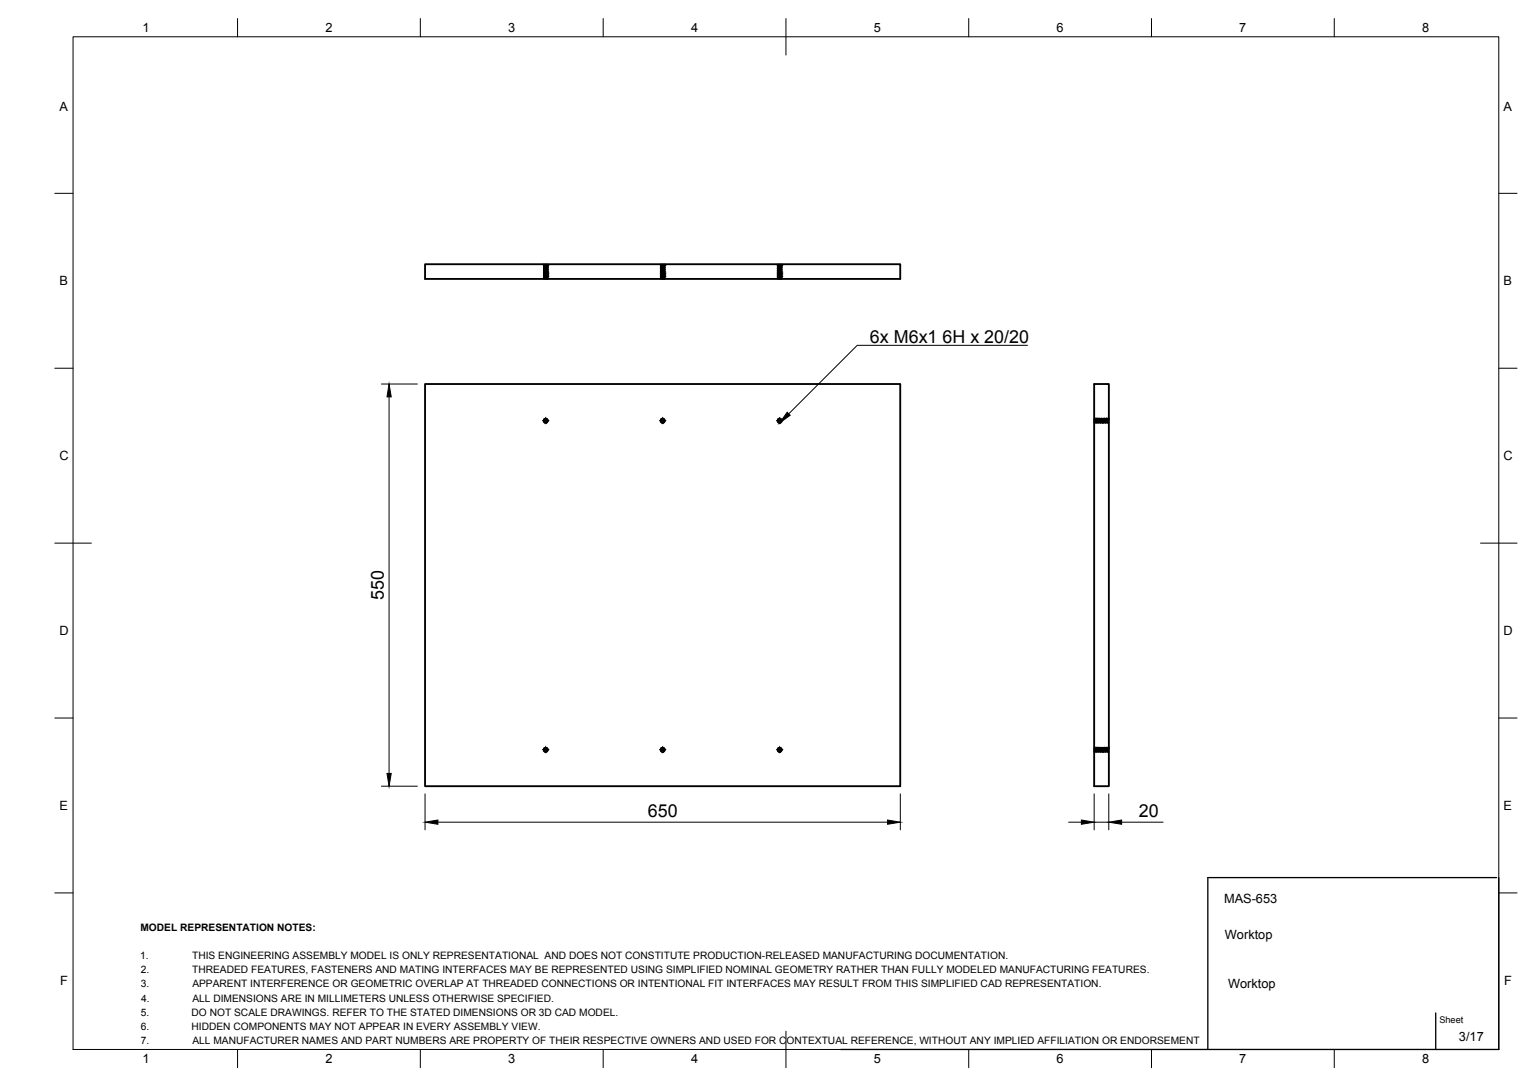
ISO-10303-21;
HEADER;
/* Generated by software containing ST-Developer
 * from STEP Tools, Inc. (www.steptools.com) 
 */

FILE_DESCRIPTION(
/* description */ ('Independent compact industrial fixture table, bolted aluminum worktop
 on connected adjustable support base. Whole-mm nominal dimensions. No
 load rating assigned.'),
/* implementation_level */ '2;1');

FILE_NAME(
/* name */ 'Worktop.step',
/* time_stamp */ '2026-11-07T17:47:58-08:00',
/* author */ (''),
/* organization */ (''),
/* preprocessor_version */ 'ST-DEVELOPER v20.2',
/* originating_system */ 'Autodesk Translation Framework v15.17.0.0',
/* authorisation */ '');

FILE_SCHEMA (('AUTOMOTIVE_DESIGN { 1 0 10303 214 3 1 1 }'));
ENDSEC;

DATA;
#10=MECHANICAL_DESIGN_GEOMETRIC_PRESENTATION_REPRESENTATION('',(#2265),#97475);
#362=B_SPLINE_SURFACE_WITH_KNOTS('',3,3,((#81643,#81644,#81645,#81646,#81647,
#81648,#81649,#81650,#81651,#81652,#81653,#81654,#81655,#81656,#81657,#81658,
#81659,#81660,#81661,#81662,#81663,#81664,#81665,#81666,#81667,#81668,#81669,
#81670,#81671,#81672,#81673,#81674,#81675,#81676,#81677,#81678,#81679,#81680,
#81681,#81682,#81683,#81684,#81685,#81686,#81687,#81688,#81689,#81690,#81691,
#81692,#81693,#81694,#81695,#81696,#81697,#81698,#81699,#81700,#81701,#81702,
#81703,#81704,#81705,#81706,#81707,#81708,#81709,#81710,#81711,#81712,#81713,
#81714,#81715,#81716,#81717,#81718,#81719,#81720,#81721,#81722,#81723,#81724,
#81725,#81726,#81727,#81728,#81729,#81730,#81731,#81732,#81733,#81734,#81735,
#81736,#81737,#81738,#81739,#81740,#81741,#81742,#81743,#81744,#81745,#81746,
#81747,#81748,#81749,#81750,#81751,#81752,#81753,#81754,#81755,#81756,#81757,
#81758,#81759,#81760,#81761,#81762,#81763,#81764,#81765,#81766,#81767,#81768,
#81769,#81770,#81771,#81772,#81773),(#81774,#81775,#81776,#81777,#81778,
#81779,#81780,#81781,#81782,#81783,#81784,#81785,#81786,#81787,#81788,#81789,
#81790,#81791,#81792,#81793,#81794,#81795,#81796,#81797,#81798,#81799,#81800,
#81801,#81802,#81803,#81804,#81805,#81806,#81807,#81808,#81809,#81810,#81811,
#81812,#81813,#81814,#81815,#81816,#81817,#81818,#81819,#81820,#81821,#81822,
#81823,#81824,#81825,#81826,#81827,#81828,#81829,#81830,#81831,#81832,#81833,
#81834,#81835,#81836,#81837,#81838,#81839,#81840,#81841,#81842,#81843,#81844,
#81845,#81846,#81847,#81848,#81849,#81850,#81851,#81852,#81853,#81854,#81855,
#81856,#81857,#81858,#81859,#81860,#81861,#81862,#81863,#81864,#81865,#81866,
#81867,#81868,#81869,#81870,#81871,#81872,#81873,#81874,#81875,#81876,#81877,
#81878,#81879,#81880,#81881,#81882,#81883,#81884,#81885,#81886,#81887,#81888,
#81889,#81890,#81891,#81892,#81893,#81894,#81895,#81896,#81897,#81898,#81899,
#81900,#81901,#81902,#81903,#81904),(#81905,#81906,#81907,#81908,#81909,
#81910,#81911,#81912,#81913,#81914,#81915,#81916,#81917,#81918,#81919,#81920,
#81921,#81922,#81923,#81924,#81925,#81926,#81927,#81928,#81929,#81930,#81931,
#81932,#81933,#81934,#81935,#81936,#81937,#81938,#81939,#81940,#81941,#81942,
#81943,#81944,#81945,#81946,#81947,#81948,#81949,#81950,#81951,#81952,#81953,
#81954,#81955,#81956,#81957,#81958,#81959,#81960,#81961,#81962,#81963,#81964,
#81965,#81966,#81967,#81968,#81969,#81970,#81971,#81972,#81973,#81974,#81975,
#81976,#81977,#81978,#81979,#81980,#81981,#81982,#81983,#81984,#81985,#81986,
#81987,#81988,#81989,#81990,#81991,#81992,#81993,#81994,#81995,#81996,#81997,
#81998,#81999,#82000,#82001,#82002,#82003,#82004,#82005,#82006,#82007,#82008,
#82009,#82010,#82011,#82012,#82013,#82014,#82015,#82016,#82017,#82018,#82019,
#82020,#82021,#82022,#82023,#82024,#82025,#82026,#82027,#82028,#82029,#82030,
#82031,#82032,#82033,#82034,#82035),(#82036,#82037,#82038,#82039,#82040,
#82041,#82042,#82043,#82044,#82045,#82046,#82047,#82048,#82049,#82050,#82051,
#82052,#82053,#82054,#82055,#82056,#82057,#82058,#82059,#82060,#82061,#82062,
#82063,#82064,#82065,#82066,#82067,#82068,#82069,#82070,#82071,#82072,#82073,
#82074,#82075,#82076,#82077,#82078,#82079,#82080,#82081,#82082,#82083,#82084,
#82085,#82086,#82087,#82088,#82089,#82090,#82091,#82092,#82093,#82094,#82095,
#82096,#82097,#82098,#82099,#82100,#82101,#82102,#82103,#82104,#82105,#82106,
#82107,#82108,#82109,#82110,#82111,#82112,#82113,#82114,#82115,#82116,#82117,
#82118,#82119,#82120,#82121,#82122,#82123,#82124,#82125,#82126,#82127,#82128,
#82129,#82130,#82131,#82132,#82133,#82134,#82135,#82136,#82137,#82138,#82139,
#82140,#82141,#82142,#82143,#82144,#82145,#82146,#82147,#82148,#82149,#82150,
#82151,#82152,#82153,#82154,#82155,#82156,#82157,#82158,#82159,#82160,#82161,
#82162,#82163,#82164,#82165,#82166)),.UNSPECIFIED.,.F.,.F.,.F.,(4,4),(4,
1,1,1,1,1,1,1,1,1,1,1,1,1,1,1,1,1,1,1,1,1,1,1,1,1,1,1,1,1,1,1,1,1,1,1,1,
1,1,1,1,1,1,1,1,1,1,1,1,1,1,1,1,1,1,1,1,1,1,1,1,1,1,1,1,1,1,1,1,1,1,1,1,
1,1,1,1,1,1,1,1,1,1,1,1,1,1,1,1,1,1,1,1,1,1,1,1,1,1,1,1,1,1,1,1,1,1,1,1,
1,1,1,1,1,1,1,1,1,1,1,1,1,1,1,1,1,1,1,4),(0.,0.0642013499338863),(11.8589888623077,
12.8564939485313,13.8539990347549,14.8515041209785,15.8490092072021,16.8465142934257,
17.8440193796493,18.8415244658729,19.8390295520965,20.8365346383201,21.8340397245437,
22.8315448107673,23.8290498969909,24.8265549832145,25.8240600694381,26.8215651556617,
27.8190702418853,28.8165753281089,29.8140804143324,30.811585500556,31.8090905867796,
32.8065956730032,33.8041007592268,34.8016058454504,35.799110931674,36.7966160178976,
37.7941211041212,38.7916261903448,39.7891312765684,40.786636362792,41.7841414490156,
42.7816465352392,43.7791516214628,44.7766567076864,45.77416179391,46.7716668801336,
47.7691719663572,48.7666770525807,49.7641821388043,50.7616872250279,51.7591923112515,
52.7566973974751,53.7542024836987,54.7517075699223,55.7492126561459,56.7467177423695,
57.7442228285931,58.7417279148167,59.7392330010403,60.7367380872639,61.7342431734875,
62.7317482597111,63.7292533459347,64.7267584321583,65.7242635183819,66.7217686046055,
67.7192736908291,68.7167787770527,69.7142838632763,70.7117889494998,71.7092940357234,
72.706799121947,73.7043042081706,74.7018092943942,75.6993143806178,76.6968194668414,
77.694324553065,78.6918296392886,79.6893347255122,80.6868398117358,81.6843448979594,
82.681849984183,83.6793550704066,84.6768601566302,85.6743652428538,86.6718703290774,
87.669375415301,88.6668805015246,89.6643855877482,90.6618906739717,91.6593957601953,
92.6569008464189,93.6544059326425,94.6519110188661,95.6494161050897,96.6469211913133,
97.6444262775369,98.6419313637605,99.6394364499841,100.636941536208,101.634446622431,
102.631951708655,103.629456794878,104.626961881102,105.624466967326,106.621972053549,
107.619477139773,108.616982225996,109.61448731222,110.611992398444,111.609497484667,
112.607002570891,113.604507657114,114.602012743338,115.599517829562,116.597022915785,
117.594528002009,118.592033088232,119.589538174456,120.58704326068,121.584548346903,
122.582053433127,123.57955851935,124.577063605574,125.574568691798,126.572073778021,
127.569578864245,128.567083950468,129.564589036692,130.562094122916,131.559599209139,
132.557104295363,133.554609381586,134.55211446781,135.549619554034,136.547124640257,
137.544629726481,138.542134812704,139.539639898928),.UNSPECIFIED.);
#363=B_SPLINE_SURFACE_WITH_KNOTS('',3,3,((#82380,#82381,#82382,#82383,#82384,
#82385,#82386,#82387,#82388,#82389,#82390,#82391,#82392,#82393,#82394,#82395,
#82396,#82397,#82398,#82399,#82400,#82401,#82402,#82403,#82404,#82405,#82406,
#82407,#82408,#82409,#82410,#82411,#82412,#82413,#82414,#82415,#82416,#82417,
#82418,#82419,#82420,#82421,#82422,#82423,#82424,#82425,#82426,#82427,#82428,
#82429,#82430,#82431,#82432,#82433,#82434,#82435,#82436,#82437,#82438,#82439,
#82440,#82441,#82442,#82443,#82444,#82445,#82446,#82447,#82448,#82449,#82450,
#82451,#82452,#82453,#82454,#82455,#82456,#82457,#82458,#82459,#82460,#82461,
#82462,#82463,#82464,#82465,#82466,#82467,#82468,#82469,#82470,#82471,#82472,
#82473,#82474,#82475,#82476,#82477,#82478,#82479,#82480,#82481,#82482,#82483,
#82484,#82485,#82486,#82487,#82488,#82489,#82490,#82491,#82492,#82493,#82494,
#82495,#82496,#82497,#82498,#82499,#82500,#82501,#82502,#82503,#82504,#82505,
#82506,#82507,#82508,#82509,#82510),(#82511,#82512,#82513,#82514,#82515,
#82516,#82517,#82518,#82519,#82520,#82521,#82522,#82523,#82524,#82525,#82526,
#82527,#82528,#82529,#82530,#82531,#82532,#82533,#82534,#82535,#82536,#82537,
#82538,#82539,#82540,#82541,#82542,#82543,#82544,#82545,#82546,#82547,#82548,
#82549,#82550,#82551,#82552,#82553,#82554,#82555,#82556,#82557,#82558,#82559,
#82560,#82561,#82562,#82563,#82564,#82565,#82566,#82567,#82568,#82569,#82570,
#82571,#82572,#82573,#82574,#82575,#82576,#82577,#82578,#82579,#82580,#82581,
#82582,#82583,#82584,#82585,#82586,#82587,#82588,#82589,#82590,#82591,#82592,
#82593,#82594,#82595,#82596,#82597,#82598,#82599,#82600,#82601,#82602,#82603,
#82604,#82605,#82606,#82607,#82608,#82609,#82610,#82611,#82612,#82613,#82614,
#82615,#82616,#82617,#82618,#82619,#82620,#82621,#82622,#82623,#82624,#82625,
#82626,#82627,#82628,#82629,#82630,#82631,#82632,#82633,#82634,#82635,#82636,
#82637,#82638,#82639,#82640,#82641),(#82642,#82643,#82644,#82645,#82646,
#82647,#82648,#82649,#82650,#82651,#82652,#82653,#82654,#82655,#82656,#82657,
#82658,#82659,#82660,#82661,#82662,#82663,#82664,#82665,#82666,#82667,#82668,
#82669,#82670,#82671,#82672,#82673,#82674,#82675,#82676,#82677,#82678,#82679,
#82680,#82681,#82682,#82683,#82684,#82685,#82686,#82687,#82688,#82689,#82690,
#82691,#82692,#82693,#82694,#82695,#82696,#82697,#82698,#82699,#82700,#82701,
#82702,#82703,#82704,#82705,#82706,#82707,#82708,#82709,#82710,#82711,#82712,
#82713,#82714,#82715,#82716,#82717,#82718,#82719,#82720,#82721,#82722,#82723,
#82724,#82725,#82726,#82727,#82728,#82729,#82730,#82731,#82732,#82733,#82734,
#82735,#82736,#82737,#82738,#82739,#82740,#82741,#82742,#82743,#82744,#82745,
#82746,#82747,#82748,#82749,#82750,#82751,#82752,#82753,#82754,#82755,#82756,
#82757,#82758,#82759,#82760,#82761,#82762,#82763,#82764,#82765,#82766,#82767,
#82768,#82769,#82770,#82771,#82772),(#82773,#82774,#82775,#82776,#82777,
#82778,#82779,#82780,#82781,#82782,#82783,#82784,#82785,#82786,#82787,#82788,
#82789,#82790,#82791,#82792,#82793,#82794,#82795,#82796,#82797,#82798,#82799,
#82800,#82801,#82802,#82803,#82804,#82805,#82806,#82807,#82808,#82809,#82810,
#82811,#82812,#82813,#82814,#82815,#82816,#82817,#82818,#82819,#82820,#82821,
#82822,#82823,#82824,#82825,#82826,#82827,#82828,#82829,#82830,#82831,#82832,
#82833,#82834,#82835,#82836,#82837,#82838,#82839,#82840,#82841,#82842,#82843,
#82844,#82845,#82846,#82847,#82848,#82849,#82850,#82851,#82852,#82853,#82854,
#82855,#82856,#82857,#82858,#82859,#82860,#82861,#82862,#82863,#82864,#82865,
#82866,#82867,#82868,#82869,#82870,#82871,#82872,#82873,#82874,#82875,#82876,
#82877,#82878,#82879,#82880,#82881,#82882,#82883,#82884,#82885,#82886,#82887,
#82888,#82889,#82890,#82891,#82892,#82893,#82894,#82895,#82896,#82897,#82898,
#82899,#82900,#82901,#82902,#82903)),.UNSPECIFIED.,.F.,.F.,.F.,(4,4),(4,
1,1,1,1,1,1,1,1,1,1,1,1,1,1,1,1,1,1,1,1,1,1,1,1,1,1,1,1,1,1,1,1,1,1,1,1,
1,1,1,1,1,1,1,1,1,1,1,1,1,1,1,1,1,1,1,1,1,1,1,1,1,1,1,1,1,1,1,1,1,1,1,1,
1,1,1,1,1,1,1,1,1,1,1,1,1,1,1,1,1,1,1,1,1,1,1,1,1,1,1,1,1,1,1,1,1,1,1,1,
1,1,1,1,1,1,1,1,1,1,1,1,1,1,1,1,1,1,1,4),(0.,0.0642013499338863),(14.3984001269718,
15.3959052131954,16.393410299419,17.3909153856426,18.3884204718662,19.3859255580897,
20.3834306443133,21.3809357305369,22.3784408167605,23.3759459029841,24.3734509892077,
25.3709560754313,26.3684611616549,27.3659662478785,28.3634713341021,29.3609764203257,
30.3584815065493,31.3559865927729,32.3534916789965,33.3509967652201,34.3485018514437,
35.3460069376673,36.3435120238909,37.3410171101145,38.3385221963381,39.3360272825616,
40.3335323687852,41.3310374550088,42.3285425412324,43.326047627456,44.3235527136796,
45.3210577999032,46.3185628861268,47.3160679723504,48.313573058574,49.3110781447976,
50.3085832310212,51.3060883172448,52.3035934034684,53.301098489692,54.2986035759156,
55.2961086621392,56.2936137483628,57.2911188345864,58.28862392081,59.2861290070336,
60.2836340932571,61.2811391794807,62.2786442657043,63.2761493519279,64.2736544381515,
65.2711595243751,66.2686646105987,67.2661696968223,68.2636747830459,69.2611798692695,
70.2586849554931,71.2561900417167,72.2536951279403,73.2512002141639,74.2487053003875,
75.2462103866111,76.2437154728347,77.2412205590583,78.2387256452818,79.2362307315055,
80.233735817729,81.2312409039526,82.2287459901762,83.2262510763998,84.2237561626234,
85.221261248847,86.2187663350706,87.2162714212942,88.2137765075178,89.2112815937414,
90.208786679965,91.2062917661886,92.2037968524122,93.2013019386358,94.1988070248594,
95.196312111083,96.1938171973066,97.1913222835302,98.1888273697538,99.1863324559774,
100.183837542201,101.181342628425,102.178847714648,103.176352800872,104.173857887095,
105.171362973319,106.168868059543,107.166373145766,108.16387823199,109.161383318213,
110.158888404437,111.15639349066,112.153898576884,113.151403663108,114.148908749331,
115.146413835555,116.143918921778,117.141424008002,118.138929094226,119.136434180449,
120.133939266673,121.131444352896,122.12894943912,123.126454525344,124.123959611567,
125.121464697791,126.118969784014,127.116474870238,128.113979956462,129.111485042685,
130.108990128909,131.106495215132,132.104000301356,133.10150538758,134.099010473803,
135.096515560027,136.09402064625,137.091525732474,138.089030818698,139.086535904921,
140.084040991145,141.081546077368,142.079051163592),.UNSPECIFIED.);
#364=B_SPLINE_SURFACE_WITH_KNOTS('',3,3,((#84085,#84086,#84087,#84088,#84089,
#84090,#84091,#84092,#84093,#84094,#84095,#84096,#84097,#84098,#84099,#84100,
#84101,#84102,#84103,#84104,#84105,#84106,#84107,#84108,#84109,#84110,#84111,
#84112,#84113,#84114,#84115,#84116,#84117,#84118,#84119,#84120,#84121,#84122,
#84123,#84124,#84125,#84126,#84127,#84128,#84129,#84130,#84131,#84132,#84133,
#84134,#84135,#84136,#84137,#84138,#84139,#84140,#84141,#84142,#84143,#84144,
#84145,#84146,#84147,#84148,#84149,#84150,#84151,#84152,#84153,#84154,#84155,
#84156,#84157,#84158,#84159,#84160,#84161,#84162,#84163,#84164,#84165,#84166,
#84167,#84168,#84169,#84170,#84171,#84172,#84173,#84174,#84175,#84176,#84177,
#84178,#84179,#84180,#84181,#84182,#84183,#84184,#84185,#84186,#84187,#84188,
#84189,#84190,#84191,#84192,#84193,#84194,#84195,#84196,#84197,#84198,#84199,
#84200,#84201,#84202,#84203,#84204,#84205,#84206,#84207,#84208,#84209,#84210,
#84211,#84212,#84213,#84214,#84215),(#84216,#84217,#84218,#84219,#84220,
#84221,#84222,#84223,#84224,#84225,#84226,#84227,#84228,#84229,#84230,#84231,
#84232,#84233,#84234,#84235,#84236,#84237,#84238,#84239,#84240,#84241,#84242,
#84243,#84244,#84245,#84246,#84247,#84248,#84249,#84250,#84251,#84252,#84253,
#84254,#84255,#84256,#84257,#84258,#84259,#84260,#84261,#84262,#84263,#84264,
#84265,#84266,#84267,#84268,#84269,#84270,#84271,#84272,#84273,#84274,#84275,
#84276,#84277,#84278,#84279,#84280,#84281,#84282,#84283,#84284,#84285,#84286,
#84287,#84288,#84289,#84290,#84291,#84292,#84293,#84294,#84295,#84296,#84297,
#84298,#84299,#84300,#84301,#84302,#84303,#84304,#84305,#84306,#84307,#84308,
#84309,#84310,#84311,#84312,#84313,#84314,#84315,#84316,#84317,#84318,#84319,
#84320,#84321,#84322,#84323,#84324,#84325,#84326,#84327,#84328,#84329,#84330,
#84331,#84332,#84333,#84334,#84335,#84336,#84337,#84338,#84339,#84340,#84341,
#84342,#84343,#84344,#84345,#84346),(#84347,#84348,#84349,#84350,#84351,
#84352,#84353,#84354,#84355,#84356,#84357,#84358,#84359,#84360,#84361,#84362,
#84363,#84364,#84365,#84366,#84367,#84368,#84369,#84370,#84371,#84372,#84373,
#84374,#84375,#84376,#84377,#84378,#84379,#84380,#84381,#84382,#84383,#84384,
#84385,#84386,#84387,#84388,#84389,#84390,#84391,#84392,#84393,#84394,#84395,
#84396,#84397,#84398,#84399,#84400,#84401,#84402,#84403,#84404,#84405,#84406,
#84407,#84408,#84409,#84410,#84411,#84412,#84413,#84414,#84415,#84416,#84417,
#84418,#84419,#84420,#84421,#84422,#84423,#84424,#84425,#84426,#84427,#84428,
#84429,#84430,#84431,#84432,#84433,#84434,#84435,#84436,#84437,#84438,#84439,
#84440,#84441,#84442,#84443,#84444,#84445,#84446,#84447,#84448,#84449,#84450,
#84451,#84452,#84453,#84454,#84455,#84456,#84457,#84458,#84459,#84460,#84461,
#84462,#84463,#84464,#84465,#84466,#84467,#84468,#84469,#84470,#84471,#84472,
#84473,#84474,#84475,#84476,#84477),(#84478,#84479,#84480,#84481,#84482,
#84483,#84484,#84485,#84486,#84487,#84488,#84489,#84490,#84491,#84492,#84493,
#84494,#84495,#84496,#84497,#84498,#84499,#84500,#84501,#84502,#84503,#84504,
#84505,#84506,#84507,#84508,#84509,#84510,#84511,#84512,#84513,#84514,#84515,
#84516,#84517,#84518,#84519,#84520,#84521,#84522,#84523,#84524,#84525,#84526,
#84527,#84528,#84529,#84530,#84531,#84532,#84533,#84534,#84535,#84536,#84537,
#84538,#84539,#84540,#84541,#84542,#84543,#84544,#84545,#84546,#84547,#84548,
#84549,#84550,#84551,#84552,#84553,#84554,#84555,#84556,#84557,#84558,#84559,
#84560,#84561,#84562,#84563,#84564,#84565,#84566,#84567,#84568,#84569,#84570,
#84571,#84572,#84573,#84574,#84575,#84576,#84577,#84578,#84579,#84580,#84581,
#84582,#84583,#84584,#84585,#84586,#84587,#84588,#84589,#84590,#84591,#84592,
#84593,#84594,#84595,#84596,#84597,#84598,#84599,#84600,#84601,#84602,#84603,
#84604,#84605,#84606,#84607,#84608)),.UNSPECIFIED.,.F.,.F.,.F.,(4,4),(4,
1,1,1,1,1,1,1,1,1,1,1,1,1,1,1,1,1,1,1,1,1,1,1,1,1,1,1,1,1,1,1,1,1,1,1,1,
1,1,1,1,1,1,1,1,1,1,1,1,1,1,1,1,1,1,1,1,1,1,1,1,1,1,1,1,1,1,1,1,1,1,1,1,
1,1,1,1,1,1,1,1,1,1,1,1,1,1,1,1,1,1,1,1,1,1,1,1,1,1,1,1,1,1,1,1,1,1,1,1,
1,1,1,1,1,1,1,1,1,1,1,1,1,1,1,1,1,1,1,4),(0.,0.0642013499338864),(11.8589888623077,
12.8564939485313,13.8539990347549,14.8515041209785,15.8490092072021,16.8465142934257,
17.8440193796493,18.8415244658729,19.8390295520965,20.8365346383201,21.8340397245437,
22.8315448107673,23.8290498969909,24.8265549832144,25.824060069438,26.8215651556616,
27.8190702418852,28.8165753281088,29.8140804143324,30.811585500556,31.8090905867796,
32.8065956730032,33.8041007592268,34.8016058454504,35.799110931674,36.7966160178976,
37.7941211041212,38.7916261903448,39.7891312765684,40.786636362792,41.7841414490156,
42.7816465352392,43.7791516214628,44.7766567076863,45.7741617939099,46.7716668801335,
47.7691719663571,48.7666770525807,49.7641821388043,50.7616872250279,51.7591923112515,
52.7566973974751,53.7542024836987,54.7517075699223,55.7492126561459,56.7467177423695,
57.7442228285931,58.7417279148167,59.7392330010403,60.7367380872639,61.7342431734875,
62.7317482597111,63.7292533459347,64.7267584321582,65.7242635183818,66.7217686046054,
67.719273690829,68.7167787770526,69.7142838632762,70.7117889494998,71.7092940357234,
72.706799121947,73.7043042081706,74.7018092943942,75.6993143806178,76.6968194668414,
77.694324553065,78.6918296392886,79.6893347255122,80.6868398117358,81.6843448979594,
82.681849984183,83.6793550704066,84.6768601566301,85.6743652428537,86.6718703290773,
87.6693754153009,88.6668805015245,89.6643855877481,90.6618906739717,91.6593957601953,
92.6569008464189,93.6544059326425,94.6519110188661,95.6494161050897,96.6469211913133,
97.6444262775369,98.6419313637605,99.6394364499841,100.636941536208,101.634446622431,
102.631951708655,103.629456794878,104.626961881102,105.624466967326,106.621972053549,
107.619477139773,108.616982225996,109.61448731222,110.611992398444,111.609497484667,
112.607002570891,113.604507657114,114.602012743338,115.599517829562,116.597022915785,
117.594528002009,118.592033088232,119.589538174456,120.58704326068,121.584548346903,
122.582053433127,123.57955851935,124.577063605574,125.574568691798,126.572073778021,
127.569578864245,128.567083950468,129.564589036692,130.562094122916,131.559599209139,
132.557104295363,133.554609381586,134.55211446781,135.549619554033,136.547124640257,
137.544629726481,138.542134812704,139.539639898928),.UNSPECIFIED.);
#365=B_SPLINE_SURFACE_WITH_KNOTS('',3,3,((#84728,#84729,#84730,#84731,#84732,
#84733,#84734,#84735,#84736,#84737,#84738,#84739,#84740,#84741,#84742,#84743,
#84744,#84745,#84746,#84747,#84748,#84749,#84750,#84751,#84752,#84753,#84754,
#84755,#84756,#84757,#84758,#84759,#84760,#84761,#84762,#84763,#84764,#84765,
#84766,#84767,#84768,#84769,#84770,#84771,#84772,#84773,#84774,#84775,#84776,
#84777,#84778,#84779,#84780,#84781,#84782,#84783,#84784,#84785,#84786,#84787,
#84788,#84789,#84790,#84791,#84792,#84793,#84794,#84795,#84796,#84797,#84798,
#84799,#84800,#84801,#84802,#84803,#84804,#84805,#84806,#84807,#84808,#84809,
#84810,#84811,#84812,#84813,#84814,#84815,#84816,#84817,#84818,#84819,#84820,
#84821,#84822,#84823,#84824,#84825,#84826,#84827,#84828,#84829,#84830,#84831,
#84832,#84833,#84834,#84835,#84836,#84837,#84838,#84839,#84840,#84841,#84842,
#84843,#84844,#84845,#84846,#84847,#84848,#84849,#84850,#84851,#84852,#84853,
#84854,#84855,#84856,#84857,#84858),(#84859,#84860,#84861,#84862,#84863,
#84864,#84865,#84866,#84867,#84868,#84869,#84870,#84871,#84872,#84873,#84874,
#84875,#84876,#84877,#84878,#84879,#84880,#84881,#84882,#84883,#84884,#84885,
#84886,#84887,#84888,#84889,#84890,#84891,#84892,#84893,#84894,#84895,#84896,
#84897,#84898,#84899,#84900,#84901,#84902,#84903,#84904,#84905,#84906,#84907,
#84908,#84909,#84910,#84911,#84912,#84913,#84914,#84915,#84916,#84917,#84918,
#84919,#84920,#84921,#84922,#84923,#84924,#84925,#84926,#84927,#84928,#84929,
#84930,#84931,#84932,#84933,#84934,#84935,#84936,#84937,#84938,#84939,#84940,
#84941,#84942,#84943,#84944,#84945,#84946,#84947,#84948,#84949,#84950,#84951,
#84952,#84953,#84954,#84955,#84956,#84957,#84958,#84959,#84960,#84961,#84962,
#84963,#84964,#84965,#84966,#84967,#84968,#84969,#84970,#84971,#84972,#84973,
#84974,#84975,#84976,#84977,#84978,#84979,#84980,#84981,#84982,#84983,#84984,
#84985,#84986,#84987,#84988,#84989),(#84990,#84991,#84992,#84993,#84994,
#84995,#84996,#84997,#84998,#84999,#85000,#85001,#85002,#85003,#85004,#85005,
#85006,#85007,#85008,#85009,#85010,#85011,#85012,#85013,#85014,#85015,#85016,
#85017,#85018,#85019,#85020,#85021,#85022,#85023,#85024,#85025,#85026,#85027,
#85028,#85029,#85030,#85031,#85032,#85033,#85034,#85035,#85036,#85037,#85038,
#85039,#85040,#85041,#85042,#85043,#85044,#85045,#85046,#85047,#85048,#85049,
#85050,#85051,#85052,#85053,#85054,#85055,#85056,#85057,#85058,#85059,#85060,
#85061,#85062,#85063,#85064,#85065,#85066,#85067,#85068,#85069,#85070,#85071,
#85072,#85073,#85074,#85075,#85076,#85077,#85078,#85079,#85080,#85081,#85082,
#85083,#85084,#85085,#85086,#85087,#85088,#85089,#85090,#85091,#85092,#85093,
#85094,#85095,#85096,#85097,#85098,#85099,#85100,#85101,#85102,#85103,#85104,
#85105,#85106,#85107,#85108,#85109,#85110,#85111,#85112,#85113,#85114,#85115,
#85116,#85117,#85118,#85119,#85120),(#85121,#85122,#85123,#85124,#85125,
#85126,#85127,#85128,#85129,#85130,#85131,#85132,#85133,#85134,#85135,#85136,
#85137,#85138,#85139,#85140,#85141,#85142,#85143,#85144,#85145,#85146,#85147,
#85148,#85149,#85150,#85151,#85152,#85153,#85154,#85155,#85156,#85157,#85158,
#85159,#85160,#85161,#85162,#85163,#85164,#85165,#85166,#85167,#85168,#85169,
#85170,#85171,#85172,#85173,#85174,#85175,#85176,#85177,#85178,#85179,#85180,
#85181,#85182,#85183,#85184,#85185,#85186,#85187,#85188,#85189,#85190,#85191,
#85192,#85193,#85194,#85195,#85196,#85197,#85198,#85199,#85200,#85201,#85202,
#85203,#85204,#85205,#85206,#85207,#85208,#85209,#85210,#85211,#85212,#85213,
#85214,#85215,#85216,#85217,#85218,#85219,#85220,#85221,#85222,#85223,#85224,
#85225,#85226,#85227,#85228,#85229,#85230,#85231,#85232,#85233,#85234,#85235,
#85236,#85237,#85238,#85239,#85240,#85241,#85242,#85243,#85244,#85245,#85246,
#85247,#85248,#85249,#85250,#85251)),.UNSPECIFIED.,.F.,.F.,.F.,(4,4),(4,
1,1,1,1,1,1,1,1,1,1,1,1,1,1,1,1,1,1,1,1,1,1,1,1,1,1,1,1,1,1,1,1,1,1,1,1,
1,1,1,1,1,1,1,1,1,1,1,1,1,1,1,1,1,1,1,1,1,1,1,1,1,1,1,1,1,1,1,1,1,1,1,1,
1,1,1,1,1,1,1,1,1,1,1,1,1,1,1,1,1,1,1,1,1,1,1,1,1,1,1,1,1,1,1,1,1,1,1,1,
1,1,1,1,1,1,1,1,1,1,1,1,1,1,1,1,1,1,1,4),(0.,0.0642013499338864),(14.3984001269717,
15.3959052131953,16.3934102994189,17.3909153856425,18.3884204718661,19.3859255580897,
20.3834306443133,21.3809357305369,22.3784408167605,23.3759459029841,24.3734509892077,
25.3709560754313,26.3684611616549,27.3659662478785,28.3634713341021,29.3609764203257,
30.3584815065493,31.3559865927729,32.3534916789965,33.3509967652201,34.3485018514437,
35.3460069376672,36.3435120238908,37.3410171101144,38.338522196338,39.3360272825616,
40.3335323687852,41.3310374550088,42.3285425412324,43.326047627456,44.3235527136796,
45.3210577999032,46.3185628861268,47.3160679723504,48.313573058574,49.3110781447976,
50.3085832310212,51.3060883172448,52.3035934034684,53.301098489692,54.2986035759156,
55.2961086621392,56.2936137483628,57.2911188345863,58.2886239208099,59.2861290070335,
60.2836340932571,61.2811391794807,62.2786442657043,63.2761493519279,64.2736544381515,
65.2711595243751,66.2686646105987,67.2661696968223,68.2636747830459,69.2611798692695,
70.2586849554931,71.2561900417167,72.2536951279403,73.2512002141639,74.2487053003875,
75.2462103866111,76.2437154728347,77.2412205590582,78.2387256452818,79.2362307315054,
80.233735817729,81.2312409039526,82.2287459901762,83.2262510763998,84.2237561626234,
85.221261248847,86.2187663350706,87.2162714212942,88.2137765075178,89.2112815937414,
90.208786679965,91.2062917661886,92.2037968524122,93.2013019386358,94.1988070248594,
95.196312111083,96.1938171973066,97.1913222835302,98.1888273697538,99.1863324559773,
100.183837542201,101.181342628425,102.178847714648,103.176352800872,104.173857887095,
105.171362973319,106.168868059543,107.166373145766,108.16387823199,109.161383318213,
110.158888404437,111.15639349066,112.153898576884,113.151403663108,114.148908749331,
115.146413835555,116.143918921778,117.141424008002,118.138929094226,119.136434180449,
120.133939266673,121.131444352896,122.12894943912,123.126454525344,124.123959611567,
125.121464697791,126.118969784014,127.116474870238,128.113979956462,129.111485042685,
130.108990128909,131.106495215132,132.104000301356,133.10150538758,134.099010473803,
135.096515560027,136.09402064625,137.091525732474,138.089030818698,139.086535904921,
140.084040991145,141.081546077368,142.079051163592),.UNSPECIFIED.);
#366=B_SPLINE_SURFACE_WITH_KNOTS('',3,3,((#85390,#85391,#85392,#85393,#85394,
#85395,#85396,#85397,#85398,#85399,#85400,#85401,#85402,#85403,#85404,#85405,
#85406,#85407,#85408,#85409,#85410,#85411,#85412,#85413,#85414,#85415,#85416,
#85417,#85418,#85419,#85420,#85421,#85422,#85423,#85424,#85425,#85426,#85427,
#85428,#85429,#85430,#85431,#85432,#85433,#85434,#85435,#85436,#85437,#85438,
#85439,#85440,#85441,#85442,#85443,#85444,#85445,#85446,#85447,#85448,#85449,
#85450,#85451,#85452,#85453,#85454,#85455,#85456,#85457,#85458,#85459,#85460,
#85461,#85462,#85463,#85464,#85465,#85466,#85467,#85468,#85469,#85470,#85471,
#85472,#85473,#85474,#85475,#85476,#85477,#85478,#85479,#85480,#85481,#85482,
#85483,#85484,#85485,#85486,#85487,#85488,#85489,#85490,#85491,#85492,#85493,
#85494,#85495,#85496,#85497,#85498,#85499,#85500,#85501,#85502,#85503,#85504,
#85505,#85506,#85507,#85508,#85509,#85510,#85511,#85512,#85513,#85514,#85515,
#85516,#85517,#85518,#85519,#85520),(#85521,#85522,#85523,#85524,#85525,
#85526,#85527,#85528,#85529,#85530,#85531,#85532,#85533,#85534,#85535,#85536,
#85537,#85538,#85539,#85540,#85541,#85542,#85543,#85544,#85545,#85546,#85547,
#85548,#85549,#85550,#85551,#85552,#85553,#85554,#85555,#85556,#85557,#85558,
#85559,#85560,#85561,#85562,#85563,#85564,#85565,#85566,#85567,#85568,#85569,
#85570,#85571,#85572,#85573,#85574,#85575,#85576,#85577,#85578,#85579,#85580,
#85581,#85582,#85583,#85584,#85585,#85586,#85587,#85588,#85589,#85590,#85591,
#85592,#85593,#85594,#85595,#85596,#85597,#85598,#85599,#85600,#85601,#85602,
#85603,#85604,#85605,#85606,#85607,#85608,#85609,#85610,#85611,#85612,#85613,
#85614,#85615,#85616,#85617,#85618,#85619,#85620,#85621,#85622,#85623,#85624,
#85625,#85626,#85627,#85628,#85629,#85630,#85631,#85632,#85633,#85634,#85635,
#85636,#85637,#85638,#85639,#85640,#85641,#85642,#85643,#85644,#85645,#85646,
#85647,#85648,#85649,#85650,#85651),(#85652,#85653,#85654,#85655,#85656,
#85657,#85658,#85659,#85660,#85661,#85662,#85663,#85664,#85665,#85666,#85667,
#85668,#85669,#85670,#85671,#85672,#85673,#85674,#85675,#85676,#85677,#85678,
#85679,#85680,#85681,#85682,#85683,#85684,#85685,#85686,#85687,#85688,#85689,
#85690,#85691,#85692,#85693,#85694,#85695,#85696,#85697,#85698,#85699,#85700,
#85701,#85702,#85703,#85704,#85705,#85706,#85707,#85708,#85709,#85710,#85711,
#85712,#85713,#85714,#85715,#85716,#85717,#85718,#85719,#85720,#85721,#85722,
#85723,#85724,#85725,#85726,#85727,#85728,#85729,#85730,#85731,#85732,#85733,
#85734,#85735,#85736,#85737,#85738,#85739,#85740,#85741,#85742,#85743,#85744,
#85745,#85746,#85747,#85748,#85749,#85750,#85751,#85752,#85753,#85754,#85755,
#85756,#85757,#85758,#85759,#85760,#85761,#85762,#85763,#85764,#85765,#85766,
#85767,#85768,#85769,#85770,#85771,#85772,#85773,#85774,#85775,#85776,#85777,
#85778,#85779,#85780,#85781,#85782),(#85783,#85784,#85785,#85786,#85787,
#85788,#85789,#85790,#85791,#85792,#85793,#85794,#85795,#85796,#85797,#85798,
#85799,#85800,#85801,#85802,#85803,#85804,#85805,#85806,#85807,#85808,#85809,
#85810,#85811,#85812,#85813,#85814,#85815,#85816,#85817,#85818,#85819,#85820,
#85821,#85822,#85823,#85824,#85825,#85826,#85827,#85828,#85829,#85830,#85831,
#85832,#85833,#85834,#85835,#85836,#85837,#85838,#85839,#85840,#85841,#85842,
#85843,#85844,#85845,#85846,#85847,#85848,#85849,#85850,#85851,#85852,#85853,
#85854,#85855,#85856,#85857,#85858,#85859,#85860,#85861,#85862,#85863,#85864,
#85865,#85866,#85867,#85868,#85869,#85870,#85871,#85872,#85873,#85874,#85875,
#85876,#85877,#85878,#85879,#85880,#85881,#85882,#85883,#85884,#85885,#85886,
#85887,#85888,#85889,#85890,#85891,#85892,#85893,#85894,#85895,#85896,#85897,
#85898,#85899,#85900,#85901,#85902,#85903,#85904,#85905,#85906,#85907,#85908,
#85909,#85910,#85911,#85912,#85913)),.UNSPECIFIED.,.F.,.F.,.F.,(4,4),(4,
1,1,1,1,1,1,1,1,1,1,1,1,1,1,1,1,1,1,1,1,1,1,1,1,1,1,1,1,1,1,1,1,1,1,1,1,
1,1,1,1,1,1,1,1,1,1,1,1,1,1,1,1,1,1,1,1,1,1,1,1,1,1,1,1,1,1,1,1,1,1,1,1,
1,1,1,1,1,1,1,1,1,1,1,1,1,1,1,1,1,1,1,1,1,1,1,1,1,1,1,1,1,1,1,1,1,1,1,1,
1,1,1,1,1,1,1,1,1,1,1,1,1,1,1,1,1,1,1,4),(0.,0.0642013499338879),(11.8589888623077,
12.8564939485313,13.8539990347549,14.8515041209785,15.8490092072021,16.8465142934257,
17.8440193796493,18.8415244658729,19.8390295520965,20.8365346383201,21.8340397245437,
22.8315448107673,23.8290498969909,24.8265549832145,25.8240600694381,26.8215651556617,
27.8190702418853,28.8165753281089,29.8140804143324,30.811585500556,31.8090905867796,
32.8065956730032,33.8041007592268,34.8016058454504,35.799110931674,36.7966160178976,
37.7941211041212,38.7916261903448,39.7891312765684,40.786636362792,41.7841414490156,
42.7816465352392,43.7791516214628,44.7766567076864,45.77416179391,46.7716668801336,
47.7691719663572,48.7666770525808,49.7641821388044,50.7616872250279,51.7591923112515,
52.7566973974751,53.7542024836987,54.7517075699223,55.7492126561459,56.7467177423695,
57.7442228285931,58.7417279148167,59.7392330010403,60.7367380872639,61.7342431734875,
62.7317482597111,63.7292533459347,64.7267584321583,65.7242635183819,66.7217686046055,
67.7192736908291,68.7167787770527,69.7142838632763,70.7117889494998,71.7092940357234,
72.706799121947,73.7043042081706,74.7018092943942,75.6993143806178,76.6968194668414,
77.694324553065,78.6918296392886,79.6893347255122,80.6868398117358,81.6843448979594,
82.681849984183,83.6793550704066,84.6768601566302,85.6743652428538,86.6718703290774,
87.669375415301,88.6668805015246,89.6643855877482,90.6618906739718,91.6593957601954,
92.6569008464189,93.6544059326425,94.6519110188661,95.6494161050897,96.6469211913133,
97.6444262775369,98.6419313637605,99.6394364499841,100.636941536208,101.634446622431,
102.631951708655,103.629456794878,104.626961881102,105.624466967326,106.621972053549,
107.619477139773,108.616982225996,109.61448731222,110.611992398444,111.609497484667,
112.607002570891,113.604507657114,114.602012743338,115.599517829562,116.597022915785,
117.594528002009,118.592033088232,119.589538174456,120.58704326068,121.584548346903,
122.582053433127,123.57955851935,124.577063605574,125.574568691798,126.572073778021,
127.569578864245,128.567083950468,129.564589036692,130.562094122916,131.559599209139,
132.557104295363,133.554609381586,134.55211446781,135.549619554034,136.547124640257,
137.544629726481,138.542134812704,139.539639898928),.UNSPECIFIED.);
#367=B_SPLINE_SURFACE_WITH_KNOTS('',3,3,((#86033,#86034,#86035,#86036,#86037,
#86038,#86039,#86040,#86041,#86042,#86043,#86044,#86045,#86046,#86047,#86048,
#86049,#86050,#86051,#86052,#86053,#86054,#86055,#86056,#86057,#86058,#86059,
#86060,#86061,#86062,#86063,#86064,#86065,#86066,#86067,#86068,#86069,#86070,
#86071,#86072,#86073,#86074,#86075,#86076,#86077,#86078,#86079,#86080,#86081,
#86082,#86083,#86084,#86085,#86086,#86087,#86088,#86089,#86090,#86091,#86092,
#86093,#86094,#86095,#86096,#86097,#86098,#86099,#86100,#86101,#86102,#86103,
#86104,#86105,#86106,#86107,#86108,#86109,#86110,#86111,#86112,#86113,#86114,
#86115,#86116,#86117,#86118,#86119,#86120,#86121,#86122,#86123,#86124,#86125,
#86126,#86127,#86128,#86129,#86130,#86131,#86132,#86133,#86134,#86135,#86136,
#86137,#86138,#86139,#86140,#86141,#86142,#86143,#86144,#86145,#86146,#86147,
#86148,#86149,#86150,#86151,#86152,#86153,#86154,#86155,#86156,#86157,#86158,
#86159,#86160,#86161,#86162,#86163),(#86164,#86165,#86166,#86167,#86168,
#86169,#86170,#86171,#86172,#86173,#86174,#86175,#86176,#86177,#86178,#86179,
#86180,#86181,#86182,#86183,#86184,#86185,#86186,#86187,#86188,#86189,#86190,
#86191,#86192,#86193,#86194,#86195,#86196,#86197,#86198,#86199,#86200,#86201,
#86202,#86203,#86204,#86205,#86206,#86207,#86208,#86209,#86210,#86211,#86212,
#86213,#86214,#86215,#86216,#86217,#86218,#86219,#86220,#86221,#86222,#86223,
#86224,#86225,#86226,#86227,#86228,#86229,#86230,#86231,#86232,#86233,#86234,
#86235,#86236,#86237,#86238,#86239,#86240,#86241,#86242,#86243,#86244,#86245,
#86246,#86247,#86248,#86249,#86250,#86251,#86252,#86253,#86254,#86255,#86256,
#86257,#86258,#86259,#86260,#86261,#86262,#86263,#86264,#86265,#86266,#86267,
#86268,#86269,#86270,#86271,#86272,#86273,#86274,#86275,#86276,#86277,#86278,
#86279,#86280,#86281,#86282,#86283,#86284,#86285,#86286,#86287,#86288,#86289,
#86290,#86291,#86292,#86293,#86294),(#86295,#86296,#86297,#86298,#86299,
#86300,#86301,#86302,#86303,#86304,#86305,#86306,#86307,#86308,#86309,#86310,
#86311,#86312,#86313,#86314,#86315,#86316,#86317,#86318,#86319,#86320,#86321,
#86322,#86323,#86324,#86325,#86326,#86327,#86328,#86329,#86330,#86331,#86332,
#86333,#86334,#86335,#86336,#86337,#86338,#86339,#86340,#86341,#86342,#86343,
#86344,#86345,#86346,#86347,#86348,#86349,#86350,#86351,#86352,#86353,#86354,
#86355,#86356,#86357,#86358,#86359,#86360,#86361,#86362,#86363,#86364,#86365,
#86366,#86367,#86368,#86369,#86370,#86371,#86372,#86373,#86374,#86375,#86376,
#86377,#86378,#86379,#86380,#86381,#86382,#86383,#86384,#86385,#86386,#86387,
#86388,#86389,#86390,#86391,#86392,#86393,#86394,#86395,#86396,#86397,#86398,
#86399,#86400,#86401,#86402,#86403,#86404,#86405,#86406,#86407,#86408,#86409,
#86410,#86411,#86412,#86413,#86414,#86415,#86416,#86417,#86418,#86419,#86420,
#86421,#86422,#86423,#86424,#86425),(#86426,#86427,#86428,#86429,#86430,
#86431,#86432,#86433,#86434,#86435,#86436,#86437,#86438,#86439,#86440,#86441,
#86442,#86443,#86444,#86445,#86446,#86447,#86448,#86449,#86450,#86451,#86452,
#86453,#86454,#86455,#86456,#86457,#86458,#86459,#86460,#86461,#86462,#86463,
#86464,#86465,#86466,#86467,#86468,#86469,#86470,#86471,#86472,#86473,#86474,
#86475,#86476,#86477,#86478,#86479,#86480,#86481,#86482,#86483,#86484,#86485,
#86486,#86487,#86488,#86489,#86490,#86491,#86492,#86493,#86494,#86495,#86496,
#86497,#86498,#86499,#86500,#86501,#86502,#86503,#86504,#86505,#86506,#86507,
#86508,#86509,#86510,#86511,#86512,#86513,#86514,#86515,#86516,#86517,#86518,
#86519,#86520,#86521,#86522,#86523,#86524,#86525,#86526,#86527,#86528,#86529,
#86530,#86531,#86532,#86533,#86534,#86535,#86536,#86537,#86538,#86539,#86540,
#86541,#86542,#86543,#86544,#86545,#86546,#86547,#86548,#86549,#86550,#86551,
#86552,#86553,#86554,#86555,#86556)),.UNSPECIFIED.,.F.,.F.,.F.,(4,4),(4,
1,1,1,1,1,1,1,1,1,1,1,1,1,1,1,1,1,1,1,1,1,1,1,1,1,1,1,1,1,1,1,1,1,1,1,1,
1,1,1,1,1,1,1,1,1,1,1,1,1,1,1,1,1,1,1,1,1,1,1,1,1,1,1,1,1,1,1,1,1,1,1,1,
1,1,1,1,1,1,1,1,1,1,1,1,1,1,1,1,1,1,1,1,1,1,1,1,1,1,1,1,1,1,1,1,1,1,1,1,
1,1,1,1,1,1,1,1,1,1,1,1,1,1,1,1,1,1,1,4),(0.,0.0642013499338879),(14.3984001269718,
15.3959052131954,16.393410299419,17.3909153856426,18.3884204718662,19.3859255580897,
20.3834306443133,21.3809357305369,22.3784408167605,23.3759459029841,24.3734509892077,
25.3709560754313,26.3684611616549,27.3659662478785,28.3634713341021,29.3609764203257,
30.3584815065493,31.3559865927729,32.3534916789965,33.3509967652201,34.3485018514437,
35.3460069376673,36.3435120238909,37.3410171101145,38.3385221963381,39.3360272825617,
40.3335323687852,41.3310374550088,42.3285425412324,43.326047627456,44.3235527136796,
45.3210577999032,46.3185628861268,47.3160679723504,48.313573058574,49.3110781447976,
50.3085832310212,51.3060883172448,52.3035934034684,53.301098489692,54.2986035759156,
55.2961086621392,56.2936137483628,57.2911188345864,58.28862392081,59.2861290070336,
60.2836340932571,61.2811391794807,62.2786442657043,63.2761493519279,64.2736544381515,
65.2711595243751,66.2686646105987,67.2661696968223,68.2636747830459,69.2611798692695,
70.2586849554931,71.2561900417167,72.2536951279403,73.2512002141639,74.2487053003875,
75.2462103866111,76.2437154728347,77.2412205590583,78.2387256452819,79.2362307315055,
80.2337358177291,81.2312409039526,82.2287459901762,83.2262510763998,84.2237561626234,
85.221261248847,86.2187663350706,87.2162714212942,88.2137765075178,89.2112815937414,
90.208786679965,91.2062917661886,92.2037968524122,93.2013019386358,94.1988070248594,
95.196312111083,96.1938171973066,97.1913222835302,98.1888273697538,99.1863324559774,
100.183837542201,101.181342628425,102.178847714648,103.176352800872,104.173857887095,
105.171362973319,106.168868059543,107.166373145766,108.16387823199,109.161383318213,
110.158888404437,111.15639349066,112.153898576884,113.151403663108,114.148908749331,
115.146413835555,116.143918921778,117.141424008002,118.138929094226,119.136434180449,
120.133939266673,121.131444352896,122.12894943912,123.126454525344,124.123959611567,
125.121464697791,126.118969784014,127.116474870238,128.113979956462,129.111485042685,
130.108990128909,131.106495215132,132.104000301356,133.10150538758,134.099010473803,
135.096515560027,136.09402064625,137.091525732474,138.089030818698,139.086535904921,
140.084040991145,141.081546077368,142.079051163592),.UNSPECIFIED.);
#368=B_SPLINE_SURFACE_WITH_KNOTS('',3,3,((#86695,#86696,#86697,#86698,#86699,
#86700,#86701,#86702,#86703,#86704,#86705,#86706,#86707,#86708,#86709,#86710,
#86711,#86712,#86713,#86714,#86715,#86716,#86717,#86718,#86719,#86720,#86721,
#86722,#86723,#86724,#86725,#86726,#86727,#86728,#86729,#86730,#86731,#86732,
#86733,#86734,#86735,#86736,#86737,#86738,#86739,#86740,#86741,#86742,#86743,
#86744,#86745,#86746,#86747,#86748,#86749,#86750,#86751,#86752,#86753,#86754,
#86755,#86756,#86757,#86758,#86759,#86760,#86761,#86762,#86763,#86764,#86765,
#86766,#86767,#86768,#86769,#86770,#86771,#86772,#86773,#86774,#86775,#86776,
#86777,#86778,#86779,#86780,#86781,#86782,#86783,#86784,#86785,#86786,#86787,
#86788,#86789,#86790,#86791,#86792,#86793,#86794,#86795,#86796,#86797,#86798,
#86799,#86800,#86801,#86802,#86803,#86804,#86805,#86806,#86807,#86808,#86809,
#86810,#86811,#86812,#86813,#86814,#86815,#86816,#86817,#86818,#86819,#86820,
#86821,#86822,#86823,#86824,#86825),(#86826,#86827,#86828,#86829,#86830,
#86831,#86832,#86833,#86834,#86835,#86836,#86837,#86838,#86839,#86840,#86841,
#86842,#86843,#86844,#86845,#86846,#86847,#86848,#86849,#86850,#86851,#86852,
#86853,#86854,#86855,#86856,#86857,#86858,#86859,#86860,#86861,#86862,#86863,
#86864,#86865,#86866,#86867,#86868,#86869,#86870,#86871,#86872,#86873,#86874,
#86875,#86876,#86877,#86878,#86879,#86880,#86881,#86882,#86883,#86884,#86885,
#86886,#86887,#86888,#86889,#86890,#86891,#86892,#86893,#86894,#86895,#86896,
#86897,#86898,#86899,#86900,#86901,#86902,#86903,#86904,#86905,#86906,#86907,
#86908,#86909,#86910,#86911,#86912,#86913,#86914,#86915,#86916,#86917,#86918,
#86919,#86920,#86921,#86922,#86923,#86924,#86925,#86926,#86927,#86928,#86929,
#86930,#86931,#86932,#86933,#86934,#86935,#86936,#86937,#86938,#86939,#86940,
#86941,#86942,#86943,#86944,#86945,#86946,#86947,#86948,#86949,#86950,#86951,
#86952,#86953,#86954,#86955,#86956),(#86957,#86958,#86959,#86960,#86961,
#86962,#86963,#86964,#86965,#86966,#86967,#86968,#86969,#86970,#86971,#86972,
#86973,#86974,#86975,#86976,#86977,#86978,#86979,#86980,#86981,#86982,#86983,
#86984,#86985,#86986,#86987,#86988,#86989,#86990,#86991,#86992,#86993,#86994,
#86995,#86996,#86997,#86998,#86999,#87000,#87001,#87002,#87003,#87004,#87005,
#87006,#87007,#87008,#87009,#87010,#87011,#87012,#87013,#87014,#87015,#87016,
#87017,#87018,#87019,#87020,#87021,#87022,#87023,#87024,#87025,#87026,#87027,
#87028,#87029,#87030,#87031,#87032,#87033,#87034,#87035,#87036,#87037,#87038,
#87039,#87040,#87041,#87042,#87043,#87044,#87045,#87046,#87047,#87048,#87049,
#87050,#87051,#87052,#87053,#87054,#87055,#87056,#87057,#87058,#87059,#87060,
#87061,#87062,#87063,#87064,#87065,#87066,#87067,#87068,#87069,#87070,#87071,
#87072,#87073,#87074,#87075,#87076,#87077,#87078,#87079,#87080,#87081,#87082,
#87083,#87084,#87085,#87086,#87087),(#87088,#87089,#87090,#87091,#87092,
#87093,#87094,#87095,#87096,#87097,#87098,#87099,#87100,#87101,#87102,#87103,
#87104,#87105,#87106,#87107,#87108,#87109,#87110,#87111,#87112,#87113,#87114,
#87115,#87116,#87117,#87118,#87119,#87120,#87121,#87122,#87123,#87124,#87125,
#87126,#87127,#87128,#87129,#87130,#87131,#87132,#87133,#87134,#87135,#87136,
#87137,#87138,#87139,#87140,#87141,#87142,#87143,#87144,#87145,#87146,#87147,
#87148,#87149,#87150,#87151,#87152,#87153,#87154,#87155,#87156,#87157,#87158,
#87159,#87160,#87161,#87162,#87163,#87164,#87165,#87166,#87167,#87168,#87169,
#87170,#87171,#87172,#87173,#87174,#87175,#87176,#87177,#87178,#87179,#87180,
#87181,#87182,#87183,#87184,#87185,#87186,#87187,#87188,#87189,#87190,#87191,
#87192,#87193,#87194,#87195,#87196,#87197,#87198,#87199,#87200,#87201,#87202,
#87203,#87204,#87205,#87206,#87207,#87208,#87209,#87210,#87211,#87212,#87213,
#87214,#87215,#87216,#87217,#87218)),.UNSPECIFIED.,.F.,.F.,.F.,(4,4),(4,
1,1,1,1,1,1,1,1,1,1,1,1,1,1,1,1,1,1,1,1,1,1,1,1,1,1,1,1,1,1,1,1,1,1,1,1,
1,1,1,1,1,1,1,1,1,1,1,1,1,1,1,1,1,1,1,1,1,1,1,1,1,1,1,1,1,1,1,1,1,1,1,1,
1,1,1,1,1,1,1,1,1,1,1,1,1,1,1,1,1,1,1,1,1,1,1,1,1,1,1,1,1,1,1,1,1,1,1,1,
1,1,1,1,1,1,1,1,1,1,1,1,1,1,1,1,1,1,1,4),(0.,0.0642013499338879),(11.8589888623077,
12.8564939485313,13.8539990347549,14.8515041209785,15.8490092072021,16.8465142934257,
17.8440193796493,18.8415244658729,19.8390295520965,20.8365346383201,21.8340397245437,
22.8315448107673,23.8290498969909,24.8265549832145,25.8240600694381,26.8215651556617,
27.8190702418853,28.8165753281089,29.8140804143324,30.811585500556,31.8090905867796,
32.8065956730032,33.8041007592268,34.8016058454504,35.799110931674,36.7966160178976,
37.7941211041212,38.7916261903448,39.7891312765684,40.786636362792,41.7841414490156,
42.7816465352392,43.7791516214628,44.7766567076864,45.77416179391,46.7716668801336,
47.7691719663572,48.7666770525807,49.7641821388043,50.7616872250279,51.7591923112515,
52.7566973974751,53.7542024836987,54.7517075699223,55.7492126561459,56.7467177423695,
57.7442228285931,58.7417279148167,59.7392330010403,60.7367380872639,61.7342431734875,
62.7317482597111,63.7292533459347,64.7267584321583,65.7242635183819,66.7217686046055,
67.7192736908291,68.7167787770527,69.7142838632763,70.7117889494998,71.7092940357234,
72.706799121947,73.7043042081706,74.7018092943942,75.6993143806178,76.6968194668414,
77.694324553065,78.6918296392886,79.6893347255122,80.6868398117358,81.6843448979594,
82.681849984183,83.6793550704066,84.6768601566302,85.6743652428538,86.6718703290774,
87.669375415301,88.6668805015246,89.6643855877482,90.6618906739717,91.6593957601953,
92.6569008464189,93.6544059326425,94.6519110188661,95.6494161050897,96.6469211913133,
97.6444262775369,98.6419313637605,99.6394364499841,100.636941536208,101.634446622431,
102.631951708655,103.629456794878,104.626961881102,105.624466967326,106.621972053549,
107.619477139773,108.616982225996,109.61448731222,110.611992398444,111.609497484667,
112.607002570891,113.604507657114,114.602012743338,115.599517829562,116.597022915785,
117.594528002009,118.592033088232,119.589538174456,120.58704326068,121.584548346903,
122.582053433127,123.57955851935,124.577063605574,125.574568691798,126.572073778021,
127.569578864245,128.567083950468,129.564589036692,130.562094122916,131.559599209139,
132.557104295363,133.554609381586,134.55211446781,135.549619554034,136.547124640257,
137.544629726481,138.542134812704,139.539639898928),.UNSPECIFIED.);
#369=B_SPLINE_SURFACE_WITH_KNOTS('',3,3,((#87338,#87339,#87340,#87341,#87342,
#87343,#87344,#87345,#87346,#87347,#87348,#87349,#87350,#87351,#87352,#87353,
#87354,#87355,#87356,#87357,#87358,#87359,#87360,#87361,#87362,#87363,#87364,
#87365,#87366,#87367,#87368,#87369,#87370,#87371,#87372,#87373,#87374,#87375,
#87376,#87377,#87378,#87379,#87380,#87381,#87382,#87383,#87384,#87385,#87386,
#87387,#87388,#87389,#87390,#87391,#87392,#87393,#87394,#87395,#87396,#87397,
#87398,#87399,#87400,#87401,#87402,#87403,#87404,#87405,#87406,#87407,#87408,
#87409,#87410,#87411,#87412,#87413,#87414,#87415,#87416,#87417,#87418,#87419,
#87420,#87421,#87422,#87423,#87424,#87425,#87426,#87427,#87428,#87429,#87430,
#87431,#87432,#87433,#87434,#87435,#87436,#87437,#87438,#87439,#87440,#87441,
#87442,#87443,#87444,#87445,#87446,#87447,#87448,#87449,#87450,#87451,#87452,
#87453,#87454,#87455,#87456,#87457,#87458,#87459,#87460,#87461,#87462,#87463,
#87464,#87465,#87466,#87467,#87468),(#87469,#87470,#87471,#87472,#87473,
#87474,#87475,#87476,#87477,#87478,#87479,#87480,#87481,#87482,#87483,#87484,
#87485,#87486,#87487,#87488,#87489,#87490,#87491,#87492,#87493,#87494,#87495,
#87496,#87497,#87498,#87499,#87500,#87501,#87502,#87503,#87504,#87505,#87506,
#87507,#87508,#87509,#87510,#87511,#87512,#87513,#87514,#87515,#87516,#87517,
#87518,#87519,#87520,#87521,#87522,#87523,#87524,#87525,#87526,#87527,#87528,
#87529,#87530,#87531,#87532,#87533,#87534,#87535,#87536,#87537,#87538,#87539,
#87540,#87541,#87542,#87543,#87544,#87545,#87546,#87547,#87548,#87549,#87550,
#87551,#87552,#87553,#87554,#87555,#87556,#87557,#87558,#87559,#87560,#87561,
#87562,#87563,#87564,#87565,#87566,#87567,#87568,#87569,#87570,#87571,#87572,
#87573,#87574,#87575,#87576,#87577,#87578,#87579,#87580,#87581,#87582,#87583,
#87584,#87585,#87586,#87587,#87588,#87589,#87590,#87591,#87592,#87593,#87594,
#87595,#87596,#87597,#87598,#87599),(#87600,#87601,#87602,#87603,#87604,
#87605,#87606,#87607,#87608,#87609,#87610,#87611,#87612,#87613,#87614,#87615,
#87616,#87617,#87618,#87619,#87620,#87621,#87622,#87623,#87624,#87625,#87626,
#87627,#87628,#87629,#87630,#87631,#87632,#87633,#87634,#87635,#87636,#87637,
#87638,#87639,#87640,#87641,#87642,#87643,#87644,#87645,#87646,#87647,#87648,
#87649,#87650,#87651,#87652,#87653,#87654,#87655,#87656,#87657,#87658,#87659,
#87660,#87661,#87662,#87663,#87664,#87665,#87666,#87667,#87668,#87669,#87670,
#87671,#87672,#87673,#87674,#87675,#87676,#87677,#87678,#87679,#87680,#87681,
#87682,#87683,#87684,#87685,#87686,#87687,#87688,#87689,#87690,#87691,#87692,
#87693,#87694,#87695,#87696,#87697,#87698,#87699,#87700,#87701,#87702,#87703,
#87704,#87705,#87706,#87707,#87708,#87709,#87710,#87711,#87712,#87713,#87714,
#87715,#87716,#87717,#87718,#87719,#87720,#87721,#87722,#87723,#87724,#87725,
#87726,#87727,#87728,#87729,#87730),(#87731,#87732,#87733,#87734,#87735,
#87736,#87737,#87738,#87739,#87740,#87741,#87742,#87743,#87744,#87745,#87746,
#87747,#87748,#87749,#87750,#87751,#87752,#87753,#87754,#87755,#87756,#87757,
#87758,#87759,#87760,#87761,#87762,#87763,#87764,#87765,#87766,#87767,#87768,
#87769,#87770,#87771,#87772,#87773,#87774,#87775,#87776,#87777,#87778,#87779,
#87780,#87781,#87782,#87783,#87784,#87785,#87786,#87787,#87788,#87789,#87790,
#87791,#87792,#87793,#87794,#87795,#87796,#87797,#87798,#87799,#87800,#87801,
#87802,#87803,#87804,#87805,#87806,#87807,#87808,#87809,#87810,#87811,#87812,
#87813,#87814,#87815,#87816,#87817,#87818,#87819,#87820,#87821,#87822,#87823,
#87824,#87825,#87826,#87827,#87828,#87829,#87830,#87831,#87832,#87833,#87834,
#87835,#87836,#87837,#87838,#87839,#87840,#87841,#87842,#87843,#87844,#87845,
#87846,#87847,#87848,#87849,#87850,#87851,#87852,#87853,#87854,#87855,#87856,
#87857,#87858,#87859,#87860,#87861)),.UNSPECIFIED.,.F.,.F.,.F.,(4,4),(4,
1,1,1,1,1,1,1,1,1,1,1,1,1,1,1,1,1,1,1,1,1,1,1,1,1,1,1,1,1,1,1,1,1,1,1,1,
1,1,1,1,1,1,1,1,1,1,1,1,1,1,1,1,1,1,1,1,1,1,1,1,1,1,1,1,1,1,1,1,1,1,1,1,
1,1,1,1,1,1,1,1,1,1,1,1,1,1,1,1,1,1,1,1,1,1,1,1,1,1,1,1,1,1,1,1,1,1,1,1,
1,1,1,1,1,1,1,1,1,1,1,1,1,1,1,1,1,1,1,4),(0.,0.0642013499338879),(14.3984001269718,
15.3959052131954,16.393410299419,17.3909153856426,18.3884204718662,19.3859255580897,
20.3834306443133,21.3809357305369,22.3784408167605,23.3759459029841,24.3734509892077,
25.3709560754313,26.3684611616549,27.3659662478785,28.3634713341021,29.3609764203257,
30.3584815065493,31.3559865927729,32.3534916789965,33.3509967652201,34.3485018514437,
35.3460069376673,36.3435120238909,37.3410171101145,38.3385221963381,39.3360272825616,
40.3335323687852,41.3310374550088,42.3285425412324,43.326047627456,44.3235527136796,
45.3210577999032,46.3185628861268,47.3160679723504,48.313573058574,49.3110781447976,
50.3085832310212,51.3060883172448,52.3035934034684,53.301098489692,54.2986035759156,
55.2961086621392,56.2936137483628,57.2911188345864,58.28862392081,59.2861290070336,
60.2836340932571,61.2811391794807,62.2786442657043,63.2761493519279,64.2736544381515,
65.2711595243751,66.2686646105987,67.2661696968223,68.2636747830459,69.2611798692695,
70.2586849554931,71.2561900417167,72.2536951279403,73.2512002141639,74.2487053003875,
75.2462103866111,76.2437154728347,77.2412205590583,78.2387256452818,79.2362307315055,
80.233735817729,81.2312409039526,82.2287459901762,83.2262510763998,84.2237561626234,
85.221261248847,86.2187663350706,87.2162714212942,88.2137765075178,89.2112815937414,
90.208786679965,91.2062917661886,92.2037968524122,93.2013019386358,94.1988070248594,
95.196312111083,96.1938171973066,97.1913222835302,98.1888273697538,99.1863324559774,
100.183837542201,101.181342628425,102.178847714648,103.176352800872,104.173857887095,
105.171362973319,106.168868059543,107.166373145766,108.16387823199,109.161383318213,
110.158888404437,111.15639349066,112.153898576884,113.151403663108,114.148908749331,
115.146413835555,116.143918921778,117.141424008002,118.138929094226,119.136434180449,
120.133939266673,121.131444352896,122.12894943912,123.126454525344,124.123959611567,
125.121464697791,126.118969784014,127.116474870238,128.113979956462,129.111485042685,
130.108990128909,131.106495215132,132.104000301356,133.10150538758,134.099010473803,
135.096515560027,136.09402064625,137.091525732474,138.089030818698,139.086535904921,
140.084040991145,141.081546077368,142.079051163592),.UNSPECIFIED.);
#370=B_SPLINE_SURFACE_WITH_KNOTS('',3,3,((#88000,#88001,#88002,#88003,#88004,
#88005,#88006,#88007,#88008,#88009,#88010,#88011,#88012,#88013,#88014,#88015,
#88016,#88017,#88018,#88019,#88020,#88021,#88022,#88023,#88024,#88025,#88026,
#88027,#88028,#88029,#88030,#88031,#88032,#88033,#88034,#88035,#88036,#88037,
#88038,#88039,#88040,#88041,#88042,#88043,#88044,#88045,#88046,#88047,#88048,
#88049,#88050,#88051,#88052,#88053,#88054,#88055,#88056,#88057,#88058,#88059,
#88060,#88061,#88062,#88063,#88064,#88065,#88066,#88067,#88068,#88069,#88070,
#88071,#88072,#88073,#88074,#88075,#88076,#88077,#88078,#88079,#88080,#88081,
#88082,#88083,#88084,#88085,#88086,#88087,#88088,#88089,#88090,#88091,#88092,
#88093,#88094,#88095,#88096,#88097,#88098,#88099,#88100,#88101,#88102,#88103,
#88104,#88105,#88106,#88107,#88108,#88109,#88110,#88111,#88112,#88113,#88114,
#88115,#88116,#88117,#88118,#88119,#88120,#88121,#88122,#88123,#88124,#88125,
#88126,#88127,#88128,#88129,#88130),(#88131,#88132,#88133,#88134,#88135,
#88136,#88137,#88138,#88139,#88140,#88141,#88142,#88143,#88144,#88145,#88146,
#88147,#88148,#88149,#88150,#88151,#88152,#88153,#88154,#88155,#88156,#88157,
#88158,#88159,#88160,#88161,#88162,#88163,#88164,#88165,#88166,#88167,#88168,
#88169,#88170,#88171,#88172,#88173,#88174,#88175,#88176,#88177,#88178,#88179,
#88180,#88181,#88182,#88183,#88184,#88185,#88186,#88187,#88188,#88189,#88190,
#88191,#88192,#88193,#88194,#88195,#88196,#88197,#88198,#88199,#88200,#88201,
#88202,#88203,#88204,#88205,#88206,#88207,#88208,#88209,#88210,#88211,#88212,
#88213,#88214,#88215,#88216,#88217,#88218,#88219,#88220,#88221,#88222,#88223,
#88224,#88225,#88226,#88227,#88228,#88229,#88230,#88231,#88232,#88233,#88234,
#88235,#88236,#88237,#88238,#88239,#88240,#88241,#88242,#88243,#88244,#88245,
#88246,#88247,#88248,#88249,#88250,#88251,#88252,#88253,#88254,#88255,#88256,
#88257,#88258,#88259,#88260,#88261),(#88262,#88263,#88264,#88265,#88266,
#88267,#88268,#88269,#88270,#88271,#88272,#88273,#88274,#88275,#88276,#88277,
#88278,#88279,#88280,#88281,#88282,#88283,#88284,#88285,#88286,#88287,#88288,
#88289,#88290,#88291,#88292,#88293,#88294,#88295,#88296,#88297,#88298,#88299,
#88300,#88301,#88302,#88303,#88304,#88305,#88306,#88307,#88308,#88309,#88310,
#88311,#88312,#88313,#88314,#88315,#88316,#88317,#88318,#88319,#88320,#88321,
#88322,#88323,#88324,#88325,#88326,#88327,#88328,#88329,#88330,#88331,#88332,
#88333,#88334,#88335,#88336,#88337,#88338,#88339,#88340,#88341,#88342,#88343,
#88344,#88345,#88346,#88347,#88348,#88349,#88350,#88351,#88352,#88353,#88354,
#88355,#88356,#88357,#88358,#88359,#88360,#88361,#88362,#88363,#88364,#88365,
#88366,#88367,#88368,#88369,#88370,#88371,#88372,#88373,#88374,#88375,#88376,
#88377,#88378,#88379,#88380,#88381,#88382,#88383,#88384,#88385,#88386,#88387,
#88388,#88389,#88390,#88391,#88392),(#88393,#88394,#88395,#88396,#88397,
#88398,#88399,#88400,#88401,#88402,#88403,#88404,#88405,#88406,#88407,#88408,
#88409,#88410,#88411,#88412,#88413,#88414,#88415,#88416,#88417,#88418,#88419,
#88420,#88421,#88422,#88423,#88424,#88425,#88426,#88427,#88428,#88429,#88430,
#88431,#88432,#88433,#88434,#88435,#88436,#88437,#88438,#88439,#88440,#88441,
#88442,#88443,#88444,#88445,#88446,#88447,#88448,#88449,#88450,#88451,#88452,
#88453,#88454,#88455,#88456,#88457,#88458,#88459,#88460,#88461,#88462,#88463,
#88464,#88465,#88466,#88467,#88468,#88469,#88470,#88471,#88472,#88473,#88474,
#88475,#88476,#88477,#88478,#88479,#88480,#88481,#88482,#88483,#88484,#88485,
#88486,#88487,#88488,#88489,#88490,#88491,#88492,#88493,#88494,#88495,#88496,
#88497,#88498,#88499,#88500,#88501,#88502,#88503,#88504,#88505,#88506,#88507,
#88508,#88509,#88510,#88511,#88512,#88513,#88514,#88515,#88516,#88517,#88518,
#88519,#88520,#88521,#88522,#88523)),.UNSPECIFIED.,.F.,.F.,.F.,(4,4),(4,
1,1,1,1,1,1,1,1,1,1,1,1,1,1,1,1,1,1,1,1,1,1,1,1,1,1,1,1,1,1,1,1,1,1,1,1,
1,1,1,1,1,1,1,1,1,1,1,1,1,1,1,1,1,1,1,1,1,1,1,1,1,1,1,1,1,1,1,1,1,1,1,1,
1,1,1,1,1,1,1,1,1,1,1,1,1,1,1,1,1,1,1,1,1,1,1,1,1,1,1,1,1,1,1,1,1,1,1,1,
1,1,1,1,1,1,1,1,1,1,1,1,1,1,1,1,1,1,1,4),(0.,0.0642013499338864),(11.8589888623077,
12.8564939485313,13.8539990347549,14.8515041209785,15.8490092072021,16.8465142934256,
17.8440193796492,18.8415244658728,19.8390295520964,20.83653463832,21.8340397245436,
22.8315448107672,23.8290498969908,24.8265549832144,25.824060069438,26.8215651556616,
27.8190702418852,28.8165753281088,29.8140804143324,30.811585500556,31.8090905867796,
32.8065956730032,33.8041007592268,34.8016058454504,35.799110931674,36.7966160178976,
37.7941211041212,38.7916261903448,39.7891312765683,40.7866363627919,41.7841414490155,
42.7816465352391,43.7791516214627,44.7766567076863,45.7741617939099,46.7716668801335,
47.7691719663571,48.7666770525807,49.7641821388043,50.7616872250279,51.7591923112515,
52.7566973974751,53.7542024836987,54.7517075699223,55.7492126561459,56.7467177423695,
57.7442228285931,58.7417279148167,59.7392330010403,60.7367380872638,61.7342431734874,
62.731748259711,63.7292533459346,64.7267584321582,65.7242635183818,66.7217686046054,
67.719273690829,68.7167787770526,69.7142838632762,70.7117889494998,71.7092940357234,
72.706799121947,73.7043042081706,74.7018092943942,75.6993143806178,76.6968194668414,
77.694324553065,78.6918296392886,79.6893347255122,80.6868398117358,81.6843448979593,
82.6818499841829,83.6793550704065,84.6768601566301,85.6743652428537,86.6718703290773,
87.6693754153009,88.6668805015245,89.6643855877481,90.6618906739717,91.6593957601953,
92.6569008464189,93.6544059326425,94.6519110188661,95.6494161050897,96.6469211913133,
97.6444262775369,98.6419313637605,99.6394364499841,100.636941536208,101.634446622431,
102.631951708655,103.629456794878,104.626961881102,105.624466967326,106.621972053549,
107.619477139773,108.616982225996,109.61448731222,110.611992398444,111.609497484667,
112.607002570891,113.604507657114,114.602012743338,115.599517829562,116.597022915785,
117.594528002009,118.592033088232,119.589538174456,120.58704326068,121.584548346903,
122.582053433127,123.57955851935,124.577063605574,125.574568691798,126.572073778021,
127.569578864245,128.567083950468,129.564589036692,130.562094122916,131.559599209139,
132.557104295363,133.554609381586,134.55211446781,135.549619554034,136.547124640257,
137.544629726481,138.542134812704,139.539639898928),.UNSPECIFIED.);
#371=B_SPLINE_SURFACE_WITH_KNOTS('',3,3,((#88643,#88644,#88645,#88646,#88647,
#88648,#88649,#88650,#88651,#88652,#88653,#88654,#88655,#88656,#88657,#88658,
#88659,#88660,#88661,#88662,#88663,#88664,#88665,#88666,#88667,#88668,#88669,
#88670,#88671,#88672,#88673,#88674,#88675,#88676,#88677,#88678,#88679,#88680,
#88681,#88682,#88683,#88684,#88685,#88686,#88687,#88688,#88689,#88690,#88691,
#88692,#88693,#88694,#88695,#88696,#88697,#88698,#88699,#88700,#88701,#88702,
#88703,#88704,#88705,#88706,#88707,#88708,#88709,#88710,#88711,#88712,#88713,
#88714,#88715,#88716,#88717,#88718,#88719,#88720,#88721,#88722,#88723,#88724,
#88725,#88726,#88727,#88728,#88729,#88730,#88731,#88732,#88733,#88734,#88735,
#88736,#88737,#88738,#88739,#88740,#88741,#88742,#88743,#88744,#88745,#88746,
#88747,#88748,#88749,#88750,#88751,#88752,#88753,#88754,#88755,#88756,#88757,
#88758,#88759,#88760,#88761,#88762,#88763,#88764,#88765,#88766,#88767,#88768,
#88769,#88770,#88771,#88772,#88773),(#88774,#88775,#88776,#88777,#88778,
#88779,#88780,#88781,#88782,#88783,#88784,#88785,#88786,#88787,#88788,#88789,
#88790,#88791,#88792,#88793,#88794,#88795,#88796,#88797,#88798,#88799,#88800,
#88801,#88802,#88803,#88804,#88805,#88806,#88807,#88808,#88809,#88810,#88811,
#88812,#88813,#88814,#88815,#88816,#88817,#88818,#88819,#88820,#88821,#88822,
#88823,#88824,#88825,#88826,#88827,#88828,#88829,#88830,#88831,#88832,#88833,
#88834,#88835,#88836,#88837,#88838,#88839,#88840,#88841,#88842,#88843,#88844,
#88845,#88846,#88847,#88848,#88849,#88850,#88851,#88852,#88853,#88854,#88855,
#88856,#88857,#88858,#88859,#88860,#88861,#88862,#88863,#88864,#88865,#88866,
#88867,#88868,#88869,#88870,#88871,#88872,#88873,#88874,#88875,#88876,#88877,
#88878,#88879,#88880,#88881,#88882,#88883,#88884,#88885,#88886,#88887,#88888,
#88889,#88890,#88891,#88892,#88893,#88894,#88895,#88896,#88897,#88898,#88899,
#88900,#88901,#88902,#88903,#88904),(#88905,#88906,#88907,#88908,#88909,
#88910,#88911,#88912,#88913,#88914,#88915,#88916,#88917,#88918,#88919,#88920,
#88921,#88922,#88923,#88924,#88925,#88926,#88927,#88928,#88929,#88930,#88931,
#88932,#88933,#88934,#88935,#88936,#88937,#88938,#88939,#88940,#88941,#88942,
#88943,#88944,#88945,#88946,#88947,#88948,#88949,#88950,#88951,#88952,#88953,
#88954,#88955,#88956,#88957,#88958,#88959,#88960,#88961,#88962,#88963,#88964,
#88965,#88966,#88967,#88968,#88969,#88970,#88971,#88972,#88973,#88974,#88975,
#88976,#88977,#88978,#88979,#88980,#88981,#88982,#88983,#88984,#88985,#88986,
#88987,#88988,#88989,#88990,#88991,#88992,#88993,#88994,#88995,#88996,#88997,
#88998,#88999,#89000,#89001,#89002,#89003,#89004,#89005,#89006,#89007,#89008,
#89009,#89010,#89011,#89012,#89013,#89014,#89015,#89016,#89017,#89018,#89019,
#89020,#89021,#89022,#89023,#89024,#89025,#89026,#89027,#89028,#89029,#89030,
#89031,#89032,#89033,#89034,#89035),(#89036,#89037,#89038,#89039,#89040,
#89041,#89042,#89043,#89044,#89045,#89046,#89047,#89048,#89049,#89050,#89051,
#89052,#89053,#89054,#89055,#89056,#89057,#89058,#89059,#89060,#89061,#89062,
#89063,#89064,#89065,#89066,#89067,#89068,#89069,#89070,#89071,#89072,#89073,
#89074,#89075,#89076,#89077,#89078,#89079,#89080,#89081,#89082,#89083,#89084,
#89085,#89086,#89087,#89088,#89089,#89090,#89091,#89092,#89093,#89094,#89095,
#89096,#89097,#89098,#89099,#89100,#89101,#89102,#89103,#89104,#89105,#89106,
#89107,#89108,#89109,#89110,#89111,#89112,#89113,#89114,#89115,#89116,#89117,
#89118,#89119,#89120,#89121,#89122,#89123,#89124,#89125,#89126,#89127,#89128,
#89129,#89130,#89131,#89132,#89133,#89134,#89135,#89136,#89137,#89138,#89139,
#89140,#89141,#89142,#89143,#89144,#89145,#89146,#89147,#89148,#89149,#89150,
#89151,#89152,#89153,#89154,#89155,#89156,#89157,#89158,#89159,#89160,#89161,
#89162,#89163,#89164,#89165,#89166)),.UNSPECIFIED.,.F.,.F.,.F.,(4,4),(4,
1,1,1,1,1,1,1,1,1,1,1,1,1,1,1,1,1,1,1,1,1,1,1,1,1,1,1,1,1,1,1,1,1,1,1,1,
1,1,1,1,1,1,1,1,1,1,1,1,1,1,1,1,1,1,1,1,1,1,1,1,1,1,1,1,1,1,1,1,1,1,1,1,
1,1,1,1,1,1,1,1,1,1,1,1,1,1,1,1,1,1,1,1,1,1,1,1,1,1,1,1,1,1,1,1,1,1,1,1,
1,1,1,1,1,1,1,1,1,1,1,1,1,1,1,1,1,1,1,4),(0.,0.0642013499338864),(14.3984001269717,
15.3959052131953,16.3934102994189,17.3909153856425,18.3884204718661,19.3859255580897,
20.3834306443133,21.3809357305369,22.3784408167605,23.3759459029841,24.3734509892077,
25.3709560754313,26.3684611616549,27.3659662478785,28.363471334102,29.3609764203256,
30.3584815065492,31.3559865927728,32.3534916789964,33.35099676522,34.3485018514436,
35.3460069376672,36.3435120238908,37.3410171101144,38.338522196338,39.3360272825616,
40.3335323687852,41.3310374550088,42.3285425412324,43.326047627456,44.3235527136796,
45.3210577999032,46.3185628861268,47.3160679723504,48.3135730585739,49.3110781447975,
50.3085832310211,51.3060883172447,52.3035934034683,53.3010984896919,54.2986035759155,
55.2961086621391,56.2936137483627,57.2911188345863,58.2886239208099,59.2861290070335,
60.2836340932571,61.2811391794807,62.2786442657043,63.2761493519279,64.2736544381515,
65.2711595243751,66.2686646105986,67.2661696968223,68.2636747830458,69.2611798692694,
70.258684955493,71.2561900417166,72.2536951279402,73.2512002141638,74.2487053003874,
75.246210386611,76.2437154728346,77.2412205590582,78.2387256452818,79.2362307315054,
80.233735817729,81.2312409039526,82.2287459901762,83.2262510763998,84.2237561626234,
85.221261248847,86.2187663350706,87.2162714212942,88.2137765075177,89.2112815937413,
90.2087866799649,91.2062917661885,92.2037968524121,93.2013019386357,94.1988070248593,
95.1963121110829,96.1938171973065,97.1913222835301,98.1888273697537,99.1863324559773,
100.183837542201,101.181342628424,102.178847714648,103.176352800872,104.173857887095,
105.171362973319,106.168868059542,107.166373145766,108.16387823199,109.161383318213,
110.158888404437,111.15639349066,112.153898576884,113.151403663108,114.148908749331,
115.146413835555,116.143918921778,117.141424008002,118.138929094226,119.136434180449,
120.133939266673,121.131444352896,122.12894943912,123.126454525344,124.123959611567,
125.121464697791,126.118969784014,127.116474870238,128.113979956462,129.111485042685,
130.108990128909,131.106495215132,132.104000301356,133.10150538758,134.099010473803,
135.096515560027,136.09402064625,137.091525732474,138.089030818697,139.086535904921,
140.084040991145,141.081546077368,142.079051163592),.UNSPECIFIED.);
#372=B_SPLINE_SURFACE_WITH_KNOTS('',3,3,((#89305,#89306,#89307,#89308,#89309,
#89310,#89311,#89312,#89313,#89314,#89315,#89316,#89317,#89318,#89319,#89320,
#89321,#89322,#89323,#89324,#89325,#89326,#89327,#89328,#89329,#89330,#89331,
#89332,#89333,#89334,#89335,#89336,#89337,#89338,#89339,#89340,#89341,#89342,
#89343,#89344,#89345,#89346,#89347,#89348,#89349,#89350,#89351,#89352,#89353,
#89354,#89355,#89356,#89357,#89358,#89359,#89360,#89361,#89362,#89363,#89364,
#89365,#89366,#89367,#89368,#89369,#89370,#89371,#89372,#89373,#89374,#89375,
#89376,#89377,#89378,#89379,#89380,#89381,#89382,#89383,#89384,#89385,#89386,
#89387,#89388,#89389,#89390,#89391,#89392,#89393,#89394,#89395,#89396,#89397,
#89398,#89399,#89400,#89401,#89402,#89403,#89404,#89405,#89406,#89407,#89408,
#89409,#89410,#89411,#89412,#89413,#89414,#89415,#89416,#89417,#89418,#89419,
#89420,#89421,#89422,#89423,#89424,#89425,#89426,#89427,#89428,#89429,#89430,
#89431,#89432,#89433,#89434,#89435),(#89436,#89437,#89438,#89439,#89440,
#89441,#89442,#89443,#89444,#89445,#89446,#89447,#89448,#89449,#89450,#89451,
#89452,#89453,#89454,#89455,#89456,#89457,#89458,#89459,#89460,#89461,#89462,
#89463,#89464,#89465,#89466,#89467,#89468,#89469,#89470,#89471,#89472,#89473,
#89474,#89475,#89476,#89477,#89478,#89479,#89480,#89481,#89482,#89483,#89484,
#89485,#89486,#89487,#89488,#89489,#89490,#89491,#89492,#89493,#89494,#89495,
#89496,#89497,#89498,#89499,#89500,#89501,#89502,#89503,#89504,#89505,#89506,
#89507,#89508,#89509,#89510,#89511,#89512,#89513,#89514,#89515,#89516,#89517,
#89518,#89519,#89520,#89521,#89522,#89523,#89524,#89525,#89526,#89527,#89528,
#89529,#89530,#89531,#89532,#89533,#89534,#89535,#89536,#89537,#89538,#89539,
#89540,#89541,#89542,#89543,#89544,#89545,#89546,#89547,#89548,#89549,#89550,
#89551,#89552,#89553,#89554,#89555,#89556,#89557,#89558,#89559,#89560,#89561,
#89562,#89563,#89564,#89565,#89566),(#89567,#89568,#89569,#89570,#89571,
#89572,#89573,#89574,#89575,#89576,#89577,#89578,#89579,#89580,#89581,#89582,
#89583,#89584,#89585,#89586,#89587,#89588,#89589,#89590,#89591,#89592,#89593,
#89594,#89595,#89596,#89597,#89598,#89599,#89600,#89601,#89602,#89603,#89604,
#89605,#89606,#89607,#89608,#89609,#89610,#89611,#89612,#89613,#89614,#89615,
#89616,#89617,#89618,#89619,#89620,#89621,#89622,#89623,#89624,#89625,#89626,
#89627,#89628,#89629,#89630,#89631,#89632,#89633,#89634,#89635,#89636,#89637,
#89638,#89639,#89640,#89641,#89642,#89643,#89644,#89645,#89646,#89647,#89648,
#89649,#89650,#89651,#89652,#89653,#89654,#89655,#89656,#89657,#89658,#89659,
#89660,#89661,#89662,#89663,#89664,#89665,#89666,#89667,#89668,#89669,#89670,
#89671,#89672,#89673,#89674,#89675,#89676,#89677,#89678,#89679,#89680,#89681,
#89682,#89683,#89684,#89685,#89686,#89687,#89688,#89689,#89690,#89691,#89692,
#89693,#89694,#89695,#89696,#89697),(#89698,#89699,#89700,#89701,#89702,
#89703,#89704,#89705,#89706,#89707,#89708,#89709,#89710,#89711,#89712,#89713,
#89714,#89715,#89716,#89717,#89718,#89719,#89720,#89721,#89722,#89723,#89724,
#89725,#89726,#89727,#89728,#89729,#89730,#89731,#89732,#89733,#89734,#89735,
#89736,#89737,#89738,#89739,#89740,#89741,#89742,#89743,#89744,#89745,#89746,
#89747,#89748,#89749,#89750,#89751,#89752,#89753,#89754,#89755,#89756,#89757,
#89758,#89759,#89760,#89761,#89762,#89763,#89764,#89765,#89766,#89767,#89768,
#89769,#89770,#89771,#89772,#89773,#89774,#89775,#89776,#89777,#89778,#89779,
#89780,#89781,#89782,#89783,#89784,#89785,#89786,#89787,#89788,#89789,#89790,
#89791,#89792,#89793,#89794,#89795,#89796,#89797,#89798,#89799,#89800,#89801,
#89802,#89803,#89804,#89805,#89806,#89807,#89808,#89809,#89810,#89811,#89812,
#89813,#89814,#89815,#89816,#89817,#89818,#89819,#89820,#89821,#89822,#89823,
#89824,#89825,#89826,#89827,#89828)),.UNSPECIFIED.,.F.,.F.,.F.,(4,4),(4,
1,1,1,1,1,1,1,1,1,1,1,1,1,1,1,1,1,1,1,1,1,1,1,1,1,1,1,1,1,1,1,1,1,1,1,1,
1,1,1,1,1,1,1,1,1,1,1,1,1,1,1,1,1,1,1,1,1,1,1,1,1,1,1,1,1,1,1,1,1,1,1,1,
1,1,1,1,1,1,1,1,1,1,1,1,1,1,1,1,1,1,1,1,1,1,1,1,1,1,1,1,1,1,1,1,1,1,1,1,
1,1,1,1,1,1,1,1,1,1,1,1,1,1,1,1,1,1,1,4),(0.,0.0642013499338863),(11.8589888623077,
12.8564939485313,13.8539990347549,14.8515041209785,15.8490092072021,16.8465142934257,
17.8440193796493,18.8415244658729,19.8390295520965,20.8365346383201,21.8340397245437,
22.8315448107673,23.8290498969909,24.8265549832145,25.8240600694381,26.8215651556617,
27.8190702418853,28.8165753281089,29.8140804143324,30.811585500556,31.8090905867796,
32.8065956730032,33.8041007592268,34.8016058454504,35.799110931674,36.7966160178976,
37.7941211041212,38.7916261903448,39.7891312765684,40.786636362792,41.7841414490156,
42.7816465352392,43.7791516214628,44.7766567076864,45.77416179391,46.7716668801336,
47.7691719663572,48.7666770525807,49.7641821388043,50.7616872250279,51.7591923112515,
52.7566973974751,53.7542024836987,54.7517075699223,55.7492126561459,56.7467177423695,
57.7442228285931,58.7417279148167,59.7392330010403,60.7367380872639,61.7342431734875,
62.7317482597111,63.7292533459347,64.7267584321583,65.7242635183819,66.7217686046055,
67.7192736908291,68.7167787770527,69.7142838632763,70.7117889494998,71.7092940357234,
72.706799121947,73.7043042081706,74.7018092943942,75.6993143806178,76.6968194668414,
77.694324553065,78.6918296392886,79.6893347255122,80.6868398117358,81.6843448979594,
82.681849984183,83.6793550704066,84.6768601566302,85.6743652428538,86.6718703290774,
87.669375415301,88.6668805015246,89.6643855877482,90.6618906739717,91.6593957601953,
92.6569008464189,93.6544059326425,94.6519110188661,95.6494161050897,96.6469211913133,
97.6444262775369,98.6419313637605,99.6394364499841,100.636941536208,101.634446622431,
102.631951708655,103.629456794878,104.626961881102,105.624466967326,106.621972053549,
107.619477139773,108.616982225996,109.61448731222,110.611992398444,111.609497484667,
112.607002570891,113.604507657114,114.602012743338,115.599517829562,116.597022915785,
117.594528002009,118.592033088232,119.589538174456,120.58704326068,121.584548346903,
122.582053433127,123.57955851935,124.577063605574,125.574568691798,126.572073778021,
127.569578864245,128.567083950468,129.564589036692,130.562094122916,131.559599209139,
132.557104295363,133.554609381586,134.55211446781,135.549619554034,136.547124640257,
137.544629726481,138.542134812704,139.539639898928),.UNSPECIFIED.);
#373=B_SPLINE_SURFACE_WITH_KNOTS('',3,3,((#89948,#89949,#89950,#89951,#89952,
#89953,#89954,#89955,#89956,#89957,#89958,#89959,#89960,#89961,#89962,#89963,
#89964,#89965,#89966,#89967,#89968,#89969,#89970,#89971,#89972,#89973,#89974,
#89975,#89976,#89977,#89978,#89979,#89980,#89981,#89982,#89983,#89984,#89985,
#89986,#89987,#89988,#89989,#89990,#89991,#89992,#89993,#89994,#89995,#89996,
#89997,#89998,#89999,#90000,#90001,#90002,#90003,#90004,#90005,#90006,#90007,
#90008,#90009,#90010,#90011,#90012,#90013,#90014,#90015,#90016,#90017,#90018,
#90019,#90020,#90021,#90022,#90023,#90024,#90025,#90026,#90027,#90028,#90029,
#90030,#90031,#90032,#90033,#90034,#90035,#90036,#90037,#90038,#90039,#90040,
#90041,#90042,#90043,#90044,#90045,#90046,#90047,#90048,#90049,#90050,#90051,
#90052,#90053,#90054,#90055,#90056,#90057,#90058,#90059,#90060,#90061,#90062,
#90063,#90064,#90065,#90066,#90067,#90068,#90069,#90070,#90071,#90072,#90073,
#90074,#90075,#90076,#90077,#90078),(#90079,#90080,#90081,#90082,#90083,
#90084,#90085,#90086,#90087,#90088,#90089,#90090,#90091,#90092,#90093,#90094,
#90095,#90096,#90097,#90098,#90099,#90100,#90101,#90102,#90103,#90104,#90105,
#90106,#90107,#90108,#90109,#90110,#90111,#90112,#90113,#90114,#90115,#90116,
#90117,#90118,#90119,#90120,#90121,#90122,#90123,#90124,#90125,#90126,#90127,
#90128,#90129,#90130,#90131,#90132,#90133,#90134,#90135,#90136,#90137,#90138,
#90139,#90140,#90141,#90142,#90143,#90144,#90145,#90146,#90147,#90148,#90149,
#90150,#90151,#90152,#90153,#90154,#90155,#90156,#90157,#90158,#90159,#90160,
#90161,#90162,#90163,#90164,#90165,#90166,#90167,#90168,#90169,#90170,#90171,
#90172,#90173,#90174,#90175,#90176,#90177,#90178,#90179,#90180,#90181,#90182,
#90183,#90184,#90185,#90186,#90187,#90188,#90189,#90190,#90191,#90192,#90193,
#90194,#90195,#90196,#90197,#90198,#90199,#90200,#90201,#90202,#90203,#90204,
#90205,#90206,#90207,#90208,#90209),(#90210,#90211,#90212,#90213,#90214,
#90215,#90216,#90217,#90218,#90219,#90220,#90221,#90222,#90223,#90224,#90225,
#90226,#90227,#90228,#90229,#90230,#90231,#90232,#90233,#90234,#90235,#90236,
#90237,#90238,#90239,#90240,#90241,#90242,#90243,#90244,#90245,#90246,#90247,
#90248,#90249,#90250,#90251,#90252,#90253,#90254,#90255,#90256,#90257,#90258,
#90259,#90260,#90261,#90262,#90263,#90264,#90265,#90266,#90267,#90268,#90269,
#90270,#90271,#90272,#90273,#90274,#90275,#90276,#90277,#90278,#90279,#90280,
#90281,#90282,#90283,#90284,#90285,#90286,#90287,#90288,#90289,#90290,#90291,
#90292,#90293,#90294,#90295,#90296,#90297,#90298,#90299,#90300,#90301,#90302,
#90303,#90304,#90305,#90306,#90307,#90308,#90309,#90310,#90311,#90312,#90313,
#90314,#90315,#90316,#90317,#90318,#90319,#90320,#90321,#90322,#90323,#90324,
#90325,#90326,#90327,#90328,#90329,#90330,#90331,#90332,#90333,#90334,#90335,
#90336,#90337,#90338,#90339,#90340),(#90341,#90342,#90343,#90344,#90345,
#90346,#90347,#90348,#90349,#90350,#90351,#90352,#90353,#90354,#90355,#90356,
#90357,#90358,#90359,#90360,#90361,#90362,#90363,#90364,#90365,#90366,#90367,
#90368,#90369,#90370,#90371,#90372,#90373,#90374,#90375,#90376,#90377,#90378,
#90379,#90380,#90381,#90382,#90383,#90384,#90385,#90386,#90387,#90388,#90389,
#90390,#90391,#90392,#90393,#90394,#90395,#90396,#90397,#90398,#90399,#90400,
#90401,#90402,#90403,#90404,#90405,#90406,#90407,#90408,#90409,#90410,#90411,
#90412,#90413,#90414,#90415,#90416,#90417,#90418,#90419,#90420,#90421,#90422,
#90423,#90424,#90425,#90426,#90427,#90428,#90429,#90430,#90431,#90432,#90433,
#90434,#90435,#90436,#90437,#90438,#90439,#90440,#90441,#90442,#90443,#90444,
#90445,#90446,#90447,#90448,#90449,#90450,#90451,#90452,#90453,#90454,#90455,
#90456,#90457,#90458,#90459,#90460,#90461,#90462,#90463,#90464,#90465,#90466,
#90467,#90468,#90469,#90470,#90471)),.UNSPECIFIED.,.F.,.F.,.F.,(4,4),(4,
1,1,1,1,1,1,1,1,1,1,1,1,1,1,1,1,1,1,1,1,1,1,1,1,1,1,1,1,1,1,1,1,1,1,1,1,
1,1,1,1,1,1,1,1,1,1,1,1,1,1,1,1,1,1,1,1,1,1,1,1,1,1,1,1,1,1,1,1,1,1,1,1,
1,1,1,1,1,1,1,1,1,1,1,1,1,1,1,1,1,1,1,1,1,1,1,1,1,1,1,1,1,1,1,1,1,1,1,1,
1,1,1,1,1,1,1,1,1,1,1,1,1,1,1,1,1,1,1,4),(0.,0.0642013499338863),(14.3984001269718,
15.3959052131954,16.393410299419,17.3909153856426,18.3884204718662,19.3859255580897,
20.3834306443133,21.3809357305369,22.3784408167605,23.3759459029841,24.3734509892077,
25.3709560754313,26.3684611616549,27.3659662478785,28.3634713341021,29.3609764203257,
30.3584815065493,31.3559865927729,32.3534916789965,33.3509967652201,34.3485018514437,
35.3460069376673,36.3435120238909,37.3410171101145,38.3385221963381,39.3360272825617,
40.3335323687852,41.3310374550088,42.3285425412324,43.326047627456,44.3235527136796,
45.3210577999032,46.3185628861268,47.3160679723504,48.313573058574,49.3110781447976,
50.3085832310212,51.3060883172448,52.3035934034684,53.301098489692,54.2986035759156,
55.2961086621392,56.2936137483628,57.2911188345864,58.28862392081,59.2861290070336,
60.2836340932571,61.2811391794807,62.2786442657043,63.2761493519279,64.2736544381515,
65.2711595243751,66.2686646105987,67.2661696968223,68.2636747830459,69.2611798692695,
70.2586849554931,71.2561900417167,72.2536951279403,73.2512002141639,74.2487053003875,
75.2462103866111,76.2437154728347,77.2412205590583,78.2387256452819,79.2362307315055,
80.2337358177291,81.2312409039527,82.2287459901763,83.2262510763998,84.2237561626234,
85.221261248847,86.2187663350706,87.2162714212942,88.2137765075178,89.2112815937414,
90.208786679965,91.2062917661886,92.2037968524122,93.2013019386358,94.1988070248594,
95.196312111083,96.1938171973066,97.1913222835302,98.1888273697538,99.1863324559774,
100.183837542201,101.181342628425,102.178847714648,103.176352800872,104.173857887095,
105.171362973319,106.168868059543,107.166373145766,108.16387823199,109.161383318213,
110.158888404437,111.156393490661,112.153898576884,113.151403663108,114.148908749331,
115.146413835555,116.143918921778,117.141424008002,118.138929094226,119.136434180449,
120.133939266673,121.131444352896,122.12894943912,123.126454525344,124.123959611567,
125.121464697791,126.118969784014,127.116474870238,128.113979956462,129.111485042685,
130.108990128909,131.106495215132,132.104000301356,133.10150538758,134.099010473803,
135.096515560027,136.09402064625,137.091525732474,138.089030818698,139.086535904921,
140.084040991145,141.081546077368,142.079051163592),.UNSPECIFIED.);
#1479=B_SPLINE_CURVE_WITH_KNOTS('',3,(#72986,#72987,#72988,#72989),
 .UNSPECIFIED.,.F.,.F.,(4,4),(126.973269284569,127.68065103662),
 .UNSPECIFIED.);
#1480=B_SPLINE_CURVE_WITH_KNOTS('',3,(#72992,#72993,#72994,#72995,#72996,
#72997,#72998,#72999,#73000,#73001),.UNSPECIFIED.,.F.,.F.,(4,3,3,4),(-125.663706143592,
-124.688135777949,-123.690630691726,-123.229495242053),.UNSPECIFIED.);
#1481=B_SPLINE_CURVE_WITH_KNOTS('',3,(#73006,#73007,#73008,#73009,#73010,
#73011,#73012,#73013,#73014,#73015,#73016,#73017,#73018,#73019,#73020,#73021,
#73022,#73023,#73024,#73025,#73026,#73027,#73028,#73029,#73030),
 .UNSPECIFIED.,.F.,.F.,(4,3,3,3,3,3,3,3,4),(120.690083977389,120.698115433055,
121.695620519279,122.693125605502,123.690630691726,124.688135777949,125.685640864173,
126.683145950397,126.973269284569),.UNSPECIFIED.);
#1482=B_SPLINE_CURVE_WITH_KNOTS('',3,(#73031,#73032,#73033,#73034,#73035,
#73036,#73037,#73038,#73039,#73040,#73041,#73042,#73043,#73044,#73045,#73046,
#73047,#73048,#73049,#73050,#73051,#73052),.UNSPECIFIED.,.F.,.F.,(4,3,3,
3,3,3,3,4),(-123.229495242053,-122.693125605502,-121.695620519279,-120.698115433055,
-119.700610346831,-118.703105260608,-117.705600174384,-116.946309934874),
 .UNSPECIFIED.);
#1483=B_SPLINE_CURVE_WITH_KNOTS('',3,(#73057,#73058,#73059,#73060,#73061,
#73062,#73063,#73064,#73065,#73066,#73067,#73068,#73069,#73070,#73071,#73072,
#73073,#73074,#73075,#73076,#73077,#73078),.UNSPECIFIED.,.F.,.F.,(4,3,3,
3,3,3,3,4),(114.40689867021,114.713084915713,115.710590001937,116.708095088161,
117.705600174384,118.703105260608,119.700610346831,120.690083977389),
 .UNSPECIFIED.);
#1484=B_SPLINE_CURVE_WITH_KNOTS('',3,(#73079,#73080,#73081,#73082,#73083,
#73084,#73085,#73086,#73087,#73088,#73089,#73090,#73091,#73092,#73093,#73094,
#73095,#73096,#73097,#73098,#73099,#73100,#73101,#73102,#73103),
 .UNSPECIFIED.,.F.,.F.,(4,3,3,3,3,3,3,3,4),(-116.946309934874,-116.708095088161,
-115.710590001937,-114.713084915713,-113.71557982949,-112.718074743266,
-111.720569657043,-110.723064570819,-110.663124627694),.UNSPECIFIED.);
#1485=B_SPLINE_CURVE_WITH_KNOTS('',3,(#73108,#73109,#73110,#73111,#73112,
#73113,#73114,#73115,#73116,#73117,#73118,#73119,#73120,#73121,#73122,#73123,
#73124,#73125,#73126,#73127,#73128,#73129),.UNSPECIFIED.,.F.,.F.,(4,3,3,
3,3,3,3,4),(108.12371336303,108.728054398372,109.725559484595,110.723064570819,
111.720569657043,112.718074743266,113.71557982949,114.40689867021),
 .UNSPECIFIED.);
#1486=B_SPLINE_CURVE_WITH_KNOTS('',3,(#73130,#73131,#73132,#73133,#73134,
#73135,#73136,#73137,#73138,#73139,#73140,#73141,#73142,#73143,#73144,#73145,
#73146,#73147,#73148,#73149,#73150,#73151),.UNSPECIFIED.,.F.,.F.,(4,3,3,
3,3,3,3,4),(-110.663124627694,-109.725559484595,-108.728054398372,-107.730549312148,
-106.733044225925,-105.735539139701,-104.738034053478,-104.379939320515),
 .UNSPECIFIED.);
#1487=B_SPLINE_CURVE_WITH_KNOTS('',3,(#73156,#73157,#73158,#73159,#73160,
#73161,#73162,#73163,#73164,#73165,#73166,#73167,#73168,#73169,#73170,#73171,
#73172,#73173,#73174,#73175,#73176,#73177),.UNSPECIFIED.,.F.,.F.,(4,3,3,
3,3,3,3,4),(101.840528055851,102.74302388103,103.740528967254,104.738034053477,
105.735539139701,106.733044225925,107.730549312148,108.12371336303),
 .UNSPECIFIED.);
#1488=B_SPLINE_CURVE_WITH_KNOTS('',3,(#73178,#73179,#73180,#73181,#73182,
#73183,#73184,#73185,#73186,#73187,#73188,#73189,#73190,#73191,#73192,#73193,
#73194,#73195,#73196,#73197,#73198,#73199),.UNSPECIFIED.,.F.,.F.,(4,3,3,
3,3,3,3,4),(-104.379939320515,-103.740528967254,-102.74302388103,-101.745518794807,
-100.748013708583,-99.7505086223595,-98.7530035361359,-98.0967540133351),
 .UNSPECIFIED.);
#1489=B_SPLINE_CURVE_WITH_KNOTS('',3,(#73204,#73205,#73206,#73207,#73208,
#73209,#73210,#73211,#73212,#73213,#73214,#73215,#73216,#73217,#73218,#73219,
#73220,#73221,#73222,#73223,#73224,#73225,#73226,#73227,#73228),
 .UNSPECIFIED.,.F.,.F.,(4,3,3,3,3,3,3,3,4),(95.5573427486709,95.7604882774651,
96.7579933636887,97.7554984499123,98.7530035361359,99.7505086223595,100.748013708583,
101.745518794807,101.840528055851),.UNSPECIFIED.);
#1490=B_SPLINE_CURVE_WITH_KNOTS('',3,(#73229,#73230,#73231,#73232,#73233,
#73234,#73235,#73236,#73237,#73238,#73239,#73240,#73241,#73242,#73243,#73244,
#73245,#73246,#73247,#73248,#73249,#73250),.UNSPECIFIED.,.F.,.F.,(4,3,3,
3,3,3,3,4),(-98.0967540133351,-97.7554984499123,-96.7579933636887,-95.7604882774651,
-94.7629831912415,-93.7654781050179,-92.7679730187944,-91.8135687061555),
 .UNSPECIFIED.);
#1491=B_SPLINE_CURVE_WITH_KNOTS('',3,(#73255,#73256,#73257,#73258,#73259,
#73260,#73261,#73262,#73263,#73264,#73265,#73266,#73267,#73268,#73269,#73270,
#73271,#73272,#73273,#73274,#73275,#73276),.UNSPECIFIED.,.F.,.F.,(4,3,3,
3,3,3,3,4),(89.2741574414913,89.7754577601236,90.7729628463471,91.7704679325708,
92.7679730187943,93.7654781050179,94.7629831912415,95.5573427486709),
 .UNSPECIFIED.);
#1492=B_SPLINE_CURVE_WITH_KNOTS('',3,(#73277,#73278,#73279,#73280,#73281,
#73282,#73283,#73284,#73285,#73286,#73287,#73288,#73289,#73290,#73291,#73292,
#73293,#73294,#73295,#73296,#73297,#73298,#73299,#73300,#73301),
 .UNSPECIFIED.,.F.,.F.,(4,3,3,3,3,3,3,3,4),(-91.8135687061555,-91.7704679325708,
-90.7729628463472,-89.7754577601236,-88.7779526739,-87.7804475876764,-86.7829425014528,
-85.7854374152292,-85.5303833989759),.UNSPECIFIED.);
#1493=B_SPLINE_CURVE_WITH_KNOTS('',3,(#73306,#73307,#73308,#73309,#73310,
#73311,#73312,#73313,#73314,#73315,#73316,#73317,#73318,#73319,#73320,#73321,
#73322,#73323,#73324,#73325,#73326,#73327),.UNSPECIFIED.,.F.,.F.,(4,3,3,
3,3,3,3,4),(82.9909721343117,83.790427242782,84.7879323290056,85.7854374152292,
86.7829425014528,87.7804475876764,88.7779526739,89.2741574414913),
 .UNSPECIFIED.);
#1494=B_SPLINE_CURVE_WITH_KNOTS('',3,(#73328,#73329,#73330,#73331,#73332,
#73333,#73334,#73335,#73336,#73337,#73338,#73339,#73340,#73341,#73342,#73343,
#73344,#73345,#73346,#73347,#73348,#73349),.UNSPECIFIED.,.F.,.F.,(4,3,3,
3,3,3,3,4),(-85.5303833989759,-84.7879323290056,-83.790427242782,-82.7929221565584,
-81.7954170703348,-80.7979119841112,-79.8004068978876,-79.2471980917963),
 .UNSPECIFIED.);
#1495=B_SPLINE_CURVE_WITH_KNOTS('',3,(#73354,#73355,#73356,#73357,#73358,
#73359,#73360,#73361,#73362,#73363,#73364,#73365,#73366,#73367,#73368,#73369,
#73370,#73371,#73372,#73373,#73374,#73375,#73376,#73377,#73378),
 .UNSPECIFIED.,.F.,.F.,(4,3,3,3,3,3,3,3,4),(76.7077868271321,76.8078916392168,
77.8053967254404,78.802901811664,79.8004068978876,80.7979119841112,81.7954170703348,
82.7929221565584,82.9909721343117),.UNSPECIFIED.);
#1496=B_SPLINE_CURVE_WITH_KNOTS('',3,(#73379,#73380,#73381,#73382,#73383,
#73384,#73385,#73386,#73387,#73388,#73389,#73390,#73391,#73392,#73393,#73394,
#73395,#73396,#73397,#73398,#73399,#73400),.UNSPECIFIED.,.F.,.F.,(4,3,3,
3,3,3,3,4),(-79.2471980917963,-78.802901811664,-77.8053967254404,-76.8078916392168,
-75.8103865529932,-74.8128814667696,-73.815376380546,-72.9640127846167),
 .UNSPECIFIED.);
#1497=B_SPLINE_CURVE_WITH_KNOTS('',3,(#73405,#73406,#73407,#73408,#73409,
#73410,#73411,#73412,#73413,#73414,#73415,#73416,#73417,#73418,#73419,#73420,
#73421,#73422,#73423,#73424,#73425,#73426),.UNSPECIFIED.,.F.,.F.,(4,3,3,
3,3,3,3,4),(70.4246015199526,70.8228611218752,71.8203662080989,72.8178712943224,
73.815376380546,74.8128814667696,75.8103865529932,76.7077868271321),
 .UNSPECIFIED.);
#1498=B_SPLINE_CURVE_WITH_KNOTS('',3,(#73427,#73428,#73429,#73430,#73431,
#73432,#73433,#73434,#73435,#73436,#73437,#73438,#73439,#73440,#73441,#73442,
#73443,#73444,#73445,#73446,#73447,#73448,#73449,#73450,#73451),
 .UNSPECIFIED.,.F.,.F.,(4,3,3,3,3,3,3,3,4),(-72.9640127846167,-72.8178712943224,
-71.8203662080988,-70.8228611218752,-69.8253560356517,-68.8278509494281,
-67.8303458632045,-66.8328407769809,-66.6808274774371),.UNSPECIFIED.);
#1499=B_SPLINE_CURVE_WITH_KNOTS('',3,(#73456,#73457,#73458,#73459,#73460,
#73461,#73462,#73463,#73464,#73465,#73466,#73467,#73468,#73469,#73470,#73471,
#73472,#73473,#73474,#73475,#73476,#73477),.UNSPECIFIED.,.F.,.F.,(4,3,3,
3,3,3,3,4),(64.141416212773,64.8378306045337,65.8353356907573,66.8328407769809,
67.8303458632045,68.8278509494281,69.8253560356517,70.4246015199526),
 .UNSPECIFIED.);
#1500=B_SPLINE_CURVE_WITH_KNOTS('',3,(#73478,#73479,#73480,#73481,#73482,
#73483,#73484,#73485,#73486,#73487,#73488,#73489,#73490,#73491,#73492,#73493,
#73494,#73495,#73496,#73497,#73498,#73499),.UNSPECIFIED.,.F.,.F.,(4,3,3,
3,3,3,3,4),(-66.6808274774371,-65.8353356907573,-64.8378306045337,-63.8403255183101,
-62.8428204320865,-61.8453153458629,-60.8478102596393,-60.3976421702575),
 .UNSPECIFIED.);
#1501=B_SPLINE_CURVE_WITH_KNOTS('',3,(#73504,#73505,#73506,#73507,#73508,
#73509,#73510,#73511,#73512,#73513,#73514,#73515,#73516,#73517,#73518,#73519,
#73520,#73521,#73522,#73523,#73524,#73525),.UNSPECIFIED.,.F.,.F.,(4,3,3,
3,3,3,3,4),(57.8582309055934,58.8528000871921,59.8503051734157,60.8478102596393,
61.8453153458629,62.8428204320865,63.8403255183101,64.141416212773),
 .UNSPECIFIED.);
#1502=B_SPLINE_CURVE_WITH_KNOTS('',3,(#73526,#73527,#73528,#73529,#73530,
#73531,#73532,#73533,#73534,#73535,#73536,#73537,#73538,#73539,#73540,#73541,
#73542,#73543,#73544,#73545,#73546,#73547),.UNSPECIFIED.,.F.,.F.,(4,3,3,
3,3,3,3,4),(-60.3976421702575,-59.8503051734157,-58.8528000871921,-57.8552950009685,
-56.8577899147449,-55.8602848285214,-54.8627797422977,-54.1144568630779),
 .UNSPECIFIED.);
#1503=B_SPLINE_CURVE_WITH_KNOTS('',3,(#73552,#73553,#73554,#73555,#73556,
#73557,#73558,#73559,#73560,#73561,#73562,#73563,#73564,#73565,#73566,#73567,
#73568,#73569,#73570,#73571,#73572,#73573,#73574,#73575,#73576),
 .UNSPECIFIED.,.F.,.F.,(4,3,3,3,3,3,3,3,4),(51.5750455984138,51.8702644836269,
52.8677695698506,53.8652746560741,54.8627797422977,55.8602848285213,56.8577899147449,
57.8552950009686,57.8582309055934),.UNSPECIFIED.);
#1504=B_SPLINE_CURVE_WITH_KNOTS('',3,(#73577,#73578,#73579,#73580,#73581,
#73582,#73583,#73584,#73585,#73586,#73587,#73588,#73589,#73590,#73591,#73592,
#73593,#73594,#73595,#73596,#73597,#73598,#73599,#73600,#73601),
 .UNSPECIFIED.,.F.,.F.,(4,3,3,3,3,3,3,3,4),(-54.1144568630779,-53.8652746560741,
-52.8677695698505,-51.870264483627,-50.8727593974034,-49.8752543111798,
-48.8777492249562,-47.8802441387326,-47.8312715558983),.UNSPECIFIED.);
#1505=B_SPLINE_CURVE_WITH_KNOTS('',3,(#73606,#73607,#73608,#73609,#73610,
#73611,#73612,#73613,#73614,#73615,#73616,#73617,#73618,#73619,#73620,#73621,
#73622,#73623,#73624,#73625,#73626,#73627),.UNSPECIFIED.,.F.,.F.,(4,3,3,
3,3,3,3,4),(45.2918602912342,45.8852339662854,46.882739052509,47.8802441387326,
48.8777492249562,49.8752543111798,50.8727593974034,51.5750455984138),
 .UNSPECIFIED.);
#1506=B_SPLINE_CURVE_WITH_KNOTS('',3,(#73628,#73629,#73630,#73631,#73632,
#73633,#73634,#73635,#73636,#73637,#73638,#73639,#73640,#73641,#73642,#73643,
#73644,#73645,#73646,#73647,#73648,#73649),.UNSPECIFIED.,.F.,.F.,(4,3,3,
3,3,3,3,4),(-47.8312715558983,-46.882739052509,-45.8852339662854,-44.8877288800618,
-43.8902237938382,-42.8927187076146,-41.895213621391,-41.5480862487187),
 .UNSPECIFIED.);
#1507=B_SPLINE_CURVE_WITH_KNOTS('',3,(#73654,#73655,#73656,#73657,#73658,
#73659,#73660,#73661,#73662,#73663,#73664,#73665,#73666,#73667,#73668,#73669,
#73670,#73671,#73672,#73673,#73674,#73675),.UNSPECIFIED.,.F.,.F.,(4,3,3,
3,3,3,3,4),(39.0086749840546,39.9002034489438,40.8977085351674,41.895213621391,
42.8927187076146,43.8902237938382,44.8877288800618,45.2918602912342),
 .UNSPECIFIED.);
#1508=B_SPLINE_CURVE_WITH_KNOTS('',3,(#73676,#73677,#73678,#73679,#73680,
#73681,#73682,#73683,#73684,#73685,#73686,#73687,#73688,#73689,#73690,#73691,
#73692,#73693,#73694,#73695,#73696,#73697),.UNSPECIFIED.,.F.,.F.,(4,3,3,
3,3,3,3,4),(-41.5480862487187,-40.8977085351674,-39.9002034489438,-38.9026983627202,
-37.9051932764966,-36.907688190273,-35.9101831040494,-35.2649009415391),
 .UNSPECIFIED.);
#1509=B_SPLINE_CURVE_WITH_KNOTS('',3,(#73702,#73703,#73704,#73705,#73706,
#73707,#73708,#73709,#73710,#73711,#73712,#73713,#73714,#73715,#73716,#73717,
#73718,#73719,#73720,#73721,#73722,#73723,#73724,#73725,#73726),
 .UNSPECIFIED.,.F.,.F.,(4,3,3,3,3,3,3,3,4),(32.725489676875,32.9176678453786,
33.9151729316022,34.9126780178258,35.9101831040494,36.907688190273,37.9051932764966,
38.9026983627202,39.0086749840546),.UNSPECIFIED.);
#1510=B_SPLINE_CURVE_WITH_KNOTS('',3,(#73727,#73728,#73729,#73730,#73731,
#73732,#73733,#73734,#73735,#73736,#73737,#73738,#73739,#73740,#73741,#73742,
#73743,#73744,#73745,#73746,#73747,#73748),.UNSPECIFIED.,.F.,.F.,(4,3,3,
3,3,3,3,4),(-35.2649009415391,-34.9126780178258,-33.9151729316022,-32.9176678453786,
-31.920162759155,-30.9226576729315,-29.9251525867079,-28.9817156343596),
 .UNSPECIFIED.);
#1511=B_SPLINE_CURVE_WITH_KNOTS('',3,(#73753,#73754,#73755,#73756,#73757,
#73758,#73759,#73760,#73761,#73762,#73763,#73764,#73765,#73766,#73767,#73768,
#73769,#73770,#73771,#73772,#73773,#73774),.UNSPECIFIED.,.F.,.F.,(4,3,3,
3,3,3,3,4),(26.4423043696954,26.9326373280371,27.9301424142607,28.9276475004843,
29.9251525867079,30.9226576729315,31.920162759155,32.725489676875),
 .UNSPECIFIED.);
#1512=B_SPLINE_CURVE_WITH_KNOTS('',3,(#73775,#73776,#73777,#73778,#73779,
#73780,#73781,#73782,#73783,#73784,#73785,#73786,#73787,#73788,#73789,#73790,
#73791,#73792,#73793,#73794,#73795,#73796,#73797,#73798,#73799),
 .UNSPECIFIED.,.F.,.F.,(4,3,3,3,3,3,3,3,4),(-28.9817156343596,-28.9276475004843,
-27.9301424142607,-26.9326373280371,-25.9351322418135,-24.9376271555899,
-23.9401220693663,-22.9426169831427,-22.69853032718),.UNSPECIFIED.);
#1513=B_SPLINE_CURVE_WITH_KNOTS('',3,(#73804,#73805,#73806,#73807,#73808,
#73809,#73810,#73811,#73812,#73813,#73814,#73815,#73816,#73817,#73818,#73819,
#73820,#73821,#73822,#73823,#73824,#73825),.UNSPECIFIED.,.F.,.F.,(4,3,3,
3,3,3,3,4),(20.1591190625158,20.9476068106955,21.9451118969191,22.9426169831427,
23.9401220693663,24.9376271555899,25.9351322418135,26.4423043696954),
 .UNSPECIFIED.);
#1514=B_SPLINE_CURVE_WITH_KNOTS('',3,(#73826,#73827,#73828,#73829,#73830,
#73831,#73832,#73833,#73834,#73835,#73836,#73837,#73838,#73839,#73840,#73841,
#73842,#73843,#73844,#73845,#73846,#73847),.UNSPECIFIED.,.F.,.F.,(4,3,3,
3,3,3,3,4),(-22.69853032718,-21.9451118969191,-20.9476068106955,-19.9501017244719,
-18.9525966382483,-17.9550915520247,-16.9575864658011,-16.4153450200004),
 .UNSPECIFIED.);
#1515=B_SPLINE_CURVE_WITH_KNOTS('',3,(#73852,#73853,#73854,#73855,#73856,
#73857,#73858,#73859,#73860,#73861,#73862,#73863,#73864,#73865,#73866,#73867,
#73868,#73869,#73870,#73871,#73872,#73873,#73874,#73875,#73876),
 .UNSPECIFIED.,.F.,.F.,(4,3,3,3,3,3,3,3,4),(13.8759337553362,13.9650712071303,
14.9625762933539,15.9600813795775,16.9575864658011,17.9550915520247,18.9525966382483,
19.9501017244719,20.1591190625158),.UNSPECIFIED.);
#1516=B_SPLINE_CURVE_WITH_KNOTS('',3,(#73877,#73878,#73879,#73880,#73881,
#73882,#73883,#73884,#73885,#73886,#73887,#73888,#73889,#73890,#73891,#73892,
#73893,#73894,#73895,#73896,#73897,#73898),.UNSPECIFIED.,.F.,.F.,(4,3,3,
3,3,3,3,4),(-16.4153450200004,-15.9600813795775,-14.9625762933539,-13.9650712071303,
-12.9675661209067,-11.9700610346831,-10.9725559484595,-10.1321597128208),
 .UNSPECIFIED.);
#1517=B_SPLINE_CURVE_WITH_KNOTS('',3,(#73904,#73905,#73906,#73907,#73908,
#73909,#73910,#73911,#73912,#73913,#73914,#73915,#73916),.UNSPECIFIED.,
 .F.,.F.,(4,3,3,3,4),(-3.8489744056412,-2.99251525867078,-1.99501017244719,
-0.997505086223591,0.),.UNSPECIFIED.);
#1518=B_SPLINE_CURVE_WITH_KNOTS('',3,(#73919,#73920,#73921,#73922,#73923,
#73924,#73925,#73926,#73927,#73928,#73929,#73930,#73931,#73932,#73933,#73934,
#73935,#73936,#73937),.UNSPECIFIED.,.F.,.F.,(4,3,3,3,3,3,4),(2.01694489302841,
2.99251525867078,3.99002034489438,4.98752543111797,5.98503051734157,6.98253560356516,
7.59274844815666),.UNSPECIFIED.);
#1519=B_SPLINE_CURVE_WITH_KNOTS('',3,(#73943,#73944,#73945,#73946),
 .UNSPECIFIED.,.F.,.F.,(4,4),(126.973269284569,127.68065103662),
 .UNSPECIFIED.);
#1520=B_SPLINE_CURVE_WITH_KNOTS('',3,(#73949,#73950,#73951,#73952,#73953,
#73954,#73955,#73956,#73957,#73958),.UNSPECIFIED.,.F.,.F.,(4,3,3,4),(-125.663706143592,
-124.688135777949,-123.690630691726,-123.229495242053),.UNSPECIFIED.);
#1521=B_SPLINE_CURVE_WITH_KNOTS('',3,(#73963,#73964,#73965,#73966,#73967,
#73968,#73969,#73970,#73971,#73972,#73973,#73974,#73975,#73976,#73977,#73978,
#73979,#73980,#73981,#73982,#73983,#73984,#73985,#73986,#73987),
 .UNSPECIFIED.,.F.,.F.,(4,3,3,3,3,3,3,3,4),(120.690083977389,120.698115433055,
121.695620519279,122.693125605502,123.690630691726,124.688135777949,125.685640864173,
126.683145950397,126.973269284569),.UNSPECIFIED.);
#1522=B_SPLINE_CURVE_WITH_KNOTS('',3,(#73988,#73989,#73990,#73991,#73992,
#73993,#73994,#73995,#73996,#73997,#73998,#73999,#74000,#74001,#74002,#74003,
#74004,#74005,#74006,#74007,#74008,#74009),.UNSPECIFIED.,.F.,.F.,(4,3,3,
3,3,3,3,4),(-123.229495242053,-122.693125605502,-121.695620519279,-120.698115433055,
-119.700610346831,-118.703105260608,-117.705600174384,-116.946309934874),
 .UNSPECIFIED.);
#1523=B_SPLINE_CURVE_WITH_KNOTS('',3,(#74014,#74015,#74016,#74017,#74018,
#74019,#74020,#74021,#74022,#74023,#74024,#74025,#74026,#74027,#74028,#74029,
#74030,#74031,#74032,#74033,#74034,#74035),.UNSPECIFIED.,.F.,.F.,(4,3,3,
3,3,3,3,4),(114.40689867021,114.713084915713,115.710590001937,116.708095088161,
117.705600174384,118.703105260608,119.700610346831,120.690083977389),
 .UNSPECIFIED.);
#1524=B_SPLINE_CURVE_WITH_KNOTS('',3,(#74036,#74037,#74038,#74039,#74040,
#74041,#74042,#74043,#74044,#74045,#74046,#74047,#74048,#74049,#74050,#74051,
#74052,#74053,#74054,#74055,#74056,#74057,#74058,#74059,#74060),
 .UNSPECIFIED.,.F.,.F.,(4,3,3,3,3,3,3,3,4),(-116.946309934874,-116.708095088161,
-115.710590001937,-114.713084915713,-113.71557982949,-112.718074743266,
-111.720569657043,-110.723064570819,-110.663124627694),.UNSPECIFIED.);
#1525=B_SPLINE_CURVE_WITH_KNOTS('',3,(#74065,#74066,#74067,#74068,#74069,
#74070,#74071,#74072,#74073,#74074,#74075,#74076,#74077,#74078,#74079,#74080,
#74081,#74082,#74083,#74084,#74085,#74086),.UNSPECIFIED.,.F.,.F.,(4,3,3,
3,3,3,3,4),(108.12371336303,108.728054398372,109.725559484595,110.723064570819,
111.720569657043,112.718074743266,113.71557982949,114.40689867021),
 .UNSPECIFIED.);
#1526=B_SPLINE_CURVE_WITH_KNOTS('',3,(#74087,#74088,#74089,#74090,#74091,
#74092,#74093,#74094,#74095,#74096,#74097,#74098,#74099,#74100,#74101,#74102,
#74103,#74104,#74105,#74106,#74107,#74108),.UNSPECIFIED.,.F.,.F.,(4,3,3,
3,3,3,3,4),(-110.663124627694,-109.725559484595,-108.728054398372,-107.730549312148,
-106.733044225925,-105.735539139701,-104.738034053477,-104.379939320515),
 .UNSPECIFIED.);
#1527=B_SPLINE_CURVE_WITH_KNOTS('',3,(#74113,#74114,#74115,#74116,#74117,
#74118,#74119,#74120,#74121,#74122,#74123,#74124,#74125,#74126,#74127,#74128,
#74129,#74130,#74131,#74132,#74133,#74134),.UNSPECIFIED.,.F.,.F.,(4,3,3,
3,3,3,3,4),(101.84052805585,102.74302388103,103.740528967254,104.738034053477,
105.735539139701,106.733044225925,107.730549312148,108.12371336303),
 .UNSPECIFIED.);
#1528=B_SPLINE_CURVE_WITH_KNOTS('',3,(#74135,#74136,#74137,#74138,#74139,
#74140,#74141,#74142,#74143,#74144,#74145,#74146,#74147,#74148,#74149,#74150,
#74151,#74152,#74153,#74154,#74155,#74156),.UNSPECIFIED.,.F.,.F.,(4,3,3,
3,3,3,3,4),(-104.379939320515,-103.740528967254,-102.74302388103,-101.745518794807,
-100.748013708583,-99.7505086223595,-98.7530035361359,-98.096754013335),
 .UNSPECIFIED.);
#1529=B_SPLINE_CURVE_WITH_KNOTS('',3,(#74161,#74162,#74163,#74164,#74165,
#74166,#74167,#74168,#74169,#74170,#74171,#74172,#74173,#74174,#74175,#74176,
#74177,#74178,#74179,#74180,#74181,#74182,#74183,#74184,#74185),
 .UNSPECIFIED.,.F.,.F.,(4,3,3,3,3,3,3,3,4),(95.5573427486709,95.7604882774651,
96.7579933636887,97.7554984499123,98.7530035361359,99.7505086223595,100.748013708583,
101.745518794807,101.84052805585),.UNSPECIFIED.);
#1530=B_SPLINE_CURVE_WITH_KNOTS('',3,(#74186,#74187,#74188,#74189,#74190,
#74191,#74192,#74193,#74194,#74195,#74196,#74197,#74198,#74199,#74200,#74201,
#74202,#74203,#74204,#74205,#74206,#74207),.UNSPECIFIED.,.F.,.F.,(4,3,3,
3,3,3,3,4),(-98.096754013335,-97.7554984499123,-96.7579933636887,-95.7604882774651,
-94.7629831912415,-93.7654781050179,-92.7679730187943,-91.8135687061554),
 .UNSPECIFIED.);
#1531=B_SPLINE_CURVE_WITH_KNOTS('',3,(#74212,#74213,#74214,#74215,#74216,
#74217,#74218,#74219,#74220,#74221,#74222,#74223,#74224,#74225,#74226,#74227,
#74228,#74229,#74230,#74231,#74232,#74233),.UNSPECIFIED.,.F.,.F.,(4,3,3,
3,3,3,3,4),(89.2741574414913,89.7754577601235,90.7729628463471,91.7704679325707,
92.7679730187943,93.7654781050179,94.7629831912415,95.5573427486709),
 .UNSPECIFIED.);
#1532=B_SPLINE_CURVE_WITH_KNOTS('',3,(#74234,#74235,#74236,#74237,#74238,
#74239,#74240,#74241,#74242,#74243,#74244,#74245,#74246,#74247,#74248,#74249,
#74250,#74251,#74252,#74253,#74254,#74255,#74256,#74257,#74258),
 .UNSPECIFIED.,.F.,.F.,(4,3,3,3,3,3,3,3,4),(-91.8135687061554,-91.7704679325708,
-90.7729628463471,-89.7754577601236,-88.7779526739,-87.7804475876764,-86.7829425014528,
-85.7854374152292,-85.5303833989758),.UNSPECIFIED.);
#1533=B_SPLINE_CURVE_WITH_KNOTS('',3,(#74263,#74264,#74265,#74266,#74267,
#74268,#74269,#74270,#74271,#74272,#74273,#74274,#74275,#74276,#74277,#74278,
#74279,#74280,#74281,#74282,#74283,#74284),.UNSPECIFIED.,.F.,.F.,(4,3,3,
3,3,3,3,4),(82.9909721343117,83.790427242782,84.7879323290056,85.7854374152292,
86.7829425014528,87.7804475876763,88.7779526739,89.2741574414913),
 .UNSPECIFIED.);
#1534=B_SPLINE_CURVE_WITH_KNOTS('',3,(#74285,#74286,#74287,#74288,#74289,
#74290,#74291,#74292,#74293,#74294,#74295,#74296,#74297,#74298,#74299,#74300,
#74301,#74302,#74303,#74304,#74305,#74306),.UNSPECIFIED.,.F.,.F.,(4,3,3,
3,3,3,3,4),(-85.5303833989758,-84.7879323290056,-83.790427242782,-82.7929221565584,
-81.7954170703348,-80.7979119841112,-79.8004068978876,-79.2471980917962),
 .UNSPECIFIED.);
#1535=B_SPLINE_CURVE_WITH_KNOTS('',3,(#74311,#74312,#74313,#74314,#74315,
#74316,#74317,#74318,#74319,#74320,#74321,#74322,#74323,#74324,#74325,#74326,
#74327,#74328,#74329,#74330,#74331,#74332,#74333,#74334,#74335),
 .UNSPECIFIED.,.F.,.F.,(4,3,3,3,3,3,3,3,4),(76.7077868271321,76.8078916392168,
77.8053967254404,78.802901811664,79.8004068978876,80.7979119841112,81.7954170703348,
82.7929221565584,82.9909721343117),.UNSPECIFIED.);
#1536=B_SPLINE_CURVE_WITH_KNOTS('',3,(#74336,#74337,#74338,#74339,#74340,
#74341,#74342,#74343,#74344,#74345,#74346,#74347,#74348,#74349,#74350,#74351,
#74352,#74353,#74354,#74355,#74356,#74357),.UNSPECIFIED.,.F.,.F.,(4,3,3,
3,3,3,3,4),(-79.2471980917962,-78.802901811664,-77.8053967254404,-76.8078916392168,
-75.8103865529932,-74.8128814667696,-73.815376380546,-72.9640127846167),
 .UNSPECIFIED.);
#1537=B_SPLINE_CURVE_WITH_KNOTS('',3,(#74362,#74363,#74364,#74365,#74366,
#74367,#74368,#74369,#74370,#74371,#74372,#74373,#74374,#74375,#74376,#74377,
#74378,#74379,#74380,#74381,#74382,#74383),.UNSPECIFIED.,.F.,.F.,(4,3,3,
3,3,3,3,4),(70.4246015199525,70.8228611218752,71.8203662080988,72.8178712943224,
73.815376380546,74.8128814667696,75.8103865529932,76.7077868271321),
 .UNSPECIFIED.);
#1538=B_SPLINE_CURVE_WITH_KNOTS('',3,(#74384,#74385,#74386,#74387,#74388,
#74389,#74390,#74391,#74392,#74393,#74394,#74395,#74396,#74397,#74398,#74399,
#74400,#74401,#74402,#74403,#74404,#74405,#74406,#74407,#74408),
 .UNSPECIFIED.,.F.,.F.,(4,3,3,3,3,3,3,3,4),(-72.9640127846167,-72.8178712943224,
-71.8203662080988,-70.8228611218752,-69.8253560356517,-68.827850949428,
-67.8303458632045,-66.8328407769809,-66.680827477437),.UNSPECIFIED.);
#1539=B_SPLINE_CURVE_WITH_KNOTS('',3,(#74413,#74414,#74415,#74416,#74417,
#74418,#74419,#74420,#74421,#74422,#74423,#74424,#74425,#74426,#74427,#74428,
#74429,#74430,#74431,#74432,#74433,#74434),.UNSPECIFIED.,.F.,.F.,(4,3,3,
3,3,3,3,4),(64.1414162127729,64.8378306045337,65.8353356907573,66.8328407769808,
67.8303458632045,68.827850949428,69.8253560356517,70.4246015199525),
 .UNSPECIFIED.);
#1540=B_SPLINE_CURVE_WITH_KNOTS('',3,(#74435,#74436,#74437,#74438,#74439,
#74440,#74441,#74442,#74443,#74444,#74445,#74446,#74447,#74448,#74449,#74450,
#74451,#74452,#74453,#74454,#74455,#74456),.UNSPECIFIED.,.F.,.F.,(4,3,3,
3,3,3,3,4),(-66.680827477437,-65.8353356907573,-64.8378306045337,-63.8403255183101,
-62.8428204320865,-61.8453153458629,-60.8478102596393,-60.3976421702575),
 .UNSPECIFIED.);
#1541=B_SPLINE_CURVE_WITH_KNOTS('',3,(#74461,#74462,#74463,#74464,#74465,
#74466,#74467,#74468,#74469,#74470,#74471,#74472,#74473,#74474,#74475,#74476,
#74477,#74478,#74479,#74480,#74481,#74482),.UNSPECIFIED.,.F.,.F.,(4,3,3,
3,3,3,3,4),(57.8582309055933,58.8528000871921,59.8503051734157,60.8478102596393,
61.8453153458629,62.8428204320865,63.8403255183101,64.1414162127729),
 .UNSPECIFIED.);
#1542=B_SPLINE_CURVE_WITH_KNOTS('',3,(#74483,#74484,#74485,#74486,#74487,
#74488,#74489,#74490,#74491,#74492,#74493,#74494,#74495,#74496,#74497,#74498,
#74499,#74500,#74501,#74502,#74503,#74504),.UNSPECIFIED.,.F.,.F.,(4,3,3,
3,3,3,3,4),(-60.3976421702575,-59.8503051734157,-58.8528000871921,-57.8552950009685,
-56.8577899147449,-55.8602848285213,-54.8627797422977,-54.1144568630779),
 .UNSPECIFIED.);
#1543=B_SPLINE_CURVE_WITH_KNOTS('',3,(#74509,#74510,#74511,#74512,#74513,
#74514,#74515,#74516,#74517,#74518,#74519,#74520,#74521,#74522,#74523,#74524,
#74525,#74526,#74527,#74528,#74529,#74530,#74531,#74532,#74533),
 .UNSPECIFIED.,.F.,.F.,(4,3,3,3,3,3,3,3,4),(51.5750455984137,51.8702644836269,
52.8677695698505,53.8652746560741,54.8627797422977,55.8602848285213,56.8577899147449,
57.8552950009685,57.8582309055933),.UNSPECIFIED.);
#1544=B_SPLINE_CURVE_WITH_KNOTS('',3,(#74534,#74535,#74536,#74537,#74538,
#74539,#74540,#74541,#74542,#74543,#74544,#74545,#74546,#74547,#74548,#74549,
#74550,#74551,#74552,#74553,#74554,#74555,#74556,#74557,#74558),
 .UNSPECIFIED.,.F.,.F.,(4,3,3,3,3,3,3,3,4),(-54.1144568630779,-53.8652746560741,
-52.8677695698505,-51.8702644836269,-50.8727593974033,-49.8752543111797,
-48.8777492249561,-47.8802441387326,-47.8312715558983),.UNSPECIFIED.);
#1545=B_SPLINE_CURVE_WITH_KNOTS('',3,(#74563,#74564,#74565,#74566,#74567,
#74568,#74569,#74570,#74571,#74572,#74573,#74574,#74575,#74576,#74577,#74578,
#74579,#74580,#74581,#74582,#74583,#74584),.UNSPECIFIED.,.F.,.F.,(4,3,3,
3,3,3,3,4),(45.2918602912341,45.8852339662854,46.882739052509,47.8802441387326,
48.8777492249562,49.8752543111798,50.8727593974033,51.5750455984137),
 .UNSPECIFIED.);
#1546=B_SPLINE_CURVE_WITH_KNOTS('',3,(#74585,#74586,#74587,#74588,#74589,
#74590,#74591,#74592,#74593,#74594,#74595,#74596,#74597,#74598,#74599,#74600,
#74601,#74602,#74603,#74604,#74605,#74606),.UNSPECIFIED.,.F.,.F.,(4,3,3,
3,3,3,3,4),(-47.8312715558983,-46.882739052509,-45.8852339662854,-44.8877288800618,
-43.8902237938382,-42.8927187076146,-41.895213621391,-41.5480862487187),
 .UNSPECIFIED.);
#1547=B_SPLINE_CURVE_WITH_KNOTS('',3,(#74611,#74612,#74613,#74614,#74615,
#74616,#74617,#74618,#74619,#74620,#74621,#74622,#74623,#74624,#74625,#74626,
#74627,#74628,#74629,#74630,#74631,#74632),.UNSPECIFIED.,.F.,.F.,(4,3,3,
3,3,3,3,4),(39.0086749840545,39.9002034489438,40.8977085351674,41.895213621391,
42.8927187076146,43.8902237938382,44.8877288800618,45.2918602912341),
 .UNSPECIFIED.);
#1548=B_SPLINE_CURVE_WITH_KNOTS('',3,(#74633,#74634,#74635,#74636,#74637,
#74638,#74639,#74640,#74641,#74642,#74643,#74644,#74645,#74646,#74647,#74648,
#74649,#74650,#74651,#74652,#74653,#74654),.UNSPECIFIED.,.F.,.F.,(4,3,3,
3,3,3,3,4),(-41.5480862487187,-40.8977085351674,-39.9002034489438,-38.9026983627202,
-37.9051932764966,-36.907688190273,-35.9101831040494,-35.2649009415391),
 .UNSPECIFIED.);
#1549=B_SPLINE_CURVE_WITH_KNOTS('',3,(#74659,#74660,#74661,#74662,#74663,
#74664,#74665,#74666,#74667,#74668,#74669,#74670,#74671,#74672,#74673,#74674,
#74675,#74676,#74677,#74678,#74679,#74680,#74681,#74682,#74683),
 .UNSPECIFIED.,.F.,.F.,(4,3,3,3,3,3,3,3,4),(32.725489676875,32.9176678453786,
33.9151729316022,34.9126780178258,35.9101831040494,36.907688190273,37.9051932764966,
38.9026983627202,39.0086749840545),.UNSPECIFIED.);
#1550=B_SPLINE_CURVE_WITH_KNOTS('',3,(#74684,#74685,#74686,#74687,#74688,
#74689,#74690,#74691,#74692,#74693,#74694,#74695,#74696,#74697,#74698,#74699,
#74700,#74701,#74702,#74703,#74704,#74705),.UNSPECIFIED.,.F.,.F.,(4,3,3,
3,3,3,3,4),(-35.2649009415391,-34.9126780178258,-33.9151729316022,-32.9176678453786,
-31.920162759155,-30.9226576729314,-29.9251525867078,-28.9817156343595),
 .UNSPECIFIED.);
#1551=B_SPLINE_CURVE_WITH_KNOTS('',3,(#74710,#74711,#74712,#74713,#74714,
#74715,#74716,#74717,#74718,#74719,#74720,#74721,#74722,#74723,#74724,#74725,
#74726,#74727,#74728,#74729,#74730,#74731),.UNSPECIFIED.,.F.,.F.,(4,3,3,
3,3,3,3,4),(26.4423043696954,26.9326373280371,27.9301424142607,28.9276475004843,
29.9251525867078,30.9226576729314,31.920162759155,32.725489676875),
 .UNSPECIFIED.);
#1552=B_SPLINE_CURVE_WITH_KNOTS('',3,(#74732,#74733,#74734,#74735,#74736,
#74737,#74738,#74739,#74740,#74741,#74742,#74743,#74744,#74745,#74746,#74747,
#74748,#74749,#74750,#74751,#74752,#74753,#74754,#74755,#74756),
 .UNSPECIFIED.,.F.,.F.,(4,3,3,3,3,3,3,3,4),(-28.9817156343595,-28.9276475004842,
-27.9301424142607,-26.9326373280371,-25.9351322418135,-24.9376271555899,
-23.9401220693663,-22.9426169831427,-22.6985303271799),.UNSPECIFIED.);
#1553=B_SPLINE_CURVE_WITH_KNOTS('',3,(#74761,#74762,#74763,#74764,#74765,
#74766,#74767,#74768,#74769,#74770,#74771,#74772,#74773,#74774,#74775,#74776,
#74777,#74778,#74779,#74780,#74781,#74782),.UNSPECIFIED.,.F.,.F.,(4,3,3,
3,3,3,3,4),(20.1591190625158,20.9476068106955,21.9451118969191,22.9426169831427,
23.9401220693663,24.9376271555899,25.9351322418135,26.4423043696954),
 .UNSPECIFIED.);
#1554=B_SPLINE_CURVE_WITH_KNOTS('',3,(#74783,#74784,#74785,#74786,#74787,
#74788,#74789,#74790,#74791,#74792,#74793,#74794,#74795,#74796,#74797,#74798,
#74799,#74800,#74801,#74802,#74803,#74804),.UNSPECIFIED.,.F.,.F.,(4,3,3,
3,3,3,3,4),(-22.6985303271799,-21.9451118969191,-20.9476068106955,-19.9501017244719,
-18.9525966382483,-17.9550915520247,-16.9575864658011,-16.4153450200003),
 .UNSPECIFIED.);
#1555=B_SPLINE_CURVE_WITH_KNOTS('',3,(#74809,#74810,#74811,#74812,#74813,
#74814,#74815,#74816,#74817,#74818,#74819,#74820,#74821,#74822,#74823,#74824,
#74825,#74826,#74827,#74828,#74829,#74830,#74831,#74832,#74833),
 .UNSPECIFIED.,.F.,.F.,(4,3,3,3,3,3,3,3,4),(13.8759337553362,13.9650712071303,
14.9625762933539,15.9600813795775,16.9575864658011,17.9550915520247,18.9525966382483,
19.9501017244719,20.1591190625158),.UNSPECIFIED.);
#1556=B_SPLINE_CURVE_WITH_KNOTS('',3,(#74834,#74835,#74836,#74837,#74838,
#74839,#74840,#74841,#74842,#74843,#74844,#74845,#74846,#74847,#74848,#74849,
#74850,#74851,#74852,#74853,#74854,#74855),.UNSPECIFIED.,.F.,.F.,(4,3,3,
3,3,3,3,4),(-16.4153450200003,-15.9600813795775,-14.9625762933539,-13.9650712071303,
-12.9675661209067,-11.9700610346831,-10.9725559484595,-10.1321597128207),
 .UNSPECIFIED.);
#1557=B_SPLINE_CURVE_WITH_KNOTS('',3,(#74861,#74862,#74863,#74864,#74865,
#74866,#74867,#74868,#74869,#74870,#74871,#74872,#74873),.UNSPECIFIED.,
 .F.,.F.,(4,3,3,3,4),(-3.84897440564117,-2.99251525867078,-1.99501017244719,
-0.997505086223592,0.),.UNSPECIFIED.);
#1558=B_SPLINE_CURVE_WITH_KNOTS('',3,(#74876,#74877,#74878,#74879,#74880,
#74881,#74882,#74883,#74884,#74885,#74886,#74887,#74888,#74889,#74890,#74891,
#74892,#74893,#74894),.UNSPECIFIED.,.F.,.F.,(4,3,3,3,3,3,4),(2.01694489302822,
2.99251525867079,3.99002034489439,4.98752543111798,5.98503051734158,6.98253560356517,
7.59274844815661),.UNSPECIFIED.);
#1559=B_SPLINE_CURVE_WITH_KNOTS('',3,(#74900,#74901,#74902,#74903),
 .UNSPECIFIED.,.F.,.F.,(4,4),(126.973269284569,127.68065103662),
 .UNSPECIFIED.);
#1560=B_SPLINE_CURVE_WITH_KNOTS('',3,(#74906,#74907,#74908,#74909,#74910,
#74911,#74912,#74913,#74914,#74915),.UNSPECIFIED.,.F.,.F.,(4,3,3,4),(-125.663706143592,
-124.688135777949,-123.690630691726,-123.229495242053),.UNSPECIFIED.);
#1561=B_SPLINE_CURVE_WITH_KNOTS('',3,(#74920,#74921,#74922,#74923,#74924,
#74925,#74926,#74927,#74928,#74929,#74930,#74931,#74932,#74933,#74934,#74935,
#74936,#74937,#74938,#74939,#74940,#74941,#74942,#74943,#74944),
 .UNSPECIFIED.,.F.,.F.,(4,3,3,3,3,3,3,3,4),(120.690083977389,120.698115433055,
121.695620519279,122.693125605502,123.690630691726,124.688135777949,125.685640864173,
126.683145950397,126.973269284569),.UNSPECIFIED.);
#1562=B_SPLINE_CURVE_WITH_KNOTS('',3,(#74945,#74946,#74947,#74948,#74949,
#74950,#74951,#74952,#74953,#74954,#74955,#74956,#74957,#74958,#74959,#74960,
#74961,#74962,#74963,#74964,#74965,#74966),.UNSPECIFIED.,.F.,.F.,(4,3,3,
3,3,3,3,4),(-123.229495242053,-122.693125605502,-121.695620519279,-120.698115433055,
-119.700610346831,-118.703105260608,-117.705600174384,-116.946309934874),
 .UNSPECIFIED.);
#1563=B_SPLINE_CURVE_WITH_KNOTS('',3,(#74971,#74972,#74973,#74974,#74975,
#74976,#74977,#74978,#74979,#74980,#74981,#74982,#74983,#74984,#74985,#74986,
#74987,#74988,#74989,#74990,#74991,#74992),.UNSPECIFIED.,.F.,.F.,(4,3,3,
3,3,3,3,4),(114.40689867021,114.713084915713,115.710590001937,116.708095088161,
117.705600174384,118.703105260608,119.700610346831,120.690083977389),
 .UNSPECIFIED.);
#1564=B_SPLINE_CURVE_WITH_KNOTS('',3,(#74993,#74994,#74995,#74996,#74997,
#74998,#74999,#75000,#75001,#75002,#75003,#75004,#75005,#75006,#75007,#75008,
#75009,#75010,#75011,#75012,#75013,#75014,#75015,#75016,#75017),
 .UNSPECIFIED.,.F.,.F.,(4,3,3,3,3,3,3,3,4),(-116.946309934874,-116.708095088161,
-115.710590001937,-114.713084915713,-113.71557982949,-112.718074743266,
-111.720569657043,-110.723064570819,-110.663124627694),.UNSPECIFIED.);
#1565=B_SPLINE_CURVE_WITH_KNOTS('',3,(#75022,#75023,#75024,#75025,#75026,
#75027,#75028,#75029,#75030,#75031,#75032,#75033,#75034,#75035,#75036,#75037,
#75038,#75039,#75040,#75041,#75042,#75043),.UNSPECIFIED.,.F.,.F.,(4,3,3,
3,3,3,3,4),(108.12371336303,108.728054398372,109.725559484595,110.723064570819,
111.720569657043,112.718074743266,113.71557982949,114.40689867021),
 .UNSPECIFIED.);
#1566=B_SPLINE_CURVE_WITH_KNOTS('',3,(#75044,#75045,#75046,#75047,#75048,
#75049,#75050,#75051,#75052,#75053,#75054,#75055,#75056,#75057,#75058,#75059,
#75060,#75061,#75062,#75063,#75064,#75065),.UNSPECIFIED.,.F.,.F.,(4,3,3,
3,3,3,3,4),(-110.663124627694,-109.725559484595,-108.728054398372,-107.730549312148,
-106.733044225925,-105.735539139701,-104.738034053477,-104.379939320515),
 .UNSPECIFIED.);
#1567=B_SPLINE_CURVE_WITH_KNOTS('',3,(#75070,#75071,#75072,#75073,#75074,
#75075,#75076,#75077,#75078,#75079,#75080,#75081,#75082,#75083,#75084,#75085,
#75086,#75087,#75088,#75089,#75090,#75091),.UNSPECIFIED.,.F.,.F.,(4,3,3,
3,3,3,3,4),(101.84052805585,102.74302388103,103.740528967254,104.738034053477,
105.735539139701,106.733044225925,107.730549312148,108.12371336303),
 .UNSPECIFIED.);
#1568=B_SPLINE_CURVE_WITH_KNOTS('',3,(#75092,#75093,#75094,#75095,#75096,
#75097,#75098,#75099,#75100,#75101,#75102,#75103,#75104,#75105,#75106,#75107,
#75108,#75109,#75110,#75111,#75112,#75113),.UNSPECIFIED.,.F.,.F.,(4,3,3,
3,3,3,3,4),(-104.379939320515,-103.740528967254,-102.74302388103,-101.745518794807,
-100.748013708583,-99.7505086223595,-98.7530035361359,-98.096754013335),
 .UNSPECIFIED.);
#1569=B_SPLINE_CURVE_WITH_KNOTS('',3,(#75118,#75119,#75120,#75121,#75122,
#75123,#75124,#75125,#75126,#75127,#75128,#75129,#75130,#75131,#75132,#75133,
#75134,#75135,#75136,#75137,#75138,#75139,#75140,#75141,#75142),
 .UNSPECIFIED.,.F.,.F.,(4,3,3,3,3,3,3,3,4),(95.5573427486709,95.7604882774651,
96.7579933636887,97.7554984499123,98.7530035361359,99.7505086223595,100.748013708583,
101.745518794807,101.84052805585),.UNSPECIFIED.);
#1570=B_SPLINE_CURVE_WITH_KNOTS('',3,(#75143,#75144,#75145,#75146,#75147,
#75148,#75149,#75150,#75151,#75152,#75153,#75154,#75155,#75156,#75157,#75158,
#75159,#75160,#75161,#75162,#75163,#75164),.UNSPECIFIED.,.F.,.F.,(4,3,3,
3,3,3,3,4),(-98.096754013335,-97.7554984499123,-96.7579933636887,-95.7604882774651,
-94.7629831912415,-93.7654781050179,-92.7679730187943,-91.8135687061554),
 .UNSPECIFIED.);
#1571=B_SPLINE_CURVE_WITH_KNOTS('',3,(#75169,#75170,#75171,#75172,#75173,
#75174,#75175,#75176,#75177,#75178,#75179,#75180,#75181,#75182,#75183,#75184,
#75185,#75186,#75187,#75188,#75189,#75190),.UNSPECIFIED.,.F.,.F.,(4,3,3,
3,3,3,3,4),(89.2741574414913,89.7754577601236,90.7729628463471,91.7704679325707,
92.7679730187943,93.7654781050179,94.7629831912415,95.5573427486709),
 .UNSPECIFIED.);
#1572=B_SPLINE_CURVE_WITH_KNOTS('',3,(#75191,#75192,#75193,#75194,#75195,
#75196,#75197,#75198,#75199,#75200,#75201,#75202,#75203,#75204,#75205,#75206,
#75207,#75208,#75209,#75210,#75211,#75212,#75213,#75214,#75215),
 .UNSPECIFIED.,.F.,.F.,(4,3,3,3,3,3,3,3,4),(-91.8135687061554,-91.7704679325708,
-90.7729628463472,-89.7754577601236,-88.7779526739,-87.7804475876764,-86.7829425014528,
-85.7854374152292,-85.5303833989758),.UNSPECIFIED.);
#1573=B_SPLINE_CURVE_WITH_KNOTS('',3,(#75220,#75221,#75222,#75223,#75224,
#75225,#75226,#75227,#75228,#75229,#75230,#75231,#75232,#75233,#75234,#75235,
#75236,#75237,#75238,#75239,#75240,#75241),.UNSPECIFIED.,.F.,.F.,(4,3,3,
3,3,3,3,4),(82.9909721343117,83.790427242782,84.7879323290056,85.7854374152292,
86.7829425014528,87.7804475876764,88.7779526739,89.2741574414913),
 .UNSPECIFIED.);
#1574=B_SPLINE_CURVE_WITH_KNOTS('',3,(#75242,#75243,#75244,#75245,#75246,
#75247,#75248,#75249,#75250,#75251,#75252,#75253,#75254,#75255,#75256,#75257,
#75258,#75259,#75260,#75261,#75262,#75263),.UNSPECIFIED.,.F.,.F.,(4,3,3,
3,3,3,3,4),(-85.5303833989758,-84.7879323290056,-83.790427242782,-82.7929221565584,
-81.7954170703348,-80.7979119841112,-79.8004068978876,-79.2471980917962),
 .UNSPECIFIED.);
#1575=B_SPLINE_CURVE_WITH_KNOTS('',3,(#75268,#75269,#75270,#75271,#75272,
#75273,#75274,#75275,#75276,#75277,#75278,#75279,#75280,#75281,#75282,#75283,
#75284,#75285,#75286,#75287,#75288,#75289,#75290,#75291,#75292),
 .UNSPECIFIED.,.F.,.F.,(4,3,3,3,3,3,3,3,4),(76.7077868271321,76.8078916392168,
77.8053967254404,78.802901811664,79.8004068978876,80.7979119841112,81.7954170703348,
82.7929221565584,82.9909721343117),.UNSPECIFIED.);
#1576=B_SPLINE_CURVE_WITH_KNOTS('',3,(#75293,#75294,#75295,#75296,#75297,
#75298,#75299,#75300,#75301,#75302,#75303,#75304,#75305,#75306,#75307,#75308,
#75309,#75310,#75311,#75312,#75313,#75314),.UNSPECIFIED.,.F.,.F.,(4,3,3,
3,3,3,3,4),(-79.2471980917962,-78.802901811664,-77.8053967254404,-76.8078916392168,
-75.8103865529932,-74.8128814667696,-73.815376380546,-72.9640127846166),
 .UNSPECIFIED.);
#1577=B_SPLINE_CURVE_WITH_KNOTS('',3,(#75319,#75320,#75321,#75322,#75323,
#75324,#75325,#75326,#75327,#75328,#75329,#75330,#75331,#75332,#75333,#75334,
#75335,#75336,#75337,#75338,#75339,#75340),.UNSPECIFIED.,.F.,.F.,(4,3,3,
3,3,3,3,4),(70.4246015199525,70.8228611218752,71.8203662080988,72.8178712943224,
73.815376380546,74.8128814667696,75.8103865529932,76.7077868271321),
 .UNSPECIFIED.);
#1578=B_SPLINE_CURVE_WITH_KNOTS('',3,(#75341,#75342,#75343,#75344,#75345,
#75346,#75347,#75348,#75349,#75350,#75351,#75352,#75353,#75354,#75355,#75356,
#75357,#75358,#75359,#75360,#75361,#75362,#75363,#75364,#75365),
 .UNSPECIFIED.,.F.,.F.,(4,3,3,3,3,3,3,3,4),(-72.9640127846166,-72.8178712943224,
-71.8203662080988,-70.8228611218752,-69.8253560356517,-68.827850949428,
-67.8303458632045,-66.8328407769809,-66.680827477437),.UNSPECIFIED.);
#1579=B_SPLINE_CURVE_WITH_KNOTS('',3,(#75370,#75371,#75372,#75373,#75374,
#75375,#75376,#75377,#75378,#75379,#75380,#75381,#75382,#75383,#75384,#75385,
#75386,#75387,#75388,#75389,#75390,#75391),.UNSPECIFIED.,.F.,.F.,(4,3,3,
3,3,3,3,4),(64.1414162127729,64.8378306045337,65.8353356907573,66.8328407769809,
67.8303458632045,68.827850949428,69.8253560356517,70.4246015199525),
 .UNSPECIFIED.);
#1580=B_SPLINE_CURVE_WITH_KNOTS('',3,(#75392,#75393,#75394,#75395,#75396,
#75397,#75398,#75399,#75400,#75401,#75402,#75403,#75404,#75405,#75406,#75407,
#75408,#75409,#75410,#75411,#75412,#75413),.UNSPECIFIED.,.F.,.F.,(4,3,3,
3,3,3,3,4),(-66.680827477437,-65.8353356907573,-64.8378306045337,-63.8403255183101,
-62.8428204320865,-61.8453153458629,-60.8478102596393,-60.3976421702574),
 .UNSPECIFIED.);
#1581=B_SPLINE_CURVE_WITH_KNOTS('',3,(#75418,#75419,#75420,#75421,#75422,
#75423,#75424,#75425,#75426,#75427,#75428,#75429,#75430,#75431,#75432,#75433,
#75434,#75435,#75436,#75437,#75438,#75439),.UNSPECIFIED.,.F.,.F.,(4,3,3,
3,3,3,3,4),(57.8582309055933,58.8528000871921,59.8503051734157,60.8478102596393,
61.8453153458629,62.8428204320865,63.8403255183101,64.1414162127729),
 .UNSPECIFIED.);
#1582=B_SPLINE_CURVE_WITH_KNOTS('',3,(#75440,#75441,#75442,#75443,#75444,
#75445,#75446,#75447,#75448,#75449,#75450,#75451,#75452,#75453,#75454,#75455,
#75456,#75457,#75458,#75459,#75460,#75461),.UNSPECIFIED.,.F.,.F.,(4,3,3,
3,3,3,3,4),(-60.3976421702574,-59.8503051734157,-58.8528000871921,-57.8552950009685,
-56.8577899147449,-55.8602848285213,-54.8627797422977,-54.1144568630778),
 .UNSPECIFIED.);
#1583=B_SPLINE_CURVE_WITH_KNOTS('',3,(#75466,#75467,#75468,#75469,#75470,
#75471,#75472,#75473,#75474,#75475,#75476,#75477,#75478,#75479,#75480,#75481,
#75482,#75483,#75484,#75485,#75486,#75487,#75488,#75489,#75490),
 .UNSPECIFIED.,.F.,.F.,(4,3,3,3,3,3,3,3,4),(51.5750455984137,51.8702644836269,
52.8677695698506,53.8652746560741,54.8627797422977,55.8602848285213,56.8577899147449,
57.8552950009685,57.8582309055933),.UNSPECIFIED.);
#1584=B_SPLINE_CURVE_WITH_KNOTS('',3,(#75491,#75492,#75493,#75494,#75495,
#75496,#75497,#75498,#75499,#75500,#75501,#75502,#75503,#75504,#75505,#75506,
#75507,#75508,#75509,#75510,#75511,#75512,#75513,#75514,#75515),
 .UNSPECIFIED.,.F.,.F.,(4,3,3,3,3,3,3,3,4),(-54.1144568630778,-53.8652746560741,
-52.8677695698505,-51.8702644836269,-50.8727593974033,-49.8752543111797,
-48.8777492249561,-47.8802441387326,-47.8312715558983),.UNSPECIFIED.);
#1585=B_SPLINE_CURVE_WITH_KNOTS('',3,(#75520,#75521,#75522,#75523,#75524,
#75525,#75526,#75527,#75528,#75529,#75530,#75531,#75532,#75533,#75534,#75535,
#75536,#75537,#75538,#75539,#75540,#75541),.UNSPECIFIED.,.F.,.F.,(4,3,3,
3,3,3,3,4),(45.2918602912341,45.8852339662854,46.882739052509,47.8802441387326,
48.8777492249562,49.8752543111798,50.8727593974034,51.5750455984137),
 .UNSPECIFIED.);
#1586=B_SPLINE_CURVE_WITH_KNOTS('',3,(#75542,#75543,#75544,#75545,#75546,
#75547,#75548,#75549,#75550,#75551,#75552,#75553,#75554,#75555,#75556,#75557,
#75558,#75559,#75560,#75561,#75562,#75563),.UNSPECIFIED.,.F.,.F.,(4,3,3,
3,3,3,3,4),(-47.8312715558983,-46.882739052509,-45.8852339662854,-44.8877288800618,
-43.8902237938382,-42.8927187076146,-41.895213621391,-41.5480862487187),
 .UNSPECIFIED.);
#1587=B_SPLINE_CURVE_WITH_KNOTS('',3,(#75568,#75569,#75570,#75571,#75572,
#75573,#75574,#75575,#75576,#75577,#75578,#75579,#75580,#75581,#75582,#75583,
#75584,#75585,#75586,#75587,#75588,#75589),.UNSPECIFIED.,.F.,.F.,(4,3,3,
3,3,3,3,4),(39.0086749840545,39.9002034489438,40.8977085351674,41.895213621391,
42.8927187076146,43.8902237938382,44.8877288800618,45.2918602912341),
 .UNSPECIFIED.);
#1588=B_SPLINE_CURVE_WITH_KNOTS('',3,(#75590,#75591,#75592,#75593,#75594,
#75595,#75596,#75597,#75598,#75599,#75600,#75601,#75602,#75603,#75604,#75605,
#75606,#75607,#75608,#75609,#75610,#75611),.UNSPECIFIED.,.F.,.F.,(4,3,3,
3,3,3,3,4),(-41.5480862487187,-40.8977085351674,-39.9002034489438,-38.9026983627202,
-37.9051932764966,-36.907688190273,-35.9101831040494,-35.2649009415391),
 .UNSPECIFIED.);
#1589=B_SPLINE_CURVE_WITH_KNOTS('',3,(#75616,#75617,#75618,#75619,#75620,
#75621,#75622,#75623,#75624,#75625,#75626,#75627,#75628,#75629,#75630,#75631,
#75632,#75633,#75634,#75635,#75636,#75637,#75638,#75639,#75640),
 .UNSPECIFIED.,.F.,.F.,(4,3,3,3,3,3,3,3,4),(32.7254896768749,32.9176678453786,
33.9151729316022,34.9126780178258,35.9101831040494,36.907688190273,37.9051932764966,
38.9026983627202,39.0086749840545),.UNSPECIFIED.);
#1590=B_SPLINE_CURVE_WITH_KNOTS('',3,(#75641,#75642,#75643,#75644,#75645,
#75646,#75647,#75648,#75649,#75650,#75651,#75652,#75653,#75654,#75655,#75656,
#75657,#75658,#75659,#75660,#75661,#75662),.UNSPECIFIED.,.F.,.F.,(4,3,3,
3,3,3,3,4),(-35.2649009415391,-34.9126780178258,-33.9151729316022,-32.9176678453786,
-31.920162759155,-30.9226576729314,-29.9251525867078,-28.9817156343595),
 .UNSPECIFIED.);
#1591=B_SPLINE_CURVE_WITH_KNOTS('',3,(#75667,#75668,#75669,#75670,#75671,
#75672,#75673,#75674,#75675,#75676,#75677,#75678,#75679,#75680,#75681,#75682,
#75683,#75684,#75685,#75686,#75687,#75688),.UNSPECIFIED.,.F.,.F.,(4,3,3,
3,3,3,3,4),(26.4423043696953,26.9326373280371,27.9301424142607,28.9276475004843,
29.9251525867078,30.9226576729314,31.920162759155,32.7254896768749),
 .UNSPECIFIED.);
#1592=B_SPLINE_CURVE_WITH_KNOTS('',3,(#75689,#75690,#75691,#75692,#75693,
#75694,#75695,#75696,#75697,#75698,#75699,#75700,#75701,#75702,#75703,#75704,
#75705,#75706,#75707,#75708,#75709,#75710,#75711,#75712,#75713),
 .UNSPECIFIED.,.F.,.F.,(4,3,3,3,3,3,3,3,4),(-28.9817156343595,-28.9276475004843,
-27.9301424142607,-26.9326373280371,-25.9351322418135,-24.9376271555899,
-23.9401220693663,-22.9426169831427,-22.6985303271799),.UNSPECIFIED.);
#1593=B_SPLINE_CURVE_WITH_KNOTS('',3,(#75718,#75719,#75720,#75721,#75722,
#75723,#75724,#75725,#75726,#75727,#75728,#75729,#75730,#75731,#75732,#75733,
#75734,#75735,#75736,#75737,#75738,#75739),.UNSPECIFIED.,.F.,.F.,(4,3,3,
3,3,3,3,4),(20.1591190625158,20.9476068106955,21.9451118969191,22.9426169831427,
23.9401220693663,24.9376271555899,25.9351322418135,26.4423043696953),
 .UNSPECIFIED.);
#1594=B_SPLINE_CURVE_WITH_KNOTS('',3,(#75740,#75741,#75742,#75743,#75744,
#75745,#75746,#75747,#75748,#75749,#75750,#75751,#75752,#75753,#75754,#75755,
#75756,#75757,#75758,#75759,#75760,#75761),.UNSPECIFIED.,.F.,.F.,(4,3,3,
3,3,3,3,4),(-22.6985303271799,-21.9451118969191,-20.9476068106955,-19.9501017244719,
-18.9525966382483,-17.9550915520247,-16.9575864658011,-16.4153450200003),
 .UNSPECIFIED.);
#1595=B_SPLINE_CURVE_WITH_KNOTS('',3,(#75766,#75767,#75768,#75769,#75770,
#75771,#75772,#75773,#75774,#75775,#75776,#75777,#75778,#75779,#75780,#75781,
#75782,#75783,#75784,#75785,#75786,#75787,#75788,#75789,#75790),
 .UNSPECIFIED.,.F.,.F.,(4,3,3,3,3,3,3,3,4),(13.8759337553362,13.9650712071303,
14.9625762933539,15.9600813795775,16.9575864658011,17.9550915520247,18.9525966382483,
19.9501017244719,20.1591190625158),.UNSPECIFIED.);
#1596=B_SPLINE_CURVE_WITH_KNOTS('',3,(#75791,#75792,#75793,#75794,#75795,
#75796,#75797,#75798,#75799,#75800,#75801,#75802,#75803,#75804,#75805,#75806,
#75807,#75808,#75809,#75810,#75811,#75812),.UNSPECIFIED.,.F.,.F.,(4,3,3,
3,3,3,3,4),(-16.4153450200003,-15.9600813795775,-14.9625762933539,-13.9650712071303,
-12.9675661209067,-11.9700610346831,-10.9725559484596,-10.1321597128207),
 .UNSPECIFIED.);
#1597=B_SPLINE_CURVE_WITH_KNOTS('',3,(#75818,#75819,#75820,#75821,#75822,
#75823,#75824,#75825,#75826,#75827,#75828,#75829,#75830),.UNSPECIFIED.,
 .F.,.F.,(4,3,3,3,4),(-3.84897440564113,-2.99251525867078,-1.99501017244719,
-0.997505086223595,0.),.UNSPECIFIED.);
#1598=B_SPLINE_CURVE_WITH_KNOTS('',3,(#75833,#75834,#75835,#75836,#75837,
#75838,#75839,#75840,#75841,#75842,#75843,#75844,#75845,#75846,#75847,#75848,
#75849,#75850,#75851),.UNSPECIFIED.,.F.,.F.,(4,3,3,3,3,3,4),(2.01694489302847,
2.99251525867078,3.99002034489437,4.98752543111797,5.98503051734157,6.98253560356516,
7.59274844815659),.UNSPECIFIED.);
#1599=B_SPLINE_CURVE_WITH_KNOTS('',3,(#75857,#75858,#75859,#75860),
 .UNSPECIFIED.,.F.,.F.,(4,4),(126.973269284569,127.68065103662),
 .UNSPECIFIED.);
#1600=B_SPLINE_CURVE_WITH_KNOTS('',3,(#75863,#75864,#75865,#75866,#75867,
#75868,#75869,#75870,#75871,#75872),.UNSPECIFIED.,.F.,.F.,(4,3,3,4),(-125.663706143592,
-124.688135777949,-123.690630691726,-123.229495242053),.UNSPECIFIED.);
#1601=B_SPLINE_CURVE_WITH_KNOTS('',3,(#75877,#75878,#75879,#75880,#75881,
#75882,#75883,#75884,#75885,#75886,#75887,#75888,#75889,#75890,#75891,#75892,
#75893,#75894,#75895,#75896,#75897,#75898,#75899,#75900,#75901),
 .UNSPECIFIED.,.F.,.F.,(4,3,3,3,3,3,3,3,4),(120.690083977389,120.698115433055,
121.695620519279,122.693125605502,123.690630691726,124.688135777949,125.685640864173,
126.683145950397,126.973269284569),.UNSPECIFIED.);
#1602=B_SPLINE_CURVE_WITH_KNOTS('',3,(#75902,#75903,#75904,#75905,#75906,
#75907,#75908,#75909,#75910,#75911,#75912,#75913,#75914,#75915,#75916,#75917,
#75918,#75919,#75920,#75921,#75922,#75923),.UNSPECIFIED.,.F.,.F.,(4,3,3,
3,3,3,3,4),(-123.229495242053,-122.693125605502,-121.695620519279,-120.698115433055,
-119.700610346831,-118.703105260608,-117.705600174384,-116.946309934874),
 .UNSPECIFIED.);
#1603=B_SPLINE_CURVE_WITH_KNOTS('',3,(#75928,#75929,#75930,#75931,#75932,
#75933,#75934,#75935,#75936,#75937,#75938,#75939,#75940,#75941,#75942,#75943,
#75944,#75945,#75946,#75947,#75948,#75949),.UNSPECIFIED.,.F.,.F.,(4,3,3,
3,3,3,3,4),(114.40689867021,114.713084915713,115.710590001937,116.708095088161,
117.705600174384,118.703105260608,119.700610346831,120.690083977389),
 .UNSPECIFIED.);
#1604=B_SPLINE_CURVE_WITH_KNOTS('',3,(#75950,#75951,#75952,#75953,#75954,
#75955,#75956,#75957,#75958,#75959,#75960,#75961,#75962,#75963,#75964,#75965,
#75966,#75967,#75968,#75969,#75970,#75971,#75972,#75973,#75974),
 .UNSPECIFIED.,.F.,.F.,(4,3,3,3,3,3,3,3,4),(-116.946309934874,-116.708095088161,
-115.710590001937,-114.713084915713,-113.71557982949,-112.718074743266,
-111.720569657043,-110.723064570819,-110.663124627694),.UNSPECIFIED.);
#1605=B_SPLINE_CURVE_WITH_KNOTS('',3,(#75979,#75980,#75981,#75982,#75983,
#75984,#75985,#75986,#75987,#75988,#75989,#75990,#75991,#75992,#75993,#75994,
#75995,#75996,#75997,#75998,#75999,#76000),.UNSPECIFIED.,.F.,.F.,(4,3,3,
3,3,3,3,4),(108.12371336303,108.728054398372,109.725559484595,110.723064570819,
111.720569657043,112.718074743266,113.71557982949,114.40689867021),
 .UNSPECIFIED.);
#1606=B_SPLINE_CURVE_WITH_KNOTS('',3,(#76001,#76002,#76003,#76004,#76005,
#76006,#76007,#76008,#76009,#76010,#76011,#76012,#76013,#76014,#76015,#76016,
#76017,#76018,#76019,#76020,#76021,#76022),.UNSPECIFIED.,.F.,.F.,(4,3,3,
3,3,3,3,4),(-110.663124627694,-109.725559484596,-108.728054398372,-107.730549312148,
-106.733044225925,-105.735539139701,-104.738034053478,-104.379939320515),
 .UNSPECIFIED.);
#1607=B_SPLINE_CURVE_WITH_KNOTS('',3,(#76027,#76028,#76029,#76030,#76031,
#76032,#76033,#76034,#76035,#76036,#76037,#76038,#76039,#76040,#76041,#76042,
#76043,#76044,#76045,#76046,#76047,#76048),.UNSPECIFIED.,.F.,.F.,(4,3,3,
3,3,3,3,4),(101.84052805585,102.74302388103,103.740528967254,104.738034053478,
105.735539139701,106.733044225925,107.730549312148,108.12371336303),
 .UNSPECIFIED.);
#1608=B_SPLINE_CURVE_WITH_KNOTS('',3,(#76049,#76050,#76051,#76052,#76053,
#76054,#76055,#76056,#76057,#76058,#76059,#76060,#76061,#76062,#76063,#76064,
#76065,#76066,#76067,#76068,#76069,#76070),.UNSPECIFIED.,.F.,.F.,(4,3,3,
3,3,3,3,4),(-104.379939320515,-103.740528967254,-102.74302388103,-101.745518794807,
-100.748013708583,-99.7505086223595,-98.7530035361359,-98.096754013335),
 .UNSPECIFIED.);
#1609=B_SPLINE_CURVE_WITH_KNOTS('',3,(#76075,#76076,#76077,#76078,#76079,
#76080,#76081,#76082,#76083,#76084,#76085,#76086,#76087,#76088,#76089,#76090,
#76091,#76092,#76093,#76094,#76095,#76096,#76097,#76098,#76099),
 .UNSPECIFIED.,.F.,.F.,(4,3,3,3,3,3,3,3,4),(95.5573427486709,95.7604882774652,
96.7579933636887,97.7554984499123,98.7530035361359,99.7505086223595,100.748013708583,
101.745518794807,101.84052805585),.UNSPECIFIED.);
#1610=B_SPLINE_CURVE_WITH_KNOTS('',3,(#76100,#76101,#76102,#76103,#76104,
#76105,#76106,#76107,#76108,#76109,#76110,#76111,#76112,#76113,#76114,#76115,
#76116,#76117,#76118,#76119,#76120,#76121),.UNSPECIFIED.,.F.,.F.,(4,3,3,
3,3,3,3,4),(-98.096754013335,-97.7554984499123,-96.7579933636887,-95.7604882774651,
-94.7629831912416,-93.7654781050179,-92.7679730187944,-91.8135687061554),
 .UNSPECIFIED.);
#1611=B_SPLINE_CURVE_WITH_KNOTS('',3,(#76126,#76127,#76128,#76129,#76130,
#76131,#76132,#76133,#76134,#76135,#76136,#76137,#76138,#76139,#76140,#76141,
#76142,#76143,#76144,#76145,#76146,#76147),.UNSPECIFIED.,.F.,.F.,(4,3,3,
3,3,3,3,4),(89.2741574414913,89.7754577601236,90.7729628463472,91.7704679325708,
92.7679730187944,93.765478105018,94.7629831912415,95.5573427486709),
 .UNSPECIFIED.);
#1612=B_SPLINE_CURVE_WITH_KNOTS('',3,(#76148,#76149,#76150,#76151,#76152,
#76153,#76154,#76155,#76156,#76157,#76158,#76159,#76160,#76161,#76162,#76163,
#76164,#76165,#76166,#76167,#76168,#76169,#76170,#76171,#76172),
 .UNSPECIFIED.,.F.,.F.,(4,3,3,3,3,3,3,3,4),(-91.8135687061554,-91.7704679325708,
-90.7729628463472,-89.7754577601236,-88.7779526739,-87.7804475876764,-86.7829425014528,
-85.7854374152292,-85.5303833989758),.UNSPECIFIED.);
#1613=B_SPLINE_CURVE_WITH_KNOTS('',3,(#76177,#76178,#76179,#76180,#76181,
#76182,#76183,#76184,#76185,#76186,#76187,#76188,#76189,#76190,#76191,#76192,
#76193,#76194,#76195,#76196,#76197,#76198),.UNSPECIFIED.,.F.,.F.,(4,3,3,
3,3,3,3,4),(82.9909721343117,83.790427242782,84.7879323290056,85.7854374152292,
86.7829425014528,87.7804475876764,88.7779526739,89.2741574414913),
 .UNSPECIFIED.);
#1614=B_SPLINE_CURVE_WITH_KNOTS('',3,(#76199,#76200,#76201,#76202,#76203,
#76204,#76205,#76206,#76207,#76208,#76209,#76210,#76211,#76212,#76213,#76214,
#76215,#76216,#76217,#76218,#76219,#76220),.UNSPECIFIED.,.F.,.F.,(4,3,3,
3,3,3,3,4),(-85.5303833989758,-84.7879323290056,-83.790427242782,-82.7929221565584,
-81.7954170703348,-80.7979119841112,-79.8004068978876,-79.2471980917962),
 .UNSPECIFIED.);
#1615=B_SPLINE_CURVE_WITH_KNOTS('',3,(#76225,#76226,#76227,#76228,#76229,
#76230,#76231,#76232,#76233,#76234,#76235,#76236,#76237,#76238,#76239,#76240,
#76241,#76242,#76243,#76244,#76245,#76246,#76247,#76248,#76249),
 .UNSPECIFIED.,.F.,.F.,(4,3,3,3,3,3,3,3,4),(76.7077868271321,76.8078916392168,
77.8053967254404,78.802901811664,79.8004068978876,80.7979119841112,81.7954170703348,
82.7929221565584,82.9909721343117),.UNSPECIFIED.);
#1616=B_SPLINE_CURVE_WITH_KNOTS('',3,(#76250,#76251,#76252,#76253,#76254,
#76255,#76256,#76257,#76258,#76259,#76260,#76261,#76262,#76263,#76264,#76265,
#76266,#76267,#76268,#76269,#76270,#76271),.UNSPECIFIED.,.F.,.F.,(4,3,3,
3,3,3,3,4),(-79.2471980917962,-78.802901811664,-77.8053967254404,-76.8078916392168,
-75.8103865529932,-74.8128814667696,-73.815376380546,-72.9640127846166),
 .UNSPECIFIED.);
#1617=B_SPLINE_CURVE_WITH_KNOTS('',3,(#76276,#76277,#76278,#76279,#76280,
#76281,#76282,#76283,#76284,#76285,#76286,#76287,#76288,#76289,#76290,#76291,
#76292,#76293,#76294,#76295,#76296,#76297),.UNSPECIFIED.,.F.,.F.,(4,3,3,
3,3,3,3,4),(70.4246015199525,70.8228611218753,71.8203662080989,72.8178712943224,
73.815376380546,74.8128814667696,75.8103865529932,76.7077868271321),
 .UNSPECIFIED.);
#1618=B_SPLINE_CURVE_WITH_KNOTS('',3,(#76298,#76299,#76300,#76301,#76302,
#76303,#76304,#76305,#76306,#76307,#76308,#76309,#76310,#76311,#76312,#76313,
#76314,#76315,#76316,#76317,#76318,#76319,#76320,#76321,#76322),
 .UNSPECIFIED.,.F.,.F.,(4,3,3,3,3,3,3,3,4),(-72.9640127846166,-72.8178712943224,
-71.8203662080988,-70.8228611218752,-69.8253560356517,-68.8278509494281,
-67.8303458632045,-66.8328407769809,-66.680827477437),.UNSPECIFIED.);
#1619=B_SPLINE_CURVE_WITH_KNOTS('',3,(#76327,#76328,#76329,#76330,#76331,
#76332,#76333,#76334,#76335,#76336,#76337,#76338,#76339,#76340,#76341,#76342,
#76343,#76344,#76345,#76346,#76347,#76348),.UNSPECIFIED.,.F.,.F.,(4,3,3,
3,3,3,3,4),(64.1414162127729,64.8378306045337,65.8353356907573,66.8328407769809,
67.8303458632045,68.8278509494281,69.8253560356517,70.4246015199525),
 .UNSPECIFIED.);
#1620=B_SPLINE_CURVE_WITH_KNOTS('',3,(#76349,#76350,#76351,#76352,#76353,
#76354,#76355,#76356,#76357,#76358,#76359,#76360,#76361,#76362,#76363,#76364,
#76365,#76366,#76367,#76368,#76369,#76370),.UNSPECIFIED.,.F.,.F.,(4,3,3,
3,3,3,3,4),(-66.680827477437,-65.8353356907573,-64.8378306045337,-63.8403255183101,
-62.8428204320865,-61.8453153458629,-60.8478102596393,-60.3976421702575),
 .UNSPECIFIED.);
#1621=B_SPLINE_CURVE_WITH_KNOTS('',3,(#76375,#76376,#76377,#76378,#76379,
#76380,#76381,#76382,#76383,#76384,#76385,#76386,#76387,#76388,#76389,#76390,
#76391,#76392,#76393,#76394,#76395,#76396),.UNSPECIFIED.,.F.,.F.,(4,3,3,
3,3,3,3,4),(57.8582309055933,58.8528000871921,59.8503051734157,60.8478102596393,
61.8453153458629,62.8428204320865,63.8403255183101,64.1414162127729),
 .UNSPECIFIED.);
#1622=B_SPLINE_CURVE_WITH_KNOTS('',3,(#76397,#76398,#76399,#76400,#76401,
#76402,#76403,#76404,#76405,#76406,#76407,#76408,#76409,#76410,#76411,#76412,
#76413,#76414,#76415,#76416,#76417,#76418),.UNSPECIFIED.,.F.,.F.,(4,3,3,
3,3,3,3,4),(-60.3976421702575,-59.8503051734157,-58.8528000871921,-57.8552950009685,
-56.8577899147449,-55.8602848285213,-54.8627797422977,-54.1144568630778),
 .UNSPECIFIED.);
#1623=B_SPLINE_CURVE_WITH_KNOTS('',3,(#76423,#76424,#76425,#76426,#76427,
#76428,#76429,#76430,#76431,#76432,#76433,#76434,#76435,#76436,#76437,#76438,
#76439,#76440,#76441,#76442,#76443,#76444,#76445,#76446,#76447),
 .UNSPECIFIED.,.F.,.F.,(4,3,3,3,3,3,3,3,4),(51.5750455984137,51.870264483627,
52.8677695698506,53.8652746560741,54.8627797422977,55.8602848285213,56.8577899147449,
57.8552950009685,57.8582309055933),.UNSPECIFIED.);
#1624=B_SPLINE_CURVE_WITH_KNOTS('',3,(#76448,#76449,#76450,#76451,#76452,
#76453,#76454,#76455,#76456,#76457,#76458,#76459,#76460,#76461,#76462,#76463,
#76464,#76465,#76466,#76467,#76468,#76469,#76470,#76471,#76472),
 .UNSPECIFIED.,.F.,.F.,(4,3,3,3,3,3,3,3,4),(-54.1144568630778,-53.8652746560741,
-52.8677695698505,-51.870264483627,-50.8727593974034,-49.8752543111798,
-48.8777492249562,-47.8802441387326,-47.8312715558983),.UNSPECIFIED.);
#1625=B_SPLINE_CURVE_WITH_KNOTS('',3,(#76477,#76478,#76479,#76480,#76481,
#76482,#76483,#76484,#76485,#76486,#76487,#76488,#76489,#76490,#76491,#76492,
#76493,#76494,#76495,#76496,#76497,#76498),.UNSPECIFIED.,.F.,.F.,(4,3,3,
3,3,3,3,4),(45.2918602912341,45.8852339662854,46.882739052509,47.8802441387326,
48.8777492249562,49.8752543111798,50.8727593974034,51.5750455984137),
 .UNSPECIFIED.);
#1626=B_SPLINE_CURVE_WITH_KNOTS('',3,(#76499,#76500,#76501,#76502,#76503,
#76504,#76505,#76506,#76507,#76508,#76509,#76510,#76511,#76512,#76513,#76514,
#76515,#76516,#76517,#76518,#76519,#76520),.UNSPECIFIED.,.F.,.F.,(4,3,3,
3,3,3,3,4),(-47.8312715558983,-46.882739052509,-45.8852339662854,-44.8877288800618,
-43.8902237938382,-42.8927187076146,-41.895213621391,-41.5480862487187),
 .UNSPECIFIED.);
#1627=B_SPLINE_CURVE_WITH_KNOTS('',3,(#76525,#76526,#76527,#76528,#76529,
#76530,#76531,#76532,#76533,#76534,#76535,#76536,#76537,#76538,#76539,#76540,
#76541,#76542,#76543,#76544,#76545,#76546),.UNSPECIFIED.,.F.,.F.,(4,3,3,
3,3,3,3,4),(39.0086749840545,39.9002034489438,40.8977085351674,41.895213621391,
42.8927187076146,43.8902237938382,44.8877288800618,45.2918602912341),
 .UNSPECIFIED.);
#1628=B_SPLINE_CURVE_WITH_KNOTS('',3,(#76547,#76548,#76549,#76550,#76551,
#76552,#76553,#76554,#76555,#76556,#76557,#76558,#76559,#76560,#76561,#76562,
#76563,#76564,#76565,#76566,#76567,#76568),.UNSPECIFIED.,.F.,.F.,(4,3,3,
3,3,3,3,4),(-41.5480862487187,-40.8977085351674,-39.9002034489438,-38.9026983627202,
-37.9051932764966,-36.907688190273,-35.9101831040494,-35.2649009415391),
 .UNSPECIFIED.);
#1629=B_SPLINE_CURVE_WITH_KNOTS('',3,(#76573,#76574,#76575,#76576,#76577,
#76578,#76579,#76580,#76581,#76582,#76583,#76584,#76585,#76586,#76587,#76588,
#76589,#76590,#76591,#76592,#76593,#76594,#76595,#76596,#76597),
 .UNSPECIFIED.,.F.,.F.,(4,3,3,3,3,3,3,3,4),(32.725489676875,32.9176678453786,
33.9151729316022,34.9126780178258,35.9101831040494,36.907688190273,37.9051932764966,
38.9026983627202,39.0086749840545),.UNSPECIFIED.);
#1630=B_SPLINE_CURVE_WITH_KNOTS('',3,(#76598,#76599,#76600,#76601,#76602,
#76603,#76604,#76605,#76606,#76607,#76608,#76609,#76610,#76611,#76612,#76613,
#76614,#76615,#76616,#76617,#76618,#76619),.UNSPECIFIED.,.F.,.F.,(4,3,3,
3,3,3,3,4),(-35.2649009415391,-34.9126780178258,-33.9151729316022,-32.9176678453786,
-31.920162759155,-30.9226576729315,-29.9251525867079,-28.9817156343595),
 .UNSPECIFIED.);
#1631=B_SPLINE_CURVE_WITH_KNOTS('',3,(#76624,#76625,#76626,#76627,#76628,
#76629,#76630,#76631,#76632,#76633,#76634,#76635,#76636,#76637,#76638,#76639,
#76640,#76641,#76642,#76643,#76644,#76645),.UNSPECIFIED.,.F.,.F.,(4,3,3,
3,3,3,3,4),(26.4423043696954,26.9326373280371,27.9301424142607,28.9276475004843,
29.9251525867079,30.9226576729315,31.920162759155,32.725489676875),
 .UNSPECIFIED.);
#1632=B_SPLINE_CURVE_WITH_KNOTS('',3,(#76646,#76647,#76648,#76649,#76650,
#76651,#76652,#76653,#76654,#76655,#76656,#76657,#76658,#76659,#76660,#76661,
#76662,#76663,#76664,#76665,#76666,#76667,#76668,#76669,#76670),
 .UNSPECIFIED.,.F.,.F.,(4,3,3,3,3,3,3,3,4),(-28.9817156343595,-28.9276475004843,
-27.9301424142607,-26.9326373280371,-25.9351322418135,-24.9376271555899,
-23.9401220693663,-22.9426169831427,-22.6985303271799),.UNSPECIFIED.);
#1633=B_SPLINE_CURVE_WITH_KNOTS('',3,(#76675,#76676,#76677,#76678,#76679,
#76680,#76681,#76682,#76683,#76684,#76685,#76686,#76687,#76688,#76689,#76690,
#76691,#76692,#76693,#76694,#76695,#76696),.UNSPECIFIED.,.F.,.F.,(4,3,3,
3,3,3,3,4),(20.1591190625158,20.9476068106955,21.9451118969191,22.9426169831427,
23.9401220693663,24.9376271555899,25.9351322418135,26.4423043696954),
 .UNSPECIFIED.);
#1634=B_SPLINE_CURVE_WITH_KNOTS('',3,(#76697,#76698,#76699,#76700,#76701,
#76702,#76703,#76704,#76705,#76706,#76707,#76708,#76709,#76710,#76711,#76712,
#76713,#76714,#76715,#76716,#76717,#76718),.UNSPECIFIED.,.F.,.F.,(4,3,3,
3,3,3,3,4),(-22.6985303271799,-21.9451118969191,-20.9476068106955,-19.9501017244719,
-18.9525966382483,-17.9550915520247,-16.9575864658011,-16.4153450200003),
 .UNSPECIFIED.);
#1635=B_SPLINE_CURVE_WITH_KNOTS('',3,(#76723,#76724,#76725,#76726,#76727,
#76728,#76729,#76730,#76731,#76732,#76733,#76734,#76735,#76736,#76737,#76738,
#76739,#76740,#76741,#76742,#76743,#76744,#76745,#76746,#76747),
 .UNSPECIFIED.,.F.,.F.,(4,3,3,3,3,3,3,3,4),(13.8759337553362,13.9650712071303,
14.9625762933539,15.9600813795775,16.9575864658011,17.9550915520247,18.9525966382483,
19.9501017244719,20.1591190625158),.UNSPECIFIED.);
#1636=B_SPLINE_CURVE_WITH_KNOTS('',3,(#76748,#76749,#76750,#76751,#76752,
#76753,#76754,#76755,#76756,#76757,#76758,#76759,#76760,#76761,#76762,#76763,
#76764,#76765,#76766,#76767,#76768,#76769),.UNSPECIFIED.,.F.,.F.,(4,3,3,
3,3,3,3,4),(-16.4153450200003,-15.9600813795775,-14.9625762933539,-13.9650712071303,
-12.9675661209067,-11.9700610346831,-10.9725559484596,-10.1321597128207),
 .UNSPECIFIED.);
#1637=B_SPLINE_CURVE_WITH_KNOTS('',3,(#76775,#76776,#76777,#76778,#76779,
#76780,#76781,#76782,#76783,#76784,#76785,#76786,#76787),.UNSPECIFIED.,
 .F.,.F.,(4,3,3,3,4),(-3.84897440564114,-2.99251525867078,-1.99501017244719,
-0.997505086223593,0.),.UNSPECIFIED.);
#1638=B_SPLINE_CURVE_WITH_KNOTS('',3,(#76790,#76791,#76792,#76793,#76794,
#76795,#76796,#76797,#76798,#76799,#76800,#76801,#76802,#76803,#76804,#76805,
#76806,#76807,#76808),.UNSPECIFIED.,.F.,.F.,(4,3,3,3,3,3,4),(2.01694489302824,
2.99251525867079,3.99002034489439,4.98752543111799,5.98503051734158,6.98253560356518,
7.5927484481566),.UNSPECIFIED.);
#1639=B_SPLINE_CURVE_WITH_KNOTS('',3,(#76814,#76815,#76816,#76817),
 .UNSPECIFIED.,.F.,.F.,(4,4),(126.973269284569,127.68065103662),
 .UNSPECIFIED.);
#1640=B_SPLINE_CURVE_WITH_KNOTS('',3,(#76820,#76821,#76822,#76823,#76824,
#76825,#76826,#76827,#76828,#76829),.UNSPECIFIED.,.F.,.F.,(4,3,3,4),(-125.663706143592,
-124.688135777949,-123.690630691726,-123.229495242053),.UNSPECIFIED.);
#1641=B_SPLINE_CURVE_WITH_KNOTS('',3,(#76834,#76835,#76836,#76837,#76838,
#76839,#76840,#76841,#76842,#76843,#76844,#76845,#76846,#76847,#76848,#76849,
#76850,#76851,#76852,#76853,#76854,#76855,#76856,#76857,#76858),
 .UNSPECIFIED.,.F.,.F.,(4,3,3,3,3,3,3,3,4),(120.690083977389,120.698115433055,
121.695620519279,122.693125605502,123.690630691726,124.688135777949,125.685640864173,
126.683145950397,126.973269284569),.UNSPECIFIED.);
#1642=B_SPLINE_CURVE_WITH_KNOTS('',3,(#76859,#76860,#76861,#76862,#76863,
#76864,#76865,#76866,#76867,#76868,#76869,#76870,#76871,#76872,#76873,#76874,
#76875,#76876,#76877,#76878,#76879,#76880),.UNSPECIFIED.,.F.,.F.,(4,3,3,
3,3,3,3,4),(-123.229495242053,-122.693125605502,-121.695620519279,-120.698115433055,
-119.700610346831,-118.703105260608,-117.705600174384,-116.946309934874),
 .UNSPECIFIED.);
#1643=B_SPLINE_CURVE_WITH_KNOTS('',3,(#76885,#76886,#76887,#76888,#76889,
#76890,#76891,#76892,#76893,#76894,#76895,#76896,#76897,#76898,#76899,#76900,
#76901,#76902,#76903,#76904,#76905,#76906),.UNSPECIFIED.,.F.,.F.,(4,3,3,
3,3,3,3,4),(114.40689867021,114.713084915713,115.710590001937,116.708095088161,
117.705600174384,118.703105260608,119.700610346831,120.690083977389),
 .UNSPECIFIED.);
#1644=B_SPLINE_CURVE_WITH_KNOTS('',3,(#76907,#76908,#76909,#76910,#76911,
#76912,#76913,#76914,#76915,#76916,#76917,#76918,#76919,#76920,#76921,#76922,
#76923,#76924,#76925,#76926,#76927,#76928,#76929,#76930,#76931),
 .UNSPECIFIED.,.F.,.F.,(4,3,3,3,3,3,3,3,4),(-116.946309934874,-116.708095088161,
-115.710590001937,-114.713084915713,-113.71557982949,-112.718074743266,
-111.720569657043,-110.723064570819,-110.663124627694),.UNSPECIFIED.);
#1645=B_SPLINE_CURVE_WITH_KNOTS('',3,(#76936,#76937,#76938,#76939,#76940,
#76941,#76942,#76943,#76944,#76945,#76946,#76947,#76948,#76949,#76950,#76951,
#76952,#76953,#76954,#76955,#76956,#76957),.UNSPECIFIED.,.F.,.F.,(4,3,3,
3,3,3,3,4),(108.12371336303,108.728054398372,109.725559484595,110.723064570819,
111.720569657043,112.718074743266,113.71557982949,114.40689867021),
 .UNSPECIFIED.);
#1646=B_SPLINE_CURVE_WITH_KNOTS('',3,(#76958,#76959,#76960,#76961,#76962,
#76963,#76964,#76965,#76966,#76967,#76968,#76969,#76970,#76971,#76972,#76973,
#76974,#76975,#76976,#76977,#76978,#76979),.UNSPECIFIED.,.F.,.F.,(4,3,3,
3,3,3,3,4),(-110.663124627694,-109.725559484595,-108.728054398372,-107.730549312148,
-106.733044225925,-105.735539139701,-104.738034053477,-104.379939320515),
 .UNSPECIFIED.);
#1647=B_SPLINE_CURVE_WITH_KNOTS('',3,(#76984,#76985,#76986,#76987,#76988,
#76989,#76990,#76991,#76992,#76993,#76994,#76995,#76996,#76997,#76998,#76999,
#77000,#77001,#77002,#77003,#77004,#77005),.UNSPECIFIED.,.F.,.F.,(4,3,3,
3,3,3,3,4),(101.84052805585,102.74302388103,103.740528967254,104.738034053478,
105.735539139701,106.733044225925,107.730549312148,108.12371336303),
 .UNSPECIFIED.);
#1648=B_SPLINE_CURVE_WITH_KNOTS('',3,(#77006,#77007,#77008,#77009,#77010,
#77011,#77012,#77013,#77014,#77015,#77016,#77017,#77018,#77019,#77020,#77021,
#77022,#77023,#77024,#77025,#77026,#77027),.UNSPECIFIED.,.F.,.F.,(4,3,3,
3,3,3,3,4),(-104.379939320515,-103.740528967254,-102.74302388103,-101.745518794807,
-100.748013708583,-99.7505086223595,-98.7530035361359,-98.096754013335),
 .UNSPECIFIED.);
#1649=B_SPLINE_CURVE_WITH_KNOTS('',3,(#77032,#77033,#77034,#77035,#77036,
#77037,#77038,#77039,#77040,#77041,#77042,#77043,#77044,#77045,#77046,#77047,
#77048,#77049,#77050,#77051,#77052,#77053,#77054,#77055,#77056),
 .UNSPECIFIED.,.F.,.F.,(4,3,3,3,3,3,3,3,4),(95.5573427486709,95.7604882774652,
96.7579933636888,97.7554984499123,98.7530035361359,99.7505086223595,100.748013708583,
101.745518794807,101.84052805585),.UNSPECIFIED.);
#1650=B_SPLINE_CURVE_WITH_KNOTS('',3,(#77057,#77058,#77059,#77060,#77061,
#77062,#77063,#77064,#77065,#77066,#77067,#77068,#77069,#77070,#77071,#77072,
#77073,#77074,#77075,#77076,#77077,#77078),.UNSPECIFIED.,.F.,.F.,(4,3,3,
3,3,3,3,4),(-98.096754013335,-97.7554984499123,-96.7579933636887,-95.7604882774651,
-94.7629831912415,-93.7654781050179,-92.7679730187943,-91.8135687061554),
 .UNSPECIFIED.);
#1651=B_SPLINE_CURVE_WITH_KNOTS('',3,(#77083,#77084,#77085,#77086,#77087,
#77088,#77089,#77090,#77091,#77092,#77093,#77094,#77095,#77096,#77097,#77098,
#77099,#77100,#77101,#77102,#77103,#77104),.UNSPECIFIED.,.F.,.F.,(4,3,3,
3,3,3,3,4),(89.2741574414913,89.7754577601236,90.7729628463472,91.7704679325708,
92.7679730187944,93.765478105018,94.7629831912416,95.5573427486709),
 .UNSPECIFIED.);
#1652=B_SPLINE_CURVE_WITH_KNOTS('',3,(#77105,#77106,#77107,#77108,#77109,
#77110,#77111,#77112,#77113,#77114,#77115,#77116,#77117,#77118,#77119,#77120,
#77121,#77122,#77123,#77124,#77125,#77126,#77127,#77128,#77129),
 .UNSPECIFIED.,.F.,.F.,(4,3,3,3,3,3,3,3,4),(-91.8135687061554,-91.7704679325707,
-90.7729628463472,-89.7754577601236,-88.7779526739,-87.7804475876764,-86.7829425014528,
-85.7854374152292,-85.5303833989758),.UNSPECIFIED.);
#1653=B_SPLINE_CURVE_WITH_KNOTS('',3,(#77134,#77135,#77136,#77137,#77138,
#77139,#77140,#77141,#77142,#77143,#77144,#77145,#77146,#77147,#77148,#77149,
#77150,#77151,#77152,#77153,#77154,#77155),.UNSPECIFIED.,.F.,.F.,(4,3,3,
3,3,3,3,4),(82.9909721343117,83.790427242782,84.7879323290056,85.7854374152292,
86.7829425014528,87.7804475876764,88.7779526739,89.2741574414913),
 .UNSPECIFIED.);
#1654=B_SPLINE_CURVE_WITH_KNOTS('',3,(#77156,#77157,#77158,#77159,#77160,
#77161,#77162,#77163,#77164,#77165,#77166,#77167,#77168,#77169,#77170,#77171,
#77172,#77173,#77174,#77175,#77176,#77177),.UNSPECIFIED.,.F.,.F.,(4,3,3,
3,3,3,3,4),(-85.5303833989758,-84.7879323290056,-83.790427242782,-82.7929221565584,
-81.7954170703348,-80.7979119841112,-79.8004068978876,-79.2471980917962),
 .UNSPECIFIED.);
#1655=B_SPLINE_CURVE_WITH_KNOTS('',3,(#77182,#77183,#77184,#77185,#77186,
#77187,#77188,#77189,#77190,#77191,#77192,#77193,#77194,#77195,#77196,#77197,
#77198,#77199,#77200,#77201,#77202,#77203,#77204,#77205,#77206),
 .UNSPECIFIED.,.F.,.F.,(4,3,3,3,3,3,3,3,4),(76.7077868271321,76.8078916392168,
77.8053967254404,78.802901811664,79.8004068978876,80.7979119841112,81.7954170703348,
82.7929221565584,82.9909721343117),.UNSPECIFIED.);
#1656=B_SPLINE_CURVE_WITH_KNOTS('',3,(#77207,#77208,#77209,#77210,#77211,
#77212,#77213,#77214,#77215,#77216,#77217,#77218,#77219,#77220,#77221,#77222,
#77223,#77224,#77225,#77226,#77227,#77228),.UNSPECIFIED.,.F.,.F.,(4,3,3,
3,3,3,3,4),(-79.2471980917962,-78.802901811664,-77.8053967254404,-76.8078916392168,
-75.8103865529932,-74.8128814667696,-73.815376380546,-72.9640127846166),
 .UNSPECIFIED.);
#1657=B_SPLINE_CURVE_WITH_KNOTS('',3,(#77233,#77234,#77235,#77236,#77237,
#77238,#77239,#77240,#77241,#77242,#77243,#77244,#77245,#77246,#77247,#77248,
#77249,#77250,#77251,#77252,#77253,#77254),.UNSPECIFIED.,.F.,.F.,(4,3,3,
3,3,3,3,4),(70.4246015199525,70.8228611218753,71.8203662080989,72.8178712943225,
73.8153763805461,74.8128814667697,75.8103865529933,76.7077868271321),
 .UNSPECIFIED.);
#1658=B_SPLINE_CURVE_WITH_KNOTS('',3,(#77255,#77256,#77257,#77258,#77259,
#77260,#77261,#77262,#77263,#77264,#77265,#77266,#77267,#77268,#77269,#77270,
#77271,#77272,#77273,#77274,#77275,#77276,#77277,#77278,#77279),
 .UNSPECIFIED.,.F.,.F.,(4,3,3,3,3,3,3,3,4),(-72.9640127846166,-72.8178712943224,
-71.8203662080988,-70.8228611218753,-69.8253560356517,-68.8278509494281,
-67.8303458632045,-66.8328407769809,-66.680827477437),.UNSPECIFIED.);
#1659=B_SPLINE_CURVE_WITH_KNOTS('',3,(#77284,#77285,#77286,#77287,#77288,
#77289,#77290,#77291,#77292,#77293,#77294,#77295,#77296,#77297,#77298,#77299,
#77300,#77301,#77302,#77303,#77304,#77305),.UNSPECIFIED.,.F.,.F.,(4,3,3,
3,3,3,3,4),(64.1414162127729,64.8378306045337,65.8353356907573,66.8328407769809,
67.8303458632045,68.8278509494281,69.8253560356517,70.4246015199525),
 .UNSPECIFIED.);
#1660=B_SPLINE_CURVE_WITH_KNOTS('',3,(#77306,#77307,#77308,#77309,#77310,
#77311,#77312,#77313,#77314,#77315,#77316,#77317,#77318,#77319,#77320,#77321,
#77322,#77323,#77324,#77325,#77326,#77327),.UNSPECIFIED.,.F.,.F.,(4,3,3,
3,3,3,3,4),(-66.680827477437,-65.8353356907573,-64.8378306045337,-63.8403255183101,
-62.8428204320865,-61.8453153458629,-60.8478102596393,-60.3976421702575),
 .UNSPECIFIED.);
#1661=B_SPLINE_CURVE_WITH_KNOTS('',3,(#77332,#77333,#77334,#77335,#77336,
#77337,#77338,#77339,#77340,#77341,#77342,#77343,#77344,#77345,#77346,#77347,
#77348,#77349,#77350,#77351,#77352,#77353),.UNSPECIFIED.,.F.,.F.,(4,3,3,
3,3,3,3,4),(57.8582309055933,58.8528000871921,59.8503051734157,60.8478102596393,
61.8453153458629,62.8428204320865,63.8403255183101,64.1414162127729),
 .UNSPECIFIED.);
#1662=B_SPLINE_CURVE_WITH_KNOTS('',3,(#77354,#77355,#77356,#77357,#77358,
#77359,#77360,#77361,#77362,#77363,#77364,#77365,#77366,#77367,#77368,#77369,
#77370,#77371,#77372,#77373,#77374,#77375),.UNSPECIFIED.,.F.,.F.,(4,3,3,
3,3,3,3,4),(-60.3976421702575,-59.8503051734157,-58.8528000871921,-57.8552950009685,
-56.8577899147449,-55.8602848285213,-54.8627797422977,-54.1144568630778),
 .UNSPECIFIED.);
#1663=B_SPLINE_CURVE_WITH_KNOTS('',3,(#77380,#77381,#77382,#77383,#77384,
#77385,#77386,#77387,#77388,#77389,#77390,#77391,#77392,#77393,#77394,#77395,
#77396,#77397,#77398,#77399,#77400,#77401,#77402,#77403,#77404),
 .UNSPECIFIED.,.F.,.F.,(4,3,3,3,3,3,3,3,4),(51.5750455984137,51.870264483627,
52.8677695698506,53.8652746560742,54.8627797422978,55.8602848285214,56.857789914745,
57.8552950009686,57.8582309055933),.UNSPECIFIED.);
#1664=B_SPLINE_CURVE_WITH_KNOTS('',3,(#77405,#77406,#77407,#77408,#77409,
#77410,#77411,#77412,#77413,#77414,#77415,#77416,#77417,#77418,#77419,#77420,
#77421,#77422,#77423,#77424,#77425,#77426,#77427,#77428,#77429),
 .UNSPECIFIED.,.F.,.F.,(4,3,3,3,3,3,3,3,4),(-54.1144568630778,-53.8652746560741,
-52.8677695698505,-51.8702644836269,-50.8727593974033,-49.8752543111798,
-48.8777492249562,-47.8802441387326,-47.8312715558983),.UNSPECIFIED.);
#1665=B_SPLINE_CURVE_WITH_KNOTS('',3,(#77434,#77435,#77436,#77437,#77438,
#77439,#77440,#77441,#77442,#77443,#77444,#77445,#77446,#77447,#77448,#77449,
#77450,#77451,#77452,#77453,#77454,#77455),.UNSPECIFIED.,.F.,.F.,(4,3,3,
3,3,3,3,4),(45.2918602912341,45.8852339662854,46.882739052509,47.8802441387326,
48.8777492249562,49.8752543111798,50.8727593974034,51.5750455984137),
 .UNSPECIFIED.);
#1666=B_SPLINE_CURVE_WITH_KNOTS('',3,(#77456,#77457,#77458,#77459,#77460,
#77461,#77462,#77463,#77464,#77465,#77466,#77467,#77468,#77469,#77470,#77471,
#77472,#77473,#77474,#77475,#77476,#77477),.UNSPECIFIED.,.F.,.F.,(4,3,3,
3,3,3,3,4),(-47.8312715558983,-46.882739052509,-45.8852339662854,-44.8877288800618,
-43.8902237938382,-42.8927187076146,-41.895213621391,-41.5480862487187),
 .UNSPECIFIED.);
#1667=B_SPLINE_CURVE_WITH_KNOTS('',3,(#77482,#77483,#77484,#77485,#77486,
#77487,#77488,#77489,#77490,#77491,#77492,#77493,#77494,#77495,#77496,#77497,
#77498,#77499,#77500,#77501,#77502,#77503),.UNSPECIFIED.,.F.,.F.,(4,3,3,
3,3,3,3,4),(39.0086749840545,39.9002034489438,40.8977085351674,41.895213621391,
42.8927187076146,43.8902237938382,44.8877288800618,45.2918602912341),
 .UNSPECIFIED.);
#1668=B_SPLINE_CURVE_WITH_KNOTS('',3,(#77504,#77505,#77506,#77507,#77508,
#77509,#77510,#77511,#77512,#77513,#77514,#77515,#77516,#77517,#77518,#77519,
#77520,#77521,#77522,#77523,#77524,#77525),.UNSPECIFIED.,.F.,.F.,(4,3,3,
3,3,3,3,4),(-41.5480862487187,-40.8977085351674,-39.9002034489438,-38.9026983627202,
-37.9051932764966,-36.907688190273,-35.9101831040494,-35.2649009415391),
 .UNSPECIFIED.);
#1669=B_SPLINE_CURVE_WITH_KNOTS('',3,(#77530,#77531,#77532,#77533,#77534,
#77535,#77536,#77537,#77538,#77539,#77540,#77541,#77542,#77543,#77544,#77545,
#77546,#77547,#77548,#77549,#77550,#77551,#77552,#77553,#77554),
 .UNSPECIFIED.,.F.,.F.,(4,3,3,3,3,3,3,3,4),(32.725489676875,32.9176678453786,
33.9151729316022,34.9126780178258,35.9101831040494,36.907688190273,37.9051932764966,
38.9026983627202,39.0086749840545),.UNSPECIFIED.);
#1670=B_SPLINE_CURVE_WITH_KNOTS('',3,(#77555,#77556,#77557,#77558,#77559,
#77560,#77561,#77562,#77563,#77564,#77565,#77566,#77567,#77568,#77569,#77570,
#77571,#77572,#77573,#77574,#77575,#77576),.UNSPECIFIED.,.F.,.F.,(4,3,3,
3,3,3,3,4),(-35.2649009415391,-34.9126780178258,-33.9151729316022,-32.9176678453786,
-31.920162759155,-30.9226576729314,-29.9251525867079,-28.9817156343595),
 .UNSPECIFIED.);
#1671=B_SPLINE_CURVE_WITH_KNOTS('',3,(#77581,#77582,#77583,#77584,#77585,
#77586,#77587,#77588,#77589,#77590,#77591,#77592,#77593,#77594,#77595,#77596,
#77597,#77598,#77599,#77600,#77601,#77602),.UNSPECIFIED.,.F.,.F.,(4,3,3,
3,3,3,3,4),(26.4423043696954,26.9326373280371,27.9301424142607,28.9276475004843,
29.9251525867079,30.9226576729315,31.920162759155,32.725489676875),
 .UNSPECIFIED.);
#1672=B_SPLINE_CURVE_WITH_KNOTS('',3,(#77603,#77604,#77605,#77606,#77607,
#77608,#77609,#77610,#77611,#77612,#77613,#77614,#77615,#77616,#77617,#77618,
#77619,#77620,#77621,#77622,#77623,#77624,#77625,#77626,#77627),
 .UNSPECIFIED.,.F.,.F.,(4,3,3,3,3,3,3,3,4),(-28.9817156343595,-28.9276475004843,
-27.9301424142607,-26.9326373280371,-25.9351322418135,-24.9376271555899,
-23.9401220693663,-22.9426169831427,-22.6985303271799),.UNSPECIFIED.);
#1673=B_SPLINE_CURVE_WITH_KNOTS('',3,(#77632,#77633,#77634,#77635,#77636,
#77637,#77638,#77639,#77640,#77641,#77642,#77643,#77644,#77645,#77646,#77647,
#77648,#77649,#77650,#77651,#77652,#77653),.UNSPECIFIED.,.F.,.F.,(4,3,3,
3,3,3,3,4),(20.1591190625158,20.9476068106955,21.9451118969191,22.9426169831427,
23.9401220693663,24.9376271555899,25.9351322418135,26.4423043696954),
 .UNSPECIFIED.);
#1674=B_SPLINE_CURVE_WITH_KNOTS('',3,(#77654,#77655,#77656,#77657,#77658,
#77659,#77660,#77661,#77662,#77663,#77664,#77665,#77666,#77667,#77668,#77669,
#77670,#77671,#77672,#77673,#77674,#77675),.UNSPECIFIED.,.F.,.F.,(4,3,3,
3,3,3,3,4),(-22.6985303271799,-21.9451118969191,-20.9476068106955,-19.9501017244719,
-18.9525966382483,-17.9550915520247,-16.9575864658011,-16.4153450200003),
 .UNSPECIFIED.);
#1675=B_SPLINE_CURVE_WITH_KNOTS('',3,(#77680,#77681,#77682,#77683,#77684,
#77685,#77686,#77687,#77688,#77689,#77690,#77691,#77692,#77693,#77694,#77695,
#77696,#77697,#77698,#77699,#77700,#77701,#77702,#77703,#77704),
 .UNSPECIFIED.,.F.,.F.,(4,3,3,3,3,3,3,3,4),(13.8759337553362,13.9650712071303,
14.9625762933539,15.9600813795775,16.9575864658011,17.9550915520247,18.9525966382483,
19.9501017244719,20.1591190625158),.UNSPECIFIED.);
#1676=B_SPLINE_CURVE_WITH_KNOTS('',3,(#77705,#77706,#77707,#77708,#77709,
#77710,#77711,#77712,#77713,#77714,#77715,#77716,#77717,#77718,#77719,#77720,
#77721,#77722,#77723,#77724,#77725,#77726),.UNSPECIFIED.,.F.,.F.,(4,3,3,
3,3,3,3,4),(-16.4153450200003,-15.9600813795775,-14.9625762933539,-13.9650712071303,
-12.9675661209067,-11.9700610346831,-10.9725559484595,-10.1321597128207),
 .UNSPECIFIED.);
#1677=B_SPLINE_CURVE_WITH_KNOTS('',3,(#77732,#77733,#77734,#77735,#77736,
#77737,#77738,#77739,#77740,#77741,#77742,#77743,#77744),.UNSPECIFIED.,
 .F.,.F.,(4,3,3,3,4),(-3.84897440564114,-2.99251525867079,-1.99501017244719,
-0.997505086223596,0.),.UNSPECIFIED.);
#1678=B_SPLINE_CURVE_WITH_KNOTS('',3,(#77747,#77748,#77749,#77750,#77751,
#77752,#77753,#77754,#77755,#77756,#77757,#77758,#77759,#77760,#77761,#77762,
#77763,#77764,#77765),.UNSPECIFIED.,.F.,.F.,(4,3,3,3,3,3,4),(2.01694489302841,
2.99251525867079,3.99002034489439,4.98752543111798,5.98503051734158,6.98253560356517,
7.5927484481566),.UNSPECIFIED.);
#1679=B_SPLINE_CURVE_WITH_KNOTS('',3,(#77771,#77772,#77773,#77774),
 .UNSPECIFIED.,.F.,.F.,(4,4),(126.973269284569,127.68065103662),
 .UNSPECIFIED.);
#1680=B_SPLINE_CURVE_WITH_KNOTS('',3,(#77777,#77778,#77779,#77780,#77781,
#77782,#77783,#77784,#77785,#77786),.UNSPECIFIED.,.F.,.F.,(4,3,3,4),(-125.663706143592,
-124.688135777949,-123.690630691726,-123.229495242053),.UNSPECIFIED.);
#1681=B_SPLINE_CURVE_WITH_KNOTS('',3,(#77791,#77792,#77793,#77794,#77795,
#77796,#77797,#77798,#77799,#77800,#77801,#77802,#77803,#77804,#77805,#77806,
#77807,#77808,#77809,#77810,#77811,#77812,#77813,#77814,#77815),
 .UNSPECIFIED.,.F.,.F.,(4,3,3,3,3,3,3,3,4),(120.690083977389,120.698115433055,
121.695620519279,122.693125605502,123.690630691726,124.688135777949,125.685640864173,
126.683145950397,126.973269284569),.UNSPECIFIED.);
#1682=B_SPLINE_CURVE_WITH_KNOTS('',3,(#77816,#77817,#77818,#77819,#77820,
#77821,#77822,#77823,#77824,#77825,#77826,#77827,#77828,#77829,#77830,#77831,
#77832,#77833,#77834,#77835,#77836,#77837),.UNSPECIFIED.,.F.,.F.,(4,3,3,
3,3,3,3,4),(-123.229495242053,-122.693125605502,-121.695620519279,-120.698115433055,
-119.700610346831,-118.703105260608,-117.705600174384,-116.946309934874),
 .UNSPECIFIED.);
#1683=B_SPLINE_CURVE_WITH_KNOTS('',3,(#77842,#77843,#77844,#77845,#77846,
#77847,#77848,#77849,#77850,#77851,#77852,#77853,#77854,#77855,#77856,#77857,
#77858,#77859,#77860,#77861,#77862,#77863),.UNSPECIFIED.,.F.,.F.,(4,3,3,
3,3,3,3,4),(114.40689867021,114.713084915713,115.710590001937,116.708095088161,
117.705600174384,118.703105260608,119.700610346831,120.690083977389),
 .UNSPECIFIED.);
#1684=B_SPLINE_CURVE_WITH_KNOTS('',3,(#77864,#77865,#77866,#77867,#77868,
#77869,#77870,#77871,#77872,#77873,#77874,#77875,#77876,#77877,#77878,#77879,
#77880,#77881,#77882,#77883,#77884,#77885,#77886,#77887,#77888),
 .UNSPECIFIED.,.F.,.F.,(4,3,3,3,3,3,3,3,4),(-116.946309934874,-116.708095088161,
-115.710590001937,-114.713084915713,-113.71557982949,-112.718074743266,
-111.720569657043,-110.723064570819,-110.663124627694),.UNSPECIFIED.);
#1685=B_SPLINE_CURVE_WITH_KNOTS('',3,(#77893,#77894,#77895,#77896,#77897,
#77898,#77899,#77900,#77901,#77902,#77903,#77904,#77905,#77906,#77907,#77908,
#77909,#77910,#77911,#77912,#77913,#77914),.UNSPECIFIED.,.F.,.F.,(4,3,3,
3,3,3,3,4),(108.12371336303,108.728054398372,109.725559484595,110.723064570819,
111.720569657043,112.718074743266,113.71557982949,114.40689867021),
 .UNSPECIFIED.);
#1686=B_SPLINE_CURVE_WITH_KNOTS('',3,(#77915,#77916,#77917,#77918,#77919,
#77920,#77921,#77922,#77923,#77924,#77925,#77926,#77927,#77928,#77929,#77930,
#77931,#77932,#77933,#77934,#77935,#77936),.UNSPECIFIED.,.F.,.F.,(4,3,3,
3,3,3,3,4),(-110.663124627694,-109.725559484595,-108.728054398372,-107.730549312148,
-106.733044225925,-105.735539139701,-104.738034053477,-104.379939320515),
 .UNSPECIFIED.);
#1687=B_SPLINE_CURVE_WITH_KNOTS('',3,(#77941,#77942,#77943,#77944,#77945,
#77946,#77947,#77948,#77949,#77950,#77951,#77952,#77953,#77954,#77955,#77956,
#77957,#77958,#77959,#77960,#77961,#77962),.UNSPECIFIED.,.F.,.F.,(4,3,3,
3,3,3,3,4),(101.84052805585,102.74302388103,103.740528967254,104.738034053478,
105.735539139701,106.733044225925,107.730549312148,108.12371336303),
 .UNSPECIFIED.);
#1688=B_SPLINE_CURVE_WITH_KNOTS('',3,(#77963,#77964,#77965,#77966,#77967,
#77968,#77969,#77970,#77971,#77972,#77973,#77974,#77975,#77976,#77977,#77978,
#77979,#77980,#77981,#77982,#77983,#77984),.UNSPECIFIED.,.F.,.F.,(4,3,3,
3,3,3,3,4),(-104.379939320515,-103.740528967254,-102.74302388103,-101.745518794807,
-100.748013708583,-99.7505086223595,-98.7530035361359,-98.096754013335),
 .UNSPECIFIED.);
#1689=B_SPLINE_CURVE_WITH_KNOTS('',3,(#77989,#77990,#77991,#77992,#77993,
#77994,#77995,#77996,#77997,#77998,#77999,#78000,#78001,#78002,#78003,#78004,
#78005,#78006,#78007,#78008,#78009,#78010,#78011,#78012,#78013),
 .UNSPECIFIED.,.F.,.F.,(4,3,3,3,3,3,3,3,4),(95.5573427486709,95.7604882774652,
96.7579933636888,97.7554984499123,98.7530035361359,99.7505086223595,100.748013708583,
101.745518794807,101.84052805585),.UNSPECIFIED.);
#1690=B_SPLINE_CURVE_WITH_KNOTS('',3,(#78014,#78015,#78016,#78017,#78018,
#78019,#78020,#78021,#78022,#78023,#78024,#78025,#78026,#78027,#78028,#78029,
#78030,#78031,#78032,#78033,#78034,#78035),.UNSPECIFIED.,.F.,.F.,(4,3,3,
3,3,3,3,4),(-98.096754013335,-97.7554984499123,-96.7579933636887,-95.7604882774651,
-94.7629831912415,-93.7654781050179,-92.7679730187943,-91.8135687061554),
 .UNSPECIFIED.);
#1691=B_SPLINE_CURVE_WITH_KNOTS('',3,(#78040,#78041,#78042,#78043,#78044,
#78045,#78046,#78047,#78048,#78049,#78050,#78051,#78052,#78053,#78054,#78055,
#78056,#78057,#78058,#78059,#78060,#78061),.UNSPECIFIED.,.F.,.F.,(4,3,3,
3,3,3,3,4),(89.2741574414913,89.7754577601236,90.7729628463472,91.7704679325708,
92.7679730187944,93.765478105018,94.7629831912416,95.5573427486709),
 .UNSPECIFIED.);
#1692=B_SPLINE_CURVE_WITH_KNOTS('',3,(#78062,#78063,#78064,#78065,#78066,
#78067,#78068,#78069,#78070,#78071,#78072,#78073,#78074,#78075,#78076,#78077,
#78078,#78079,#78080,#78081,#78082,#78083,#78084,#78085,#78086),
 .UNSPECIFIED.,.F.,.F.,(4,3,3,3,3,3,3,3,4),(-91.8135687061554,-91.7704679325708,
-90.7729628463472,-89.7754577601236,-88.7779526739,-87.7804475876764,-86.7829425014528,
-85.7854374152292,-85.5303833989758),.UNSPECIFIED.);
#1693=B_SPLINE_CURVE_WITH_KNOTS('',3,(#78091,#78092,#78093,#78094,#78095,
#78096,#78097,#78098,#78099,#78100,#78101,#78102,#78103,#78104,#78105,#78106,
#78107,#78108,#78109,#78110,#78111,#78112),.UNSPECIFIED.,.F.,.F.,(4,3,3,
3,3,3,3,4),(82.9909721343117,83.790427242782,84.7879323290056,85.7854374152292,
86.7829425014528,87.7804475876764,88.7779526739,89.2741574414913),
 .UNSPECIFIED.);
#1694=B_SPLINE_CURVE_WITH_KNOTS('',3,(#78113,#78114,#78115,#78116,#78117,
#78118,#78119,#78120,#78121,#78122,#78123,#78124,#78125,#78126,#78127,#78128,
#78129,#78130,#78131,#78132,#78133,#78134),.UNSPECIFIED.,.F.,.F.,(4,3,3,
3,3,3,3,4),(-85.5303833989758,-84.7879323290056,-83.790427242782,-82.7929221565584,
-81.7954170703348,-80.7979119841112,-79.8004068978876,-79.2471980917962),
 .UNSPECIFIED.);
#1695=B_SPLINE_CURVE_WITH_KNOTS('',3,(#78139,#78140,#78141,#78142,#78143,
#78144,#78145,#78146,#78147,#78148,#78149,#78150,#78151,#78152,#78153,#78154,
#78155,#78156,#78157,#78158,#78159,#78160,#78161,#78162,#78163),
 .UNSPECIFIED.,.F.,.F.,(4,3,3,3,3,3,3,3,4),(76.7077868271321,76.8078916392168,
77.8053967254404,78.802901811664,79.8004068978876,80.7979119841112,81.7954170703348,
82.7929221565584,82.9909721343117),.UNSPECIFIED.);
#1696=B_SPLINE_CURVE_WITH_KNOTS('',3,(#78164,#78165,#78166,#78167,#78168,
#78169,#78170,#78171,#78172,#78173,#78174,#78175,#78176,#78177,#78178,#78179,
#78180,#78181,#78182,#78183,#78184,#78185),.UNSPECIFIED.,.F.,.F.,(4,3,3,
3,3,3,3,4),(-79.2471980917962,-78.802901811664,-77.8053967254404,-76.8078916392168,
-75.8103865529932,-74.8128814667696,-73.815376380546,-72.9640127846166),
 .UNSPECIFIED.);
#1697=B_SPLINE_CURVE_WITH_KNOTS('',3,(#78190,#78191,#78192,#78193,#78194,
#78195,#78196,#78197,#78198,#78199,#78200,#78201,#78202,#78203,#78204,#78205,
#78206,#78207,#78208,#78209,#78210,#78211),.UNSPECIFIED.,.F.,.F.,(4,3,3,
3,3,3,3,4),(70.4246015199525,70.8228611218753,71.8203662080989,72.8178712943224,
73.8153763805461,74.8128814667696,75.8103865529933,76.7077868271321),
 .UNSPECIFIED.);
#1698=B_SPLINE_CURVE_WITH_KNOTS('',3,(#78212,#78213,#78214,#78215,#78216,
#78217,#78218,#78219,#78220,#78221,#78222,#78223,#78224,#78225,#78226,#78227,
#78228,#78229,#78230,#78231,#78232,#78233,#78234,#78235,#78236),
 .UNSPECIFIED.,.F.,.F.,(4,3,3,3,3,3,3,3,4),(-72.9640127846166,-72.8178712943224,
-71.8203662080988,-70.8228611218752,-69.8253560356517,-68.827850949428,
-67.8303458632045,-66.8328407769809,-66.680827477437),.UNSPECIFIED.);
#1699=B_SPLINE_CURVE_WITH_KNOTS('',3,(#78241,#78242,#78243,#78244,#78245,
#78246,#78247,#78248,#78249,#78250,#78251,#78252,#78253,#78254,#78255,#78256,
#78257,#78258,#78259,#78260,#78261,#78262),.UNSPECIFIED.,.F.,.F.,(4,3,3,
3,3,3,3,4),(64.1414162127729,64.8378306045337,65.8353356907573,66.8328407769809,
67.8303458632045,68.8278509494281,69.8253560356517,70.4246015199525),
 .UNSPECIFIED.);
#1700=B_SPLINE_CURVE_WITH_KNOTS('',3,(#78263,#78264,#78265,#78266,#78267,
#78268,#78269,#78270,#78271,#78272,#78273,#78274,#78275,#78276,#78277,#78278,
#78279,#78280,#78281,#78282,#78283,#78284),.UNSPECIFIED.,.F.,.F.,(4,3,3,
3,3,3,3,4),(-66.680827477437,-65.8353356907573,-64.8378306045337,-63.8403255183101,
-62.8428204320865,-61.8453153458629,-60.8478102596393,-60.3976421702574),
 .UNSPECIFIED.);
#1701=B_SPLINE_CURVE_WITH_KNOTS('',3,(#78289,#78290,#78291,#78292,#78293,
#78294,#78295,#78296,#78297,#78298,#78299,#78300,#78301,#78302,#78303,#78304,
#78305,#78306,#78307,#78308,#78309,#78310),.UNSPECIFIED.,.F.,.F.,(4,3,3,
3,3,3,3,4),(57.8582309055933,58.8528000871921,59.8503051734157,60.8478102596393,
61.8453153458629,62.8428204320865,63.8403255183101,64.1414162127729),
 .UNSPECIFIED.);
#1702=B_SPLINE_CURVE_WITH_KNOTS('',3,(#78311,#78312,#78313,#78314,#78315,
#78316,#78317,#78318,#78319,#78320,#78321,#78322,#78323,#78324,#78325,#78326,
#78327,#78328,#78329,#78330,#78331,#78332),.UNSPECIFIED.,.F.,.F.,(4,3,3,
3,3,3,3,4),(-60.3976421702574,-59.8503051734157,-58.8528000871921,-57.8552950009685,
-56.8577899147449,-55.8602848285213,-54.8627797422977,-54.1144568630778),
 .UNSPECIFIED.);
#1703=B_SPLINE_CURVE_WITH_KNOTS('',3,(#78337,#78338,#78339,#78340,#78341,
#78342,#78343,#78344,#78345,#78346,#78347,#78348,#78349,#78350,#78351,#78352,
#78353,#78354,#78355,#78356,#78357,#78358,#78359,#78360,#78361),
 .UNSPECIFIED.,.F.,.F.,(4,3,3,3,3,3,3,3,4),(51.5750455984137,51.870264483627,
52.8677695698506,53.8652746560742,54.8627797422977,55.8602848285214,56.8577899147449,
57.8552950009685,57.8582309055933),.UNSPECIFIED.);
#1704=B_SPLINE_CURVE_WITH_KNOTS('',3,(#78362,#78363,#78364,#78365,#78366,
#78367,#78368,#78369,#78370,#78371,#78372,#78373,#78374,#78375,#78376,#78377,
#78378,#78379,#78380,#78381,#78382,#78383,#78384,#78385,#78386),
 .UNSPECIFIED.,.F.,.F.,(4,3,3,3,3,3,3,3,4),(-54.1144568630778,-53.8652746560741,
-52.8677695698505,-51.8702644836269,-50.8727593974033,-49.8752543111797,
-48.8777492249561,-47.8802441387326,-47.8312715558983),.UNSPECIFIED.);
#1705=B_SPLINE_CURVE_WITH_KNOTS('',3,(#78391,#78392,#78393,#78394,#78395,
#78396,#78397,#78398,#78399,#78400,#78401,#78402,#78403,#78404,#78405,#78406,
#78407,#78408,#78409,#78410,#78411,#78412),.UNSPECIFIED.,.F.,.F.,(4,3,3,
3,3,3,3,4),(45.2918602912341,45.8852339662854,46.882739052509,47.8802441387326,
48.8777492249562,49.8752543111798,50.8727593974034,51.5750455984137),
 .UNSPECIFIED.);
#1706=B_SPLINE_CURVE_WITH_KNOTS('',3,(#78413,#78414,#78415,#78416,#78417,
#78418,#78419,#78420,#78421,#78422,#78423,#78424,#78425,#78426,#78427,#78428,
#78429,#78430,#78431,#78432,#78433,#78434),.UNSPECIFIED.,.F.,.F.,(4,3,3,
3,3,3,3,4),(-47.8312715558983,-46.882739052509,-45.8852339662854,-44.8877288800618,
-43.8902237938382,-42.8927187076146,-41.895213621391,-41.5480862487187),
 .UNSPECIFIED.);
#1707=B_SPLINE_CURVE_WITH_KNOTS('',3,(#78439,#78440,#78441,#78442,#78443,
#78444,#78445,#78446,#78447,#78448,#78449,#78450,#78451,#78452,#78453,#78454,
#78455,#78456,#78457,#78458,#78459,#78460),.UNSPECIFIED.,.F.,.F.,(4,3,3,
3,3,3,3,4),(39.0086749840545,39.9002034489438,40.8977085351674,41.895213621391,
42.8927187076146,43.8902237938382,44.8877288800618,45.2918602912341),
 .UNSPECIFIED.);
#1708=B_SPLINE_CURVE_WITH_KNOTS('',3,(#78461,#78462,#78463,#78464,#78465,
#78466,#78467,#78468,#78469,#78470,#78471,#78472,#78473,#78474,#78475,#78476,
#78477,#78478,#78479,#78480,#78481,#78482),.UNSPECIFIED.,.F.,.F.,(4,3,3,
3,3,3,3,4),(-41.5480862487187,-40.8977085351674,-39.9002034489438,-38.9026983627202,
-37.9051932764966,-36.907688190273,-35.9101831040494,-35.2649009415391),
 .UNSPECIFIED.);
#1709=B_SPLINE_CURVE_WITH_KNOTS('',3,(#78487,#78488,#78489,#78490,#78491,
#78492,#78493,#78494,#78495,#78496,#78497,#78498,#78499,#78500,#78501,#78502,
#78503,#78504,#78505,#78506,#78507,#78508,#78509,#78510,#78511),
 .UNSPECIFIED.,.F.,.F.,(4,3,3,3,3,3,3,3,4),(32.7254896768749,32.9176678453786,
33.9151729316022,34.9126780178258,35.9101831040494,36.907688190273,37.9051932764966,
38.9026983627202,39.0086749840545),.UNSPECIFIED.);
#1710=B_SPLINE_CURVE_WITH_KNOTS('',3,(#78512,#78513,#78514,#78515,#78516,
#78517,#78518,#78519,#78520,#78521,#78522,#78523,#78524,#78525,#78526,#78527,
#78528,#78529,#78530,#78531,#78532,#78533),.UNSPECIFIED.,.F.,.F.,(4,3,3,
3,3,3,3,4),(-35.2649009415391,-34.9126780178258,-33.9151729316022,-32.9176678453786,
-31.920162759155,-30.9226576729314,-29.9251525867078,-28.9817156343595),
 .UNSPECIFIED.);
#1711=B_SPLINE_CURVE_WITH_KNOTS('',3,(#78538,#78539,#78540,#78541,#78542,
#78543,#78544,#78545,#78546,#78547,#78548,#78549,#78550,#78551,#78552,#78553,
#78554,#78555,#78556,#78557,#78558,#78559),.UNSPECIFIED.,.F.,.F.,(4,3,3,
3,3,3,3,4),(26.4423043696953,26.9326373280371,27.9301424142607,28.9276475004843,
29.9251525867079,30.9226576729315,31.920162759155,32.7254896768749),
 .UNSPECIFIED.);
#1712=B_SPLINE_CURVE_WITH_KNOTS('',3,(#78560,#78561,#78562,#78563,#78564,
#78565,#78566,#78567,#78568,#78569,#78570,#78571,#78572,#78573,#78574,#78575,
#78576,#78577,#78578,#78579,#78580,#78581,#78582,#78583,#78584),
 .UNSPECIFIED.,.F.,.F.,(4,3,3,3,3,3,3,3,4),(-28.9817156343595,-28.9276475004843,
-27.9301424142607,-26.9326373280371,-25.9351322418135,-24.9376271555899,
-23.9401220693663,-22.9426169831427,-22.6985303271799),.UNSPECIFIED.);
#1713=B_SPLINE_CURVE_WITH_KNOTS('',3,(#78589,#78590,#78591,#78592,#78593,
#78594,#78595,#78596,#78597,#78598,#78599,#78600,#78601,#78602,#78603,#78604,
#78605,#78606,#78607,#78608,#78609,#78610),.UNSPECIFIED.,.F.,.F.,(4,3,3,
3,3,3,3,4),(20.1591190625158,20.9476068106955,21.9451118969191,22.9426169831427,
23.9401220693663,24.9376271555899,25.9351322418135,26.4423043696953),
 .UNSPECIFIED.);
#1714=B_SPLINE_CURVE_WITH_KNOTS('',3,(#78611,#78612,#78613,#78614,#78615,
#78616,#78617,#78618,#78619,#78620,#78621,#78622,#78623,#78624,#78625,#78626,
#78627,#78628,#78629,#78630,#78631,#78632),.UNSPECIFIED.,.F.,.F.,(4,3,3,
3,3,3,3,4),(-22.6985303271799,-21.9451118969191,-20.9476068106955,-19.9501017244719,
-18.9525966382483,-17.9550915520247,-16.9575864658011,-16.4153450200003),
 .UNSPECIFIED.);
#1715=B_SPLINE_CURVE_WITH_KNOTS('',3,(#78637,#78638,#78639,#78640,#78641,
#78642,#78643,#78644,#78645,#78646,#78647,#78648,#78649,#78650,#78651,#78652,
#78653,#78654,#78655,#78656,#78657,#78658,#78659,#78660,#78661),
 .UNSPECIFIED.,.F.,.F.,(4,3,3,3,3,3,3,3,4),(13.8759337553362,13.9650712071303,
14.9625762933539,15.9600813795775,16.9575864658011,17.9550915520247,18.9525966382483,
19.9501017244719,20.1591190625158),.UNSPECIFIED.);
#1716=B_SPLINE_CURVE_WITH_KNOTS('',3,(#78662,#78663,#78664,#78665,#78666,
#78667,#78668,#78669,#78670,#78671,#78672,#78673,#78674,#78675,#78676,#78677,
#78678,#78679,#78680,#78681,#78682,#78683),.UNSPECIFIED.,.F.,.F.,(4,3,3,
3,3,3,3,4),(-16.4153450200003,-15.9600813795775,-14.9625762933539,-13.9650712071303,
-12.9675661209067,-11.9700610346831,-10.9725559484596,-10.1321597128207),
 .UNSPECIFIED.);
#1717=B_SPLINE_CURVE_WITH_KNOTS('',3,(#78689,#78690,#78691,#78692,#78693,
#78694,#78695,#78696,#78697,#78698,#78699,#78700,#78701),.UNSPECIFIED.,
 .F.,.F.,(4,3,3,3,4),(-3.84897440564113,-2.99251525867078,-1.99501017244719,
-0.997505086223595,0.),.UNSPECIFIED.);
#1718=B_SPLINE_CURVE_WITH_KNOTS('',3,(#78704,#78705,#78706,#78707,#78708,
#78709,#78710,#78711,#78712,#78713,#78714,#78715,#78716,#78717,#78718,#78719,
#78720,#78721,#78722),.UNSPECIFIED.,.F.,.F.,(4,3,3,3,3,3,4),(2.01694489302833,
2.99251525867079,3.99002034489438,4.98752543111798,5.98503051734158,6.98253560356517,
7.59274844815659),.UNSPECIFIED.);
#1719=B_SPLINE_CURVE_WITH_KNOTS('',3,(#78728,#78729,#78730,#78731,#78732,
#78733,#78734,#78735),.UNSPECIFIED.,.F.,.F.,(4,1,1,1,1,4),(135.088484104361,
135.549619554034,136.547124640257,137.544629726481,138.542134812704,139.539639898928),
 .UNSPECIFIED.);
#1720=B_SPLINE_CURVE_WITH_KNOTS('',3,(#78738,#78739,#78740,#78741,#78742,
#78743,#78744,#78745,#78746),.UNSPECIFIED.,.F.,.F.,(4,1,1,1,1,1,4),(135.088484104361,
135.096515560027,136.09402064625,137.091525732474,138.089030818698,139.086535904921,
140.062106270563),.UNSPECIFIED.);
#1721=B_SPLINE_CURVE_WITH_KNOTS('',3,(#78751,#78752,#78753,#78754,#78755,
#78756,#78757,#78758,#78759,#78760),.UNSPECIFIED.,.F.,.F.,(4,1,1,1,1,1,
1,4),(128.805298797182,129.564589036692,130.562094122916,131.559599209139,
132.557104295363,133.554609381586,134.55211446781,135.088484104361),
 .UNSPECIFIED.);
#1722=B_SPLINE_CURVE_WITH_KNOTS('',3,(#78761,#78762,#78763,#78764,#78765,
#78766,#78767,#78768,#78769,#78770),.UNSPECIFIED.,.F.,.F.,(4,1,1,1,1,1,
1,4),(128.805298797182,129.111485042685,130.108990128909,131.106495215132,
132.104000301356,133.10150538758,134.099010473803,135.088484104361),
 .UNSPECIFIED.);
#1723=B_SPLINE_CURVE_WITH_KNOTS('',3,(#78775,#78776,#78777,#78778,#78779,
#78780,#78781,#78782,#78783,#78784,#78785),.UNSPECIFIED.,.F.,.F.,(4,1,1,
1,1,1,1,1,4),(122.522113490002,122.582053433127,123.57955851935,124.577063605574,
125.574568691798,126.572073778021,127.569578864245,128.567083950468,128.805298797182),
 .UNSPECIFIED.);
#1724=B_SPLINE_CURVE_WITH_KNOTS('',3,(#78786,#78787,#78788,#78789,#78790,
#78791,#78792,#78793,#78794,#78795),.UNSPECIFIED.,.F.,.F.,(4,1,1,1,1,1,
1,4),(122.522113490002,123.126454525344,124.123959611567,125.121464697791,
126.118969784014,127.116474870238,128.113979956462,128.805298797182),
 .UNSPECIFIED.);
#1725=B_SPLINE_CURVE_WITH_KNOTS('',3,(#78800,#78801,#78802,#78803,#78804,
#78805,#78806,#78807,#78808,#78809),.UNSPECIFIED.,.F.,.F.,(4,1,1,1,1,1,
1,4),(116.238928182822,116.597022915785,117.594528002009,118.592033088232,
119.589538174456,120.58704326068,121.584548346903,122.522113490002),
 .UNSPECIFIED.);
#1726=B_SPLINE_CURVE_WITH_KNOTS('',3,(#78810,#78811,#78812,#78813,#78814,
#78815,#78816,#78817,#78818,#78819),.UNSPECIFIED.,.F.,.F.,(4,1,1,1,1,1,
1,4),(116.238928182822,117.141424008002,118.138929094226,119.136434180449,
120.133939266673,121.131444352896,122.12894943912,122.522113490002),
 .UNSPECIFIED.);
#1727=B_SPLINE_CURVE_WITH_KNOTS('',3,(#78824,#78825,#78826,#78827,#78828,
#78829,#78830,#78831,#78832,#78833),.UNSPECIFIED.,.F.,.F.,(4,1,1,1,1,1,
1,4),(109.955742875643,110.611992398444,111.609497484667,112.607002570891,
113.604507657114,114.602012743338,115.599517829562,116.238928182822),
 .UNSPECIFIED.);
#1728=B_SPLINE_CURVE_WITH_KNOTS('',3,(#78834,#78835,#78836,#78837,#78838,
#78839,#78840,#78841,#78842,#78843,#78844),.UNSPECIFIED.,.F.,.F.,(4,1,1,
1,1,1,1,1,4),(109.955742875643,110.158888404437,111.156393490661,112.153898576884,
113.151403663108,114.148908749331,115.146413835555,116.143918921778,116.238928182822),
 .UNSPECIFIED.);
#1729=B_SPLINE_CURVE_WITH_KNOTS('',3,(#78849,#78850,#78851,#78852,#78853,
#78854,#78855,#78856,#78857,#78858),.UNSPECIFIED.,.F.,.F.,(4,1,1,1,1,1,
1,4),(103.672557568463,104.626961881102,105.624466967326,106.621972053549,
107.619477139773,108.616982225996,109.61448731222,109.955742875643),
 .UNSPECIFIED.);
#1730=B_SPLINE_CURVE_WITH_KNOTS('',3,(#78859,#78860,#78861,#78862,#78863,
#78864,#78865,#78866,#78867,#78868),.UNSPECIFIED.,.F.,.F.,(4,1,1,1,1,1,
1,4),(103.672557568463,104.173857887095,105.171362973319,106.168868059543,
107.166373145766,108.16387823199,109.161383318213,109.955742875643),
 .UNSPECIFIED.);
#1731=B_SPLINE_CURVE_WITH_KNOTS('',3,(#78873,#78874,#78875,#78876,#78877,
#78878,#78879,#78880,#78881,#78882,#78883),.UNSPECIFIED.,.F.,.F.,(4,1,1,
1,1,1,1,1,4),(97.3893722612835,97.6444262775369,98.6419313637605,99.6394364499841,
100.636941536208,101.634446622431,102.631951708655,103.629456794878,103.672557568463),
 .UNSPECIFIED.);
#1732=B_SPLINE_CURVE_WITH_KNOTS('',3,(#78884,#78885,#78886,#78887,#78888,
#78889,#78890,#78891,#78892,#78893),.UNSPECIFIED.,.F.,.F.,(4,1,1,1,1,1,
1,4),(97.3893722612836,98.1888273697538,99.1863324559774,100.183837542201,
101.181342628425,102.178847714648,103.176352800872,103.672557568463),
 .UNSPECIFIED.);
#1733=B_SPLINE_CURVE_WITH_KNOTS('',3,(#78898,#78899,#78900,#78901,#78902,
#78903,#78904,#78905,#78906,#78907),.UNSPECIFIED.,.F.,.F.,(4,1,1,1,1,1,
1,4),(91.106186954104,91.6593957601953,92.6569008464189,93.6544059326425,
94.6519110188661,95.6494161050897,96.6469211913133,97.3893722612835),
 .UNSPECIFIED.);
#1734=B_SPLINE_CURVE_WITH_KNOTS('',3,(#78908,#78909,#78910,#78911,#78912,
#78913,#78914,#78915,#78916,#78917,#78918),.UNSPECIFIED.,.F.,.F.,(4,1,1,
1,1,1,1,1,4),(91.106186954104,91.2062917661886,92.2037968524122,93.2013019386358,
94.1988070248594,95.196312111083,96.1938171973066,97.1913222835302,97.3893722612836),
 .UNSPECIFIED.);
#1735=B_SPLINE_CURVE_WITH_KNOTS('',3,(#78923,#78924,#78925,#78926,#78927,
#78928,#78929,#78930,#78931,#78932),.UNSPECIFIED.,.F.,.F.,(4,1,1,1,1,1,
1,4),(84.8230016469244,85.6743652428538,86.6718703290774,87.669375415301,
88.6668805015246,89.6643855877482,90.6618906739717,91.106186954104),
 .UNSPECIFIED.);
#1736=B_SPLINE_CURVE_WITH_KNOTS('',3,(#78933,#78934,#78935,#78936,#78937,
#78938,#78939,#78940,#78941,#78942),.UNSPECIFIED.,.F.,.F.,(4,1,1,1,1,1,
1,4),(84.8230016469244,85.221261248847,86.2187663350706,87.2162714212942,
88.2137765075178,89.2112815937414,90.208786679965,91.106186954104),
 .UNSPECIFIED.);
#1737=B_SPLINE_CURVE_WITH_KNOTS('',3,(#78947,#78948,#78949,#78950,#78951,
#78952,#78953,#78954,#78955,#78956,#78957),.UNSPECIFIED.,.F.,.F.,(4,1,1,
1,1,1,1,1,4),(78.5398163397448,78.6918296392886,79.6893347255122,80.6868398117358,
81.6843448979594,82.681849984183,83.6793550704066,84.6768601566302,84.8230016469244),
 .UNSPECIFIED.);
#1738=B_SPLINE_CURVE_WITH_KNOTS('',3,(#78958,#78959,#78960,#78961,#78962,
#78963,#78964,#78965,#78966,#78967),.UNSPECIFIED.,.F.,.F.,(4,1,1,1,1,1,
1,4),(78.5398163397448,79.2362307315055,80.2337358177291,81.2312409039527,
82.2287459901763,83.2262510763998,84.2237561626234,84.8230016469244),
 .UNSPECIFIED.);
#1739=B_SPLINE_CURVE_WITH_KNOTS('',3,(#78972,#78973,#78974,#78975,#78976,
#78977,#78978,#78979,#78980,#78981),.UNSPECIFIED.,.F.,.F.,(4,1,1,1,1,1,
1,4),(72.2566310325652,72.706799121947,73.7043042081706,74.7018092943942,
75.6993143806178,76.6968194668414,77.694324553065,78.5398163397448),
 .UNSPECIFIED.);
#1740=B_SPLINE_CURVE_WITH_KNOTS('',3,(#78982,#78983,#78984,#78985,#78986,
#78987,#78988,#78989,#78990,#78991),.UNSPECIFIED.,.F.,.F.,(4,1,1,1,1,1,
1,4),(72.2566310325652,73.2512002141639,74.2487053003875,75.2462103866111,
76.2437154728347,77.2412205590583,78.2387256452819,78.5398163397448),
 .UNSPECIFIED.);
#1741=B_SPLINE_CURVE_WITH_KNOTS('',3,(#78996,#78997,#78998,#78999,#79000,
#79001,#79002,#79003,#79004,#79005),.UNSPECIFIED.,.F.,.F.,(4,1,1,1,1,1,
1,4),(65.9734457253856,66.7217686046055,67.7192736908291,68.7167787770527,
69.7142838632763,70.7117889494998,71.7092940357234,72.2566310325652),
 .UNSPECIFIED.);
#1742=B_SPLINE_CURVE_WITH_KNOTS('',3,(#79006,#79007,#79008,#79009,#79010,
#79011,#79012,#79013,#79014,#79015,#79016),.UNSPECIFIED.,.F.,.F.,(4,1,1,
1,1,1,1,1,4),(65.9734457253856,66.2686646105987,67.2661696968223,68.2636747830459,
69.2611798692695,70.2586849554931,71.2561900417167,72.2536951279403,72.2566310325652),
 .UNSPECIFIED.);
#1743=B_SPLINE_CURVE_WITH_KNOTS('',3,(#79021,#79022,#79023,#79024,#79025,
#79026,#79027,#79028,#79029,#79030,#79031),.UNSPECIFIED.,.F.,.F.,(4,1,1,
1,1,1,1,1,4),(59.690260418206,59.7392330010403,60.7367380872639,61.7342431734875,
62.7317482597111,63.7292533459347,64.7267584321583,65.7242635183819,65.9734457253856),
 .UNSPECIFIED.);
#1744=B_SPLINE_CURVE_WITH_KNOTS('',3,(#79032,#79033,#79034,#79035,#79036,
#79037,#79038,#79039,#79040,#79041),.UNSPECIFIED.,.F.,.F.,(4,1,1,1,1,1,
1,4),(59.690260418206,60.2836340932571,61.2811391794807,62.2786442657043,
63.2761493519279,64.2736544381515,65.2711595243751,65.9734457253856),
 .UNSPECIFIED.);
#1745=B_SPLINE_CURVE_WITH_KNOTS('',3,(#79046,#79047,#79048,#79049,#79050,
#79051,#79052,#79053,#79054,#79055),.UNSPECIFIED.,.F.,.F.,(4,1,1,1,1,1,
1,4),(53.4070751110264,53.7542024836987,54.7517075699223,55.7492126561459,
56.7467177423695,57.7442228285931,58.7417279148167,59.690260418206),
 .UNSPECIFIED.);
#1746=B_SPLINE_CURVE_WITH_KNOTS('',3,(#79056,#79057,#79058,#79059,#79060,
#79061,#79062,#79063,#79064,#79065),.UNSPECIFIED.,.F.,.F.,(4,1,1,1,1,1,
1,4),(53.4070751110264,54.2986035759156,55.2961086621392,56.2936137483628,
57.2911188345864,58.28862392081,59.2861290070336,59.690260418206),
 .UNSPECIFIED.);
#1747=B_SPLINE_CURVE_WITH_KNOTS('',3,(#79070,#79071,#79072,#79073,#79074,
#79075,#79076,#79077,#79078,#79079),.UNSPECIFIED.,.F.,.F.,(4,1,1,1,1,1,
1,4),(47.1238898038468,47.7691719663572,48.7666770525807,49.7641821388043,
50.7616872250279,51.7591923112515,52.7566973974751,53.4070751110264),
 .UNSPECIFIED.);
#1748=B_SPLINE_CURVE_WITH_KNOTS('',3,(#79080,#79081,#79082,#79083,#79084,
#79085,#79086,#79087,#79088,#79089,#79090),.UNSPECIFIED.,.F.,.F.,(4,1,1,
1,1,1,1,1,4),(47.1238898038468,47.3160679723504,48.313573058574,49.3110781447976,
50.3085832310212,51.3060883172448,52.3035934034684,53.301098489692,53.4070751110264),
 .UNSPECIFIED.);
#1749=B_SPLINE_CURVE_WITH_KNOTS('',3,(#79095,#79096,#79097,#79098,#79099,
#79100,#79101,#79102,#79103,#79104),.UNSPECIFIED.,.F.,.F.,(4,1,1,1,1,1,
1,4),(40.8407044966672,41.7841414490156,42.7816465352392,43.7791516214628,
44.7766567076864,45.77416179391,46.7716668801336,47.1238898038468),
 .UNSPECIFIED.);
#1750=B_SPLINE_CURVE_WITH_KNOTS('',3,(#79105,#79106,#79107,#79108,#79109,
#79110,#79111,#79112,#79113,#79114),.UNSPECIFIED.,.F.,.F.,(4,1,1,1,1,1,
1,4),(40.8407044966673,41.3310374550088,42.3285425412324,43.326047627456,
44.3235527136796,45.3210577999032,46.3185628861268,47.1238898038468),
 .UNSPECIFIED.);
#1751=B_SPLINE_CURVE_WITH_KNOTS('',3,(#79119,#79120,#79121,#79122,#79123,
#79124,#79125,#79126,#79127,#79128,#79129),.UNSPECIFIED.,.F.,.F.,(4,1,1,
1,1,1,1,1,4),(34.5575191894876,34.8016058454504,35.799110931674,36.7966160178976,
37.7941211041212,38.7916261903448,39.7891312765684,40.786636362792,40.8407044966672),
 .UNSPECIFIED.);
#1752=B_SPLINE_CURVE_WITH_KNOTS('',3,(#79130,#79131,#79132,#79133,#79134,
#79135,#79136,#79137,#79138,#79139),.UNSPECIFIED.,.F.,.F.,(4,1,1,1,1,1,
1,4),(34.5575191894877,35.3460069376673,36.3435120238909,37.3410171101145,
38.3385221963381,39.3360272825617,40.3335323687852,40.8407044966673),
 .UNSPECIFIED.);
#1753=B_SPLINE_CURVE_WITH_KNOTS('',3,(#79144,#79145,#79146,#79147,#79148,
#79149,#79150,#79151,#79152,#79153),.UNSPECIFIED.,.F.,.F.,(4,1,1,1,1,1,
1,4),(28.274333882308,28.8165753281089,29.8140804143324,30.811585500556,
31.8090905867796,32.8065956730032,33.8041007592268,34.5575191894876),
 .UNSPECIFIED.);
#1754=B_SPLINE_CURVE_WITH_KNOTS('',3,(#79154,#79155,#79156,#79157,#79158,
#79159,#79160,#79161,#79162,#79163,#79164),.UNSPECIFIED.,.F.,.F.,(4,1,1,
1,1,1,1,1,4),(28.2743338823081,28.3634713341021,29.3609764203257,30.3584815065493,
31.3559865927729,32.3534916789965,33.3509967652201,34.3485018514437,34.5575191894877),
 .UNSPECIFIED.);
#1755=B_SPLINE_CURVE_WITH_KNOTS('',3,(#79169,#79170,#79171,#79172,#79173,
#79174,#79175,#79176,#79177,#79178),.UNSPECIFIED.,.F.,.F.,(4,1,1,1,1,1,
1,4),(21.9911485751285,22.8315448107673,23.8290498969909,24.8265549832145,
25.8240600694381,26.8215651556617,27.8190702418853,28.274333882308),
 .UNSPECIFIED.);
#1756=B_SPLINE_CURVE_WITH_KNOTS('',3,(#79179,#79180,#79181,#79182,#79183,
#79184,#79185,#79186,#79187,#79188),.UNSPECIFIED.,.F.,.F.,(4,1,1,1,1,1,
1,4),(21.9911485751285,22.3784408167605,23.3759459029841,24.3734509892077,
25.3709560754313,26.3684611616549,27.3659662478785,28.2743338823081),
 .UNSPECIFIED.);
#1757=B_SPLINE_CURVE_WITH_KNOTS('',3,(#79194,#79195,#79196,#79197,#79198),
 .UNSPECIFIED.,.F.,.F.,(4,1,4),(14.3984001269718,15.3959052131954,15.7079632679489),
 .UNSPECIFIED.);
#1758=B_SPLINE_CURVE_WITH_KNOTS('',3,(#79201,#79202,#79203,#79204,#79205),
 .UNSPECIFIED.,.F.,.F.,(4,1,4),(13.8759337553362,14.8515041209785,15.7079632679489),
 .UNSPECIFIED.);
#1759=B_SPLINE_CURVE_WITH_KNOTS('',3,(#79211,#79212,#79213,#79214,#79215,
#79216,#79217,#79218),.UNSPECIFIED.,.F.,.F.,(4,1,1,1,1,4),(135.088484104361,
135.549619554034,136.547124640257,137.544629726481,138.542134812704,139.539639898928),
 .UNSPECIFIED.);
#1760=B_SPLINE_CURVE_WITH_KNOTS('',3,(#79221,#79222,#79223,#79224,#79225,
#79226,#79227,#79228,#79229),.UNSPECIFIED.,.F.,.F.,(4,1,1,1,1,1,4),(135.088484104361,
135.096515560027,136.09402064625,137.091525732474,138.089030818697,139.086535904921,
140.062106270563),.UNSPECIFIED.);
#1761=B_SPLINE_CURVE_WITH_KNOTS('',3,(#79234,#79235,#79236,#79237,#79238,
#79239,#79240,#79241,#79242,#79243),.UNSPECIFIED.,.F.,.F.,(4,1,1,1,1,1,
1,4),(128.805298797182,129.564589036692,130.562094122916,131.559599209139,
132.557104295363,133.554609381586,134.55211446781,135.088484104361),
 .UNSPECIFIED.);
#1762=B_SPLINE_CURVE_WITH_KNOTS('',3,(#79244,#79245,#79246,#79247,#79248,
#79249,#79250,#79251,#79252,#79253),.UNSPECIFIED.,.F.,.F.,(4,1,1,1,1,1,
1,4),(128.805298797182,129.111485042685,130.108990128909,131.106495215132,
132.104000301356,133.10150538758,134.099010473803,135.088484104361),
 .UNSPECIFIED.);
#1763=B_SPLINE_CURVE_WITH_KNOTS('',3,(#79258,#79259,#79260,#79261,#79262,
#79263,#79264,#79265,#79266,#79267,#79268),.UNSPECIFIED.,.F.,.F.,(4,1,1,
1,1,1,1,1,4),(122.522113490002,122.582053433127,123.57955851935,124.577063605574,
125.574568691798,126.572073778021,127.569578864245,128.567083950468,128.805298797182),
 .UNSPECIFIED.);
#1764=B_SPLINE_CURVE_WITH_KNOTS('',3,(#79269,#79270,#79271,#79272,#79273,
#79274,#79275,#79276,#79277,#79278),.UNSPECIFIED.,.F.,.F.,(4,1,1,1,1,1,
1,4),(122.522113490002,123.126454525344,124.123959611567,125.121464697791,
126.118969784014,127.116474870238,128.113979956462,128.805298797182),
 .UNSPECIFIED.);
#1765=B_SPLINE_CURVE_WITH_KNOTS('',3,(#79283,#79284,#79285,#79286,#79287,
#79288,#79289,#79290,#79291,#79292),.UNSPECIFIED.,.F.,.F.,(4,1,1,1,1,1,
1,4),(116.238928182822,116.597022915785,117.594528002009,118.592033088232,
119.589538174456,120.58704326068,121.584548346903,122.522113490002),
 .UNSPECIFIED.);
#1766=B_SPLINE_CURVE_WITH_KNOTS('',3,(#79293,#79294,#79295,#79296,#79297,
#79298,#79299,#79300,#79301,#79302),.UNSPECIFIED.,.F.,.F.,(4,1,1,1,1,1,
1,4),(116.238928182822,117.141424008002,118.138929094226,119.136434180449,
120.133939266673,121.131444352896,122.12894943912,122.522113490002),
 .UNSPECIFIED.);
#1767=B_SPLINE_CURVE_WITH_KNOTS('',3,(#79307,#79308,#79309,#79310,#79311,
#79312,#79313,#79314,#79315,#79316),.UNSPECIFIED.,.F.,.F.,(4,1,1,1,1,1,
1,4),(109.955742875643,110.611992398444,111.609497484667,112.607002570891,
113.604507657114,114.602012743338,115.599517829562,116.238928182822),
 .UNSPECIFIED.);
#1768=B_SPLINE_CURVE_WITH_KNOTS('',3,(#79317,#79318,#79319,#79320,#79321,
#79322,#79323,#79324,#79325,#79326,#79327),.UNSPECIFIED.,.F.,.F.,(4,1,1,
1,1,1,1,1,4),(109.955742875643,110.158888404437,111.15639349066,112.153898576884,
113.151403663108,114.148908749331,115.146413835555,116.143918921778,116.238928182822),
 .UNSPECIFIED.);
#1769=B_SPLINE_CURVE_WITH_KNOTS('',3,(#79332,#79333,#79334,#79335,#79336,
#79337,#79338,#79339,#79340,#79341),.UNSPECIFIED.,.F.,.F.,(4,1,1,1,1,1,
1,4),(103.672557568463,104.626961881102,105.624466967326,106.621972053549,
107.619477139773,108.616982225996,109.61448731222,109.955742875643),
 .UNSPECIFIED.);
#1770=B_SPLINE_CURVE_WITH_KNOTS('',3,(#79342,#79343,#79344,#79345,#79346,
#79347,#79348,#79349,#79350,#79351),.UNSPECIFIED.,.F.,.F.,(4,1,1,1,1,1,
1,4),(103.672557568463,104.173857887095,105.171362973319,106.168868059542,
107.166373145766,108.16387823199,109.161383318213,109.955742875643),
 .UNSPECIFIED.);
#1771=B_SPLINE_CURVE_WITH_KNOTS('',3,(#79356,#79357,#79358,#79359,#79360,
#79361,#79362,#79363,#79364,#79365,#79366),.UNSPECIFIED.,.F.,.F.,(4,1,1,
1,1,1,1,1,4),(97.3893722612835,97.6444262775369,98.6419313637605,99.6394364499841,
100.636941536208,101.634446622431,102.631951708655,103.629456794878,103.672557568463),
 .UNSPECIFIED.);
#1772=B_SPLINE_CURVE_WITH_KNOTS('',3,(#79367,#79368,#79369,#79370,#79371,
#79372,#79373,#79374,#79375,#79376),.UNSPECIFIED.,.F.,.F.,(4,1,1,1,1,1,
1,4),(97.3893722612836,98.1888273697537,99.1863324559773,100.183837542201,
101.181342628424,102.178847714648,103.176352800872,103.672557568463),
 .UNSPECIFIED.);
#1773=B_SPLINE_CURVE_WITH_KNOTS('',3,(#79381,#79382,#79383,#79384,#79385,
#79386,#79387,#79388,#79389,#79390),.UNSPECIFIED.,.F.,.F.,(4,1,1,1,1,1,
1,4),(91.106186954104,91.6593957601953,92.6569008464189,93.6544059326425,
94.6519110188661,95.6494161050897,96.6469211913133,97.3893722612835),
 .UNSPECIFIED.);
#1774=B_SPLINE_CURVE_WITH_KNOTS('',3,(#79391,#79392,#79393,#79394,#79395,
#79396,#79397,#79398,#79399,#79400,#79401),.UNSPECIFIED.,.F.,.F.,(4,1,1,
1,1,1,1,1,4),(91.106186954104,91.2062917661885,92.2037968524121,93.2013019386357,
94.1988070248593,95.1963121110829,96.1938171973065,97.1913222835301,97.3893722612836),
 .UNSPECIFIED.);
#1775=B_SPLINE_CURVE_WITH_KNOTS('',3,(#79406,#79407,#79408,#79409,#79410,
#79411,#79412,#79413,#79414,#79415),.UNSPECIFIED.,.F.,.F.,(4,1,1,1,1,1,
1,4),(84.8230016469244,85.6743652428537,86.6718703290773,87.6693754153009,
88.6668805015245,89.6643855877481,90.6618906739717,91.106186954104),
 .UNSPECIFIED.);
#1776=B_SPLINE_CURVE_WITH_KNOTS('',3,(#79416,#79417,#79418,#79419,#79420,
#79421,#79422,#79423,#79424,#79425),.UNSPECIFIED.,.F.,.F.,(4,1,1,1,1,1,
1,4),(84.8230016469244,85.221261248847,86.2187663350706,87.2162714212942,
88.2137765075177,89.2112815937413,90.2087866799649,91.106186954104),
 .UNSPECIFIED.);
#1777=B_SPLINE_CURVE_WITH_KNOTS('',3,(#79430,#79431,#79432,#79433,#79434,
#79435,#79436,#79437,#79438,#79439,#79440),.UNSPECIFIED.,.F.,.F.,(4,1,1,
1,1,1,1,1,4),(78.5398163397448,78.6918296392886,79.6893347255122,80.6868398117358,
81.6843448979593,82.6818499841829,83.6793550704065,84.6768601566301,84.8230016469244),
 .UNSPECIFIED.);
#1778=B_SPLINE_CURVE_WITH_KNOTS('',3,(#79441,#79442,#79443,#79444,#79445,
#79446,#79447,#79448,#79449,#79450),.UNSPECIFIED.,.F.,.F.,(4,1,1,1,1,1,
1,4),(78.5398163397448,79.2362307315054,80.233735817729,81.2312409039526,
82.2287459901762,83.2262510763998,84.2237561626234,84.8230016469244),
 .UNSPECIFIED.);
#1779=B_SPLINE_CURVE_WITH_KNOTS('',3,(#79455,#79456,#79457,#79458,#79459,
#79460,#79461,#79462,#79463,#79464),.UNSPECIFIED.,.F.,.F.,(4,1,1,1,1,1,
1,4),(72.2566310325652,72.706799121947,73.7043042081706,74.7018092943942,
75.6993143806178,76.6968194668414,77.694324553065,78.5398163397448),
 .UNSPECIFIED.);
#1780=B_SPLINE_CURVE_WITH_KNOTS('',3,(#79465,#79466,#79467,#79468,#79469,
#79470,#79471,#79472,#79473,#79474),.UNSPECIFIED.,.F.,.F.,(4,1,1,1,1,1,
1,4),(72.2566310325652,73.2512002141638,74.2487053003874,75.246210386611,
76.2437154728346,77.2412205590582,78.2387256452818,78.5398163397448),
 .UNSPECIFIED.);
#1781=B_SPLINE_CURVE_WITH_KNOTS('',3,(#79479,#79480,#79481,#79482,#79483,
#79484,#79485,#79486,#79487,#79488),.UNSPECIFIED.,.F.,.F.,(4,1,1,1,1,1,
1,4),(65.9734457253856,66.7217686046054,67.719273690829,68.7167787770526,
69.7142838632762,70.7117889494998,71.7092940357234,72.2566310325652),
 .UNSPECIFIED.);
#1782=B_SPLINE_CURVE_WITH_KNOTS('',3,(#79489,#79490,#79491,#79492,#79493,
#79494,#79495,#79496,#79497,#79498,#79499),.UNSPECIFIED.,.F.,.F.,(4,1,1,
1,1,1,1,1,4),(65.9734457253856,66.2686646105986,67.2661696968223,68.2636747830458,
69.2611798692694,70.258684955493,71.2561900417166,72.2536951279402,72.2566310325652),
 .UNSPECIFIED.);
#1783=B_SPLINE_CURVE_WITH_KNOTS('',3,(#79504,#79505,#79506,#79507,#79508,
#79509,#79510,#79511,#79512,#79513,#79514),.UNSPECIFIED.,.F.,.F.,(4,1,1,
1,1,1,1,1,4),(59.690260418206,59.7392330010403,60.7367380872638,61.7342431734874,
62.731748259711,63.7292533459346,64.7267584321582,65.7242635183818,65.9734457253856),
 .UNSPECIFIED.);
#1784=B_SPLINE_CURVE_WITH_KNOTS('',3,(#79515,#79516,#79517,#79518,#79519,
#79520,#79521,#79522,#79523,#79524),.UNSPECIFIED.,.F.,.F.,(4,1,1,1,1,1,
1,4),(59.690260418206,60.2836340932571,61.2811391794807,62.2786442657043,
63.2761493519279,64.2736544381515,65.2711595243751,65.9734457253856),
 .UNSPECIFIED.);
#1785=B_SPLINE_CURVE_WITH_KNOTS('',3,(#79529,#79530,#79531,#79532,#79533,
#79534,#79535,#79536,#79537,#79538),.UNSPECIFIED.,.F.,.F.,(4,1,1,1,1,1,
1,4),(53.4070751110264,53.7542024836987,54.7517075699223,55.7492126561459,
56.7467177423695,57.7442228285931,58.7417279148167,59.690260418206),
 .UNSPECIFIED.);
#1786=B_SPLINE_CURVE_WITH_KNOTS('',3,(#79539,#79540,#79541,#79542,#79543,
#79544,#79545,#79546,#79547,#79548),.UNSPECIFIED.,.F.,.F.,(4,1,1,1,1,1,
1,4),(53.4070751110264,54.2986035759155,55.2961086621391,56.2936137483627,
57.2911188345863,58.2886239208099,59.2861290070335,59.690260418206),
 .UNSPECIFIED.);
#1787=B_SPLINE_CURVE_WITH_KNOTS('',3,(#79553,#79554,#79555,#79556,#79557,
#79558,#79559,#79560,#79561,#79562),.UNSPECIFIED.,.F.,.F.,(4,1,1,1,1,1,
1,4),(47.1238898038468,47.7691719663571,48.7666770525807,49.7641821388043,
50.7616872250279,51.7591923112515,52.7566973974751,53.4070751110264),
 .UNSPECIFIED.);
#1788=B_SPLINE_CURVE_WITH_KNOTS('',3,(#79563,#79564,#79565,#79566,#79567,
#79568,#79569,#79570,#79571,#79572,#79573),.UNSPECIFIED.,.F.,.F.,(4,1,1,
1,1,1,1,1,4),(47.1238898038468,47.3160679723504,48.3135730585739,49.3110781447975,
50.3085832310211,51.3060883172447,52.3035934034683,53.3010984896919,53.4070751110264),
 .UNSPECIFIED.);
#1789=B_SPLINE_CURVE_WITH_KNOTS('',3,(#79578,#79579,#79580,#79581,#79582,
#79583,#79584,#79585,#79586,#79587),.UNSPECIFIED.,.F.,.F.,(4,1,1,1,1,1,
1,4),(40.8407044966672,41.7841414490155,42.7816465352391,43.7791516214627,
44.7766567076863,45.7741617939099,46.7716668801335,47.1238898038468),
 .UNSPECIFIED.);
#1790=B_SPLINE_CURVE_WITH_KNOTS('',3,(#79588,#79589,#79590,#79591,#79592,
#79593,#79594,#79595,#79596,#79597),.UNSPECIFIED.,.F.,.F.,(4,1,1,1,1,1,
1,4),(40.8407044966673,41.3310374550088,42.3285425412324,43.326047627456,
44.3235527136796,45.3210577999032,46.3185628861268,47.1238898038468),
 .UNSPECIFIED.);
#1791=B_SPLINE_CURVE_WITH_KNOTS('',3,(#79602,#79603,#79604,#79605,#79606,
#79607,#79608,#79609,#79610,#79611,#79612),.UNSPECIFIED.,.F.,.F.,(4,1,1,
1,1,1,1,1,4),(34.5575191894876,34.8016058454504,35.799110931674,36.7966160178976,
37.7941211041212,38.7916261903448,39.7891312765683,40.7866363627919,40.8407044966672),
 .UNSPECIFIED.);
#1792=B_SPLINE_CURVE_WITH_KNOTS('',3,(#79613,#79614,#79615,#79616,#79617,
#79618,#79619,#79620,#79621,#79622),.UNSPECIFIED.,.F.,.F.,(4,1,1,1,1,1,
1,4),(34.5575191894877,35.3460069376672,36.3435120238908,37.3410171101144,
38.338522196338,39.3360272825616,40.3335323687852,40.8407044966673),
 .UNSPECIFIED.);
#1793=B_SPLINE_CURVE_WITH_KNOTS('',3,(#79627,#79628,#79629,#79630,#79631,
#79632,#79633,#79634,#79635,#79636),.UNSPECIFIED.,.F.,.F.,(4,1,1,1,1,1,
1,4),(28.2743338823081,28.8165753281088,29.8140804143324,30.811585500556,
31.8090905867796,32.8065956730032,33.8041007592268,34.5575191894876),
 .UNSPECIFIED.);
#1794=B_SPLINE_CURVE_WITH_KNOTS('',3,(#79637,#79638,#79639,#79640,#79641,
#79642,#79643,#79644,#79645,#79646,#79647),.UNSPECIFIED.,.F.,.F.,(4,1,1,
1,1,1,1,1,4),(28.2743338823081,28.363471334102,29.3609764203256,30.3584815065492,
31.3559865927728,32.3534916789964,33.35099676522,34.3485018514436,34.5575191894877),
 .UNSPECIFIED.);
#1795=B_SPLINE_CURVE_WITH_KNOTS('',3,(#79652,#79653,#79654,#79655,#79656,
#79657,#79658,#79659,#79660,#79661),.UNSPECIFIED.,.F.,.F.,(4,1,1,1,1,1,
1,4),(21.9911485751285,22.8315448107672,23.8290498969908,24.8265549832144,
25.824060069438,26.8215651556616,27.8190702418852,28.2743338823081),
 .UNSPECIFIED.);
#1796=B_SPLINE_CURVE_WITH_KNOTS('',3,(#79662,#79663,#79664,#79665,#79666,
#79667,#79668,#79669,#79670,#79671),.UNSPECIFIED.,.F.,.F.,(4,1,1,1,1,1,
1,4),(21.9911485751285,22.3784408167605,23.3759459029841,24.3734509892077,
25.3709560754313,26.3684611616549,27.3659662478785,28.2743338823081),
 .UNSPECIFIED.);
#1797=B_SPLINE_CURVE_WITH_KNOTS('',3,(#79677,#79678,#79679,#79680,#79681),
 .UNSPECIFIED.,.F.,.F.,(4,1,4),(14.3984001269717,15.3959052131953,15.7079632679489),
 .UNSPECIFIED.);
#1798=B_SPLINE_CURVE_WITH_KNOTS('',3,(#79684,#79685,#79686,#79687,#79688),
 .UNSPECIFIED.,.F.,.F.,(4,1,4),(13.8759337553361,14.8515041209785,15.7079632679489),
 .UNSPECIFIED.);
#1799=B_SPLINE_CURVE_WITH_KNOTS('',3,(#79694,#79695,#79696,#79697,#79698,
#79699,#79700,#79701),.UNSPECIFIED.,.F.,.F.,(4,1,1,1,1,4),(135.088484104361,
135.549619554034,136.547124640257,137.544629726481,138.542134812704,139.539639898928),
 .UNSPECIFIED.);
#1800=B_SPLINE_CURVE_WITH_KNOTS('',3,(#79704,#79705,#79706,#79707,#79708,
#79709,#79710,#79711,#79712),.UNSPECIFIED.,.F.,.F.,(4,1,1,1,1,1,4),(135.088484104361,
135.096515560027,136.09402064625,137.091525732474,138.089030818698,139.086535904921,
140.062106270563),.UNSPECIFIED.);
#1801=B_SPLINE_CURVE_WITH_KNOTS('',3,(#79717,#79718,#79719,#79720,#79721,
#79722,#79723,#79724,#79725,#79726),.UNSPECIFIED.,.F.,.F.,(4,1,1,1,1,1,
1,4),(128.805298797182,129.564589036692,130.562094122916,131.559599209139,
132.557104295363,133.554609381586,134.55211446781,135.088484104361),
 .UNSPECIFIED.);
#1802=B_SPLINE_CURVE_WITH_KNOTS('',3,(#79727,#79728,#79729,#79730,#79731,
#79732,#79733,#79734,#79735,#79736),.UNSPECIFIED.,.F.,.F.,(4,1,1,1,1,1,
1,4),(128.805298797182,129.111485042685,130.108990128909,131.106495215132,
132.104000301356,133.10150538758,134.099010473803,135.088484104361),
 .UNSPECIFIED.);
#1803=B_SPLINE_CURVE_WITH_KNOTS('',3,(#79741,#79742,#79743,#79744,#79745,
#79746,#79747,#79748,#79749,#79750,#79751),.UNSPECIFIED.,.F.,.F.,(4,1,1,
1,1,1,1,1,4),(122.522113490002,122.582053433127,123.57955851935,124.577063605574,
125.574568691798,126.572073778021,127.569578864245,128.567083950468,128.805298797182),
 .UNSPECIFIED.);
#1804=B_SPLINE_CURVE_WITH_KNOTS('',3,(#79752,#79753,#79754,#79755,#79756,
#79757,#79758,#79759,#79760,#79761),.UNSPECIFIED.,.F.,.F.,(4,1,1,1,1,1,
1,4),(122.522113490002,123.126454525344,124.123959611567,125.121464697791,
126.118969784014,127.116474870238,128.113979956462,128.805298797182),
 .UNSPECIFIED.);
#1805=B_SPLINE_CURVE_WITH_KNOTS('',3,(#79766,#79767,#79768,#79769,#79770,
#79771,#79772,#79773,#79774,#79775),.UNSPECIFIED.,.F.,.F.,(4,1,1,1,1,1,
1,4),(116.238928182822,116.597022915785,117.594528002009,118.592033088232,
119.589538174456,120.58704326068,121.584548346903,122.522113490002),
 .UNSPECIFIED.);
#1806=B_SPLINE_CURVE_WITH_KNOTS('',3,(#79776,#79777,#79778,#79779,#79780,
#79781,#79782,#79783,#79784,#79785),.UNSPECIFIED.,.F.,.F.,(4,1,1,1,1,1,
1,4),(116.238928182822,117.141424008002,118.138929094226,119.136434180449,
120.133939266673,121.131444352896,122.12894943912,122.522113490002),
 .UNSPECIFIED.);
#1807=B_SPLINE_CURVE_WITH_KNOTS('',3,(#79790,#79791,#79792,#79793,#79794,
#79795,#79796,#79797,#79798,#79799),.UNSPECIFIED.,.F.,.F.,(4,1,1,1,1,1,
1,4),(109.955742875643,110.611992398444,111.609497484667,112.607002570891,
113.604507657114,114.602012743338,115.599517829562,116.238928182822),
 .UNSPECIFIED.);
#1808=B_SPLINE_CURVE_WITH_KNOTS('',3,(#79800,#79801,#79802,#79803,#79804,
#79805,#79806,#79807,#79808,#79809,#79810),.UNSPECIFIED.,.F.,.F.,(4,1,1,
1,1,1,1,1,4),(109.955742875643,110.158888404437,111.15639349066,112.153898576884,
113.151403663108,114.148908749331,115.146413835555,116.143918921778,116.238928182822),
 .UNSPECIFIED.);
#1809=B_SPLINE_CURVE_WITH_KNOTS('',3,(#79815,#79816,#79817,#79818,#79819,
#79820,#79821,#79822,#79823,#79824),.UNSPECIFIED.,.F.,.F.,(4,1,1,1,1,1,
1,4),(103.672557568463,104.626961881102,105.624466967326,106.621972053549,
107.619477139773,108.616982225996,109.61448731222,109.955742875643),
 .UNSPECIFIED.);
#1810=B_SPLINE_CURVE_WITH_KNOTS('',3,(#79825,#79826,#79827,#79828,#79829,
#79830,#79831,#79832,#79833,#79834),.UNSPECIFIED.,.F.,.F.,(4,1,1,1,1,1,
1,4),(103.672557568463,104.173857887095,105.171362973319,106.168868059543,
107.166373145766,108.16387823199,109.161383318213,109.955742875643),
 .UNSPECIFIED.);
#1811=B_SPLINE_CURVE_WITH_KNOTS('',3,(#79839,#79840,#79841,#79842,#79843,
#79844,#79845,#79846,#79847,#79848,#79849),.UNSPECIFIED.,.F.,.F.,(4,1,1,
1,1,1,1,1,4),(97.3893722612836,97.6444262775369,98.6419313637605,99.6394364499841,
100.636941536208,101.634446622431,102.631951708655,103.629456794878,103.672557568463),
 .UNSPECIFIED.);
#1812=B_SPLINE_CURVE_WITH_KNOTS('',3,(#79850,#79851,#79852,#79853,#79854,
#79855,#79856,#79857,#79858,#79859),.UNSPECIFIED.,.F.,.F.,(4,1,1,1,1,1,
1,4),(97.3893722612836,98.1888273697538,99.1863324559774,100.183837542201,
101.181342628425,102.178847714648,103.176352800872,103.672557568463),
 .UNSPECIFIED.);
#1813=B_SPLINE_CURVE_WITH_KNOTS('',3,(#79864,#79865,#79866,#79867,#79868,
#79869,#79870,#79871,#79872,#79873),.UNSPECIFIED.,.F.,.F.,(4,1,1,1,1,1,
1,4),(91.106186954104,91.6593957601953,92.6569008464189,93.6544059326425,
94.6519110188661,95.6494161050897,96.6469211913133,97.3893722612836),
 .UNSPECIFIED.);
#1814=B_SPLINE_CURVE_WITH_KNOTS('',3,(#79874,#79875,#79876,#79877,#79878,
#79879,#79880,#79881,#79882,#79883,#79884),.UNSPECIFIED.,.F.,.F.,(4,1,1,
1,1,1,1,1,4),(91.106186954104,91.2062917661886,92.2037968524122,93.2013019386358,
94.1988070248594,95.196312111083,96.1938171973066,97.1913222835302,97.3893722612836),
 .UNSPECIFIED.);
#1815=B_SPLINE_CURVE_WITH_KNOTS('',3,(#79889,#79890,#79891,#79892,#79893,
#79894,#79895,#79896,#79897,#79898),.UNSPECIFIED.,.F.,.F.,(4,1,1,1,1,1,
1,4),(84.8230016469244,85.6743652428538,86.6718703290774,87.669375415301,
88.6668805015246,89.6643855877482,90.6618906739717,91.106186954104),
 .UNSPECIFIED.);
#1816=B_SPLINE_CURVE_WITH_KNOTS('',3,(#79899,#79900,#79901,#79902,#79903,
#79904,#79905,#79906,#79907,#79908),.UNSPECIFIED.,.F.,.F.,(4,1,1,1,1,1,
1,4),(84.8230016469244,85.221261248847,86.2187663350706,87.2162714212942,
88.2137765075178,89.2112815937414,90.208786679965,91.106186954104),
 .UNSPECIFIED.);
#1817=B_SPLINE_CURVE_WITH_KNOTS('',3,(#79913,#79914,#79915,#79916,#79917,
#79918,#79919,#79920,#79921,#79922,#79923),.UNSPECIFIED.,.F.,.F.,(4,1,1,
1,1,1,1,1,4),(78.5398163397448,78.6918296392886,79.6893347255122,80.6868398117358,
81.6843448979594,82.681849984183,83.6793550704066,84.6768601566302,84.8230016469244),
 .UNSPECIFIED.);
#1818=B_SPLINE_CURVE_WITH_KNOTS('',3,(#79924,#79925,#79926,#79927,#79928,
#79929,#79930,#79931,#79932,#79933),.UNSPECIFIED.,.F.,.F.,(4,1,1,1,1,1,
1,4),(78.5398163397448,79.2362307315055,80.233735817729,81.2312409039526,
82.2287459901762,83.2262510763998,84.2237561626234,84.8230016469244),
 .UNSPECIFIED.);
#1819=B_SPLINE_CURVE_WITH_KNOTS('',3,(#79938,#79939,#79940,#79941,#79942,
#79943,#79944,#79945,#79946,#79947),.UNSPECIFIED.,.F.,.F.,(4,1,1,1,1,1,
1,4),(72.2566310325652,72.706799121947,73.7043042081706,74.7018092943942,
75.6993143806178,76.6968194668414,77.694324553065,78.5398163397448),
 .UNSPECIFIED.);
#1820=B_SPLINE_CURVE_WITH_KNOTS('',3,(#79948,#79949,#79950,#79951,#79952,
#79953,#79954,#79955,#79956,#79957),.UNSPECIFIED.,.F.,.F.,(4,1,1,1,1,1,
1,4),(72.2566310325652,73.2512002141639,74.2487053003875,75.2462103866111,
76.2437154728347,77.2412205590583,78.2387256452818,78.5398163397448),
 .UNSPECIFIED.);
#1821=B_SPLINE_CURVE_WITH_KNOTS('',3,(#79962,#79963,#79964,#79965,#79966,
#79967,#79968,#79969,#79970,#79971),.UNSPECIFIED.,.F.,.F.,(4,1,1,1,1,1,
1,4),(65.9734457253856,66.7217686046055,67.7192736908291,68.7167787770527,
69.7142838632763,70.7117889494998,71.7092940357234,72.2566310325652),
 .UNSPECIFIED.);
#1822=B_SPLINE_CURVE_WITH_KNOTS('',3,(#79972,#79973,#79974,#79975,#79976,
#79977,#79978,#79979,#79980,#79981,#79982),.UNSPECIFIED.,.F.,.F.,(4,1,1,
1,1,1,1,1,4),(65.9734457253856,66.2686646105987,67.2661696968223,68.2636747830459,
69.2611798692695,70.2586849554931,71.2561900417167,72.2536951279403,72.2566310325652),
 .UNSPECIFIED.);
#1823=B_SPLINE_CURVE_WITH_KNOTS('',3,(#79987,#79988,#79989,#79990,#79991,
#79992,#79993,#79994,#79995,#79996,#79997),.UNSPECIFIED.,.F.,.F.,(4,1,1,
1,1,1,1,1,4),(59.690260418206,59.7392330010403,60.7367380872639,61.7342431734875,
62.7317482597111,63.7292533459347,64.7267584321583,65.7242635183819,65.9734457253856),
 .UNSPECIFIED.);
#1824=B_SPLINE_CURVE_WITH_KNOTS('',3,(#79998,#79999,#80000,#80001,#80002,
#80003,#80004,#80005,#80006,#80007),.UNSPECIFIED.,.F.,.F.,(4,1,1,1,1,1,
1,4),(59.690260418206,60.2836340932571,61.2811391794807,62.2786442657043,
63.2761493519279,64.2736544381515,65.2711595243751,65.9734457253856),
 .UNSPECIFIED.);
#1825=B_SPLINE_CURVE_WITH_KNOTS('',3,(#80012,#80013,#80014,#80015,#80016,
#80017,#80018,#80019,#80020,#80021),.UNSPECIFIED.,.F.,.F.,(4,1,1,1,1,1,
1,4),(53.4070751110264,53.7542024836987,54.7517075699223,55.7492126561459,
56.7467177423695,57.7442228285931,58.7417279148167,59.690260418206),
 .UNSPECIFIED.);
#1826=B_SPLINE_CURVE_WITH_KNOTS('',3,(#80022,#80023,#80024,#80025,#80026,
#80027,#80028,#80029,#80030,#80031),.UNSPECIFIED.,.F.,.F.,(4,1,1,1,1,1,
1,4),(53.4070751110264,54.2986035759156,55.2961086621392,56.2936137483628,
57.2911188345864,58.28862392081,59.2861290070336,59.690260418206),
 .UNSPECIFIED.);
#1827=B_SPLINE_CURVE_WITH_KNOTS('',3,(#80036,#80037,#80038,#80039,#80040,
#80041,#80042,#80043,#80044,#80045),.UNSPECIFIED.,.F.,.F.,(4,1,1,1,1,1,
1,4),(47.1238898038468,47.7691719663572,48.7666770525807,49.7641821388043,
50.7616872250279,51.7591923112515,52.7566973974751,53.4070751110264),
 .UNSPECIFIED.);
#1828=B_SPLINE_CURVE_WITH_KNOTS('',3,(#80046,#80047,#80048,#80049,#80050,
#80051,#80052,#80053,#80054,#80055,#80056),.UNSPECIFIED.,.F.,.F.,(4,1,1,
1,1,1,1,1,4),(47.1238898038468,47.3160679723504,48.313573058574,49.3110781447976,
50.3085832310212,51.3060883172448,52.3035934034684,53.301098489692,53.4070751110264),
 .UNSPECIFIED.);
#1829=B_SPLINE_CURVE_WITH_KNOTS('',3,(#80061,#80062,#80063,#80064,#80065,
#80066,#80067,#80068,#80069,#80070),.UNSPECIFIED.,.F.,.F.,(4,1,1,1,1,1,
1,4),(40.8407044966673,41.7841414490156,42.7816465352392,43.7791516214628,
44.7766567076864,45.77416179391,46.7716668801336,47.1238898038468),
 .UNSPECIFIED.);
#1830=B_SPLINE_CURVE_WITH_KNOTS('',3,(#80071,#80072,#80073,#80074,#80075,
#80076,#80077,#80078,#80079,#80080),.UNSPECIFIED.,.F.,.F.,(4,1,1,1,1,1,
1,4),(40.8407044966673,41.3310374550088,42.3285425412324,43.326047627456,
44.3235527136796,45.3210577999032,46.3185628861268,47.1238898038468),
 .UNSPECIFIED.);
#1831=B_SPLINE_CURVE_WITH_KNOTS('',3,(#80085,#80086,#80087,#80088,#80089,
#80090,#80091,#80092,#80093,#80094,#80095),.UNSPECIFIED.,.F.,.F.,(4,1,1,
1,1,1,1,1,4),(34.5575191894877,34.8016058454504,35.799110931674,36.7966160178976,
37.7941211041212,38.7916261903448,39.7891312765684,40.786636362792,40.8407044966673),
 .UNSPECIFIED.);
#1832=B_SPLINE_CURVE_WITH_KNOTS('',3,(#80096,#80097,#80098,#80099,#80100,
#80101,#80102,#80103,#80104,#80105),.UNSPECIFIED.,.F.,.F.,(4,1,1,1,1,1,
1,4),(34.5575191894877,35.3460069376673,36.3435120238909,37.3410171101145,
38.3385221963381,39.3360272825616,40.3335323687852,40.8407044966673),
 .UNSPECIFIED.);
#1833=B_SPLINE_CURVE_WITH_KNOTS('',3,(#80110,#80111,#80112,#80113,#80114,
#80115,#80116,#80117,#80118,#80119),.UNSPECIFIED.,.F.,.F.,(4,1,1,1,1,1,
1,4),(28.2743338823081,28.8165753281089,29.8140804143324,30.811585500556,
31.8090905867796,32.8065956730032,33.8041007592268,34.5575191894877),
 .UNSPECIFIED.);
#1834=B_SPLINE_CURVE_WITH_KNOTS('',3,(#80120,#80121,#80122,#80123,#80124,
#80125,#80126,#80127,#80128,#80129,#80130),.UNSPECIFIED.,.F.,.F.,(4,1,1,
1,1,1,1,1,4),(28.2743338823081,28.3634713341021,29.3609764203257,30.3584815065493,
31.3559865927729,32.3534916789965,33.3509967652201,34.3485018514437,34.5575191894877),
 .UNSPECIFIED.);
#1835=B_SPLINE_CURVE_WITH_KNOTS('',3,(#80135,#80136,#80137,#80138,#80139,
#80140,#80141,#80142,#80143,#80144),.UNSPECIFIED.,.F.,.F.,(4,1,1,1,1,1,
1,4),(21.9911485751285,22.8315448107673,23.8290498969909,24.8265549832145,
25.8240600694381,26.8215651556617,27.8190702418853,28.2743338823081),
 .UNSPECIFIED.);
#1836=B_SPLINE_CURVE_WITH_KNOTS('',3,(#80145,#80146,#80147,#80148,#80149,
#80150,#80151,#80152,#80153,#80154),.UNSPECIFIED.,.F.,.F.,(4,1,1,1,1,1,
1,4),(21.9911485751285,22.3784408167605,23.3759459029841,24.3734509892077,
25.3709560754313,26.3684611616549,27.3659662478785,28.2743338823081),
 .UNSPECIFIED.);
#1837=B_SPLINE_CURVE_WITH_KNOTS('',3,(#80160,#80161,#80162,#80163,#80164),
 .UNSPECIFIED.,.F.,.F.,(4,1,4),(14.3984001269718,15.3959052131954,15.7079632679489),
 .UNSPECIFIED.);
#1838=B_SPLINE_CURVE_WITH_KNOTS('',3,(#80167,#80168,#80169,#80170,#80171),
 .UNSPECIFIED.,.F.,.F.,(4,1,4),(13.8759337553362,14.8515041209785,15.7079632679489),
 .UNSPECIFIED.);
#1839=B_SPLINE_CURVE_WITH_KNOTS('',3,(#80177,#80178,#80179,#80180,#80181,
#80182,#80183,#80184),.UNSPECIFIED.,.F.,.F.,(4,1,1,1,1,4),(135.088484104361,
135.549619554034,136.547124640257,137.544629726481,138.542134812704,139.539639898928),
 .UNSPECIFIED.);
#1840=B_SPLINE_CURVE_WITH_KNOTS('',3,(#80187,#80188,#80189,#80190,#80191,
#80192,#80193,#80194,#80195),.UNSPECIFIED.,.F.,.F.,(4,1,1,1,1,1,4),(135.088484104361,
135.096515560027,136.09402064625,137.091525732474,138.089030818698,139.086535904921,
140.062106270563),.UNSPECIFIED.);
#1841=B_SPLINE_CURVE_WITH_KNOTS('',3,(#80200,#80201,#80202,#80203,#80204,
#80205,#80206,#80207,#80208,#80209),.UNSPECIFIED.,.F.,.F.,(4,1,1,1,1,1,
1,4),(128.805298797182,129.564589036692,130.562094122916,131.559599209139,
132.557104295363,133.554609381586,134.55211446781,135.088484104361),
 .UNSPECIFIED.);
#1842=B_SPLINE_CURVE_WITH_KNOTS('',3,(#80210,#80211,#80212,#80213,#80214,
#80215,#80216,#80217,#80218,#80219),.UNSPECIFIED.,.F.,.F.,(4,1,1,1,1,1,
1,4),(128.805298797182,129.111485042685,130.108990128909,131.106495215132,
132.104000301356,133.10150538758,134.099010473803,135.088484104361),
 .UNSPECIFIED.);
#1843=B_SPLINE_CURVE_WITH_KNOTS('',3,(#80224,#80225,#80226,#80227,#80228,
#80229,#80230,#80231,#80232,#80233,#80234),.UNSPECIFIED.,.F.,.F.,(4,1,1,
1,1,1,1,1,4),(122.522113490002,122.582053433127,123.57955851935,124.577063605574,
125.574568691798,126.572073778021,127.569578864245,128.567083950468,128.805298797182),
 .UNSPECIFIED.);
#1844=B_SPLINE_CURVE_WITH_KNOTS('',3,(#80235,#80236,#80237,#80238,#80239,
#80240,#80241,#80242,#80243,#80244),.UNSPECIFIED.,.F.,.F.,(4,1,1,1,1,1,
1,4),(122.522113490002,123.126454525344,124.123959611567,125.121464697791,
126.118969784014,127.116474870238,128.113979956462,128.805298797182),
 .UNSPECIFIED.);
#1845=B_SPLINE_CURVE_WITH_KNOTS('',3,(#80249,#80250,#80251,#80252,#80253,
#80254,#80255,#80256,#80257,#80258),.UNSPECIFIED.,.F.,.F.,(4,1,1,1,1,1,
1,4),(116.238928182822,116.597022915785,117.594528002009,118.592033088232,
119.589538174456,120.58704326068,121.584548346903,122.522113490002),
 .UNSPECIFIED.);
#1846=B_SPLINE_CURVE_WITH_KNOTS('',3,(#80259,#80260,#80261,#80262,#80263,
#80264,#80265,#80266,#80267,#80268),.UNSPECIFIED.,.F.,.F.,(4,1,1,1,1,1,
1,4),(116.238928182822,117.141424008002,118.138929094226,119.136434180449,
120.133939266673,121.131444352896,122.12894943912,122.522113490002),
 .UNSPECIFIED.);
#1847=B_SPLINE_CURVE_WITH_KNOTS('',3,(#80273,#80274,#80275,#80276,#80277,
#80278,#80279,#80280,#80281,#80282),.UNSPECIFIED.,.F.,.F.,(4,1,1,1,1,1,
1,4),(109.955742875643,110.611992398444,111.609497484667,112.607002570891,
113.604507657114,114.602012743338,115.599517829562,116.238928182822),
 .UNSPECIFIED.);
#1848=B_SPLINE_CURVE_WITH_KNOTS('',3,(#80283,#80284,#80285,#80286,#80287,
#80288,#80289,#80290,#80291,#80292,#80293),.UNSPECIFIED.,.F.,.F.,(4,1,1,
1,1,1,1,1,4),(109.955742875643,110.158888404437,111.15639349066,112.153898576884,
113.151403663108,114.148908749331,115.146413835555,116.143918921778,116.238928182822),
 .UNSPECIFIED.);
#1849=B_SPLINE_CURVE_WITH_KNOTS('',3,(#80298,#80299,#80300,#80301,#80302,
#80303,#80304,#80305,#80306,#80307),.UNSPECIFIED.,.F.,.F.,(4,1,1,1,1,1,
1,4),(103.672557568463,104.626961881102,105.624466967326,106.621972053549,
107.619477139773,108.616982225996,109.61448731222,109.955742875643),
 .UNSPECIFIED.);
#1850=B_SPLINE_CURVE_WITH_KNOTS('',3,(#80308,#80309,#80310,#80311,#80312,
#80313,#80314,#80315,#80316,#80317),.UNSPECIFIED.,.F.,.F.,(4,1,1,1,1,1,
1,4),(103.672557568463,104.173857887095,105.171362973319,106.168868059543,
107.166373145766,108.16387823199,109.161383318213,109.955742875643),
 .UNSPECIFIED.);
#1851=B_SPLINE_CURVE_WITH_KNOTS('',3,(#80322,#80323,#80324,#80325,#80326,
#80327,#80328,#80329,#80330,#80331,#80332),.UNSPECIFIED.,.F.,.F.,(4,1,1,
1,1,1,1,1,4),(97.3893722612835,97.6444262775369,98.6419313637605,99.6394364499841,
100.636941536208,101.634446622431,102.631951708655,103.629456794878,103.672557568463),
 .UNSPECIFIED.);
#1852=B_SPLINE_CURVE_WITH_KNOTS('',3,(#80333,#80334,#80335,#80336,#80337,
#80338,#80339,#80340,#80341,#80342),.UNSPECIFIED.,.F.,.F.,(4,1,1,1,1,1,
1,4),(97.3893722612836,98.1888273697538,99.1863324559774,100.183837542201,
101.181342628425,102.178847714648,103.176352800872,103.672557568463),
 .UNSPECIFIED.);
#1853=B_SPLINE_CURVE_WITH_KNOTS('',3,(#80347,#80348,#80349,#80350,#80351,
#80352,#80353,#80354,#80355,#80356),.UNSPECIFIED.,.F.,.F.,(4,1,1,1,1,1,
1,4),(91.106186954104,91.6593957601954,92.6569008464189,93.6544059326425,
94.6519110188661,95.6494161050897,96.6469211913133,97.3893722612835),
 .UNSPECIFIED.);
#1854=B_SPLINE_CURVE_WITH_KNOTS('',3,(#80357,#80358,#80359,#80360,#80361,
#80362,#80363,#80364,#80365,#80366,#80367),.UNSPECIFIED.,.F.,.F.,(4,1,1,
1,1,1,1,1,4),(91.106186954104,91.2062917661886,92.2037968524122,93.2013019386358,
94.1988070248594,95.196312111083,96.1938171973066,97.1913222835302,97.3893722612836),
 .UNSPECIFIED.);
#1855=B_SPLINE_CURVE_WITH_KNOTS('',3,(#80372,#80373,#80374,#80375,#80376,
#80377,#80378,#80379,#80380,#80381),.UNSPECIFIED.,.F.,.F.,(4,1,1,1,1,1,
1,4),(84.8230016469244,85.6743652428538,86.6718703290774,87.669375415301,
88.6668805015246,89.6643855877482,90.6618906739718,91.106186954104),
 .UNSPECIFIED.);
#1856=B_SPLINE_CURVE_WITH_KNOTS('',3,(#80382,#80383,#80384,#80385,#80386,
#80387,#80388,#80389,#80390,#80391),.UNSPECIFIED.,.F.,.F.,(4,1,1,1,1,1,
1,4),(84.8230016469244,85.221261248847,86.2187663350706,87.2162714212942,
88.2137765075178,89.2112815937414,90.208786679965,91.106186954104),
 .UNSPECIFIED.);
#1857=B_SPLINE_CURVE_WITH_KNOTS('',3,(#80396,#80397,#80398,#80399,#80400,
#80401,#80402,#80403,#80404,#80405,#80406),.UNSPECIFIED.,.F.,.F.,(4,1,1,
1,1,1,1,1,4),(78.5398163397448,78.6918296392886,79.6893347255122,80.6868398117358,
81.6843448979594,82.681849984183,83.6793550704066,84.6768601566302,84.8230016469244),
 .UNSPECIFIED.);
#1858=B_SPLINE_CURVE_WITH_KNOTS('',3,(#80407,#80408,#80409,#80410,#80411,
#80412,#80413,#80414,#80415,#80416),.UNSPECIFIED.,.F.,.F.,(4,1,1,1,1,1,
1,4),(78.5398163397448,79.2362307315055,80.2337358177291,81.2312409039526,
82.2287459901762,83.2262510763998,84.2237561626234,84.8230016469244),
 .UNSPECIFIED.);
#1859=B_SPLINE_CURVE_WITH_KNOTS('',3,(#80421,#80422,#80423,#80424,#80425,
#80426,#80427,#80428,#80429,#80430),.UNSPECIFIED.,.F.,.F.,(4,1,1,1,1,1,
1,4),(72.2566310325652,72.706799121947,73.7043042081706,74.7018092943942,
75.6993143806178,76.6968194668414,77.694324553065,78.5398163397448),
 .UNSPECIFIED.);
#1860=B_SPLINE_CURVE_WITH_KNOTS('',3,(#80431,#80432,#80433,#80434,#80435,
#80436,#80437,#80438,#80439,#80440),.UNSPECIFIED.,.F.,.F.,(4,1,1,1,1,1,
1,4),(72.2566310325652,73.2512002141639,74.2487053003875,75.2462103866111,
76.2437154728347,77.2412205590583,78.2387256452819,78.5398163397448),
 .UNSPECIFIED.);
#1861=B_SPLINE_CURVE_WITH_KNOTS('',3,(#80445,#80446,#80447,#80448,#80449,
#80450,#80451,#80452,#80453,#80454),.UNSPECIFIED.,.F.,.F.,(4,1,1,1,1,1,
1,4),(65.9734457253856,66.7217686046055,67.7192736908291,68.7167787770527,
69.7142838632763,70.7117889494998,71.7092940357234,72.2566310325652),
 .UNSPECIFIED.);
#1862=B_SPLINE_CURVE_WITH_KNOTS('',3,(#80455,#80456,#80457,#80458,#80459,
#80460,#80461,#80462,#80463,#80464,#80465),.UNSPECIFIED.,.F.,.F.,(4,1,1,
1,1,1,1,1,4),(65.9734457253856,66.2686646105987,67.2661696968223,68.2636747830459,
69.2611798692695,70.2586849554931,71.2561900417167,72.2536951279403,72.2566310325652),
 .UNSPECIFIED.);
#1863=B_SPLINE_CURVE_WITH_KNOTS('',3,(#80470,#80471,#80472,#80473,#80474,
#80475,#80476,#80477,#80478,#80479,#80480),.UNSPECIFIED.,.F.,.F.,(4,1,1,
1,1,1,1,1,4),(59.690260418206,59.7392330010403,60.7367380872639,61.7342431734875,
62.7317482597111,63.7292533459347,64.7267584321583,65.7242635183819,65.9734457253856),
 .UNSPECIFIED.);
#1864=B_SPLINE_CURVE_WITH_KNOTS('',3,(#80481,#80482,#80483,#80484,#80485,
#80486,#80487,#80488,#80489,#80490),.UNSPECIFIED.,.F.,.F.,(4,1,1,1,1,1,
1,4),(59.690260418206,60.2836340932571,61.2811391794807,62.2786442657043,
63.2761493519279,64.2736544381515,65.2711595243751,65.9734457253856),
 .UNSPECIFIED.);
#1865=B_SPLINE_CURVE_WITH_KNOTS('',3,(#80495,#80496,#80497,#80498,#80499,
#80500,#80501,#80502,#80503,#80504),.UNSPECIFIED.,.F.,.F.,(4,1,1,1,1,1,
1,4),(53.4070751110264,53.7542024836987,54.7517075699223,55.7492126561459,
56.7467177423695,57.7442228285931,58.7417279148167,59.690260418206),
 .UNSPECIFIED.);
#1866=B_SPLINE_CURVE_WITH_KNOTS('',3,(#80505,#80506,#80507,#80508,#80509,
#80510,#80511,#80512,#80513,#80514),.UNSPECIFIED.,.F.,.F.,(4,1,1,1,1,1,
1,4),(53.4070751110264,54.2986035759156,55.2961086621392,56.2936137483628,
57.2911188345864,58.28862392081,59.2861290070336,59.690260418206),
 .UNSPECIFIED.);
#1867=B_SPLINE_CURVE_WITH_KNOTS('',3,(#80519,#80520,#80521,#80522,#80523,
#80524,#80525,#80526,#80527,#80528),.UNSPECIFIED.,.F.,.F.,(4,1,1,1,1,1,
1,4),(47.1238898038468,47.7691719663572,48.7666770525808,49.7641821388044,
50.7616872250279,51.7591923112515,52.7566973974751,53.4070751110264),
 .UNSPECIFIED.);
#1868=B_SPLINE_CURVE_WITH_KNOTS('',3,(#80529,#80530,#80531,#80532,#80533,
#80534,#80535,#80536,#80537,#80538,#80539),.UNSPECIFIED.,.F.,.F.,(4,1,1,
1,1,1,1,1,4),(47.1238898038468,47.3160679723504,48.313573058574,49.3110781447976,
50.3085832310212,51.3060883172448,52.3035934034684,53.301098489692,53.4070751110264),
 .UNSPECIFIED.);
#1869=B_SPLINE_CURVE_WITH_KNOTS('',3,(#80544,#80545,#80546,#80547,#80548,
#80549,#80550,#80551,#80552,#80553),.UNSPECIFIED.,.F.,.F.,(4,1,1,1,1,1,
1,4),(40.8407044966672,41.7841414490156,42.7816465352392,43.7791516214628,
44.7766567076864,45.77416179391,46.7716668801336,47.1238898038468),
 .UNSPECIFIED.);
#1870=B_SPLINE_CURVE_WITH_KNOTS('',3,(#80554,#80555,#80556,#80557,#80558,
#80559,#80560,#80561,#80562,#80563),.UNSPECIFIED.,.F.,.F.,(4,1,1,1,1,1,
1,4),(40.8407044966673,41.3310374550088,42.3285425412324,43.326047627456,
44.3235527136796,45.3210577999032,46.3185628861268,47.1238898038468),
 .UNSPECIFIED.);
#1871=B_SPLINE_CURVE_WITH_KNOTS('',3,(#80568,#80569,#80570,#80571,#80572,
#80573,#80574,#80575,#80576,#80577,#80578),.UNSPECIFIED.,.F.,.F.,(4,1,1,
1,1,1,1,1,4),(34.5575191894876,34.8016058454504,35.799110931674,36.7966160178976,
37.7941211041212,38.7916261903448,39.7891312765684,40.786636362792,40.8407044966672),
 .UNSPECIFIED.);
#1872=B_SPLINE_CURVE_WITH_KNOTS('',3,(#80579,#80580,#80581,#80582,#80583,
#80584,#80585,#80586,#80587,#80588),.UNSPECIFIED.,.F.,.F.,(4,1,1,1,1,1,
1,4),(34.5575191894877,35.3460069376673,36.3435120238909,37.3410171101145,
38.3385221963381,39.3360272825617,40.3335323687852,40.8407044966673),
 .UNSPECIFIED.);
#1873=B_SPLINE_CURVE_WITH_KNOTS('',3,(#80593,#80594,#80595,#80596,#80597,
#80598,#80599,#80600,#80601,#80602),.UNSPECIFIED.,.F.,.F.,(4,1,1,1,1,1,
1,4),(28.2743338823081,28.8165753281089,29.8140804143324,30.811585500556,
31.8090905867796,32.8065956730032,33.8041007592268,34.5575191894876),
 .UNSPECIFIED.);
#1874=B_SPLINE_CURVE_WITH_KNOTS('',3,(#80603,#80604,#80605,#80606,#80607,
#80608,#80609,#80610,#80611,#80612,#80613),.UNSPECIFIED.,.F.,.F.,(4,1,1,
1,1,1,1,1,4),(28.2743338823081,28.3634713341021,29.3609764203257,30.3584815065493,
31.3559865927729,32.3534916789965,33.3509967652201,34.3485018514437,34.5575191894877),
 .UNSPECIFIED.);
#1875=B_SPLINE_CURVE_WITH_KNOTS('',3,(#80618,#80619,#80620,#80621,#80622,
#80623,#80624,#80625,#80626,#80627),.UNSPECIFIED.,.F.,.F.,(4,1,1,1,1,1,
1,4),(21.9911485751285,22.8315448107673,23.8290498969909,24.8265549832145,
25.8240600694381,26.8215651556617,27.8190702418853,28.2743338823081),
 .UNSPECIFIED.);
#1876=B_SPLINE_CURVE_WITH_KNOTS('',3,(#80628,#80629,#80630,#80631,#80632,
#80633,#80634,#80635,#80636,#80637),.UNSPECIFIED.,.F.,.F.,(4,1,1,1,1,1,
1,4),(21.9911485751285,22.3784408167605,23.3759459029841,24.3734509892077,
25.3709560754313,26.3684611616549,27.3659662478785,28.2743338823081),
 .UNSPECIFIED.);
#1877=B_SPLINE_CURVE_WITH_KNOTS('',3,(#80643,#80644,#80645,#80646,#80647),
 .UNSPECIFIED.,.F.,.F.,(4,1,4),(14.3984001269718,15.3959052131954,15.7079632679489),
 .UNSPECIFIED.);
#1878=B_SPLINE_CURVE_WITH_KNOTS('',3,(#80650,#80651,#80652,#80653,#80654),
 .UNSPECIFIED.,.F.,.F.,(4,1,4),(13.8759337553362,14.8515041209785,15.7079632679489),
 .UNSPECIFIED.);
#1879=B_SPLINE_CURVE_WITH_KNOTS('',3,(#80660,#80661,#80662,#80663,#80664,
#80665,#80666,#80667),.UNSPECIFIED.,.F.,.F.,(4,1,1,1,1,4),(135.088484104361,
135.549619554033,136.547124640257,137.544629726481,138.542134812704,139.539639898928),
 .UNSPECIFIED.);
#1880=B_SPLINE_CURVE_WITH_KNOTS('',3,(#80670,#80671,#80672,#80673,#80674,
#80675,#80676,#80677,#80678),.UNSPECIFIED.,.F.,.F.,(4,1,1,1,1,1,4),(135.088484104361,
135.096515560027,136.09402064625,137.091525732474,138.089030818698,139.086535904921,
140.062106270563),.UNSPECIFIED.);
#1881=B_SPLINE_CURVE_WITH_KNOTS('',3,(#80683,#80684,#80685,#80686,#80687,
#80688,#80689,#80690,#80691,#80692),.UNSPECIFIED.,.F.,.F.,(4,1,1,1,1,1,
1,4),(128.805298797182,129.564589036692,130.562094122916,131.559599209139,
132.557104295363,133.554609381586,134.55211446781,135.088484104361),
 .UNSPECIFIED.);
#1882=B_SPLINE_CURVE_WITH_KNOTS('',3,(#80693,#80694,#80695,#80696,#80697,
#80698,#80699,#80700,#80701,#80702),.UNSPECIFIED.,.F.,.F.,(4,1,1,1,1,1,
1,4),(128.805298797182,129.111485042685,130.108990128909,131.106495215132,
132.104000301356,133.10150538758,134.099010473803,135.088484104361),
 .UNSPECIFIED.);
#1883=B_SPLINE_CURVE_WITH_KNOTS('',3,(#80707,#80708,#80709,#80710,#80711,
#80712,#80713,#80714,#80715,#80716,#80717),.UNSPECIFIED.,.F.,.F.,(4,1,1,
1,1,1,1,1,4),(122.522113490002,122.582053433127,123.57955851935,124.577063605574,
125.574568691798,126.572073778021,127.569578864245,128.567083950468,128.805298797182),
 .UNSPECIFIED.);
#1884=B_SPLINE_CURVE_WITH_KNOTS('',3,(#80718,#80719,#80720,#80721,#80722,
#80723,#80724,#80725,#80726,#80727),.UNSPECIFIED.,.F.,.F.,(4,1,1,1,1,1,
1,4),(122.522113490002,123.126454525344,124.123959611567,125.121464697791,
126.118969784014,127.116474870238,128.113979956462,128.805298797182),
 .UNSPECIFIED.);
#1885=B_SPLINE_CURVE_WITH_KNOTS('',3,(#80732,#80733,#80734,#80735,#80736,
#80737,#80738,#80739,#80740,#80741),.UNSPECIFIED.,.F.,.F.,(4,1,1,1,1,1,
1,4),(116.238928182822,116.597022915785,117.594528002009,118.592033088232,
119.589538174456,120.58704326068,121.584548346903,122.522113490002),
 .UNSPECIFIED.);
#1886=B_SPLINE_CURVE_WITH_KNOTS('',3,(#80742,#80743,#80744,#80745,#80746,
#80747,#80748,#80749,#80750,#80751),.UNSPECIFIED.,.F.,.F.,(4,1,1,1,1,1,
1,4),(116.238928182822,117.141424008002,118.138929094226,119.136434180449,
120.133939266673,121.131444352896,122.12894943912,122.522113490002),
 .UNSPECIFIED.);
#1887=B_SPLINE_CURVE_WITH_KNOTS('',3,(#80756,#80757,#80758,#80759,#80760,
#80761,#80762,#80763,#80764,#80765),.UNSPECIFIED.,.F.,.F.,(4,1,1,1,1,1,
1,4),(109.955742875643,110.611992398444,111.609497484667,112.607002570891,
113.604507657114,114.602012743338,115.599517829562,116.238928182822),
 .UNSPECIFIED.);
#1888=B_SPLINE_CURVE_WITH_KNOTS('',3,(#80766,#80767,#80768,#80769,#80770,
#80771,#80772,#80773,#80774,#80775,#80776),.UNSPECIFIED.,.F.,.F.,(4,1,1,
1,1,1,1,1,4),(109.955742875643,110.158888404437,111.15639349066,112.153898576884,
113.151403663108,114.148908749331,115.146413835555,116.143918921778,116.238928182822),
 .UNSPECIFIED.);
#1889=B_SPLINE_CURVE_WITH_KNOTS('',3,(#80781,#80782,#80783,#80784,#80785,
#80786,#80787,#80788,#80789,#80790),.UNSPECIFIED.,.F.,.F.,(4,1,1,1,1,1,
1,4),(103.672557568463,104.626961881102,105.624466967326,106.621972053549,
107.619477139773,108.616982225996,109.61448731222,109.955742875643),
 .UNSPECIFIED.);
#1890=B_SPLINE_CURVE_WITH_KNOTS('',3,(#80791,#80792,#80793,#80794,#80795,
#80796,#80797,#80798,#80799,#80800),.UNSPECIFIED.,.F.,.F.,(4,1,1,1,1,1,
1,4),(103.672557568463,104.173857887095,105.171362973319,106.168868059543,
107.166373145766,108.16387823199,109.161383318213,109.955742875643),
 .UNSPECIFIED.);
#1891=B_SPLINE_CURVE_WITH_KNOTS('',3,(#80805,#80806,#80807,#80808,#80809,
#80810,#80811,#80812,#80813,#80814,#80815),.UNSPECIFIED.,.F.,.F.,(4,1,1,
1,1,1,1,1,4),(97.3893722612835,97.6444262775369,98.6419313637605,99.6394364499841,
100.636941536208,101.634446622431,102.631951708655,103.629456794878,103.672557568463),
 .UNSPECIFIED.);
#1892=B_SPLINE_CURVE_WITH_KNOTS('',3,(#80816,#80817,#80818,#80819,#80820,
#80821,#80822,#80823,#80824,#80825),.UNSPECIFIED.,.F.,.F.,(4,1,1,1,1,1,
1,4),(97.3893722612836,98.1888273697538,99.1863324559773,100.183837542201,
101.181342628425,102.178847714648,103.176352800872,103.672557568463),
 .UNSPECIFIED.);
#1893=B_SPLINE_CURVE_WITH_KNOTS('',3,(#80830,#80831,#80832,#80833,#80834,
#80835,#80836,#80837,#80838,#80839),.UNSPECIFIED.,.F.,.F.,(4,1,1,1,1,1,
1,4),(91.106186954104,91.6593957601953,92.6569008464189,93.6544059326425,
94.6519110188661,95.6494161050897,96.6469211913133,97.3893722612835),
 .UNSPECIFIED.);
#1894=B_SPLINE_CURVE_WITH_KNOTS('',3,(#80840,#80841,#80842,#80843,#80844,
#80845,#80846,#80847,#80848,#80849,#80850),.UNSPECIFIED.,.F.,.F.,(4,1,1,
1,1,1,1,1,4),(91.106186954104,91.2062917661886,92.2037968524122,93.2013019386358,
94.1988070248594,95.196312111083,96.1938171973066,97.1913222835302,97.3893722612836),
 .UNSPECIFIED.);
#1895=B_SPLINE_CURVE_WITH_KNOTS('',3,(#80855,#80856,#80857,#80858,#80859,
#80860,#80861,#80862,#80863,#80864),.UNSPECIFIED.,.F.,.F.,(4,1,1,1,1,1,
1,4),(84.8230016469244,85.6743652428537,86.6718703290773,87.6693754153009,
88.6668805015245,89.6643855877481,90.6618906739717,91.106186954104),
 .UNSPECIFIED.);
#1896=B_SPLINE_CURVE_WITH_KNOTS('',3,(#80865,#80866,#80867,#80868,#80869,
#80870,#80871,#80872,#80873,#80874),.UNSPECIFIED.,.F.,.F.,(4,1,1,1,1,1,
1,4),(84.8230016469244,85.221261248847,86.2187663350706,87.2162714212942,
88.2137765075178,89.2112815937414,90.208786679965,91.106186954104),
 .UNSPECIFIED.);
#1897=B_SPLINE_CURVE_WITH_KNOTS('',3,(#80879,#80880,#80881,#80882,#80883,
#80884,#80885,#80886,#80887,#80888,#80889),.UNSPECIFIED.,.F.,.F.,(4,1,1,
1,1,1,1,1,4),(78.5398163397448,78.6918296392886,79.6893347255122,80.6868398117358,
81.6843448979594,82.681849984183,83.6793550704066,84.6768601566301,84.8230016469244),
 .UNSPECIFIED.);
#1898=B_SPLINE_CURVE_WITH_KNOTS('',3,(#80890,#80891,#80892,#80893,#80894,
#80895,#80896,#80897,#80898,#80899),.UNSPECIFIED.,.F.,.F.,(4,1,1,1,1,1,
1,4),(78.5398163397448,79.2362307315054,80.233735817729,81.2312409039526,
82.2287459901762,83.2262510763998,84.2237561626234,84.8230016469244),
 .UNSPECIFIED.);
#1899=B_SPLINE_CURVE_WITH_KNOTS('',3,(#80904,#80905,#80906,#80907,#80908,
#80909,#80910,#80911,#80912,#80913),.UNSPECIFIED.,.F.,.F.,(4,1,1,1,1,1,
1,4),(72.2566310325652,72.706799121947,73.7043042081706,74.7018092943942,
75.6993143806178,76.6968194668414,77.694324553065,78.5398163397448),
 .UNSPECIFIED.);
#1900=B_SPLINE_CURVE_WITH_KNOTS('',3,(#80914,#80915,#80916,#80917,#80918,
#80919,#80920,#80921,#80922,#80923),.UNSPECIFIED.,.F.,.F.,(4,1,1,1,1,1,
1,4),(72.2566310325652,73.2512002141639,74.2487053003875,75.2462103866111,
76.2437154728347,77.2412205590582,78.2387256452818,78.5398163397448),
 .UNSPECIFIED.);
#1901=B_SPLINE_CURVE_WITH_KNOTS('',3,(#80928,#80929,#80930,#80931,#80932,
#80933,#80934,#80935,#80936,#80937),.UNSPECIFIED.,.F.,.F.,(4,1,1,1,1,1,
1,4),(65.9734457253856,66.7217686046054,67.719273690829,68.7167787770526,
69.7142838632762,70.7117889494998,71.7092940357234,72.2566310325652),
 .UNSPECIFIED.);
#1902=B_SPLINE_CURVE_WITH_KNOTS('',3,(#80938,#80939,#80940,#80941,#80942,
#80943,#80944,#80945,#80946,#80947,#80948),.UNSPECIFIED.,.F.,.F.,(4,1,1,
1,1,1,1,1,4),(65.9734457253856,66.2686646105987,67.2661696968223,68.2636747830459,
69.2611798692695,70.2586849554931,71.2561900417167,72.2536951279403,72.2566310325652),
 .UNSPECIFIED.);
#1903=B_SPLINE_CURVE_WITH_KNOTS('',3,(#80953,#80954,#80955,#80956,#80957,
#80958,#80959,#80960,#80961,#80962,#80963),.UNSPECIFIED.,.F.,.F.,(4,1,1,
1,1,1,1,1,4),(59.690260418206,59.7392330010403,60.7367380872639,61.7342431734875,
62.7317482597111,63.7292533459347,64.7267584321582,65.7242635183818,65.9734457253856),
 .UNSPECIFIED.);
#1904=B_SPLINE_CURVE_WITH_KNOTS('',3,(#80964,#80965,#80966,#80967,#80968,
#80969,#80970,#80971,#80972,#80973),.UNSPECIFIED.,.F.,.F.,(4,1,1,1,1,1,
1,4),(59.690260418206,60.2836340932571,61.2811391794807,62.2786442657043,
63.2761493519279,64.2736544381515,65.2711595243751,65.9734457253856),
 .UNSPECIFIED.);
#1905=B_SPLINE_CURVE_WITH_KNOTS('',3,(#80978,#80979,#80980,#80981,#80982,
#80983,#80984,#80985,#80986,#80987),.UNSPECIFIED.,.F.,.F.,(4,1,1,1,1,1,
1,4),(53.4070751110264,53.7542024836987,54.7517075699223,55.7492126561459,
56.7467177423695,57.7442228285931,58.7417279148167,59.690260418206),
 .UNSPECIFIED.);
#1906=B_SPLINE_CURVE_WITH_KNOTS('',3,(#80988,#80989,#80990,#80991,#80992,
#80993,#80994,#80995,#80996,#80997),.UNSPECIFIED.,.F.,.F.,(4,1,1,1,1,1,
1,4),(53.4070751110264,54.2986035759156,55.2961086621392,56.2936137483628,
57.2911188345863,58.2886239208099,59.2861290070335,59.690260418206),
 .UNSPECIFIED.);
#1907=B_SPLINE_CURVE_WITH_KNOTS('',3,(#81002,#81003,#81004,#81005,#81006,
#81007,#81008,#81009,#81010,#81011),.UNSPECIFIED.,.F.,.F.,(4,1,1,1,1,1,
1,4),(47.1238898038468,47.7691719663571,48.7666770525807,49.7641821388043,
50.7616872250279,51.7591923112515,52.7566973974751,53.4070751110264),
 .UNSPECIFIED.);
#1908=B_SPLINE_CURVE_WITH_KNOTS('',3,(#81012,#81013,#81014,#81015,#81016,
#81017,#81018,#81019,#81020,#81021,#81022),.UNSPECIFIED.,.F.,.F.,(4,1,1,
1,1,1,1,1,4),(47.1238898038468,47.3160679723504,48.313573058574,49.3110781447976,
50.3085832310212,51.3060883172448,52.3035934034684,53.301098489692,53.4070751110264),
 .UNSPECIFIED.);
#1909=B_SPLINE_CURVE_WITH_KNOTS('',3,(#81027,#81028,#81029,#81030,#81031,
#81032,#81033,#81034,#81035,#81036),.UNSPECIFIED.,.F.,.F.,(4,1,1,1,1,1,
1,4),(40.8407044966672,41.7841414490156,42.7816465352392,43.7791516214628,
44.7766567076863,45.7741617939099,46.7716668801335,47.1238898038468),
 .UNSPECIFIED.);
#1910=B_SPLINE_CURVE_WITH_KNOTS('',3,(#81037,#81038,#81039,#81040,#81041,
#81042,#81043,#81044,#81045,#81046),.UNSPECIFIED.,.F.,.F.,(4,1,1,1,1,1,
1,4),(40.8407044966673,41.3310374550088,42.3285425412324,43.326047627456,
44.3235527136796,45.3210577999032,46.3185628861268,47.1238898038468),
 .UNSPECIFIED.);
#1911=B_SPLINE_CURVE_WITH_KNOTS('',3,(#81051,#81052,#81053,#81054,#81055,
#81056,#81057,#81058,#81059,#81060,#81061),.UNSPECIFIED.,.F.,.F.,(4,1,1,
1,1,1,1,1,4),(34.5575191894876,34.8016058454504,35.799110931674,36.7966160178976,
37.7941211041212,38.7916261903448,39.7891312765684,40.786636362792,40.8407044966672),
 .UNSPECIFIED.);
#1912=B_SPLINE_CURVE_WITH_KNOTS('',3,(#81062,#81063,#81064,#81065,#81066,
#81067,#81068,#81069,#81070,#81071),.UNSPECIFIED.,.F.,.F.,(4,1,1,1,1,1,
1,4),(34.5575191894877,35.3460069376672,36.3435120238908,37.3410171101144,
38.338522196338,39.3360272825616,40.3335323687852,40.8407044966673),
 .UNSPECIFIED.);
#1913=B_SPLINE_CURVE_WITH_KNOTS('',3,(#81076,#81077,#81078,#81079,#81080,
#81081,#81082,#81083,#81084,#81085),.UNSPECIFIED.,.F.,.F.,(4,1,1,1,1,1,
1,4),(28.2743338823081,28.8165753281088,29.8140804143324,30.811585500556,
31.8090905867796,32.8065956730032,33.8041007592268,34.5575191894876),
 .UNSPECIFIED.);
#1914=B_SPLINE_CURVE_WITH_KNOTS('',3,(#81086,#81087,#81088,#81089,#81090,
#81091,#81092,#81093,#81094,#81095,#81096),.UNSPECIFIED.,.F.,.F.,(4,1,1,
1,1,1,1,1,4),(28.2743338823081,28.3634713341021,29.3609764203257,30.3584815065493,
31.3559865927729,32.3534916789965,33.3509967652201,34.3485018514437,34.5575191894877),
 .UNSPECIFIED.);
#1915=B_SPLINE_CURVE_WITH_KNOTS('',3,(#81101,#81102,#81103,#81104,#81105,
#81106,#81107,#81108,#81109,#81110),.UNSPECIFIED.,.F.,.F.,(4,1,1,1,1,1,
1,4),(21.9911485751285,22.8315448107673,23.8290498969909,24.8265549832144,
25.824060069438,26.8215651556616,27.8190702418852,28.2743338823081),
 .UNSPECIFIED.);
#1916=B_SPLINE_CURVE_WITH_KNOTS('',3,(#81111,#81112,#81113,#81114,#81115,
#81116,#81117,#81118,#81119,#81120),.UNSPECIFIED.,.F.,.F.,(4,1,1,1,1,1,
1,4),(21.9911485751285,22.3784408167605,23.3759459029841,24.3734509892077,
25.3709560754313,26.3684611616549,27.3659662478785,28.2743338823081),
 .UNSPECIFIED.);
#1917=B_SPLINE_CURVE_WITH_KNOTS('',3,(#81126,#81127,#81128,#81129,#81130),
 .UNSPECIFIED.,.F.,.F.,(4,1,4),(14.3984001269717,15.3959052131953,15.7079632679489),
 .UNSPECIFIED.);
#1918=B_SPLINE_CURVE_WITH_KNOTS('',3,(#81133,#81134,#81135,#81136,#81137),
 .UNSPECIFIED.,.F.,.F.,(4,1,4),(13.8759337553361,14.8515041209785,15.7079632679489),
 .UNSPECIFIED.);
#1919=B_SPLINE_CURVE_WITH_KNOTS('',3,(#81143,#81144,#81145,#81146,#81147,
#81148,#81149,#81150),.UNSPECIFIED.,.F.,.F.,(4,1,1,1,1,4),(135.088484104361,
135.549619554034,136.547124640257,137.544629726481,138.542134812704,139.539639898928),
 .UNSPECIFIED.);
#1920=B_SPLINE_CURVE_WITH_KNOTS('',3,(#81153,#81154,#81155,#81156,#81157,
#81158,#81159,#81160,#81161),.UNSPECIFIED.,.F.,.F.,(4,1,1,1,1,1,4),(135.088484104361,
135.096515560027,136.09402064625,137.091525732474,138.089030818698,139.086535904921,
140.062106270563),.UNSPECIFIED.);
#1921=B_SPLINE_CURVE_WITH_KNOTS('',3,(#81166,#81167,#81168,#81169,#81170,
#81171,#81172,#81173,#81174,#81175),.UNSPECIFIED.,.F.,.F.,(4,1,1,1,1,1,
1,4),(128.805298797182,129.564589036692,130.562094122916,131.559599209139,
132.557104295363,133.554609381586,134.55211446781,135.088484104361),
 .UNSPECIFIED.);
#1922=B_SPLINE_CURVE_WITH_KNOTS('',3,(#81176,#81177,#81178,#81179,#81180,
#81181,#81182,#81183,#81184,#81185),.UNSPECIFIED.,.F.,.F.,(4,1,1,1,1,1,
1,4),(128.805298797182,129.111485042685,130.108990128909,131.106495215132,
132.104000301356,133.10150538758,134.099010473803,135.088484104361),
 .UNSPECIFIED.);
#1923=B_SPLINE_CURVE_WITH_KNOTS('',3,(#81190,#81191,#81192,#81193,#81194,
#81195,#81196,#81197,#81198,#81199,#81200),.UNSPECIFIED.,.F.,.F.,(4,1,1,
1,1,1,1,1,4),(122.522113490002,122.582053433127,123.57955851935,124.577063605574,
125.574568691798,126.572073778021,127.569578864245,128.567083950468,128.805298797182),
 .UNSPECIFIED.);
#1924=B_SPLINE_CURVE_WITH_KNOTS('',3,(#81201,#81202,#81203,#81204,#81205,
#81206,#81207,#81208,#81209,#81210),.UNSPECIFIED.,.F.,.F.,(4,1,1,1,1,1,
1,4),(122.522113490002,123.126454525344,124.123959611567,125.121464697791,
126.118969784014,127.116474870238,128.113979956462,128.805298797182),
 .UNSPECIFIED.);
#1925=B_SPLINE_CURVE_WITH_KNOTS('',3,(#81215,#81216,#81217,#81218,#81219,
#81220,#81221,#81222,#81223,#81224),.UNSPECIFIED.,.F.,.F.,(4,1,1,1,1,1,
1,4),(116.238928182822,116.597022915785,117.594528002009,118.592033088232,
119.589538174456,120.58704326068,121.584548346903,122.522113490002),
 .UNSPECIFIED.);
#1926=B_SPLINE_CURVE_WITH_KNOTS('',3,(#81225,#81226,#81227,#81228,#81229,
#81230,#81231,#81232,#81233,#81234),.UNSPECIFIED.,.F.,.F.,(4,1,1,1,1,1,
1,4),(116.238928182822,117.141424008002,118.138929094226,119.136434180449,
120.133939266673,121.131444352896,122.12894943912,122.522113490002),
 .UNSPECIFIED.);
#1927=B_SPLINE_CURVE_WITH_KNOTS('',3,(#81239,#81240,#81241,#81242,#81243,
#81244,#81245,#81246,#81247,#81248),.UNSPECIFIED.,.F.,.F.,(4,1,1,1,1,1,
1,4),(109.955742875643,110.611992398444,111.609497484667,112.607002570891,
113.604507657114,114.602012743338,115.599517829562,116.238928182822),
 .UNSPECIFIED.);
#1928=B_SPLINE_CURVE_WITH_KNOTS('',3,(#81249,#81250,#81251,#81252,#81253,
#81254,#81255,#81256,#81257,#81258,#81259),.UNSPECIFIED.,.F.,.F.,(4,1,1,
1,1,1,1,1,4),(109.955742875643,110.158888404437,111.15639349066,112.153898576884,
113.151403663108,114.148908749331,115.146413835555,116.143918921778,116.238928182822),
 .UNSPECIFIED.);
#1929=B_SPLINE_CURVE_WITH_KNOTS('',3,(#81264,#81265,#81266,#81267,#81268,
#81269,#81270,#81271,#81272,#81273),.UNSPECIFIED.,.F.,.F.,(4,1,1,1,1,1,
1,4),(103.672557568463,104.626961881102,105.624466967326,106.621972053549,
107.619477139773,108.616982225996,109.61448731222,109.955742875643),
 .UNSPECIFIED.);
#1930=B_SPLINE_CURVE_WITH_KNOTS('',3,(#81274,#81275,#81276,#81277,#81278,
#81279,#81280,#81281,#81282,#81283),.UNSPECIFIED.,.F.,.F.,(4,1,1,1,1,1,
1,4),(103.672557568463,104.173857887095,105.171362973319,106.168868059543,
107.166373145766,108.16387823199,109.161383318213,109.955742875643),
 .UNSPECIFIED.);
#1931=B_SPLINE_CURVE_WITH_KNOTS('',3,(#81288,#81289,#81290,#81291,#81292,
#81293,#81294,#81295,#81296,#81297,#81298),.UNSPECIFIED.,.F.,.F.,(4,1,1,
1,1,1,1,1,4),(97.3893722612835,97.6444262775369,98.6419313637605,99.6394364499841,
100.636941536208,101.634446622431,102.631951708655,103.629456794878,103.672557568463),
 .UNSPECIFIED.);
#1932=B_SPLINE_CURVE_WITH_KNOTS('',3,(#81299,#81300,#81301,#81302,#81303,
#81304,#81305,#81306,#81307,#81308),.UNSPECIFIED.,.F.,.F.,(4,1,1,1,1,1,
1,4),(97.3893722612836,98.1888273697538,99.1863324559774,100.183837542201,
101.181342628425,102.178847714648,103.176352800872,103.672557568463),
 .UNSPECIFIED.);
#1933=B_SPLINE_CURVE_WITH_KNOTS('',3,(#81313,#81314,#81315,#81316,#81317,
#81318,#81319,#81320,#81321,#81322),.UNSPECIFIED.,.F.,.F.,(4,1,1,1,1,1,
1,4),(91.106186954104,91.6593957601953,92.6569008464189,93.6544059326425,
94.6519110188661,95.6494161050897,96.6469211913133,97.3893722612835),
 .UNSPECIFIED.);
#1934=B_SPLINE_CURVE_WITH_KNOTS('',3,(#81323,#81324,#81325,#81326,#81327,
#81328,#81329,#81330,#81331,#81332,#81333),.UNSPECIFIED.,.F.,.F.,(4,1,1,
1,1,1,1,1,4),(91.106186954104,91.2062917661886,92.2037968524122,93.2013019386358,
94.1988070248594,95.196312111083,96.1938171973066,97.1913222835302,97.3893722612836),
 .UNSPECIFIED.);
#1935=B_SPLINE_CURVE_WITH_KNOTS('',3,(#81338,#81339,#81340,#81341,#81342,
#81343,#81344,#81345,#81346,#81347),.UNSPECIFIED.,.F.,.F.,(4,1,1,1,1,1,
1,4),(84.8230016469244,85.6743652428538,86.6718703290774,87.669375415301,
88.6668805015246,89.6643855877482,90.6618906739717,91.106186954104),
 .UNSPECIFIED.);
#1936=B_SPLINE_CURVE_WITH_KNOTS('',3,(#81348,#81349,#81350,#81351,#81352,
#81353,#81354,#81355,#81356,#81357),.UNSPECIFIED.,.F.,.F.,(4,1,1,1,1,1,
1,4),(84.8230016469244,85.221261248847,86.2187663350706,87.2162714212942,
88.2137765075178,89.2112815937414,90.208786679965,91.106186954104),
 .UNSPECIFIED.);
#1937=B_SPLINE_CURVE_WITH_KNOTS('',3,(#81362,#81363,#81364,#81365,#81366,
#81367,#81368,#81369,#81370,#81371,#81372),.UNSPECIFIED.,.F.,.F.,(4,1,1,
1,1,1,1,1,4),(78.5398163397448,78.6918296392886,79.6893347255122,80.6868398117358,
81.6843448979594,82.681849984183,83.6793550704066,84.6768601566302,84.8230016469244),
 .UNSPECIFIED.);
#1938=B_SPLINE_CURVE_WITH_KNOTS('',3,(#81373,#81374,#81375,#81376,#81377,
#81378,#81379,#81380,#81381,#81382),.UNSPECIFIED.,.F.,.F.,(4,1,1,1,1,1,
1,4),(78.5398163397448,79.2362307315055,80.233735817729,81.2312409039526,
82.2287459901762,83.2262510763998,84.2237561626234,84.8230016469244),
 .UNSPECIFIED.);
#1939=B_SPLINE_CURVE_WITH_KNOTS('',3,(#81387,#81388,#81389,#81390,#81391,
#81392,#81393,#81394,#81395,#81396),.UNSPECIFIED.,.F.,.F.,(4,1,1,1,1,1,
1,4),(72.2566310325652,72.706799121947,73.7043042081706,74.7018092943942,
75.6993143806178,76.6968194668414,77.694324553065,78.5398163397448),
 .UNSPECIFIED.);
#1940=B_SPLINE_CURVE_WITH_KNOTS('',3,(#81397,#81398,#81399,#81400,#81401,
#81402,#81403,#81404,#81405,#81406),.UNSPECIFIED.,.F.,.F.,(4,1,1,1,1,1,
1,4),(72.2566310325652,73.2512002141639,74.2487053003875,75.2462103866111,
76.2437154728347,77.2412205590583,78.2387256452818,78.5398163397448),
 .UNSPECIFIED.);
#1941=B_SPLINE_CURVE_WITH_KNOTS('',3,(#81411,#81412,#81413,#81414,#81415,
#81416,#81417,#81418,#81419,#81420),.UNSPECIFIED.,.F.,.F.,(4,1,1,1,1,1,
1,4),(65.9734457253856,66.7217686046055,67.7192736908291,68.7167787770527,
69.7142838632763,70.7117889494998,71.7092940357234,72.2566310325652),
 .UNSPECIFIED.);
#1942=B_SPLINE_CURVE_WITH_KNOTS('',3,(#81421,#81422,#81423,#81424,#81425,
#81426,#81427,#81428,#81429,#81430,#81431),.UNSPECIFIED.,.F.,.F.,(4,1,1,
1,1,1,1,1,4),(65.9734457253856,66.2686646105987,67.2661696968223,68.2636747830459,
69.2611798692695,70.2586849554931,71.2561900417167,72.2536951279403,72.2566310325652),
 .UNSPECIFIED.);
#1943=B_SPLINE_CURVE_WITH_KNOTS('',3,(#81436,#81437,#81438,#81439,#81440,
#81441,#81442,#81443,#81444,#81445,#81446),.UNSPECIFIED.,.F.,.F.,(4,1,1,
1,1,1,1,1,4),(59.690260418206,59.7392330010403,60.7367380872639,61.7342431734875,
62.7317482597111,63.7292533459347,64.7267584321583,65.7242635183819,65.9734457253856),
 .UNSPECIFIED.);
#1944=B_SPLINE_CURVE_WITH_KNOTS('',3,(#81447,#81448,#81449,#81450,#81451,
#81452,#81453,#81454,#81455,#81456),.UNSPECIFIED.,.F.,.F.,(4,1,1,1,1,1,
1,4),(59.690260418206,60.2836340932571,61.2811391794807,62.2786442657043,
63.2761493519279,64.2736544381515,65.2711595243751,65.9734457253856),
 .UNSPECIFIED.);
#1945=B_SPLINE_CURVE_WITH_KNOTS('',3,(#81461,#81462,#81463,#81464,#81465,
#81466,#81467,#81468,#81469,#81470),.UNSPECIFIED.,.F.,.F.,(4,1,1,1,1,1,
1,4),(53.4070751110264,53.7542024836987,54.7517075699223,55.7492126561459,
56.7467177423695,57.7442228285931,58.7417279148167,59.690260418206),
 .UNSPECIFIED.);
#1946=B_SPLINE_CURVE_WITH_KNOTS('',3,(#81471,#81472,#81473,#81474,#81475,
#81476,#81477,#81478,#81479,#81480),.UNSPECIFIED.,.F.,.F.,(4,1,1,1,1,1,
1,4),(53.4070751110264,54.2986035759156,55.2961086621392,56.2936137483628,
57.2911188345864,58.28862392081,59.2861290070336,59.690260418206),
 .UNSPECIFIED.);
#1947=B_SPLINE_CURVE_WITH_KNOTS('',3,(#81485,#81486,#81487,#81488,#81489,
#81490,#81491,#81492,#81493,#81494),.UNSPECIFIED.,.F.,.F.,(4,1,1,1,1,1,
1,4),(47.1238898038468,47.7691719663572,48.7666770525807,49.7641821388043,
50.7616872250279,51.7591923112515,52.7566973974751,53.4070751110264),
 .UNSPECIFIED.);
#1948=B_SPLINE_CURVE_WITH_KNOTS('',3,(#81495,#81496,#81497,#81498,#81499,
#81500,#81501,#81502,#81503,#81504,#81505),.UNSPECIFIED.,.F.,.F.,(4,1,1,
1,1,1,1,1,4),(47.1238898038468,47.3160679723504,48.313573058574,49.3110781447976,
50.3085832310212,51.3060883172448,52.3035934034684,53.301098489692,53.4070751110264),
 .UNSPECIFIED.);
#1949=B_SPLINE_CURVE_WITH_KNOTS('',3,(#81510,#81511,#81512,#81513,#81514,
#81515,#81516,#81517,#81518,#81519),.UNSPECIFIED.,.F.,.F.,(4,1,1,1,1,1,
1,4),(40.8407044966672,41.7841414490156,42.7816465352392,43.7791516214628,
44.7766567076864,45.77416179391,46.7716668801336,47.1238898038468),
 .UNSPECIFIED.);
#1950=B_SPLINE_CURVE_WITH_KNOTS('',3,(#81520,#81521,#81522,#81523,#81524,
#81525,#81526,#81527,#81528,#81529),.UNSPECIFIED.,.F.,.F.,(4,1,1,1,1,1,
1,4),(40.8407044966673,41.3310374550088,42.3285425412324,43.326047627456,
44.3235527136796,45.3210577999032,46.3185628861268,47.1238898038468),
 .UNSPECIFIED.);
#1951=B_SPLINE_CURVE_WITH_KNOTS('',3,(#81534,#81535,#81536,#81537,#81538,
#81539,#81540,#81541,#81542,#81543,#81544),.UNSPECIFIED.,.F.,.F.,(4,1,1,
1,1,1,1,1,4),(34.5575191894876,34.8016058454504,35.799110931674,36.7966160178976,
37.7941211041212,38.7916261903448,39.7891312765684,40.786636362792,40.8407044966672),
 .UNSPECIFIED.);
#1952=B_SPLINE_CURVE_WITH_KNOTS('',3,(#81545,#81546,#81547,#81548,#81549,
#81550,#81551,#81552,#81553,#81554),.UNSPECIFIED.,.F.,.F.,(4,1,1,1,1,1,
1,4),(34.5575191894877,35.3460069376673,36.3435120238909,37.3410171101145,
38.3385221963381,39.3360272825616,40.3335323687852,40.8407044966673),
 .UNSPECIFIED.);
#1953=B_SPLINE_CURVE_WITH_KNOTS('',3,(#81559,#81560,#81561,#81562,#81563,
#81564,#81565,#81566,#81567,#81568),.UNSPECIFIED.,.F.,.F.,(4,1,1,1,1,1,
1,4),(28.274333882308,28.8165753281089,29.8140804143324,30.811585500556,
31.8090905867796,32.8065956730032,33.8041007592268,34.5575191894876),
 .UNSPECIFIED.);
#1954=B_SPLINE_CURVE_WITH_KNOTS('',3,(#81569,#81570,#81571,#81572,#81573,
#81574,#81575,#81576,#81577,#81578,#81579),.UNSPECIFIED.,.F.,.F.,(4,1,1,
1,1,1,1,1,4),(28.2743338823081,28.3634713341021,29.3609764203257,30.3584815065493,
31.3559865927729,32.3534916789965,33.3509967652201,34.3485018514437,34.5575191894877),
 .UNSPECIFIED.);
#1955=B_SPLINE_CURVE_WITH_KNOTS('',3,(#81584,#81585,#81586,#81587,#81588,
#81589,#81590,#81591,#81592,#81593),.UNSPECIFIED.,.F.,.F.,(4,1,1,1,1,1,
1,4),(21.9911485751285,22.8315448107673,23.8290498969909,24.8265549832145,
25.8240600694381,26.8215651556617,27.8190702418853,28.274333882308),
 .UNSPECIFIED.);
#1956=B_SPLINE_CURVE_WITH_KNOTS('',3,(#81594,#81595,#81596,#81597,#81598,
#81599,#81600,#81601,#81602,#81603),.UNSPECIFIED.,.F.,.F.,(4,1,1,1,1,1,
1,4),(21.9911485751285,22.3784408167605,23.3759459029841,24.3734509892077,
25.3709560754313,26.3684611616549,27.3659662478785,28.2743338823081),
 .UNSPECIFIED.);
#1957=B_SPLINE_CURVE_WITH_KNOTS('',3,(#81609,#81610,#81611,#81612,#81613),
 .UNSPECIFIED.,.F.,.F.,(4,1,4),(14.3984001269718,15.3959052131954,15.7079632679489),
 .UNSPECIFIED.);
#1958=B_SPLINE_CURVE_WITH_KNOTS('',3,(#81616,#81617,#81618,#81619,#81620),
 .UNSPECIFIED.,.F.,.F.,(4,1,4),(13.8759337553362,14.8515041209785,15.7079632679489),
 .UNSPECIFIED.);
#1959=B_SPLINE_CURVE_WITH_KNOTS('',3,(#81622,#81623,#81624,#81625,#81626,
#81627,#81628,#81629,#81630,#81631,#81632),.UNSPECIFIED.,.F.,.F.,(4,1,1,
1,1,1,1,1,4),(15.7079632679489,15.8490092072021,16.8465142934257,17.8440193796493,
18.8415244658729,19.8390295520965,20.8365346383201,21.8340397245437,21.9911485751285),
 .UNSPECIFIED.);
#1960=B_SPLINE_CURVE_WITH_KNOTS('',3,(#81633,#81634,#81635,#81636,#81637,
#81638,#81639,#81640,#81641,#81642),.UNSPECIFIED.,.F.,.F.,(4,1,1,1,1,1,
1,4),(15.7079632679489,16.393410299419,17.3909153856426,18.3884204718662,
19.3859255580897,20.3834306443133,21.3809357305369,21.9911485751285),
 .UNSPECIFIED.);
#1961=B_SPLINE_CURVE_WITH_KNOTS('',3,(#82167,#82168,#82169,#82170,#82171,
#82172,#82173,#82174,#82175,#82176,#82177,#82178,#82179,#82180,#82181,#82182,
#82183,#82184,#82185,#82186,#82187,#82188,#82189,#82190,#82191,#82192,#82193,
#82194,#82195,#82196,#82197,#82198,#82199,#82200,#82201,#82202,#82203,#82204,
#82205,#82206,#82207,#82208,#82209,#82210,#82211,#82212,#82213,#82214,#82215,
#82216,#82217,#82218,#82219,#82220,#82221,#82222,#82223,#82224,#82225,#82226,
#82227,#82228,#82229,#82230,#82231,#82232,#82233,#82234,#82235,#82236,#82237,
#82238,#82239,#82240,#82241,#82242,#82243,#82244,#82245,#82246,#82247,#82248,
#82249,#82250,#82251,#82252,#82253,#82254,#82255,#82256,#82257,#82258,#82259,
#82260),.UNSPECIFIED.,.F.,.F.,(4,3,3,3,3,3,3,3,3,3,3,3,3,3,3,3,3,3,3,3,
3,3,3,3,3,3,3,3,3,3,3,4),(0.,0.0297230920696365,0.060107320285424,0.0895195747239277,
0.115255297357618,0.120660678709402,0.150423453169379,0.180022111707072,
0.208867922728668,0.221306013693075,0.229868731119957,0.234141593208093,
0.262685293208723,0.290598240531792,0.295405355793454,0.324357010294601,
0.334002571891444,0.339561520558749,0.343329583411178,0.371420199829295,
0.399566425708994,0.427315118725961,0.438104957742258,0.444429055894153,
0.449092671597708,0.477735779253812,0.499218109995891,0.505823880640041,
0.512084154674993,0.538002247703493,0.563665102222126,0.569248610399162),
 .UNSPECIFIED.);
#1962=B_SPLINE_CURVE_WITH_KNOTS('',3,(#82261,#82262,#82263,#82264,#82265,
#82266,#82267,#82268,#82269,#82270,#82271,#82272,#82273,#82274,#82275,#82276,
#82277,#82278,#82279,#82280,#82281,#82282,#82283,#82284,#82285,#82286,#82287,
#82288,#82289,#82290,#82291,#82292,#82293,#82294,#82295,#82296,#82297,#82298,
#82299,#82300,#82301,#82302,#82303,#82304,#82305,#82306,#82307,#82308,#82309,
#82310,#82311,#82312,#82313,#82314,#82315,#82316,#82317,#82318,#82319,#82320,
#82321,#82322,#82323,#82324,#82325,#82326,#82327,#82328,#82329,#82330,#82331,
#82332,#82333,#82334,#82335,#82336,#82337,#82338,#82339,#82340,#82341,#82342,
#82343,#82344,#82345,#82346,#82347,#82348,#82349,#82350,#82351,#82352,#82353,
#82354),.UNSPECIFIED.,.F.,.F.,(4,3,3,3,3,3,3,3,3,3,3,3,3,3,3,3,3,3,3,3,
3,3,3,3,3,3,3,3,3,3,3,4),(0.,0.0253621307813173,0.0513960159531074,0.0783235863046206,
0.0901043983334076,0.0965513395257098,0.102699668506175,0.130003032742825,
0.157757927018835,0.185022589955429,0.195825015771935,0.202226748487186,
0.206464577520137,0.235066962137,0.263572732749935,0.266816578765213,0.29472472571341,
0.305720896315937,0.310511082927085,0.314321197018662,0.342377239119157,
0.371487374222168,0.40093453850437,0.42163088746293,0.426693903714044,0.456743080020748,
0.482584342224751,0.492084926665187,0.49816865914989,0.529138393993325,
0.560108128836759,0.566847306048098),.UNSPECIFIED.);
#1963=B_SPLINE_CURVE_WITH_KNOTS('',3,(#82355,#82356,#82357,#82358,#82359,
#82360,#82361,#82362,#82363,#82364,#82365,#82366,#82367,#82368,#82369,#82370,
#82371,#82372,#82373,#82374,#82375,#82376,#82377,#82378,#82379),
 .UNSPECIFIED.,.F.,.F.,(4,3,3,3,3,3,3,3,4),(-10.1321597128207,-9.97505086223596,
-8.97754577601236,-7.98004068978877,-6.98253560356517,-5.98503051734157,
-4.98752543111798,-3.99002034489438,-3.84897440564113),.UNSPECIFIED.);
#1964=B_SPLINE_CURVE_WITH_KNOTS('',3,(#82904,#82905,#82906,#82907,#82908,
#82909,#82910,#82911,#82912,#82913,#82914,#82915,#82916,#82917,#82918,#82919,
#82920,#82921,#82922,#82923,#82924,#82925,#82926,#82927,#82928,#82929,#82930,
#82931,#82932,#82933,#82934,#82935,#82936,#82937,#82938,#82939,#82940,#82941,
#82942,#82943,#82944,#82945,#82946,#82947,#82948,#82949,#82950,#82951,#82952,
#82953,#82954,#82955,#82956,#82957,#82958,#82959,#82960,#82961,#82962,#82963,
#82964,#82965,#82966,#82967,#82968,#82969,#82970,#82971,#82972,#82973,#82974,
#82975,#82976,#82977,#82978,#82979,#82980,#82981,#82982,#82983,#82984,#82985,
#82986,#82987,#82988,#82989,#82990,#82991,#82992,#82993,#82994,#82995,#82996,
#82997),.UNSPECIFIED.,.F.,.F.,(4,3,3,3,3,3,3,3,3,3,3,3,3,3,3,3,3,3,3,3,
3,3,3,3,3,3,3,3,3,3,3,4),(0.,0.0253621358123242,0.0513960255360089,0.0783235946896633,
0.0901044061943871,0.096551342870137,0.102699667472934,0.130003035212993,
0.157757931226256,0.185022593111003,0.195825016620202,0.202226749482005,
0.206464578172652,0.23506696366167,0.263572732773266,0.266816578765244,
0.294724723356824,0.305720891161005,0.310511051384319,0.314321165540805,
0.342377203317934,0.371487336243674,0.400934499931709,0.421630800975239,
0.426693905360061,0.456743080929668,0.482584342906447,0.492084927719568,
0.498168658941421,0.529138393889102,0.560108128836783,0.56684730604811),
 .UNSPECIFIED.);
#1965=B_SPLINE_CURVE_WITH_KNOTS('',3,(#82998,#82999,#83000,#83001,#83002,
#83003,#83004,#83005,#83006,#83007,#83008,#83009,#83010,#83011,#83012,#83013,
#83014,#83015,#83016,#83017,#83018,#83019),.UNSPECIFIED.,.F.,.F.,(4,3,3,
3,3,3,3,4),(7.59274844815659,7.98004068978876,8.97754577601235,9.97505086223595,
10.9725559484595,11.9700610346831,12.9675661209067,13.8759337553362),
 .UNSPECIFIED.);
#1966=B_SPLINE_CURVE_WITH_KNOTS('',3,(#83020,#83021,#83022,#83023,#83024,
#83025,#83026,#83027,#83028,#83029,#83030,#83031,#83032,#83033,#83034,#83035,
#83036,#83037,#83038,#83039,#83040,#83041,#83042,#83043,#83044,#83045,#83046,
#83047,#83048,#83049,#83050,#83051,#83052,#83053,#83054,#83055,#83056,#83057,
#83058,#83059,#83060,#83061,#83062,#83063,#83064,#83065,#83066,#83067,#83068,
#83069,#83070,#83071,#83072,#83073,#83074,#83075,#83076,#83077,#83078,#83079,
#83080,#83081,#83082,#83083,#83084,#83085,#83086,#83087,#83088,#83089,#83090,
#83091,#83092,#83093,#83094,#83095,#83096,#83097,#83098,#83099,#83100,#83101,
#83102,#83103,#83104,#83105,#83106,#83107,#83108,#83109,#83110,#83111,#83112,
#83113),.UNSPECIFIED.,.F.,.F.,(4,3,3,3,3,3,3,3,3,3,3,3,3,3,3,3,3,3,3,3,
3,3,3,3,3,3,3,3,3,3,3,4),(0.,0.0297230962841146,0.0601073265980457,0.0895195802474777,
0.115255302190731,0.120660679792265,0.150423454314909,0.180022111713584,
0.208867922733564,0.221306013172714,0.229868724984429,0.234141588316278,
0.262685287083846,0.290598233431208,0.295405355793502,0.324357010515701,
0.334002571531716,0.339561519177542,0.343329581677685,0.371420198215134,
0.399566424158773,0.427315116346681,0.438104952273844,0.444429615489231,
0.449093069854903,0.477736077946735,0.499218334015609,0.505825295727651,
0.512084636520009,0.538002720680382,0.56366510222223,0.569248610399263),
 .UNSPECIFIED.);
#1967=B_SPLINE_CURVE_WITH_KNOTS('',3,(#83123,#83124,#83125,#83126,#83127,
#83128,#83129,#83130,#83131,#83132,#83133,#83134,#83135,#83136,#83137,#83138,
#83139,#83140,#83141,#83142,#83143,#83144,#83145,#83146,#83147,#83148,#83149,
#83150,#83151,#83152,#83153,#83154,#83155,#83156,#83157,#83158,#83159,#83160,
#83161,#83162,#83163,#83164,#83165,#83166,#83167,#83168,#83169,#83170,#83171,
#83172,#83173,#83174,#83175,#83176,#83177,#83178,#83179,#83180,#83181,#83182,
#83183,#83184,#83185,#83186,#83187,#83188,#83189,#83190,#83191,#83192,#83193,
#83194,#83195,#83196,#83197,#83198,#83199,#83200,#83201,#83202,#83203,#83204,
#83205,#83206,#83207,#83208,#83209,#83210,#83211,#83212,#83213,#83214,#83215,
#83216),.UNSPECIFIED.,.F.,.F.,(4,3,3,3,3,3,3,3,3,3,3,3,3,3,3,3,3,3,3,3,
3,3,3,3,3,3,3,3,3,3,3,4),(0.,0.0253579125993778,0.0513879730614739,0.078316548774439,
0.0900978006488612,0.096548549645776,0.10270053274012,0.130000942709176,
0.157754349497768,0.185019906814624,0.195824290931949,0.202225875665695,
0.206464010191211,0.235065614019142,0.263572590767915,0.266816578765194,
0.294726657909301,0.305725121816185,0.310537053618177,0.314348115889946,
0.342407723431573,0.37151966691571,0.400967327702673,0.42170458042185,0.426696514650315,
0.456746347586265,0.48258679289888,0.492091395740311,0.498168674804682,
0.529138401820704,0.560108128836725,0.566847306048067),.UNSPECIFIED.);
#1968=B_SPLINE_CURVE_WITH_KNOTS('',3,(#83217,#83218,#83219,#83220,#83221,
#83222,#83223,#83224,#83225,#83226,#83227,#83228,#83229,#83230,#83231,#83232,
#83233,#83234,#83235,#83236,#83237,#83238,#83239,#83240,#83241,#83242,#83243,
#83244,#83245,#83246,#83247,#83248,#83249,#83250,#83251,#83252,#83253,#83254,
#83255,#83256,#83257,#83258,#83259,#83260,#83261,#83262,#83263,#83264,#83265,
#83266,#83267,#83268,#83269,#83270,#83271,#83272,#83273,#83274,#83275,#83276,
#83277,#83278,#83279,#83280,#83281,#83282,#83283,#83284,#83285,#83286,#83287,
#83288,#83289,#83290,#83291,#83292,#83293,#83294,#83295,#83296,#83297,#83298,
#83299,#83300,#83301,#83302,#83303,#83304,#83305,#83306,#83307,#83308,#83309,
#83310),.UNSPECIFIED.,.F.,.F.,(4,3,3,3,3,3,3,3,3,3,3,3,3,3,3,3,3,3,3,3,
3,3,3,3,3,3,3,3,3,3,3,4),(0.,0.0297195669091192,0.0601020231284386,0.0895149397115918,
0.115251241721851,0.120659860690465,0.150422557383199,0.180022130955462,
0.208867937165012,0.221306452872675,0.229873833252823,0.234145682630168,
0.262690377679548,0.290604115247869,0.295405355793664,0.324356811547779,
0.334002824582243,0.339562575308007,0.343331007503921,0.371421512409186,
0.399567651381716,0.427316966374198,0.438109225720769,0.444058097014762,
0.44893104271735,0.47761455759364,0.499127193750858,0.50770469889405,0.513577910280885,
0.539477043608626,0.56366510222251,0.569248610399544),.UNSPECIFIED.);
#1969=B_SPLINE_CURVE_WITH_KNOTS('',3,(#83311,#83312,#83313,#83314,#83315,
#83316,#83317,#83318,#83319,#83320,#83321,#83322,#83323,#83324,#83325,#83326,
#83327,#83328,#83329,#83330,#83331,#83332,#83333,#83334,#83335,#83336,#83337,
#83338,#83339,#83340,#83341,#83342,#83343,#83344,#83345,#83346,#83347,#83348,
#83349,#83350,#83351,#83352,#83353,#83354,#83355,#83356,#83357,#83358,#83359,
#83360,#83361,#83362,#83363,#83364,#83365,#83366,#83367,#83368,#83369,#83370,
#83371,#83372,#83373,#83374,#83375,#83376,#83377,#83378,#83379,#83380,#83381,
#83382,#83383,#83384,#83385,#83386,#83387,#83388,#83389,#83390,#83391,#83392,
#83393,#83394,#83395,#83396,#83397,#83398,#83399,#83400,#83401,#83402,#83403,
#83404),.UNSPECIFIED.,.F.,.F.,(4,3,3,3,3,3,3,3,3,3,3,3,3,3,3,3,3,3,3,3,
3,3,3,3,3,3,3,3,3,3,3,4),(0.,0.0253579295510885,0.0513880054150265,0.0783165770837972,
0.0900978271888843,0.0965485607956795,0.102700529268948,0.13000095118214,
0.157754364082486,0.185019917753162,0.195824293899418,0.202225879318517,
0.206464012585979,0.235065619713782,0.263572591829656,0.266816578765192,
0.294726650343867,0.305725105274476,0.31053695159628,0.314348006525504,
0.342407600038078,0.371519536354756,0.400967195164478,0.421704281841331,
0.426696487776643,0.45674631791978,0.482586770649004,0.492091339583941,
0.498168675460501,0.529138402148588,0.560108128836676,0.566847306048011),
 .UNSPECIFIED.);
#1970=B_SPLINE_CURVE_WITH_KNOTS('',3,(#83405,#83406,#83407,#83408,#83409,
#83410,#83411,#83412,#83413,#83414,#83415,#83416,#83417,#83418,#83419,#83420,
#83421,#83422,#83423,#83424,#83425,#83426,#83427,#83428,#83429,#83430,#83431,
#83432,#83433,#83434,#83435,#83436,#83437,#83438,#83439,#83440,#83441,#83442,
#83443,#83444,#83445,#83446,#83447,#83448,#83449,#83450,#83451,#83452,#83453,
#83454,#83455,#83456,#83457,#83458,#83459,#83460,#83461,#83462,#83463,#83464,
#83465,#83466,#83467,#83468,#83469,#83470,#83471,#83472,#83473,#83474,#83475,
#83476,#83477,#83478,#83479,#83480,#83481,#83482,#83483,#83484,#83485,#83486,
#83487,#83488,#83489,#83490,#83491,#83492,#83493,#83494,#83495,#83496,#83497,
#83498),.UNSPECIFIED.,.F.,.F.,(4,3,3,3,3,3,3,3,3,3,3,3,3,3,3,3,3,3,3,3,
3,3,3,3,3,3,3,3,3,3,3,4),(0.,0.0297195615165264,0.0601020150014339,0.0895149326004449,
0.115251235499579,0.120659859449144,0.150422555982469,0.180022130905293,
0.20886793712735,0.221306453444634,0.229873839859354,0.2341456879374,0.26269038447235,
0.290604123217553,0.295405355793521,0.324356811216375,0.334002824878165,
0.339562576600837,0.343331009278728,0.371421513989523,0.399567652778866,
0.427316968616493,0.43810923101463,0.444057706366695,0.448930977598555,
0.47761450875452,0.499127157121493,0.507704470575279,0.513577860048999,
0.53947699656382,0.563665102222413,0.569248610399444),.UNSPECIFIED.);
#1971=B_SPLINE_CURVE_WITH_KNOTS('',3,(#83499,#83500,#83501,#83502,#83503,
#83504,#83505,#83506,#83507,#83508,#83509,#83510,#83511,#83512,#83513,#83514,
#83515,#83516,#83517,#83518,#83519,#83520,#83521,#83522,#83523,#83524,#83525,
#83526,#83527,#83528,#83529,#83530,#83531,#83532,#83533,#83534,#83535,#83536,
#83537,#83538,#83539,#83540,#83541,#83542,#83543,#83544,#83545,#83546,#83547,
#83548,#83549,#83550,#83551,#83552,#83553,#83554,#83555,#83556,#83557,#83558,
#83559,#83560,#83561,#83562,#83563,#83564,#83565,#83566,#83567,#83568,#83569,
#83570,#83571,#83572,#83573,#83574,#83575,#83576,#83577,#83578,#83579,#83580,
#83581,#83582,#83583,#83584,#83585,#83586,#83587,#83588,#83589,#83590,#83591,
#83592),.UNSPECIFIED.,.F.,.F.,(4,3,3,3,3,3,3,3,3,3,3,3,3,3,3,3,3,3,3,3,
3,3,3,3,3,3,3,3,3,3,3,4),(0.,0.0253579233504778,0.0513879935816182,0.078316566729565,
0.0900978174817918,0.0965485567174404,0.102700530547917,0.130000948093196,
0.157754358758536,0.1850199137602,0.195824292816032,0.202225877982008,0.206464011702015,
0.235065617622659,0.263572591433621,0.266816578765193,0.294726653110754,
0.305725111324118,0.310536988839073,0.314348046434504,0.342407645075261,
0.371519584011882,0.400967243544213,0.421704390831952,0.426696497574283,
0.456746328737469,0.482586778762282,0.492091360063141,0.498168675247584,
0.529138402042152,0.560108128836719,0.56684730604806),.UNSPECIFIED.);
#1972=B_SPLINE_CURVE_WITH_KNOTS('',3,(#83593,#83594,#83595,#83596,#83597,
#83598,#83599,#83600,#83601,#83602,#83603,#83604,#83605,#83606,#83607,#83608,
#83609,#83610,#83611,#83612,#83613,#83614,#83615,#83616,#83617,#83618,#83619,
#83620,#83621,#83622,#83623,#83624,#83625,#83626,#83627,#83628,#83629,#83630,
#83631,#83632,#83633,#83634,#83635,#83636,#83637,#83638,#83639,#83640,#83641,
#83642,#83643,#83644,#83645,#83646,#83647,#83648,#83649,#83650,#83651,#83652,
#83653,#83654,#83655,#83656,#83657,#83658,#83659,#83660,#83661,#83662,#83663,
#83664,#83665,#83666,#83667,#83668,#83669,#83670,#83671,#83672,#83673,#83674,
#83675,#83676,#83677,#83678,#83679,#83680,#83681,#83682,#83683,#83684,#83685,
#83686),.UNSPECIFIED.,.F.,.F.,(4,3,3,3,3,3,3,3,3,3,3,3,3,3,3,3,3,3,3,3,
3,3,3,3,3,3,3,3,3,3,3,4),(0.,0.02971955658432,0.0601020075682883,0.0895149260964493,
0.11525122980859,0.120659858309036,0.150422554696353,0.180022130854125,
0.208867937088988,0.221306453963038,0.229873845849775,0.234145692673294,
0.262690390567024,0.290604130388979,0.295405355793577,0.324356810915373,
0.334002825153036,0.339562577828411,0.343331010981896,0.371421515515497,
0.39956765413632,0.427316970744013,0.438109236017469,0.444057339059148,
0.448930916434902,0.47761446288177,0.49912712271692,0.507704256104763,0.513577812862897,
0.53947695230609,0.563665102222372,0.569248610399409),.UNSPECIFIED.);
#1973=B_SPLINE_CURVE_WITH_KNOTS('',3,(#83687,#83688,#83689,#83690,#83691,
#83692,#83693,#83694,#83695,#83696,#83697,#83698,#83699,#83700,#83701,#83702,
#83703,#83704,#83705,#83706,#83707,#83708,#83709,#83710,#83711,#83712,#83713,
#83714,#83715,#83716,#83717,#83718,#83719,#83720,#83721,#83722,#83723,#83724,
#83725,#83726,#83727,#83728,#83729,#83730,#83731,#83732,#83733,#83734,#83735,
#83736,#83737,#83738,#83739,#83740,#83741,#83742,#83743,#83744,#83745,#83746,
#83747,#83748,#83749,#83750,#83751,#83752,#83753,#83754,#83755,#83756,#83757,
#83758,#83759,#83760,#83761,#83762,#83763,#83764,#83765,#83766,#83767,#83768,
#83769,#83770,#83771,#83772,#83773,#83774,#83775,#83776,#83777,#83778,#83779,
#83780),.UNSPECIFIED.,.F.,.F.,(4,3,3,3,3,3,3,3,3,3,3,3,3,3,3,3,3,3,3,3,
3,3,3,3,3,3,3,3,3,3,3,4),(0.,0.0253579177000947,0.0513879827971935,0.0783165572931898,
0.0900978086351882,0.096548553000782,0.10270053169639,0.130000945260459,
0.15775435388846,0.185019910107636,0.195824291825238,0.202225876764932,
0.206464010941052,0.235065615761965,0.263572591116789,0.266816578765164,
0.294726655632965,0.305725116839123,0.310537022942245,0.314348082986944,
0.342407686307513,0.371519627634975,0.400967287826622,0.421704490588119,
0.42669650652894,0.456746338622913,0.482586786176388,0.492091378775912,
0.49816867504133,0.529138401939073,0.560108128836816,0.566847306048155),
 .UNSPECIFIED.);
#1974=B_SPLINE_CURVE_WITH_KNOTS('',3,(#83781,#83782,#83783,#83784,#83785,
#83786,#83787,#83788,#83789,#83790,#83791,#83792,#83793,#83794,#83795,#83796,
#83797,#83798,#83799,#83800,#83801,#83802,#83803,#83804,#83805,#83806,#83807,
#83808,#83809,#83810,#83811,#83812,#83813,#83814,#83815,#83816,#83817,#83818,
#83819,#83820,#83821,#83822,#83823,#83824,#83825,#83826,#83827,#83828,#83829,
#83830,#83831,#83832,#83833,#83834,#83835,#83836,#83837,#83838,#83839,#83840,
#83841,#83842,#83843,#83844,#83845,#83846,#83847,#83848,#83849,#83850,#83851,
#83852,#83853,#83854,#83855,#83856,#83857,#83858,#83859,#83860,#83861,#83862,
#83863,#83864,#83865,#83866,#83867,#83868,#83869,#83870,#83871,#83872,#83873,
#83874),.UNSPECIFIED.,.F.,.F.,(4,3,3,3,3,3,3,3,3,3,3,3,3,3,3,3,3,3,3,3,
3,3,3,3,3,3,3,3,3,3,3,4),(0.,0.0297195727594163,0.0601020319440672,0.0895149474252613,
0.115251248471306,0.120659862032104,0.150422558897904,0.180022131005185,
0.208867937202294,0.221306452247928,0.229873826038458,0.234145676897509,
0.262690370335612,0.290604106627827,0.29540535579362,0.32435681190214,0.334002824250451,
0.339562573810048,0.343331005503615,0.371421510618914,0.399567649790246,
0.427316963867809,0.43810921982249,0.444058531569151,0.448931115602164,
0.477614612257223,0.499127234748518,0.507704954507689,0.513577966546108,
0.539477096392581,0.563665102222402,0.569248610399436),.UNSPECIFIED.);
#1975=B_SPLINE_CURVE_WITH_KNOTS('',3,(#83875,#83876,#83877,#83878,#83879,
#83880,#83881,#83882,#83883,#83884,#83885,#83886,#83887,#83888,#83889,#83890,
#83891,#83892,#83893,#83894,#83895,#83896,#83897,#83898,#83899,#83900,#83901,
#83902,#83903,#83904,#83905,#83906,#83907,#83908,#83909,#83910,#83911,#83912,
#83913,#83914,#83915,#83916,#83917,#83918,#83919,#83920,#83921,#83922,#83923,
#83924,#83925,#83926,#83927,#83928,#83929,#83930,#83931,#83932,#83933,#83934,
#83935,#83936,#83937,#83938,#83939,#83940,#83941,#83942,#83943,#83944,#83945,
#83946,#83947,#83948,#83949,#83950,#83951,#83952,#83953,#83954,#83955,#83956,
#83957,#83958,#83959,#83960,#83961,#83962,#83963,#83964,#83965,#83966,#83967,
#83968),.UNSPECIFIED.,.F.,.F.,(4,3,3,3,3,3,3,3,3,3,3,3,3,3,3,3,3,3,3,3,
3,3,3,3,3,3,3,3,3,3,3,4),(0.,0.0253621238738449,0.051396002794732,0.078323574791042,
0.0901043875394277,0.0965513349313581,0.102699669924291,0.130003029352741,
0.157757921246207,0.185022585625959,0.195825014607035,0.202226747115019,
0.206464576640171,0.235066960042815,0.263572732714624,0.266816578765213,
0.294724728954443,0.305720903404729,0.310511126288789,0.314321240463125,
0.34237728851459,0.371487426613087,0.400934591712638,0.421631006765666,
0.426693901339546,0.456743078656559,0.482584341201609,0.492084925019561,
0.498168659606258,0.529138394221508,0.560108128836759,0.566847306048098),
 .UNSPECIFIED.);
#1976=B_SPLINE_CURVE_WITH_KNOTS('',3,(#83969,#83970,#83971,#83972,#83973,
#83974,#83975,#83976,#83977,#83978,#83979,#83980,#83981,#83982,#83983,#83984,
#83985,#83986,#83987,#83988,#83989,#83990,#83991,#83992,#83993,#83994,#83995,
#83996,#83997,#83998,#83999,#84000,#84001,#84002,#84003,#84004,#84005,#84006,
#84007,#84008,#84009,#84010,#84011,#84012,#84013,#84014,#84015,#84016,#84017,
#84018,#84019,#84020,#84021,#84022,#84023,#84024,#84025,#84026,#84027,#84028,
#84029,#84030,#84031,#84032,#84033,#84034,#84035,#84036,#84037,#84038,#84039,
#84040,#84041,#84042,#84043,#84044,#84045,#84046,#84047,#84048,#84049,#84050,
#84051,#84052,#84053,#84054,#84055,#84056,#84057,#84058,#84059,#84060,#84061,
#84062),.UNSPECIFIED.,.F.,.F.,(4,3,3,3,3,3,3,3,3,3,3,3,3,3,3,3,3,3,3,3,
3,3,3,3,3,3,3,3,3,3,3,4),(0.,0.0297231029452647,0.0601073365800704,0.0895195889817508,
0.115255309833221,0.120660681336277,0.15042345595793,0.18002211156947,0.208867922625481,
0.221306012212383,0.22986871379436,0.23414157933724,0.262685276183272,0.290598221000729,
0.295405355793514,0.324357010860702,0.334002570950606,0.339561516830048,
0.34332957848535,0.371420195205431,0.399566421251306,0.427315112131658,
0.438104942680454,0.444430605284565,0.449093775635353,0.477736607282077,
0.49921873101712,0.505827805964956,0.512085493792728,0.538003562612052,
0.56366510222225,0.569248610399281),.UNSPECIFIED.);
#1977=B_SPLINE_CURVE_WITH_KNOTS('',3,(#84064,#84065,#84066,#84067,#84068,
#84069,#84070,#84071,#84072,#84073,#84074),.UNSPECIFIED.,.F.,.F.,(4,1,1,
1,1,1,1,1,4),(15.7079632679489,15.8490092072021,16.8465142934257,17.8440193796493,
18.8415244658729,19.8390295520965,20.8365346383201,21.8340397245437,21.9911485751285),
 .UNSPECIFIED.);
#1978=B_SPLINE_CURVE_WITH_KNOTS('',3,(#84075,#84076,#84077,#84078,#84079,
#84080,#84081,#84082,#84083,#84084),.UNSPECIFIED.,.F.,.F.,(4,1,1,1,1,1,
1,4),(15.7079632679489,16.3934102994189,17.3909153856425,18.3884204718661,
19.3859255580897,20.3834306443133,21.3809357305369,21.9911485751285),
 .UNSPECIFIED.);
#1979=B_SPLINE_CURVE_WITH_KNOTS('',3,(#84609,#84610,#84611,#84612,#84613,
#84614,#84615,#84616,#84617,#84618,#84619,#84620,#84621,#84622,#84623,#84624,
#84625,#84626,#84627,#84628,#84629,#84630,#84631,#84632,#84633,#84634,#84635,
#84636,#84637,#84638,#84639,#84640,#84641,#84642,#84643,#84644,#84645,#84646,
#84647,#84648,#84649,#84650,#84651,#84652,#84653,#84654,#84655,#84656,#84657,
#84658,#84659,#84660,#84661,#84662,#84663,#84664,#84665,#84666,#84667,#84668,
#84669,#84670,#84671,#84672,#84673,#84674,#84675,#84676,#84677,#84678,#84679,
#84680,#84681,#84682,#84683,#84684,#84685,#84686,#84687,#84688,#84689,#84690,
#84691,#84692,#84693,#84694,#84695,#84696,#84697,#84698,#84699,#84700,#84701,
#84702),.UNSPECIFIED.,.F.,.F.,(4,3,3,3,3,3,3,3,3,3,3,3,3,3,3,3,3,3,3,3,
3,3,3,3,3,3,3,3,3,3,3,4),(0.,0.029719553462866,0.0601020028625436,0.0895149219789189,
0.115251226205747,0.120659857597101,0.150422553890565,0.180022130829953,
0.208867937070851,0.221306454298592,0.229873849718833,0.234145695936532,
0.262690394687643,0.290604135187481,0.295405355793546,0.324356810724873,
0.334002825327806,0.339562578752343,0.343331012311981,0.37142151673717,
0.39956765525167,0.427316972340056,0.438109239708711,0.44405706477218,0.448930870596609,
0.477614428503011,0.499127096932812,0.507704095272053,0.513577777440086,
0.539476918814607,0.563665102222215,0.569248610399244),.UNSPECIFIED.);
#1980=B_SPLINE_CURVE_WITH_KNOTS('',3,(#84703,#84704,#84705,#84706,#84707,
#84708,#84709,#84710,#84711,#84712,#84713,#84714,#84715,#84716,#84717,#84718,
#84719,#84720,#84721,#84722,#84723,#84724,#84725,#84726,#84727),
 .UNSPECIFIED.,.F.,.F.,(4,3,3,3,3,3,3,3,4),(-10.1321597128207,-9.97505086223594,
-8.97754577601236,-7.98004068978876,-6.98253560356516,-5.98503051734157,
-4.98752543111798,-3.99002034489438,-3.84897440564114),.UNSPECIFIED.);
#1981=B_SPLINE_CURVE_WITH_KNOTS('',3,(#85252,#85253,#85254,#85255,#85256,
#85257,#85258,#85259,#85260,#85261,#85262,#85263,#85264,#85265,#85266,#85267,
#85268,#85269,#85270,#85271,#85272,#85273,#85274,#85275,#85276,#85277,#85278,
#85279,#85280,#85281,#85282,#85283,#85284,#85285,#85286,#85287,#85288,#85289,
#85290,#85291,#85292,#85293,#85294,#85295,#85296,#85297,#85298,#85299,#85300,
#85301,#85302,#85303,#85304,#85305,#85306,#85307,#85308,#85309,#85310,#85311,
#85312,#85313,#85314,#85315,#85316,#85317,#85318,#85319,#85320,#85321,#85322,
#85323,#85324,#85325,#85326,#85327,#85328,#85329,#85330,#85331,#85332,#85333,
#85334,#85335,#85336,#85337,#85338,#85339,#85340,#85341,#85342,#85343,#85344,
#85345),.UNSPECIFIED.,.F.,.F.,(4,3,3,3,3,3,3,3,3,3,3,3,3,3,3,3,3,3,3,3,
3,3,3,3,3,3,3,3,3,3,3,4),(0.,0.0253579406450752,0.0513880265848102,0.0783165956073515,
0.0900978445547133,0.0965485680929113,0.102700527035756,0.130000956771981,
0.157754373672949,0.185019924945997,0.19582429585153,0.202225881705843,
0.206464013995299,0.235065623259909,0.26357259234097,0.26681657876514,0.294726645398039,
0.305725094458983,0.31053688482791,0.314347935050642,0.342407519392621,
0.371519451018736,0.400967108531887,0.42170408668503,0.426696470332184,
0.456746298642485,0.48258675619102,0.492091303088876,0.498168676068964,
0.529138402452796,0.560108128836627,0.566847306047961),.UNSPECIFIED.);
#1982=B_SPLINE_CURVE_WITH_KNOTS('',3,(#85346,#85347,#85348,#85349,#85350,
#85351,#85352,#85353,#85354,#85355,#85356,#85357,#85358,#85359,#85360,#85361,
#85362,#85363,#85364,#85365,#85366,#85367),.UNSPECIFIED.,.F.,.F.,(4,3,3,
3,3,3,3,4),(7.5927484481566,7.98004068978877,8.97754577601236,9.97505086223596,
10.9725559484596,11.9700610346831,12.9675661209067,13.8759337553362),
 .UNSPECIFIED.);
#1983=B_SPLINE_CURVE_WITH_KNOTS('',3,(#85369,#85370,#85371,#85372,#85373,
#85374,#85375,#85376,#85377,#85378,#85379),.UNSPECIFIED.,.F.,.F.,(4,1,1,
1,1,1,1,1,4),(15.7079632679489,15.8490092072021,16.8465142934257,17.8440193796493,
18.8415244658729,19.8390295520965,20.8365346383201,21.8340397245437,21.9911485751285),
 .UNSPECIFIED.);
#1984=B_SPLINE_CURVE_WITH_KNOTS('',3,(#85380,#85381,#85382,#85383,#85384,
#85385,#85386,#85387,#85388,#85389),.UNSPECIFIED.,.F.,.F.,(4,1,1,1,1,1,
1,4),(15.7079632679489,16.393410299419,17.3909153856426,18.3884204718662,
19.3859255580897,20.3834306443133,21.3809357305369,21.9911485751285),
 .UNSPECIFIED.);
#1985=B_SPLINE_CURVE_WITH_KNOTS('',3,(#85914,#85915,#85916,#85917,#85918,
#85919,#85920,#85921,#85922,#85923,#85924,#85925,#85926,#85927,#85928,#85929,
#85930,#85931,#85932,#85933,#85934,#85935,#85936,#85937,#85938,#85939,#85940,
#85941,#85942,#85943,#85944,#85945,#85946,#85947,#85948,#85949,#85950,#85951,
#85952,#85953,#85954,#85955,#85956,#85957,#85958,#85959,#85960,#85961,#85962,
#85963,#85964,#85965,#85966,#85967,#85968,#85969,#85970,#85971,#85972,#85973,
#85974,#85975,#85976,#85977,#85978,#85979,#85980,#85981,#85982,#85983,#85984,
#85985,#85986,#85987,#85988,#85989,#85990,#85991,#85992,#85993,#85994,#85995,
#85996,#85997,#85998,#85999,#86000,#86001,#86002,#86003,#86004,#86005,#86006,
#86007),.UNSPECIFIED.,.F.,.F.,(4,3,3,3,3,3,3,3,3,3,3,3,3,3,3,3,3,3,3,3,
3,3,3,3,3,3,3,3,3,3,3,4),(0.,0.0297195582152991,0.0601020100219757,0.0895149282434353,
0.115251231687213,0.120659858671462,0.150422555105996,0.180022130855786,
0.208867937090253,0.221306453778133,0.229873843701529,0.234145691059075,
0.262690388500622,0.290604127966643,0.295405355793653,0.324356811014206,
0.334002825060996,0.33956257734427,0.343331010204372,0.371421514794185,
0.399567653472246,0.427316969833453,0.43810923392799,0.444057492748723,
0.448930941962885,0.477614482027788,0.499127137076466,0.50770434571683,
0.51357783260646,0.539476971024577,0.563665102222498,0.569248610399526),
 .UNSPECIFIED.);
#1986=B_SPLINE_CURVE_WITH_KNOTS('',3,(#86008,#86009,#86010,#86011,#86012,
#86013,#86014,#86015,#86016,#86017,#86018,#86019,#86020,#86021,#86022,#86023,
#86024,#86025,#86026,#86027,#86028,#86029,#86030,#86031,#86032),
 .UNSPECIFIED.,.F.,.F.,(4,3,3,3,3,3,3,3,4),(-10.1321597128207,-9.97505086223596,
-8.97754577601236,-7.98004068978876,-6.98253560356516,-5.98503051734157,
-4.98752543111797,-3.99002034489438,-3.84897440564114),.UNSPECIFIED.);
#1987=B_SPLINE_CURVE_WITH_KNOTS('',3,(#86557,#86558,#86559,#86560,#86561,
#86562,#86563,#86564,#86565,#86566,#86567,#86568,#86569,#86570,#86571,#86572,
#86573,#86574,#86575,#86576,#86577,#86578,#86579,#86580,#86581,#86582,#86583,
#86584,#86585,#86586,#86587,#86588,#86589,#86590,#86591,#86592,#86593,#86594,
#86595,#86596,#86597,#86598,#86599,#86600,#86601,#86602,#86603,#86604,#86605,
#86606,#86607,#86608,#86609,#86610,#86611,#86612,#86613,#86614,#86615,#86616,
#86617,#86618,#86619,#86620,#86621,#86622,#86623,#86624,#86625,#86626,#86627,
#86628,#86629,#86630,#86631,#86632,#86633,#86634,#86635,#86636,#86637,#86638,
#86639,#86640,#86641,#86642,#86643,#86644,#86645,#86646,#86647,#86648,#86649,
#86650),.UNSPECIFIED.,.F.,.F.,(4,3,3,3,3,3,3,3,3,3,3,3,3,3,3,3,3,3,3,3,
3,3,3,3,3,3,3,3,3,3,3,4),(0.,0.0253579214134435,0.0513879898823703,0.0783165634927302,
0.0900978144472627,0.0965485554423931,0.10270053085291,0.130000947031645,
0.157754356995756,0.18501991243813,0.19582429245781,0.202225877564684,0.206464011401675,
0.235065616933209,0.263572591275628,0.26681657876525,0.294726653975806,
0.305725113216564,0.310537000090899,0.314348058459022,0.342407658669726,
0.371519598417381,0.400967258172793,0.421704423796584,0.42669650037878,
0.456746331848251,0.482586781095382,0.492091365967282,0.498168675056121,
0.529138401946449,0.560108128836777,0.56684730604809),.UNSPECIFIED.);
#1988=B_SPLINE_CURVE_WITH_KNOTS('',3,(#86651,#86652,#86653,#86654,#86655,
#86656,#86657,#86658,#86659,#86660,#86661,#86662,#86663,#86664,#86665,#86666,
#86667,#86668,#86669,#86670,#86671,#86672),.UNSPECIFIED.,.F.,.F.,(4,3,3,
3,3,3,3,4),(7.5927484481566,7.98004068978878,8.97754577601237,9.97505086223597,
10.9725559484596,11.9700610346831,12.9675661209067,13.8759337553362),
 .UNSPECIFIED.);
#1989=B_SPLINE_CURVE_WITH_KNOTS('',3,(#86674,#86675,#86676,#86677,#86678,
#86679,#86680,#86681,#86682,#86683,#86684),.UNSPECIFIED.,.F.,.F.,(4,1,1,
1,1,1,1,1,4),(15.7079632679489,15.8490092072021,16.8465142934257,17.8440193796493,
18.8415244658729,19.8390295520965,20.8365346383201,21.8340397245437,21.9911485751285),
 .UNSPECIFIED.);
#1990=B_SPLINE_CURVE_WITH_KNOTS('',3,(#86685,#86686,#86687,#86688,#86689,
#86690,#86691,#86692,#86693,#86694),.UNSPECIFIED.,.F.,.F.,(4,1,1,1,1,1,
1,4),(15.7079632679489,16.393410299419,17.3909153856426,18.3884204718662,
19.3859255580897,20.3834306443133,21.3809357305369,21.9911485751285),
 .UNSPECIFIED.);
#1991=B_SPLINE_CURVE_WITH_KNOTS('',3,(#87219,#87220,#87221,#87222,#87223,
#87224,#87225,#87226,#87227,#87228,#87229,#87230,#87231,#87232,#87233,#87234,
#87235,#87236,#87237,#87238,#87239,#87240,#87241,#87242,#87243,#87244,#87245,
#87246,#87247,#87248,#87249,#87250,#87251,#87252,#87253,#87254,#87255,#87256,
#87257,#87258,#87259,#87260,#87261,#87262,#87263,#87264,#87265,#87266,#87267,
#87268,#87269,#87270,#87271,#87272,#87273,#87274,#87275,#87276,#87277,#87278,
#87279,#87280,#87281,#87282,#87283,#87284,#87285,#87286,#87287,#87288,#87289,
#87290,#87291,#87292,#87293,#87294,#87295,#87296,#87297,#87298,#87299,#87300,
#87301,#87302,#87303,#87304,#87305,#87306,#87307,#87308,#87309,#87310,#87311,
#87312),.UNSPECIFIED.,.F.,.F.,(4,3,3,3,3,3,3,3,3,3,3,3,3,3,3,3,3,3,3,3,
3,3,3,3,3,3,3,3,3,3,3,4),(0.,0.0297195634297971,0.0601020178864358,0.089514935124822,
0.11525123770841,0.120659859971453,0.150422556566061,0.180022131006724,
0.208867937203424,0.221306453316953,0.229873838332913,0.234145686845126,
0.262690382844274,0.290604121164851,0.295405355793526,0.324356811328018,
0.334002824758734,0.33956257605137,0.343331008699606,0.371421513479927,
0.399567652332435,0.427316967866253,0.438109229229592,0.444057835021416,
0.448930999083887,0.477614524868509,0.499127169206975,0.507704545860101,
0.513577876601892,0.539477012001364,0.563665102222374,0.569248610399403),
 .UNSPECIFIED.);
#1992=B_SPLINE_CURVE_WITH_KNOTS('',3,(#87313,#87314,#87315,#87316,#87317,
#87318,#87319,#87320,#87321,#87322,#87323,#87324,#87325,#87326,#87327,#87328,
#87329,#87330,#87331,#87332,#87333,#87334,#87335,#87336,#87337),
 .UNSPECIFIED.,.F.,.F.,(4,3,3,3,3,3,3,3,4),(-10.1321597128207,-9.97505086223594,
-8.97754577601235,-7.98004068978876,-6.98253560356516,-5.98503051734157,
-4.98752543111797,-3.99002034489438,-3.84897440564117),.UNSPECIFIED.);
#1993=B_SPLINE_CURVE_WITH_KNOTS('',3,(#87862,#87863,#87864,#87865,#87866,
#87867,#87868,#87869,#87870,#87871,#87872,#87873,#87874,#87875,#87876,#87877,
#87878,#87879,#87880,#87881,#87882,#87883,#87884,#87885,#87886,#87887,#87888,
#87889,#87890,#87891,#87892,#87893,#87894,#87895,#87896,#87897,#87898,#87899,
#87900,#87901,#87902,#87903,#87904,#87905,#87906,#87907,#87908,#87909,#87910,
#87911,#87912,#87913,#87914,#87915,#87916,#87917,#87918,#87919,#87920,#87921,
#87922,#87923,#87924,#87925,#87926,#87927,#87928,#87929,#87930,#87931,#87932,
#87933,#87934,#87935,#87936,#87937,#87938,#87939,#87940,#87941,#87942,#87943,
#87944,#87945,#87946,#87947,#87948,#87949,#87950,#87951,#87952,#87953,#87954,
#87955),.UNSPECIFIED.,.F.,.F.,(4,3,3,3,3,3,3,3,3,3,3,3,3,3,3,3,3,3,3,3,
3,3,3,3,3,3,3,3,3,3,3,4),(0.,0.025357927272923,0.0513880010661254,0.0783165732785213,
0.0900978236214444,0.0965485592962299,0.10270052975136,0.130000950059032,
0.157754362139206,0.185019916295728,0.195824293504795,0.202225878835774,
0.206464012200268,0.235065618877475,0.263572591616992,0.266816578765292,
0.294726651357313,0.305725107490194,0.310536965130431,0.31434802098446,
0.342407616366947,0.371519553641245,0.400967212719098,0.421704321387406,
0.426696491317579,0.456746321829517,0.482586773581365,0.492091346987436,
0.498168675113734,0.52913840197532,0.560108128836907,0.566847306048237),
 .UNSPECIFIED.);
#1994=B_SPLINE_CURVE_WITH_KNOTS('',3,(#87956,#87957,#87958,#87959,#87960,
#87961,#87962,#87963,#87964,#87965,#87966,#87967,#87968,#87969,#87970,#87971,
#87972,#87973,#87974,#87975,#87976,#87977),.UNSPECIFIED.,.F.,.F.,(4,3,3,
3,3,3,3,4),(7.59274844815661,7.98004068978877,8.97754577601236,9.97505086223595,
10.9725559484595,11.9700610346831,12.9675661209067,13.8759337553362),
 .UNSPECIFIED.);
#1995=B_SPLINE_CURVE_WITH_KNOTS('',3,(#87979,#87980,#87981,#87982,#87983,
#87984,#87985,#87986,#87987,#87988,#87989),.UNSPECIFIED.,.F.,.F.,(4,1,1,
1,1,1,1,1,4),(15.7079632679489,15.8490092072021,16.8465142934256,17.8440193796492,
18.8415244658728,19.8390295520964,20.83653463832,21.8340397245436,21.9911485751285),
 .UNSPECIFIED.);
#1996=B_SPLINE_CURVE_WITH_KNOTS('',3,(#87990,#87991,#87992,#87993,#87994,
#87995,#87996,#87997,#87998,#87999),.UNSPECIFIED.,.F.,.F.,(4,1,1,1,1,1,
1,4),(15.7079632679489,16.3934102994189,17.3909153856425,18.3884204718661,
19.3859255580897,20.3834306443133,21.3809357305369,21.9911485751285),
 .UNSPECIFIED.);
#1997=B_SPLINE_CURVE_WITH_KNOTS('',3,(#88524,#88525,#88526,#88527,#88528,
#88529,#88530,#88531,#88532,#88533,#88534,#88535,#88536,#88537,#88538,#88539,
#88540,#88541,#88542,#88543,#88544,#88545,#88546,#88547,#88548,#88549,#88550,
#88551,#88552,#88553,#88554,#88555,#88556,#88557,#88558,#88559,#88560,#88561,
#88562,#88563,#88564,#88565,#88566,#88567,#88568,#88569,#88570,#88571,#88572,
#88573,#88574,#88575,#88576,#88577,#88578,#88579,#88580,#88581,#88582,#88583,
#88584,#88585,#88586,#88587,#88588,#88589,#88590,#88591,#88592,#88593,#88594,
#88595,#88596,#88597,#88598,#88599,#88600,#88601,#88602,#88603,#88604,#88605,
#88606,#88607,#88608,#88609,#88610,#88611,#88612,#88613,#88614,#88615,#88616,
#88617),.UNSPECIFIED.,.F.,.F.,(4,3,3,3,3,3,3,3,3,3,3,3,3,3,3,3,3,3,3,3,
3,3,3,3,3,3,3,3,3,3,3,4),(0.,0.0297195491700754,0.0601019963903511,0.0895149163157588,
0.11525122125049,0.120659856525908,0.150422552697531,0.180022130709648,
0.208867936980639,0.221306454680905,0.229873854178296,0.234145699383138,
0.262690399330253,0.290604140778558,0.295405355793612,0.324356810461168,
0.334002825560677,0.339562579599788,0.343331013402581,0.371421517667901,
0.399567656038419,0.427316973809471,0.438109243258802,0.444056806999033,
0.448930828212018,0.477614396714627,0.499127073091584,0.507703946830402,
0.513577744863538,0.539476888668399,0.563665102222456,0.569248610399499),
 .UNSPECIFIED.);
#1998=B_SPLINE_CURVE_WITH_KNOTS('',3,(#88618,#88619,#88620,#88621,#88622,
#88623,#88624,#88625,#88626,#88627,#88628,#88629,#88630,#88631,#88632,#88633,
#88634,#88635,#88636,#88637,#88638,#88639,#88640,#88641,#88642),
 .UNSPECIFIED.,.F.,.F.,(4,3,3,3,3,3,3,3,4),(-10.1321597128208,-9.97505086223595,
-8.97754577601236,-7.98004068978876,-6.98253560356516,-5.98503051734157,
-4.98752543111797,-3.99002034489437,-3.8489744056412),.UNSPECIFIED.);
#1999=B_SPLINE_CURVE_WITH_KNOTS('',3,(#89167,#89168,#89169,#89170,#89171,
#89172,#89173,#89174,#89175,#89176,#89177,#89178,#89179,#89180,#89181,#89182,
#89183,#89184,#89185,#89186,#89187,#89188,#89189,#89190,#89191,#89192,#89193,
#89194,#89195,#89196,#89197,#89198,#89199,#89200,#89201,#89202,#89203,#89204,
#89205,#89206,#89207,#89208,#89209,#89210,#89211,#89212,#89213,#89214,#89215,
#89216,#89217,#89218,#89219,#89220,#89221,#89222,#89223,#89224,#89225,#89226,
#89227,#89228,#89229,#89230,#89231,#89232,#89233,#89234,#89235,#89236,#89237,
#89238,#89239,#89240,#89241,#89242,#89243,#89244,#89245,#89246,#89247,#89248,
#89249,#89250,#89251,#89252,#89253,#89254,#89255,#89256,#89257,#89258,#89259,
#89260),.UNSPECIFIED.,.F.,.F.,(4,3,3,3,3,3,3,3,3,3,3,3,3,3,3,3,3,3,3,3,
3,3,3,3,3,3,3,3,3,3,3,4),(0.,0.0253579336883674,0.0513880133105813,0.0783165839924162,
0.0900978336657191,0.0965485635161028,0.102700528459906,0.130000953296085,
0.157754367684311,0.185019920454548,0.195824294631711,0.202225880214181,
0.206464013245021,0.235065621182224,0.263572592161767,0.266816578765261,
0.294726648497761,0.305725101238404,0.310536926466407,0.314347979466994,
0.342407569538569,0.371519504099032,0.400967162424359,0.421704208089393,
0.426696481095096,0.456746310536251,0.482586765111401,0.492091325612755,
0.498168675511062,0.529138402173956,0.56010812883685,0.566847306048169),
 .UNSPECIFIED.);
#2000=B_SPLINE_CURVE_WITH_KNOTS('',3,(#89261,#89262,#89263,#89264,#89265,
#89266,#89267,#89268,#89269,#89270,#89271,#89272,#89273,#89274,#89275,#89276,
#89277,#89278,#89279,#89280,#89281,#89282),.UNSPECIFIED.,.F.,.F.,(4,3,3,
3,3,3,3,4),(7.59274844815666,7.98004068978876,8.97754577601236,9.97505086223596,
10.9725559484595,11.9700610346831,12.9675661209067,13.8759337553362),
 .UNSPECIFIED.);
#2001=B_SPLINE_CURVE_WITH_KNOTS('',3,(#89284,#89285,#89286,#89287,#89288,
#89289,#89290,#89291,#89292,#89293,#89294),.UNSPECIFIED.,.F.,.F.,(4,1,1,
1,1,1,1,1,4),(15.7079632679489,15.8490092072021,16.8465142934257,17.8440193796493,
18.8415244658729,19.8390295520965,20.8365346383201,21.8340397245437,21.9911485751285),
 .UNSPECIFIED.);
#2002=B_SPLINE_CURVE_WITH_KNOTS('',3,(#89295,#89296,#89297,#89298,#89299,
#89300,#89301,#89302,#89303,#89304),.UNSPECIFIED.,.F.,.F.,(4,1,1,1,1,1,
1,4),(15.7079632679489,16.393410299419,17.3909153856426,18.3884204718662,
19.3859255580897,20.3834306443133,21.3809357305369,21.9911485751285),
 .UNSPECIFIED.);
#2003=B_SPLINE_CURVE_WITH_KNOTS('',3,(#89829,#89830,#89831,#89832,#89833,
#89834,#89835,#89836,#89837,#89838,#89839,#89840,#89841,#89842,#89843,#89844,
#89845,#89846,#89847,#89848,#89849,#89850,#89851,#89852,#89853,#89854,#89855,
#89856,#89857,#89858,#89859,#89860,#89861,#89862,#89863,#89864,#89865,#89866,
#89867,#89868,#89869,#89870,#89871,#89872,#89873,#89874,#89875,#89876,#89877,
#89878,#89879,#89880,#89881,#89882,#89883,#89884,#89885,#89886,#89887,#89888,
#89889,#89890,#89891,#89892,#89893,#89894,#89895,#89896,#89897,#89898,#89899,
#89900,#89901,#89902,#89903,#89904,#89905,#89906,#89907,#89908,#89909,#89910,
#89911,#89912,#89913,#89914,#89915,#89916,#89917,#89918,#89919,#89920,#89921,
#89922),.UNSPECIFIED.,.F.,.F.,(4,3,3,3,3,3,3,3,3,3,3,3,3,3,3,3,3,3,3,3,
3,3,3,3,3,3,3,3,3,3,3,4),(0.,0.0297230862766818,0.0601073115992879,0.0895195671235586,
0.115255290707296,0.120660677481967,0.150423451858438,0.180022111936673,
0.208867922900868,0.22130601462086,0.229868741866763,0.23414160178478,0.262685303441991,
0.290598252086167,0.295405355793454,0.324357009993761,0.334002572396988,
0.339561522550512,0.343329586354325,0.371420202614893,0.399566428404089,
0.42731512255639,0.438104966431693,0.444428160156713,0.4490920349478,0.477735301766382,
0.499217751880318,0.505821620193661,0.512083386782307,0.538001493461072,
0.563665102222126,0.569248610399162),.UNSPECIFIED.);
#2004=B_SPLINE_CURVE_WITH_KNOTS('',3,(#89923,#89924,#89925,#89926,#89927,
#89928,#89929,#89930,#89931,#89932,#89933,#89934,#89935,#89936,#89937,#89938,
#89939,#89940,#89941,#89942,#89943,#89944,#89945,#89946,#89947),
 .UNSPECIFIED.,.F.,.F.,(4,3,3,3,3,3,3,3,4),(-10.1321597128207,-9.97505086223596,
-8.97754577601236,-7.98004068978877,-6.98253560356517,-5.98503051734157,
-4.98752543111798,-3.99002034489438,-3.84897440564113),.UNSPECIFIED.);
#2005=B_SPLINE_CURVE_WITH_KNOTS('',3,(#90472,#90473,#90474,#90475,#90476,
#90477,#90478,#90479,#90480,#90481,#90482,#90483,#90484,#90485,#90486,#90487,
#90488,#90489,#90490,#90491,#90492,#90493,#90494,#90495,#90496,#90497,#90498,
#90499,#90500,#90501,#90502,#90503,#90504,#90505,#90506,#90507,#90508,#90509,
#90510,#90511,#90512,#90513,#90514,#90515,#90516,#90517,#90518,#90519,#90520,
#90521,#90522,#90523,#90524,#90525,#90526,#90527,#90528,#90529,#90530,#90531,
#90532,#90533,#90534,#90535,#90536,#90537,#90538,#90539,#90540,#90541,#90542,
#90543,#90544,#90545,#90546,#90547,#90548,#90549,#90550,#90551,#90552,#90553,
#90554,#90555,#90556,#90557,#90558,#90559,#90560,#90561,#90562,#90563,#90564,
#90565),.UNSPECIFIED.,.F.,.F.,(4,3,3,3,3,3,3,3,3,3,3,3,3,3,3,3,3,3,3,3,
3,3,3,3,3,3,3,3,3,3,3,4),(0.,0.0253621437511135,0.051396040655139,0.0783236079188992,
0.0901044185967943,0.096551348149287,0.102699665837524,0.130003039099533,
0.157757937849826,0.185022598078675,0.195825017956751,0.202226751064942,
0.206464579201341,0.235066966115335,0.263572732855357,0.266816578765221,
0.294724719624713,0.30572088299975,0.310511001289213,0.31432111535445,0.342377146267348,
0.371487275744893,0.400934438497277,0.421630663231168,0.426693908186306,
0.45674308258997,0.482584344151671,0.492084929769549,0.498168658059089,
0.529138393447932,0.560108128836774,0.566847306048129),.UNSPECIFIED.);
#2006=B_SPLINE_CURVE_WITH_KNOTS('',3,(#90566,#90567,#90568,#90569,#90570,
#90571,#90572,#90573,#90574,#90575,#90576,#90577,#90578,#90579,#90580,#90581,
#90582,#90583,#90584,#90585,#90586,#90587),.UNSPECIFIED.,.F.,.F.,(4,3,3,
3,3,3,3,4),(7.59274844815659,7.98004068978877,8.97754577601236,9.97505086223596,
10.9725559484595,11.9700610346831,12.9675661209067,13.8759337553362),
 .UNSPECIFIED.);
#2227=SHAPE_REPRESENTATION_RELATIONSHIP('SRR','None',#97621,#2246);
#2246=ADVANCED_BREP_SHAPE_REPRESENTATION('',(#2284),#97471);
#2265=STYLED_ITEM('',(#97721),#2284);
#2284=MANIFOLD_SOLID_BREP('Body1',#21826);
#2361=FACE_BOUND('',#4770,.T.);
#2362=FACE_BOUND('',#4771,.T.);
#2363=FACE_BOUND('',#4772,.T.);
#2364=FACE_BOUND('',#4773,.T.);
#2365=FACE_BOUND('',#4774,.T.);
#2366=FACE_BOUND('',#4775,.T.);
#2367=FACE_BOUND('',#4802,.T.);
#2368=FACE_BOUND('',#4803,.T.);
#2369=FACE_BOUND('',#4804,.T.);
#2370=FACE_BOUND('',#4805,.T.);
#2371=FACE_BOUND('',#4806,.T.);
#2372=FACE_BOUND('',#4807,.T.);
#2517=PLANE('',#23308);
#2518=PLANE('',#23320);
#2519=PLANE('',#23321);
#2520=PLANE('',#23322);
#2521=PLANE('',#23323);
#2522=PLANE('',#23324);
#3299=FACE_OUTER_BOUND('',#4526,.T.);
#3300=FACE_OUTER_BOUND('',#4527,.T.);
#3301=FACE_OUTER_BOUND('',#4528,.T.);
#3302=FACE_OUTER_BOUND('',#4529,.T.);
#3303=FACE_OUTER_BOUND('',#4530,.T.);
#3304=FACE_OUTER_BOUND('',#4531,.T.);
#3305=FACE_OUTER_BOUND('',#4532,.T.);
#3306=FACE_OUTER_BOUND('',#4533,.T.);
#3307=FACE_OUTER_BOUND('',#4534,.T.);
#3308=FACE_OUTER_BOUND('',#4535,.T.);
#3309=FACE_OUTER_BOUND('',#4536,.T.);
#3310=FACE_OUTER_BOUND('',#4537,.T.);
#3311=FACE_OUTER_BOUND('',#4538,.T.);
#3312=FACE_OUTER_BOUND('',#4539,.T.);
#3313=FACE_OUTER_BOUND('',#4540,.T.);
#3314=FACE_OUTER_BOUND('',#4541,.T.);
#3315=FACE_OUTER_BOUND('',#4542,.T.);
#3316=FACE_OUTER_BOUND('',#4543,.T.);
#3317=FACE_OUTER_BOUND('',#4544,.T.);
#3318=FACE_OUTER_BOUND('',#4545,.T.);
#3319=FACE_OUTER_BOUND('',#4546,.T.);
#3320=FACE_OUTER_BOUND('',#4547,.T.);
#3321=FACE_OUTER_BOUND('',#4548,.T.);
#3322=FACE_OUTER_BOUND('',#4549,.T.);
#3323=FACE_OUTER_BOUND('',#4550,.T.);
#3324=FACE_OUTER_BOUND('',#4551,.T.);
#3325=FACE_OUTER_BOUND('',#4552,.T.);
#3326=FACE_OUTER_BOUND('',#4553,.T.);
#3327=FACE_OUTER_BOUND('',#4554,.T.);
#3328=FACE_OUTER_BOUND('',#4555,.T.);
#3329=FACE_OUTER_BOUND('',#4556,.T.);
#3330=FACE_OUTER_BOUND('',#4557,.T.);
#3331=FACE_OUTER_BOUND('',#4558,.T.);
#3332=FACE_OUTER_BOUND('',#4559,.T.);
#3333=FACE_OUTER_BOUND('',#4560,.T.);
#3334=FACE_OUTER_BOUND('',#4561,.T.);
#3335=FACE_OUTER_BOUND('',#4562,.T.);
#3336=FACE_OUTER_BOUND('',#4563,.T.);
#3337=FACE_OUTER_BOUND('',#4564,.T.);
#3338=FACE_OUTER_BOUND('',#4565,.T.);
#3339=FACE_OUTER_BOUND('',#4566,.T.);
#3340=FACE_OUTER_BOUND('',#4567,.T.);
#3341=FACE_OUTER_BOUND('',#4568,.T.);
#3342=FACE_OUTER_BOUND('',#4569,.T.);
#3343=FACE_OUTER_BOUND('',#4570,.T.);
#3344=FACE_OUTER_BOUND('',#4571,.T.);
#3345=FACE_OUTER_BOUND('',#4572,.T.);
#3346=FACE_OUTER_BOUND('',#4573,.T.);
#3347=FACE_OUTER_BOUND('',#4574,.T.);
#3348=FACE_OUTER_BOUND('',#4575,.T.);
#3349=FACE_OUTER_BOUND('',#4576,.T.);
#3350=FACE_OUTER_BOUND('',#4577,.T.);
#3351=FACE_OUTER_BOUND('',#4578,.T.);
#3352=FACE_OUTER_BOUND('',#4579,.T.);
#3353=FACE_OUTER_BOUND('',#4580,.T.);
#3354=FACE_OUTER_BOUND('',#4581,.T.);
#3355=FACE_OUTER_BOUND('',#4582,.T.);
#3356=FACE_OUTER_BOUND('',#4583,.T.);
#3357=FACE_OUTER_BOUND('',#4584,.T.);
#3358=FACE_OUTER_BOUND('',#4585,.T.);
#3359=FACE_OUTER_BOUND('',#4586,.T.);
#3360=FACE_OUTER_BOUND('',#4587,.T.);
#3361=FACE_OUTER_BOUND('',#4588,.T.);
#3362=FACE_OUTER_BOUND('',#4589,.T.);
#3363=FACE_OUTER_BOUND('',#4590,.T.);
#3364=FACE_OUTER_BOUND('',#4591,.T.);
#3365=FACE_OUTER_BOUND('',#4592,.T.);
#3366=FACE_OUTER_BOUND('',#4593,.T.);
#3367=FACE_OUTER_BOUND('',#4594,.T.);
#3368=FACE_OUTER_BOUND('',#4595,.T.);
#3369=FACE_OUTER_BOUND('',#4596,.T.);
#3370=FACE_OUTER_BOUND('',#4597,.T.);
#3371=FACE_OUTER_BOUND('',#4598,.T.);
#3372=FACE_OUTER_BOUND('',#4599,.T.);
#3373=FACE_OUTER_BOUND('',#4600,.T.);
#3374=FACE_OUTER_BOUND('',#4601,.T.);
#3375=FACE_OUTER_BOUND('',#4602,.T.);
#3376=FACE_OUTER_BOUND('',#4603,.T.);
#3377=FACE_OUTER_BOUND('',#4604,.T.);
#3378=FACE_OUTER_BOUND('',#4605,.T.);
#3379=FACE_OUTER_BOUND('',#4606,.T.);
#3380=FACE_OUTER_BOUND('',#4607,.T.);
#3381=FACE_OUTER_BOUND('',#4608,.T.);
#3382=FACE_OUTER_BOUND('',#4609,.T.);
#3383=FACE_OUTER_BOUND('',#4610,.T.);
#3384=FACE_OUTER_BOUND('',#4611,.T.);
#3385=FACE_OUTER_BOUND('',#4612,.T.);
#3386=FACE_OUTER_BOUND('',#4613,.T.);
#3387=FACE_OUTER_BOUND('',#4614,.T.);
#3388=FACE_OUTER_BOUND('',#4615,.T.);
#3389=FACE_OUTER_BOUND('',#4616,.T.);
#3390=FACE_OUTER_BOUND('',#4617,.T.);
#3391=FACE_OUTER_BOUND('',#4618,.T.);
#3392=FACE_OUTER_BOUND('',#4619,.T.);
#3393=FACE_OUTER_BOUND('',#4620,.T.);
#3394=FACE_OUTER_BOUND('',#4621,.T.);
#3395=FACE_OUTER_BOUND('',#4622,.T.);
#3396=FACE_OUTER_BOUND('',#4623,.T.);
#3397=FACE_OUTER_BOUND('',#4624,.T.);
#3398=FACE_OUTER_BOUND('',#4625,.T.);
#3399=FACE_OUTER_BOUND('',#4626,.T.);
#3400=FACE_OUTER_BOUND('',#4627,.T.);
#3401=FACE_OUTER_BOUND('',#4628,.T.);
#3402=FACE_OUTER_BOUND('',#4629,.T.);
#3403=FACE_OUTER_BOUND('',#4630,.T.);
#3404=FACE_OUTER_BOUND('',#4631,.T.);
#3405=FACE_OUTER_BOUND('',#4632,.T.);
#3406=FACE_OUTER_BOUND('',#4633,.T.);
#3407=FACE_OUTER_BOUND('',#4634,.T.);
#3408=FACE_OUTER_BOUND('',#4635,.T.);
#3409=FACE_OUTER_BOUND('',#4636,.T.);
#3410=FACE_OUTER_BOUND('',#4637,.T.);
#3411=FACE_OUTER_BOUND('',#4638,.T.);
#3412=FACE_OUTER_BOUND('',#4639,.T.);
#3413=FACE_OUTER_BOUND('',#4640,.T.);
#3414=FACE_OUTER_BOUND('',#4641,.T.);
#3415=FACE_OUTER_BOUND('',#4642,.T.);
#3416=FACE_OUTER_BOUND('',#4643,.T.);
#3417=FACE_OUTER_BOUND('',#4644,.T.);
#3418=FACE_OUTER_BOUND('',#4645,.T.);
#3419=FACE_OUTER_BOUND('',#4646,.T.);
#3420=FACE_OUTER_BOUND('',#4647,.T.);
#3421=FACE_OUTER_BOUND('',#4648,.T.);
#3422=FACE_OUTER_BOUND('',#4649,.T.);
#3423=FACE_OUTER_BOUND('',#4650,.T.);
#3424=FACE_OUTER_BOUND('',#4651,.T.);
#3425=FACE_OUTER_BOUND('',#4652,.T.);
#3426=FACE_OUTER_BOUND('',#4653,.T.);
#3427=FACE_OUTER_BOUND('',#4654,.T.);
#3428=FACE_OUTER_BOUND('',#4655,.T.);
#3429=FACE_OUTER_BOUND('',#4656,.T.);
#3430=FACE_OUTER_BOUND('',#4657,.T.);
#3431=FACE_OUTER_BOUND('',#4658,.T.);
#3432=FACE_OUTER_BOUND('',#4659,.T.);
#3433=FACE_OUTER_BOUND('',#4660,.T.);
#3434=FACE_OUTER_BOUND('',#4661,.T.);
#3435=FACE_OUTER_BOUND('',#4662,.T.);
#3436=FACE_OUTER_BOUND('',#4663,.T.);
#3437=FACE_OUTER_BOUND('',#4664,.T.);
#3438=FACE_OUTER_BOUND('',#4665,.T.);
#3439=FACE_OUTER_BOUND('',#4666,.T.);
#3440=FACE_OUTER_BOUND('',#4667,.T.);
#3441=FACE_OUTER_BOUND('',#4668,.T.);
#3442=FACE_OUTER_BOUND('',#4669,.T.);
#3443=FACE_OUTER_BOUND('',#4670,.T.);
#3444=FACE_OUTER_BOUND('',#4671,.T.);
#3445=FACE_OUTER_BOUND('',#4672,.T.);
#3446=FACE_OUTER_BOUND('',#4673,.T.);
#3447=FACE_OUTER_BOUND('',#4674,.T.);
#3448=FACE_OUTER_BOUND('',#4675,.T.);
#3449=FACE_OUTER_BOUND('',#4676,.T.);
#3450=FACE_OUTER_BOUND('',#4677,.T.);
#3451=FACE_OUTER_BOUND('',#4678,.T.);
#3452=FACE_OUTER_BOUND('',#4679,.T.);
#3453=FACE_OUTER_BOUND('',#4680,.T.);
#3454=FACE_OUTER_BOUND('',#4681,.T.);
#3455=FACE_OUTER_BOUND('',#4682,.T.);
#3456=FACE_OUTER_BOUND('',#4683,.T.);
#3457=FACE_OUTER_BOUND('',#4684,.T.);
#3458=FACE_OUTER_BOUND('',#4685,.T.);
#3459=FACE_OUTER_BOUND('',#4686,.T.);
#3460=FACE_OUTER_BOUND('',#4687,.T.);
#3461=FACE_OUTER_BOUND('',#4688,.T.);
#3462=FACE_OUTER_BOUND('',#4689,.T.);
#3463=FACE_OUTER_BOUND('',#4690,.T.);
#3464=FACE_OUTER_BOUND('',#4691,.T.);
#3465=FACE_OUTER_BOUND('',#4692,.T.);
#3466=FACE_OUTER_BOUND('',#4693,.T.);
#3467=FACE_OUTER_BOUND('',#4694,.T.);
#3468=FACE_OUTER_BOUND('',#4695,.T.);
#3469=FACE_OUTER_BOUND('',#4696,.T.);
#3470=FACE_OUTER_BOUND('',#4697,.T.);
#3471=FACE_OUTER_BOUND('',#4698,.T.);
#3472=FACE_OUTER_BOUND('',#4699,.T.);
#3473=FACE_OUTER_BOUND('',#4700,.T.);
#3474=FACE_OUTER_BOUND('',#4701,.T.);
#3475=FACE_OUTER_BOUND('',#4702,.T.);
#3476=FACE_OUTER_BOUND('',#4703,.T.);
#3477=FACE_OUTER_BOUND('',#4704,.T.);
#3478=FACE_OUTER_BOUND('',#4705,.T.);
#3479=FACE_OUTER_BOUND('',#4706,.T.);
#3480=FACE_OUTER_BOUND('',#4707,.T.);
#3481=FACE_OUTER_BOUND('',#4708,.T.);
#3482=FACE_OUTER_BOUND('',#4709,.T.);
#3483=FACE_OUTER_BOUND('',#4710,.T.);
#3484=FACE_OUTER_BOUND('',#4711,.T.);
#3485=FACE_OUTER_BOUND('',#4712,.T.);
#3486=FACE_OUTER_BOUND('',#4713,.T.);
#3487=FACE_OUTER_BOUND('',#4714,.T.);
#3488=FACE_OUTER_BOUND('',#4715,.T.);
#3489=FACE_OUTER_BOUND('',#4716,.T.);
#3490=FACE_OUTER_BOUND('',#4717,.T.);
#3491=FACE_OUTER_BOUND('',#4718,.T.);
#3492=FACE_OUTER_BOUND('',#4719,.T.);
#3493=FACE_OUTER_BOUND('',#4720,.T.);
#3494=FACE_OUTER_BOUND('',#4721,.T.);
#3495=FACE_OUTER_BOUND('',#4722,.T.);
#3496=FACE_OUTER_BOUND('',#4723,.T.);
#3497=FACE_OUTER_BOUND('',#4724,.T.);
#3498=FACE_OUTER_BOUND('',#4725,.T.);
#3499=FACE_OUTER_BOUND('',#4726,.T.);
#3500=FACE_OUTER_BOUND('',#4727,.T.);
#3501=FACE_OUTER_BOUND('',#4728,.T.);
#3502=FACE_OUTER_BOUND('',#4729,.T.);
#3503=FACE_OUTER_BOUND('',#4730,.T.);
#3504=FACE_OUTER_BOUND('',#4731,.T.);
#3505=FACE_OUTER_BOUND('',#4732,.T.);
#3506=FACE_OUTER_BOUND('',#4733,.T.);
#3507=FACE_OUTER_BOUND('',#4734,.T.);
#3508=FACE_OUTER_BOUND('',#4735,.T.);
#3509=FACE_OUTER_BOUND('',#4736,.T.);
#3510=FACE_OUTER_BOUND('',#4737,.T.);
#3511=FACE_OUTER_BOUND('',#4738,.T.);
#3512=FACE_OUTER_BOUND('',#4739,.T.);
#3513=FACE_OUTER_BOUND('',#4740,.T.);
#3514=FACE_OUTER_BOUND('',#4741,.T.);
#3515=FACE_OUTER_BOUND('',#4742,.T.);
#3516=FACE_OUTER_BOUND('',#4743,.T.);
#3517=FACE_OUTER_BOUND('',#4744,.T.);
#3518=FACE_OUTER_BOUND('',#4745,.T.);
#3519=FACE_OUTER_BOUND('',#4746,.T.);
#3520=FACE_OUTER_BOUND('',#4747,.T.);
#3521=FACE_OUTER_BOUND('',#4748,.T.);
#3522=FACE_OUTER_BOUND('',#4749,.T.);
#3523=FACE_OUTER_BOUND('',#4750,.T.);
#3524=FACE_OUTER_BOUND('',#4751,.T.);
#3525=FACE_OUTER_BOUND('',#4752,.T.);
#3526=FACE_OUTER_BOUND('',#4753,.T.);
#3527=FACE_OUTER_BOUND('',#4754,.T.);
#3528=FACE_OUTER_BOUND('',#4755,.T.);
#3529=FACE_OUTER_BOUND('',#4756,.T.);
#3530=FACE_OUTER_BOUND('',#4757,.T.);
#3531=FACE_OUTER_BOUND('',#4758,.T.);
#3532=FACE_OUTER_BOUND('',#4759,.T.);
#3533=FACE_OUTER_BOUND('',#4760,.T.);
#3534=FACE_OUTER_BOUND('',#4761,.T.);
#3535=FACE_OUTER_BOUND('',#4762,.T.);
#3536=FACE_OUTER_BOUND('',#4763,.T.);
#3537=FACE_OUTER_BOUND('',#4764,.T.);
#3538=FACE_OUTER_BOUND('',#4765,.T.);
#3539=FACE_OUTER_BOUND('',#4766,.T.);
#3540=FACE_OUTER_BOUND('',#4767,.T.);
#3541=FACE_OUTER_BOUND('',#4768,.T.);
#3542=FACE_OUTER_BOUND('',#4769,.T.);
#3543=FACE_OUTER_BOUND('',#4776,.T.);
#3544=FACE_OUTER_BOUND('',#4777,.T.);
#3545=FACE_OUTER_BOUND('',#4778,.T.);
#3546=FACE_OUTER_BOUND('',#4779,.T.);
#3547=FACE_OUTER_BOUND('',#4780,.T.);
#3548=FACE_OUTER_BOUND('',#4781,.T.);
#3549=FACE_OUTER_BOUND('',#4782,.T.);
#3550=FACE_OUTER_BOUND('',#4783,.T.);
#3551=FACE_OUTER_BOUND('',#4784,.T.);
#3552=FACE_OUTER_BOUND('',#4785,.T.);
#3553=FACE_OUTER_BOUND('',#4786,.T.);
#3554=FACE_OUTER_BOUND('',#4787,.T.);
#3555=FACE_OUTER_BOUND('',#4788,.T.);
#3556=FACE_OUTER_BOUND('',#4789,.T.);
#3557=FACE_OUTER_BOUND('',#4790,.T.);
#3558=FACE_OUTER_BOUND('',#4791,.T.);
#3559=FACE_OUTER_BOUND('',#4792,.T.);
#3560=FACE_OUTER_BOUND('',#4793,.T.);
#3561=FACE_OUTER_BOUND('',#4794,.T.);
#3562=FACE_OUTER_BOUND('',#4795,.T.);
#3563=FACE_OUTER_BOUND('',#4796,.T.);
#3564=FACE_OUTER_BOUND('',#4797,.T.);
#3565=FACE_OUTER_BOUND('',#4798,.T.);
#3566=FACE_OUTER_BOUND('',#4799,.T.);
#3567=FACE_OUTER_BOUND('',#4800,.T.);
#3568=FACE_OUTER_BOUND('',#4801,.T.);
#4526=EDGE_LOOP('',(#17418,#17419,#17420,#17421));
#4527=EDGE_LOOP('',(#17422,#17423,#17424,#17425));
#4528=EDGE_LOOP('',(#17426,#17427,#17428,#17429));
#4529=EDGE_LOOP('',(#17430,#17431,#17432,#17433));
#4530=EDGE_LOOP('',(#17434,#17435,#17436,#17437));
#4531=EDGE_LOOP('',(#17438,#17439,#17440,#17441));
#4532=EDGE_LOOP('',(#17442,#17443,#17444,#17445));
#4533=EDGE_LOOP('',(#17446,#17447,#17448,#17449));
#4534=EDGE_LOOP('',(#17450,#17451,#17452,#17453));
#4535=EDGE_LOOP('',(#17454,#17455,#17456,#17457));
#4536=EDGE_LOOP('',(#17458,#17459,#17460,#17461));
#4537=EDGE_LOOP('',(#17462,#17463,#17464,#17465));
#4538=EDGE_LOOP('',(#17466,#17467,#17468,#17469));
#4539=EDGE_LOOP('',(#17470,#17471,#17472,#17473));
#4540=EDGE_LOOP('',(#17474,#17475,#17476,#17477));
#4541=EDGE_LOOP('',(#17478,#17479,#17480,#17481));
#4542=EDGE_LOOP('',(#17482,#17483,#17484,#17485));
#4543=EDGE_LOOP('',(#17486,#17487,#17488,#17489));
#4544=EDGE_LOOP('',(#17490,#17491,#17492,#17493));
#4545=EDGE_LOOP('',(#17494,#17495,#17496,#17497));
#4546=EDGE_LOOP('',(#17498,#17499,#17500,#17501));
#4547=EDGE_LOOP('',(#17502,#17503,#17504,#17505));
#4548=EDGE_LOOP('',(#17506,#17507,#17508,#17509));
#4549=EDGE_LOOP('',(#17510,#17511,#17512,#17513));
#4550=EDGE_LOOP('',(#17514,#17515,#17516,#17517));
#4551=EDGE_LOOP('',(#17518,#17519,#17520,#17521));
#4552=EDGE_LOOP('',(#17522,#17523,#17524,#17525));
#4553=EDGE_LOOP('',(#17526,#17527,#17528,#17529));
#4554=EDGE_LOOP('',(#17530,#17531,#17532,#17533));
#4555=EDGE_LOOP('',(#17534,#17535,#17536,#17537));
#4556=EDGE_LOOP('',(#17538,#17539,#17540,#17541));
#4557=EDGE_LOOP('',(#17542,#17543,#17544,#17545));
#4558=EDGE_LOOP('',(#17546,#17547,#17548,#17549));
#4559=EDGE_LOOP('',(#17550,#17551,#17552,#17553));
#4560=EDGE_LOOP('',(#17554,#17555,#17556,#17557));
#4561=EDGE_LOOP('',(#17558,#17559,#17560,#17561));
#4562=EDGE_LOOP('',(#17562,#17563,#17564,#17565));
#4563=EDGE_LOOP('',(#17566,#17567,#17568,#17569));
#4564=EDGE_LOOP('',(#17570,#17571,#17572,#17573));
#4565=EDGE_LOOP('',(#17574,#17575,#17576,#17577));
#4566=EDGE_LOOP('',(#17578,#17579,#17580,#17581));
#4567=EDGE_LOOP('',(#17582,#17583,#17584,#17585));
#4568=EDGE_LOOP('',(#17586,#17587,#17588,#17589));
#4569=EDGE_LOOP('',(#17590,#17591,#17592,#17593));
#4570=EDGE_LOOP('',(#17594,#17595,#17596,#17597));
#4571=EDGE_LOOP('',(#17598,#17599,#17600,#17601));
#4572=EDGE_LOOP('',(#17602,#17603,#17604,#17605));
#4573=EDGE_LOOP('',(#17606,#17607,#17608,#17609));
#4574=EDGE_LOOP('',(#17610,#17611,#17612,#17613));
#4575=EDGE_LOOP('',(#17614,#17615,#17616,#17617));
#4576=EDGE_LOOP('',(#17618,#17619,#17620,#17621));
#4577=EDGE_LOOP('',(#17622,#17623,#17624,#17625));
#4578=EDGE_LOOP('',(#17626,#17627,#17628,#17629));
#4579=EDGE_LOOP('',(#17630,#17631,#17632,#17633));
#4580=EDGE_LOOP('',(#17634,#17635,#17636,#17637));
#4581=EDGE_LOOP('',(#17638,#17639,#17640,#17641));
#4582=EDGE_LOOP('',(#17642,#17643,#17644,#17645));
#4583=EDGE_LOOP('',(#17646,#17647,#17648,#17649));
#4584=EDGE_LOOP('',(#17650,#17651,#17652,#17653));
#4585=EDGE_LOOP('',(#17654,#17655,#17656,#17657));
#4586=EDGE_LOOP('',(#17658,#17659,#17660,#17661));
#4587=EDGE_LOOP('',(#17662,#17663,#17664,#17665));
#4588=EDGE_LOOP('',(#17666,#17667,#17668,#17669));
#4589=EDGE_LOOP('',(#17670,#17671,#17672,#17673));
#4590=EDGE_LOOP('',(#17674,#17675,#17676,#17677));
#4591=EDGE_LOOP('',(#17678,#17679,#17680,#17681));
#4592=EDGE_LOOP('',(#17682,#17683,#17684,#17685));
#4593=EDGE_LOOP('',(#17686,#17687,#17688,#17689));
#4594=EDGE_LOOP('',(#17690,#17691,#17692,#17693));
#4595=EDGE_LOOP('',(#17694,#17695,#17696,#17697));
#4596=EDGE_LOOP('',(#17698,#17699,#17700,#17701));
#4597=EDGE_LOOP('',(#17702,#17703,#17704,#17705));
#4598=EDGE_LOOP('',(#17706,#17707,#17708,#17709));
#4599=EDGE_LOOP('',(#17710,#17711,#17712,#17713));
#4600=EDGE_LOOP('',(#17714,#17715,#17716,#17717));
#4601=EDGE_LOOP('',(#17718,#17719,#17720,#17721));
#4602=EDGE_LOOP('',(#17722,#17723,#17724,#17725));
#4603=EDGE_LOOP('',(#17726,#17727,#17728,#17729));
#4604=EDGE_LOOP('',(#17730,#17731,#17732,#17733));
#4605=EDGE_LOOP('',(#17734,#17735,#17736,#17737));
#4606=EDGE_LOOP('',(#17738,#17739,#17740,#17741));
#4607=EDGE_LOOP('',(#17742,#17743,#17744,#17745));
#4608=EDGE_LOOP('',(#17746,#17747,#17748,#17749));
#4609=EDGE_LOOP('',(#17750,#17751,#17752,#17753));
#4610=EDGE_LOOP('',(#17754,#17755,#17756,#17757));
#4611=EDGE_LOOP('',(#17758,#17759,#17760,#17761));
#4612=EDGE_LOOP('',(#17762,#17763,#17764,#17765));
#4613=EDGE_LOOP('',(#17766,#17767,#17768,#17769));
#4614=EDGE_LOOP('',(#17770,#17771,#17772,#17773));
#4615=EDGE_LOOP('',(#17774,#17775,#17776,#17777));
#4616=EDGE_LOOP('',(#17778,#17779,#17780,#17781));
#4617=EDGE_LOOP('',(#17782,#17783,#17784,#17785));
#4618=EDGE_LOOP('',(#17786,#17787,#17788,#17789));
#4619=EDGE_LOOP('',(#17790,#17791,#17792,#17793));
#4620=EDGE_LOOP('',(#17794,#17795,#17796,#17797));
#4621=EDGE_LOOP('',(#17798,#17799,#17800,#17801));
#4622=EDGE_LOOP('',(#17802,#17803,#17804,#17805));
#4623=EDGE_LOOP('',(#17806,#17807,#17808,#17809));
#4624=EDGE_LOOP('',(#17810,#17811,#17812,#17813));
#4625=EDGE_LOOP('',(#17814,#17815,#17816,#17817));
#4626=EDGE_LOOP('',(#17818,#17819,#17820,#17821));
#4627=EDGE_LOOP('',(#17822,#17823,#17824,#17825));
#4628=EDGE_LOOP('',(#17826,#17827,#17828,#17829));
#4629=EDGE_LOOP('',(#17830,#17831,#17832,#17833));
#4630=EDGE_LOOP('',(#17834,#17835,#17836,#17837));
#4631=EDGE_LOOP('',(#17838,#17839,#17840,#17841));
#4632=EDGE_LOOP('',(#17842,#17843,#17844,#17845));
#4633=EDGE_LOOP('',(#17846,#17847,#17848,#17849));
#4634=EDGE_LOOP('',(#17850,#17851,#17852,#17853));
#4635=EDGE_LOOP('',(#17854,#17855,#17856,#17857));
#4636=EDGE_LOOP('',(#17858,#17859,#17860,#17861));
#4637=EDGE_LOOP('',(#17862,#17863,#17864,#17865));
#4638=EDGE_LOOP('',(#17866,#17867,#17868,#17869));
#4639=EDGE_LOOP('',(#17870,#17871,#17872,#17873));
#4640=EDGE_LOOP('',(#17874,#17875,#17876,#17877));
#4641=EDGE_LOOP('',(#17878,#17879,#17880,#17881));
#4642=EDGE_LOOP('',(#17882,#17883,#17884,#17885));
#4643=EDGE_LOOP('',(#17886,#17887,#17888,#17889));
#4644=EDGE_LOOP('',(#17890,#17891,#17892,#17893));
#4645=EDGE_LOOP('',(#17894,#17895,#17896,#17897));
#4646=EDGE_LOOP('',(#17898,#17899,#17900,#17901));
#4647=EDGE_LOOP('',(#17902,#17903,#17904,#17905));
#4648=EDGE_LOOP('',(#17906,#17907,#17908,#17909));
#4649=EDGE_LOOP('',(#17910,#17911,#17912,#17913));
#4650=EDGE_LOOP('',(#17914,#17915,#17916,#17917));
#4651=EDGE_LOOP('',(#17918,#17919,#17920,#17921));
#4652=EDGE_LOOP('',(#17922,#17923,#17924,#17925));
#4653=EDGE_LOOP('',(#17926,#17927,#17928,#17929));
#4654=EDGE_LOOP('',(#17930,#17931,#17932,#17933));
#4655=EDGE_LOOP('',(#17934,#17935,#17936,#17937));
#4656=EDGE_LOOP('',(#17938,#17939,#17940,#17941));
#4657=EDGE_LOOP('',(#17942,#17943,#17944,#17945));
#4658=EDGE_LOOP('',(#17946,#17947,#17948,#17949));
#4659=EDGE_LOOP('',(#17950,#17951,#17952,#17953));
#4660=EDGE_LOOP('',(#17954,#17955,#17956,#17957));
#4661=EDGE_LOOP('',(#17958,#17959,#17960,#17961));
#4662=EDGE_LOOP('',(#17962,#17963,#17964,#17965));
#4663=EDGE_LOOP('',(#17966,#17967,#17968,#17969));
#4664=EDGE_LOOP('',(#17970,#17971,#17972,#17973));
#4665=EDGE_LOOP('',(#17974,#17975,#17976,#17977));
#4666=EDGE_LOOP('',(#17978,#17979,#17980,#17981));
#4667=EDGE_LOOP('',(#17982,#17983,#17984,#17985));
#4668=EDGE_LOOP('',(#17986,#17987,#17988,#17989));
#4669=EDGE_LOOP('',(#17990,#17991,#17992,#17993));
#4670=EDGE_LOOP('',(#17994,#17995,#17996,#17997));
#4671=EDGE_LOOP('',(#17998,#17999,#18000,#18001));
#4672=EDGE_LOOP('',(#18002,#18003,#18004,#18005));
#4673=EDGE_LOOP('',(#18006,#18007,#18008,#18009));
#4674=EDGE_LOOP('',(#18010,#18011,#18012,#18013));
#4675=EDGE_LOOP('',(#18014,#18015,#18016,#18017));
#4676=EDGE_LOOP('',(#18018,#18019,#18020,#18021));
#4677=EDGE_LOOP('',(#18022,#18023,#18024,#18025));
#4678=EDGE_LOOP('',(#18026,#18027,#18028,#18029));
#4679=EDGE_LOOP('',(#18030,#18031,#18032,#18033));
#4680=EDGE_LOOP('',(#18034,#18035,#18036,#18037));
#4681=EDGE_LOOP('',(#18038,#18039,#18040,#18041));
#4682=EDGE_LOOP('',(#18042,#18043,#18044,#18045));
#4683=EDGE_LOOP('',(#18046,#18047,#18048,#18049));
#4684=EDGE_LOOP('',(#18050,#18051,#18052,#18053));
#4685=EDGE_LOOP('',(#18054,#18055,#18056,#18057));
#4686=EDGE_LOOP('',(#18058,#18059,#18060,#18061));
#4687=EDGE_LOOP('',(#18062,#18063,#18064,#18065));
#4688=EDGE_LOOP('',(#18066,#18067,#18068,#18069));
#4689=EDGE_LOOP('',(#18070,#18071,#18072,#18073));
#4690=EDGE_LOOP('',(#18074,#18075,#18076,#18077));
#4691=EDGE_LOOP('',(#18078,#18079,#18080,#18081));
#4692=EDGE_LOOP('',(#18082,#18083,#18084,#18085));
#4693=EDGE_LOOP('',(#18086,#18087,#18088,#18089));
#4694=EDGE_LOOP('',(#18090,#18091,#18092,#18093));
#4695=EDGE_LOOP('',(#18094,#18095,#18096,#18097));
#4696=EDGE_LOOP('',(#18098,#18099,#18100,#18101));
#4697=EDGE_LOOP('',(#18102,#18103,#18104,#18105));
#4698=EDGE_LOOP('',(#18106,#18107,#18108,#18109));
#4699=EDGE_LOOP('',(#18110,#18111,#18112,#18113));
#4700=EDGE_LOOP('',(#18114,#18115,#18116,#18117));
#4701=EDGE_LOOP('',(#18118,#18119,#18120,#18121));
#4702=EDGE_LOOP('',(#18122,#18123,#18124,#18125));
#4703=EDGE_LOOP('',(#18126,#18127,#18128,#18129));
#4704=EDGE_LOOP('',(#18130,#18131,#18132,#18133));
#4705=EDGE_LOOP('',(#18134,#18135,#18136,#18137));
#4706=EDGE_LOOP('',(#18138,#18139,#18140,#18141));
#4707=EDGE_LOOP('',(#18142,#18143,#18144,#18145));
#4708=EDGE_LOOP('',(#18146,#18147,#18148,#18149));
#4709=EDGE_LOOP('',(#18150,#18151,#18152,#18153));
#4710=EDGE_LOOP('',(#18154,#18155,#18156,#18157));
#4711=EDGE_LOOP('',(#18158,#18159,#18160,#18161));
#4712=EDGE_LOOP('',(#18162,#18163,#18164,#18165));
#4713=EDGE_LOOP('',(#18166,#18167,#18168,#18169));
#4714=EDGE_LOOP('',(#18170,#18171,#18172,#18173));
#4715=EDGE_LOOP('',(#18174,#18175,#18176,#18177));
#4716=EDGE_LOOP('',(#18178,#18179,#18180,#18181));
#4717=EDGE_LOOP('',(#18182,#18183,#18184,#18185));
#4718=EDGE_LOOP('',(#18186,#18187,#18188,#18189));
#4719=EDGE_LOOP('',(#18190,#18191,#18192,#18193));
#4720=EDGE_LOOP('',(#18194,#18195,#18196,#18197));
#4721=EDGE_LOOP('',(#18198,#18199,#18200,#18201));
#4722=EDGE_LOOP('',(#18202,#18203,#18204,#18205));
#4723=EDGE_LOOP('',(#18206,#18207,#18208,#18209));
#4724=EDGE_LOOP('',(#18210,#18211,#18212,#18213));
#4725=EDGE_LOOP('',(#18214,#18215,#18216,#18217));
#4726=EDGE_LOOP('',(#18218,#18219,#18220,#18221));
#4727=EDGE_LOOP('',(#18222,#18223,#18224,#18225));
#4728=EDGE_LOOP('',(#18226,#18227,#18228,#18229));
#4729=EDGE_LOOP('',(#18230,#18231,#18232,#18233));
#4730=EDGE_LOOP('',(#18234,#18235,#18236,#18237));
#4731=EDGE_LOOP('',(#18238,#18239,#18240,#18241));
#4732=EDGE_LOOP('',(#18242,#18243,#18244,#18245));
#4733=EDGE_LOOP('',(#18246,#18247,#18248,#18249));
#4734=EDGE_LOOP('',(#18250,#18251,#18252,#18253));
#4735=EDGE_LOOP('',(#18254,#18255,#18256,#18257));
#4736=EDGE_LOOP('',(#18258,#18259,#18260,#18261));
#4737=EDGE_LOOP('',(#18262,#18263,#18264,#18265));
#4738=EDGE_LOOP('',(#18266,#18267,#18268,#18269));
#4739=EDGE_LOOP('',(#18270,#18271,#18272,#18273));
#4740=EDGE_LOOP('',(#18274,#18275,#18276,#18277));
#4741=EDGE_LOOP('',(#18278,#18279,#18280,#18281));
#4742=EDGE_LOOP('',(#18282,#18283,#18284,#18285));
#4743=EDGE_LOOP('',(#18286,#18287,#18288,#18289));
#4744=EDGE_LOOP('',(#18290,#18291,#18292,#18293));
#4745=EDGE_LOOP('',(#18294,#18295,#18296,#18297));
#4746=EDGE_LOOP('',(#18298,#18299,#18300,#18301));
#4747=EDGE_LOOP('',(#18302,#18303,#18304,#18305));
#4748=EDGE_LOOP('',(#18306,#18307,#18308,#18309));
#4749=EDGE_LOOP('',(#18310,#18311,#18312,#18313));
#4750=EDGE_LOOP('',(#18314,#18315,#18316,#18317));
#4751=EDGE_LOOP('',(#18318,#18319,#18320,#18321));
#4752=EDGE_LOOP('',(#18322,#18323,#18324,#18325));
#4753=EDGE_LOOP('',(#18326,#18327,#18328,#18329));
#4754=EDGE_LOOP('',(#18330,#18331,#18332,#18333));
#4755=EDGE_LOOP('',(#18334,#18335,#18336,#18337));
#4756=EDGE_LOOP('',(#18338,#18339,#18340,#18341));
#4757=EDGE_LOOP('',(#18342,#18343,#18344,#18345));
#4758=EDGE_LOOP('',(#18346,#18347,#18348,#18349));
#4759=EDGE_LOOP('',(#18350,#18351,#18352,#18353));
#4760=EDGE_LOOP('',(#18354,#18355,#18356,#18357));
#4761=EDGE_LOOP('',(#18358,#18359,#18360,#18361));
#4762=EDGE_LOOP('',(#18362,#18363,#18364,#18365));
#4763=EDGE_LOOP('',(#18366,#18367,#18368,#18369));
#4764=EDGE_LOOP('',(#18370,#18371,#18372,#18373));
#4765=EDGE_LOOP('',(#18374,#18375,#18376,#18377));
#4766=EDGE_LOOP('',(#18378,#18379,#18380,#18381));
#4767=EDGE_LOOP('',(#18382,#18383,#18384,#18385,#18386,#18387,#18388,#18389,
#18390,#18391,#18392,#18393,#18394,#18395,#18396,#18397,#18398,#18399,#18400,
#18401,#18402,#18403,#18404,#18405,#18406,#18407,#18408,#18409,#18410,#18411,
#18412,#18413,#18414,#18415,#18416,#18417,#18418,#18419,#18420,#18421,#18422,
#18423,#18424,#18425));
#4768=EDGE_LOOP('',(#18426,#18427,#18428,#18429,#18430,#18431,#18432,#18433,
#18434,#18435,#18436,#18437,#18438,#18439,#18440,#18441,#18442,#18443,#18444,
#18445,#18446,#18447,#18448,#18449,#18450,#18451,#18452,#18453,#18454,#18455,
#18456,#18457,#18458,#18459,#18460,#18461,#18462,#18463,#18464,#18465,#18466,
#18467,#18468,#18469));
#4769=EDGE_LOOP('',(#18470,#18471,#18472,#18473));
#4770=EDGE_LOOP('',(#18474,#18475,#18476,#18477));
#4771=EDGE_LOOP('',(#18478,#18479,#18480,#18481));
#4772=EDGE_LOOP('',(#18482,#18483,#18484,#18485));
#4773=EDGE_LOOP('',(#18486,#18487,#18488,#18489));
#4774=EDGE_LOOP('',(#18490,#18491,#18492,#18493));
#4775=EDGE_LOOP('',(#18494,#18495,#18496,#18497));
#4776=EDGE_LOOP('',(#18498,#18499,#18500,#18501));
#4777=EDGE_LOOP('',(#18502,#18503,#18504,#18505,#18506,#18507,#18508,#18509,
#18510,#18511,#18512,#18513,#18514,#18515,#18516,#18517,#18518,#18519,#18520,
#18521,#18522,#18523,#18524,#18525,#18526,#18527,#18528,#18529,#18530,#18531,
#18532,#18533,#18534,#18535,#18536,#18537,#18538,#18539,#18540,#18541,#18542,
#18543,#18544,#18545));
#4778=EDGE_LOOP('',(#18546,#18547,#18548,#18549,#18550,#18551,#18552,#18553,
#18554,#18555,#18556,#18557,#18558,#18559,#18560,#18561,#18562,#18563,#18564,
#18565,#18566,#18567,#18568,#18569,#18570,#18571,#18572,#18573,#18574,#18575,
#18576,#18577,#18578,#18579,#18580,#18581,#18582,#18583,#18584,#18585,#18586,
#18587,#18588,#18589));
#4779=EDGE_LOOP('',(#18590,#18591,#18592,#18593));
#4780=EDGE_LOOP('',(#18594,#18595,#18596,#18597,#18598,#18599,#18600,#18601,
#18602,#18603,#18604,#18605,#18606,#18607,#18608,#18609,#18610,#18611,#18612,
#18613,#18614,#18615,#18616,#18617,#18618,#18619,#18620,#18621,#18622,#18623,
#18624,#18625,#18626,#18627,#18628,#18629,#18630,#18631,#18632,#18633,#18634,
#18635,#18636,#18637));
#4781=EDGE_LOOP('',(#18638,#18639,#18640,#18641,#18642,#18643,#18644,#18645,
#18646,#18647,#18648,#18649,#18650,#18651,#18652,#18653,#18654,#18655,#18656,
#18657,#18658,#18659,#18660,#18661,#18662,#18663,#18664,#18665,#18666,#18667,
#18668,#18669,#18670,#18671,#18672,#18673,#18674,#18675,#18676,#18677,#18678,
#18679,#18680,#18681));
#4782=EDGE_LOOP('',(#18682,#18683,#18684,#18685));
#4783=EDGE_LOOP('',(#18686,#18687,#18688,#18689,#18690,#18691,#18692,#18693,
#18694,#18695,#18696,#18697,#18698,#18699,#18700,#18701,#18702,#18703,#18704,
#18705,#18706,#18707,#18708,#18709,#18710,#18711,#18712,#18713,#18714,#18715,
#18716,#18717,#18718,#18719,#18720,#18721,#18722,#18723,#18724,#18725,#18726,
#18727,#18728,#18729));
#4784=EDGE_LOOP('',(#18730,#18731,#18732,#18733,#18734,#18735,#18736,#18737,
#18738,#18739,#18740,#18741,#18742,#18743,#18744,#18745,#18746,#18747,#18748,
#18749,#18750,#18751,#18752,#18753,#18754,#18755,#18756,#18757,#18758,#18759,
#18760,#18761,#18762,#18763,#18764,#18765,#18766,#18767,#18768,#18769,#18770,
#18771,#18772,#18773));
#4785=EDGE_LOOP('',(#18774,#18775,#18776,#18777));
#4786=EDGE_LOOP('',(#18778,#18779,#18780,#18781,#18782,#18783,#18784,#18785,
#18786,#18787,#18788,#18789,#18790,#18791,#18792,#18793,#18794,#18795,#18796,
#18797,#18798,#18799,#18800,#18801,#18802,#18803,#18804,#18805,#18806,#18807,
#18808,#18809,#18810,#18811,#18812,#18813,#18814,#18815,#18816,#18817,#18818,
#18819,#18820,#18821));
#4787=EDGE_LOOP('',(#18822,#18823,#18824,#18825,#18826,#18827,#18828,#18829,
#18830,#18831,#18832,#18833,#18834,#18835,#18836,#18837,#18838,#18839,#18840,
#18841,#18842,#18843,#18844,#18845,#18846,#18847,#18848,#18849,#18850,#18851,
#18852,#18853,#18854,#18855,#18856,#18857,#18858,#18859,#18860,#18861,#18862,
#18863,#18864,#18865));
#4788=EDGE_LOOP('',(#18866,#18867,#18868,#18869));
#4789=EDGE_LOOP('',(#18870,#18871,#18872,#18873,#18874,#18875,#18876,#18877,
#18878,#18879,#18880,#18881,#18882,#18883,#18884,#18885,#18886,#18887,#18888,
#18889,#18890,#18891,#18892,#18893,#18894,#18895,#18896,#18897,#18898,#18899,
#18900,#18901,#18902,#18903,#18904,#18905,#18906,#18907,#18908,#18909,#18910,
#18911,#18912,#18913));
#4790=EDGE_LOOP('',(#18914,#18915,#18916,#18917,#18918,#18919,#18920,#18921,
#18922,#18923,#18924,#18925,#18926,#18927,#18928,#18929,#18930,#18931,#18932,
#18933,#18934,#18935,#18936,#18937,#18938,#18939,#18940,#18941,#18942,#18943,
#18944,#18945,#18946,#18947,#18948,#18949,#18950,#18951,#18952,#18953,#18954,
#18955,#18956,#18957));
#4791=EDGE_LOOP('',(#18958,#18959,#18960,#18961));
#4792=EDGE_LOOP('',(#18962,#18963,#18964,#18965));
#4793=EDGE_LOOP('',(#18966,#18967,#18968,#18969));
#4794=EDGE_LOOP('',(#18970,#18971,#18972,#18973));
#4795=EDGE_LOOP('',(#18974,#18975,#18976,#18977));
#4796=EDGE_LOOP('',(#18978,#18979,#18980,#18981));
#4797=EDGE_LOOP('',(#18982,#18983,#18984,#18985));
#4798=EDGE_LOOP('',(#18986,#18987,#18988,#18989));
#4799=EDGE_LOOP('',(#18990,#18991,#18992,#18993));
#4800=EDGE_LOOP('',(#18994,#18995,#18996,#18997));
#4801=EDGE_LOOP('',(#18998,#18999,#19000,#19001));
#4802=EDGE_LOOP('',(#19002,#19003,#19004,#19005));
#4803=EDGE_LOOP('',(#19006,#19007,#19008,#19009));
#4804=EDGE_LOOP('',(#19010,#19011,#19012,#19013));
#4805=EDGE_LOOP('',(#19014,#19015,#19016,#19017));
#4806=EDGE_LOOP('',(#19018,#19019,#19020,#19021));
#4807=EDGE_LOOP('',(#19022,#19023,#19024,#19025));
#5776=LINE('',#72984,#6990);
#5777=LINE('',#73005,#6991);
#5778=LINE('',#73056,#6992);
#5779=LINE('',#73107,#6993);
#5780=LINE('',#73155,#6994);
#5781=LINE('',#73203,#6995);
#5782=LINE('',#73254,#6996);
#5783=LINE('',#73305,#6997);
#5784=LINE('',#73353,#6998);
#5785=LINE('',#73404,#6999);
#5786=LINE('',#73455,#7000);
#5787=LINE('',#73503,#7001);
#5788=LINE('',#73551,#7002);
#5789=LINE('',#73605,#7003);
#5790=LINE('',#73653,#7004);
#5791=LINE('',#73701,#7005);
#5792=LINE('',#73752,#7006);
#5793=LINE('',#73803,#7007);
#5794=LINE('',#73851,#7008);
#5795=LINE('',#73902,#7009);
#5796=LINE('',#73941,#7010);
#5797=LINE('',#73962,#7011);
#5798=LINE('',#74013,#7012);
#5799=LINE('',#74064,#7013);
#5800=LINE('',#74112,#7014);
#5801=LINE('',#74160,#7015);
#5802=LINE('',#74211,#7016);
#5803=LINE('',#74262,#7017);
#5804=LINE('',#74310,#7018);
#5805=LINE('',#74361,#7019);
#5806=LINE('',#74412,#7020);
#5807=LINE('',#74460,#7021);
#5808=LINE('',#74508,#7022);
#5809=LINE('',#74562,#7023);
#5810=LINE('',#74610,#7024);
#5811=LINE('',#74658,#7025);
#5812=LINE('',#74709,#7026);
#5813=LINE('',#74760,#7027);
#5814=LINE('',#74808,#7028);
#5815=LINE('',#74859,#7029);
#5816=LINE('',#74898,#7030);
#5817=LINE('',#74919,#7031);
#5818=LINE('',#74970,#7032);
#5819=LINE('',#75021,#7033);
#5820=LINE('',#75069,#7034);
#5821=LINE('',#75117,#7035);
#5822=LINE('',#75168,#7036);
#5823=LINE('',#75219,#7037);
#5824=LINE('',#75267,#7038);
#5825=LINE('',#75318,#7039);
#5826=LINE('',#75369,#7040);
#5827=LINE('',#75417,#7041);
#5828=LINE('',#75465,#7042);
#5829=LINE('',#75519,#7043);
#5830=LINE('',#75567,#7044);
#5831=LINE('',#75615,#7045);
#5832=LINE('',#75666,#7046);
#5833=LINE('',#75717,#7047);
#5834=LINE('',#75765,#7048);
#5835=LINE('',#75816,#7049);
#5836=LINE('',#75855,#7050);
#5837=LINE('',#75876,#7051);
#5838=LINE('',#75927,#7052);
#5839=LINE('',#75978,#7053);
#5840=LINE('',#76026,#7054);
#5841=LINE('',#76074,#7055);
#5842=LINE('',#76125,#7056);
#5843=LINE('',#76176,#7057);
#5844=LINE('',#76224,#7058);
#5845=LINE('',#76275,#7059);
#5846=LINE('',#76326,#7060);
#5847=LINE('',#76374,#7061);
#5848=LINE('',#76422,#7062);
#5849=LINE('',#76476,#7063);
#5850=LINE('',#76524,#7064);
#5851=LINE('',#76572,#7065);
#5852=LINE('',#76623,#7066);
#5853=LINE('',#76674,#7067);
#5854=LINE('',#76722,#7068);
#5855=LINE('',#76773,#7069);
#5856=LINE('',#76812,#7070);
#5857=LINE('',#76833,#7071);
#5858=LINE('',#76884,#7072);
#5859=LINE('',#76935,#7073);
#5860=LINE('',#76983,#7074);
#5861=LINE('',#77031,#7075);
#5862=LINE('',#77082,#7076);
#5863=LINE('',#77133,#7077);
#5864=LINE('',#77181,#7078);
#5865=LINE('',#77232,#7079);
#5866=LINE('',#77283,#7080);
#5867=LINE('',#77331,#7081);
#5868=LINE('',#77379,#7082);
#5869=LINE('',#77433,#7083);
#5870=LINE('',#77481,#7084);
#5871=LINE('',#77529,#7085);
#5872=LINE('',#77580,#7086);
#5873=LINE('',#77631,#7087);
#5874=LINE('',#77679,#7088);
#5875=LINE('',#77730,#7089);
#5876=LINE('',#77769,#7090);
#5877=LINE('',#77790,#7091);
#5878=LINE('',#77841,#7092);
#5879=LINE('',#77892,#7093);
#5880=LINE('',#77940,#7094);
#5881=LINE('',#77988,#7095);
#5882=LINE('',#78039,#7096);
#5883=LINE('',#78090,#7097);
#5884=LINE('',#78138,#7098);
#5885=LINE('',#78189,#7099);
#5886=LINE('',#78240,#7100);
#5887=LINE('',#78288,#7101);
#5888=LINE('',#78336,#7102);
#5889=LINE('',#78390,#7103);
#5890=LINE('',#78438,#7104);
#5891=LINE('',#78486,#7105);
#5892=LINE('',#78537,#7106);
#5893=LINE('',#78588,#7107);
#5894=LINE('',#78636,#7108);
#5895=LINE('',#78687,#7109);
#5896=LINE('',#78726,#7110);
#5897=LINE('',#78750,#7111);
#5898=LINE('',#78774,#7112);
#5899=LINE('',#78799,#7113);
#5900=LINE('',#78823,#7114);
#5901=LINE('',#78848,#7115);
#5902=LINE('',#78872,#7116);
#5903=LINE('',#78897,#7117);
#5904=LINE('',#78922,#7118);
#5905=LINE('',#78946,#7119);
#5906=LINE('',#78971,#7120);
#5907=LINE('',#78995,#7121);
#5908=LINE('',#79020,#7122);
#5909=LINE('',#79045,#7123);
#5910=LINE('',#79069,#7124);
#5911=LINE('',#79094,#7125);
#5912=LINE('',#79118,#7126);
#5913=LINE('',#79143,#7127);
#5914=LINE('',#79168,#7128);
#5915=LINE('',#79192,#7129);
#5916=LINE('',#79209,#7130);
#5917=LINE('',#79233,#7131);
#5918=LINE('',#79257,#7132);
#5919=LINE('',#79282,#7133);
#5920=LINE('',#79306,#7134);
#5921=LINE('',#79331,#7135);
#5922=LINE('',#79355,#7136);
#5923=LINE('',#79380,#7137);
#5924=LINE('',#79405,#7138);
#5925=LINE('',#79429,#7139);
#5926=LINE('',#79454,#7140);
#5927=LINE('',#79478,#7141);
#5928=LINE('',#79503,#7142);
#5929=LINE('',#79528,#7143);
#5930=LINE('',#79552,#7144);
#5931=LINE('',#79577,#7145);
#5932=LINE('',#79601,#7146);
#5933=LINE('',#79626,#7147);
#5934=LINE('',#79651,#7148);
#5935=LINE('',#79675,#7149);
#5936=LINE('',#79692,#7150);
#5937=LINE('',#79716,#7151);
#5938=LINE('',#79740,#7152);
#5939=LINE('',#79765,#7153);
#5940=LINE('',#79789,#7154);
#5941=LINE('',#79814,#7155);
#5942=LINE('',#79838,#7156);
#5943=LINE('',#79863,#7157);
#5944=LINE('',#79888,#7158);
#5945=LINE('',#79912,#7159);
#5946=LINE('',#79937,#7160);
#5947=LINE('',#79961,#7161);
#5948=LINE('',#79986,#7162);
#5949=LINE('',#80011,#7163);
#5950=LINE('',#80035,#7164);
#5951=LINE('',#80060,#7165);
#5952=LINE('',#80084,#7166);
#5953=LINE('',#80109,#7167);
#5954=LINE('',#80134,#7168);
#5955=LINE('',#80158,#7169);
#5956=LINE('',#80175,#7170);
#5957=LINE('',#80199,#7171);
#5958=LINE('',#80223,#7172);
#5959=LINE('',#80248,#7173);
#5960=LINE('',#80272,#7174);
#5961=LINE('',#80297,#7175);
#5962=LINE('',#80321,#7176);
#5963=LINE('',#80346,#7177);
#5964=LINE('',#80371,#7178);
#5965=LINE('',#80395,#7179);
#5966=LINE('',#80420,#7180);
#5967=LINE('',#80444,#7181);
#5968=LINE('',#80469,#7182);
#5969=LINE('',#80494,#7183);
#5970=LINE('',#80518,#7184);
#5971=LINE('',#80543,#7185);
#5972=LINE('',#80567,#7186);
#5973=LINE('',#80592,#7187);
#5974=LINE('',#80617,#7188);
#5975=LINE('',#80641,#7189);
#5976=LINE('',#80658,#7190);
#5977=LINE('',#80682,#7191);
#5978=LINE('',#80706,#7192);
#5979=LINE('',#80731,#7193);
#5980=LINE('',#80755,#7194);
#5981=LINE('',#80780,#7195);
#5982=LINE('',#80804,#7196);
#5983=LINE('',#80829,#7197);
#5984=LINE('',#80854,#7198);
#5985=LINE('',#80878,#7199);
#5986=LINE('',#80903,#7200);
#5987=LINE('',#80927,#7201);
#5988=LINE('',#80952,#7202);
#5989=LINE('',#80977,#7203);
#5990=LINE('',#81001,#7204);
#5991=LINE('',#81026,#7205);
#5992=LINE('',#81050,#7206);
#5993=LINE('',#81075,#7207);
#5994=LINE('',#81100,#7208);
#5995=LINE('',#81124,#7209);
#5996=LINE('',#81141,#7210);
#5997=LINE('',#81165,#7211);
#5998=LINE('',#81189,#7212);
#5999=LINE('',#81214,#7213);
#6000=LINE('',#81238,#7214);
#6001=LINE('',#81263,#7215);
#6002=LINE('',#81287,#7216);
#6003=LINE('',#81312,#7217);
#6004=LINE('',#81337,#7218);
#6005=LINE('',#81361,#7219);
#6006=LINE('',#81386,#7220);
#6007=LINE('',#81410,#7221);
#6008=LINE('',#81435,#7222);
#6009=LINE('',#81460,#7223);
#6010=LINE('',#81484,#7224);
#6011=LINE('',#81509,#7225);
#6012=LINE('',#81533,#7226);
#6013=LINE('',#81558,#7227);
#6014=LINE('',#81583,#7228);
#6015=LINE('',#81607,#7229);
#6016=LINE('',#83117,#7230);
#6017=LINE('',#83119,#7231);
#6018=LINE('',#83121,#7232);
#6019=LINE('',#83122,#7233);
#6020=LINE('',#90597,#7234);
#6021=LINE('',#90598,#7235);
#6022=LINE('',#90599,#7236);
#6023=LINE('',#90602,#7237);
#6024=LINE('',#90603,#7238);
#6025=LINE('',#90606,#7239);
#6026=LINE('',#90607,#7240);
#6027=LINE('',#90609,#7241);
#6990=VECTOR('',#26350,3.);
#6991=VECTOR('',#26355,3.);
#6992=VECTOR('',#26358,3.);
#6993=VECTOR('',#26361,3.);
#6994=VECTOR('',#26364,3.);
#6995=VECTOR('',#26367,3.);
#6996=VECTOR('',#26370,3.);
#6997=VECTOR('',#26373,3.);
#6998=VECTOR('',#26376,3.);
#6999=VECTOR('',#26379,3.);
#7000=VECTOR('',#26382,3.);
#7001=VECTOR('',#26385,3.);
#7002=VECTOR('',#26388,3.);
#7003=VECTOR('',#26391,3.);
#7004=VECTOR('',#26394,3.);
#7005=VECTOR('',#26397,3.);
#7006=VECTOR('',#26400,3.);
#7007=VECTOR('',#26403,3.);
#7008=VECTOR('',#26406,3.);
#7009=VECTOR('',#26409,3.);
#7010=VECTOR('',#26414,3.);
#7011=VECTOR('',#26419,3.);
#7012=VECTOR('',#26422,3.);
#7013=VECTOR('',#26425,3.);
#7014=VECTOR('',#26428,3.);
#7015=VECTOR('',#26431,3.);
#7016=VECTOR('',#26434,3.);
#7017=VECTOR('',#26437,3.);
#7018=VECTOR('',#26440,3.);
#7019=VECTOR('',#26443,3.);
#7020=VECTOR('',#26446,3.);
#7021=VECTOR('',#26449,3.);
#7022=VECTOR('',#26452,3.);
#7023=VECTOR('',#26455,3.);
#7024=VECTOR('',#26458,3.);
#7025=VECTOR('',#26461,3.);
#7026=VECTOR('',#26464,3.);
#7027=VECTOR('',#26467,3.);
#7028=VECTOR('',#26470,3.);
#7029=VECTOR('',#26473,3.);
#7030=VECTOR('',#26478,3.);
#7031=VECTOR('',#26483,3.);
#7032=VECTOR('',#26486,3.);
#7033=VECTOR('',#26489,3.);
#7034=VECTOR('',#26492,3.);
#7035=VECTOR('',#26495,3.);
#7036=VECTOR('',#26498,3.);
#7037=VECTOR('',#26501,3.);
#7038=VECTOR('',#26504,3.);
#7039=VECTOR('',#26507,3.);
#7040=VECTOR('',#26510,3.);
#7041=VECTOR('',#26513,3.);
#7042=VECTOR('',#26516,3.);
#7043=VECTOR('',#26519,3.);
#7044=VECTOR('',#26522,3.);
#7045=VECTOR('',#26525,3.);
#7046=VECTOR('',#26528,3.);
#7047=VECTOR('',#26531,3.);
#7048=VECTOR('',#26534,3.);
#7049=VECTOR('',#26537,3.);
#7050=VECTOR('',#26542,3.);
#7051=VECTOR('',#26547,3.);
#7052=VECTOR('',#26550,3.);
#7053=VECTOR('',#26553,3.);
#7054=VECTOR('',#26556,3.);
#7055=VECTOR('',#26559,3.);
#7056=VECTOR('',#26562,3.);
#7057=VECTOR('',#26565,3.);
#7058=VECTOR('',#26568,3.);
#7059=VECTOR('',#26571,3.);
#7060=VECTOR('',#26574,3.);
#7061=VECTOR('',#26577,3.);
#7062=VECTOR('',#26580,3.);
#7063=VECTOR('',#26583,3.);
#7064=VECTOR('',#26586,3.);
#7065=VECTOR('',#26589,3.);
#7066=VECTOR('',#26592,3.);
#7067=VECTOR('',#26595,3.);
#7068=VECTOR('',#26598,3.);
#7069=VECTOR('',#26601,3.);
#7070=VECTOR('',#26606,3.);
#7071=VECTOR('',#26611,3.);
#7072=VECTOR('',#26614,3.);
#7073=VECTOR('',#26617,3.);
#7074=VECTOR('',#26620,3.);
#7075=VECTOR('',#26623,3.);
#7076=VECTOR('',#26626,3.);
#7077=VECTOR('',#26629,3.);
#7078=VECTOR('',#26632,3.);
#7079=VECTOR('',#26635,3.);
#7080=VECTOR('',#26638,3.);
#7081=VECTOR('',#26641,3.);
#7082=VECTOR('',#26644,3.);
#7083=VECTOR('',#26647,3.);
#7084=VECTOR('',#26650,3.);
#7085=VECTOR('',#26653,3.);
#7086=VECTOR('',#26656,3.);
#7087=VECTOR('',#26659,3.);
#7088=VECTOR('',#26662,3.);
#7089=VECTOR('',#26665,3.);
#7090=VECTOR('',#26670,3.);
#7091=VECTOR('',#26675,3.);
#7092=VECTOR('',#26678,3.);
#7093=VECTOR('',#26681,3.);
#7094=VECTOR('',#26684,3.);
#7095=VECTOR('',#26687,3.);
#7096=VECTOR('',#26690,3.);
#7097=VECTOR('',#26693,3.);
#7098=VECTOR('',#26696,3.);
#7099=VECTOR('',#26699,3.);
#7100=VECTOR('',#26702,3.);
#7101=VECTOR('',#26705,3.);
#7102=VECTOR('',#26708,3.);
#7103=VECTOR('',#26711,3.);
#7104=VECTOR('',#26714,3.);
#7105=VECTOR('',#26717,3.);
#7106=VECTOR('',#26720,3.);
#7107=VECTOR('',#26723,3.);
#7108=VECTOR('',#26726,3.);
#7109=VECTOR('',#26729,3.);
#7110=VECTOR('',#26734,3.0735);
#7111=VECTOR('',#26739,3.0735);
#7112=VECTOR('',#26742,3.0735);
#7113=VECTOR('',#26745,3.0735);
#7114=VECTOR('',#26748,3.0735);
#7115=VECTOR('',#26751,3.0735);
#7116=VECTOR('',#26754,3.0735);
#7117=VECTOR('',#26757,3.0735);
#7118=VECTOR('',#26760,3.0735);
#7119=VECTOR('',#26763,3.0735);
#7120=VECTOR('',#26766,3.0735);
#7121=VECTOR('',#26769,3.0735);
#7122=VECTOR('',#26772,3.0735);
#7123=VECTOR('',#26775,3.0735);
#7124=VECTOR('',#26778,3.0735);
#7125=VECTOR('',#26781,3.0735);
#7126=VECTOR('',#26784,3.0735);
#7127=VECTOR('',#26787,3.0735);
#7128=VECTOR('',#26790,3.0735);
#7129=VECTOR('',#26793,3.0735);
#7130=VECTOR('',#26798,3.0735);
#7131=VECTOR('',#26803,3.0735);
#7132=VECTOR('',#26806,3.0735);
#7133=VECTOR('',#26809,3.0735);
#7134=VECTOR('',#26812,3.0735);
#7135=VECTOR('',#26815,3.0735);
#7136=VECTOR('',#26818,3.0735);
#7137=VECTOR('',#26821,3.0735);
#7138=VECTOR('',#26824,3.0735);
#7139=VECTOR('',#26827,3.0735);
#7140=VECTOR('',#26830,3.0735);
#7141=VECTOR('',#26833,3.0735);
#7142=VECTOR('',#26836,3.0735);
#7143=VECTOR('',#26839,3.0735);
#7144=VECTOR('',#26842,3.0735);
#7145=VECTOR('',#26845,3.0735);
#7146=VECTOR('',#26848,3.0735);
#7147=VECTOR('',#26851,3.0735);
#7148=VECTOR('',#26854,3.0735);
#7149=VECTOR('',#26857,3.0735);
#7150=VECTOR('',#26862,3.07349999999996);
#7151=VECTOR('',#26867,3.07349999999996);
#7152=VECTOR('',#26870,3.07349999999996);
#7153=VECTOR('',#26873,3.07349999999996);
#7154=VECTOR('',#26876,3.07349999999996);
#7155=VECTOR('',#26879,3.07349999999996);
#7156=VECTOR('',#26882,3.07349999999996);
#7157=VECTOR('',#26885,3.07349999999996);
#7158=VECTOR('',#26888,3.07349999999996);
#7159=VECTOR('',#26891,3.07349999999996);
#7160=VECTOR('',#26894,3.07349999999996);
#7161=VECTOR('',#26897,3.07349999999996);
#7162=VECTOR('',#26900,3.07349999999996);
#7163=VECTOR('',#26903,3.07349999999996);
#7164=VECTOR('',#26906,3.07349999999996);
#7165=VECTOR('',#26909,3.07349999999996);
#7166=VECTOR('',#26912,3.07349999999996);
#7167=VECTOR('',#26915,3.07349999999996);
#7168=VECTOR('',#26918,3.07349999999996);
#7169=VECTOR('',#26921,3.07349999999996);
#7170=VECTOR('',#26926,3.07349999999996);
#7171=VECTOR('',#26931,3.07349999999996);
#7172=VECTOR('',#26934,3.07349999999996);
#7173=VECTOR('',#26937,3.07349999999996);
#7174=VECTOR('',#26940,3.07349999999996);
#7175=VECTOR('',#26943,3.07349999999996);
#7176=VECTOR('',#26946,3.07349999999996);
#7177=VECTOR('',#26949,3.07349999999996);
#7178=VECTOR('',#26952,3.07349999999996);
#7179=VECTOR('',#26955,3.07349999999996);
#7180=VECTOR('',#26958,3.07349999999996);
#7181=VECTOR('',#26961,3.07349999999996);
#7182=VECTOR('',#26964,3.07349999999996);
#7183=VECTOR('',#26967,3.07349999999996);
#7184=VECTOR('',#26970,3.07349999999996);
#7185=VECTOR('',#26973,3.07349999999996);
#7186=VECTOR('',#26976,3.07349999999996);
#7187=VECTOR('',#26979,3.07349999999996);
#7188=VECTOR('',#26982,3.07349999999996);
#7189=VECTOR('',#26985,3.07349999999996);
#7190=VECTOR('',#26990,3.0735);
#7191=VECTOR('',#26995,3.0735);
#7192=VECTOR('',#26998,3.0735);
#7193=VECTOR('',#27001,3.0735);
#7194=VECTOR('',#27004,3.0735);
#7195=VECTOR('',#27007,3.0735);
#7196=VECTOR('',#27010,3.0735);
#7197=VECTOR('',#27013,3.0735);
#7198=VECTOR('',#27016,3.0735);
#7199=VECTOR('',#27019,3.0735);
#7200=VECTOR('',#27022,3.0735);
#7201=VECTOR('',#27025,3.0735);
#7202=VECTOR('',#27028,3.0735);
#7203=VECTOR('',#27031,3.0735);
#7204=VECTOR('',#27034,3.0735);
#7205=VECTOR('',#27037,3.0735);
#7206=VECTOR('',#27040,3.0735);
#7207=VECTOR('',#27043,3.0735);
#7208=VECTOR('',#27046,3.0735);
#7209=VECTOR('',#27049,3.0735);
#7210=VECTOR('',#27054,3.0735);
#7211=VECTOR('',#27059,3.0735);
#7212=VECTOR('',#27062,3.0735);
#7213=VECTOR('',#27065,3.0735);
#7214=VECTOR('',#27068,3.0735);
#7215=VECTOR('',#27071,3.0735);
#7216=VECTOR('',#27074,3.0735);
#7217=VECTOR('',#27077,3.0735);
#7218=VECTOR('',#27080,3.0735);
#7219=VECTOR('',#27083,3.0735);
#7220=VECTOR('',#27086,3.0735);
#7221=VECTOR('',#27089,3.0735);
#7222=VECTOR('',#27092,3.0735);
#7223=VECTOR('',#27095,3.0735);
#7224=VECTOR('',#27098,3.0735);
#7225=VECTOR('',#27101,3.0735);
#7226=VECTOR('',#27104,3.0735);
#7227=VECTOR('',#27107,3.0735);
#7228=VECTOR('',#27110,3.0735);
#7229=VECTOR('',#27113,3.0735);
#7230=VECTOR('',#27120,10.);
#7231=VECTOR('',#27121,10.);
#7232=VECTOR('',#27122,10.);
#7233=VECTOR('',#27123,10.);
#7234=VECTOR('',#27148,10.);
#7235=VECTOR('',#27149,10.);
#7236=VECTOR('',#27150,10.);
#7237=VECTOR('',#27153,10.);
#7238=VECTOR('',#27154,10.);
#7239=VECTOR('',#27157,10.);
#7240=VECTOR('',#27158,10.);
#7241=VECTOR('',#27161,10.);
#7574=CIRCLE('',#23044,2.5175);
#7575=CIRCLE('',#23064,2.5175);
#7576=CIRCLE('',#23066,2.5175);
#7577=CIRCLE('',#23086,2.5175);
#7578=CIRCLE('',#23088,2.5175);
#7579=CIRCLE('',#23108,2.5175);
#7580=CIRCLE('',#23110,2.5175);
#7581=CIRCLE('',#23130,2.5175);
#7582=CIRCLE('',#23132,2.5175);
#7583=CIRCLE('',#23152,2.5175);
#7584=CIRCLE('',#23154,2.5175);
#7585=CIRCLE('',#23174,2.5175);
#7586=CIRCLE('',#23176,3.0735);
#7587=CIRCLE('',#23196,3.0735);
#7588=CIRCLE('',#23198,3.07349999999999);
#7589=CIRCLE('',#23218,3.0735);
#7590=CIRCLE('',#23220,3.07349999999996);
#7591=CIRCLE('',#23240,3.07349999999996);
#7592=CIRCLE('',#23242,3.07349999999996);
#7593=CIRCLE('',#23262,3.07349999999996);
#7594=CIRCLE('',#23264,3.07349999999999);
#7595=CIRCLE('',#23284,3.0735);
#7596=CIRCLE('',#23286,3.0735);
#7597=CIRCLE('',#23306,3.0735);
#9049=VERTEX_POINT('',#72982);
#9050=VERTEX_POINT('',#72983);
#9051=VERTEX_POINT('',#72985);
#9052=VERTEX_POINT('',#72990);
#9053=VERTEX_POINT('',#73003);
#9054=VERTEX_POINT('',#73004);
#9055=VERTEX_POINT('',#73054);
#9056=VERTEX_POINT('',#73055);
#9057=VERTEX_POINT('',#73105);
#9058=VERTEX_POINT('',#73106);
#9059=VERTEX_POINT('',#73153);
#9060=VERTEX_POINT('',#73154);
#9061=VERTEX_POINT('',#73201);
#9062=VERTEX_POINT('',#73202);
#9063=VERTEX_POINT('',#73252);
#9064=VERTEX_POINT('',#73253);
#9065=VERTEX_POINT('',#73303);
#9066=VERTEX_POINT('',#73304);
#9067=VERTEX_POINT('',#73351);
#9068=VERTEX_POINT('',#73352);
#9069=VERTEX_POINT('',#73402);
#9070=VERTEX_POINT('',#73403);
#9071=VERTEX_POINT('',#73453);
#9072=VERTEX_POINT('',#73454);
#9073=VERTEX_POINT('',#73501);
#9074=VERTEX_POINT('',#73502);
#9075=VERTEX_POINT('',#73549);
#9076=VERTEX_POINT('',#73550);
#9077=VERTEX_POINT('',#73603);
#9078=VERTEX_POINT('',#73604);
#9079=VERTEX_POINT('',#73651);
#9080=VERTEX_POINT('',#73652);
#9081=VERTEX_POINT('',#73699);
#9082=VERTEX_POINT('',#73700);
#9083=VERTEX_POINT('',#73750);
#9084=VERTEX_POINT('',#73751);
#9085=VERTEX_POINT('',#73801);
#9086=VERTEX_POINT('',#73802);
#9087=VERTEX_POINT('',#73849);
#9088=VERTEX_POINT('',#73850);
#9089=VERTEX_POINT('',#73900);
#9090=VERTEX_POINT('',#73901);
#9091=VERTEX_POINT('',#73903);
#9092=VERTEX_POINT('',#73917);
#9093=VERTEX_POINT('',#73939);
#9094=VERTEX_POINT('',#73940);
#9095=VERTEX_POINT('',#73942);
#9096=VERTEX_POINT('',#73947);
#9097=VERTEX_POINT('',#73960);
#9098=VERTEX_POINT('',#73961);
#9099=VERTEX_POINT('',#74011);
#9100=VERTEX_POINT('',#74012);
#9101=VERTEX_POINT('',#74062);
#9102=VERTEX_POINT('',#74063);
#9103=VERTEX_POINT('',#74110);
#9104=VERTEX_POINT('',#74111);
#9105=VERTEX_POINT('',#74158);
#9106=VERTEX_POINT('',#74159);
#9107=VERTEX_POINT('',#74209);
#9108=VERTEX_POINT('',#74210);
#9109=VERTEX_POINT('',#74260);
#9110=VERTEX_POINT('',#74261);
#9111=VERTEX_POINT('',#74308);
#9112=VERTEX_POINT('',#74309);
#9113=VERTEX_POINT('',#74359);
#9114=VERTEX_POINT('',#74360);
#9115=VERTEX_POINT('',#74410);
#9116=VERTEX_POINT('',#74411);
#9117=VERTEX_POINT('',#74458);
#9118=VERTEX_POINT('',#74459);
#9119=VERTEX_POINT('',#74506);
#9120=VERTEX_POINT('',#74507);
#9121=VERTEX_POINT('',#74560);
#9122=VERTEX_POINT('',#74561);
#9123=VERTEX_POINT('',#74608);
#9124=VERTEX_POINT('',#74609);
#9125=VERTEX_POINT('',#74656);
#9126=VERTEX_POINT('',#74657);
#9127=VERTEX_POINT('',#74707);
#9128=VERTEX_POINT('',#74708);
#9129=VERTEX_POINT('',#74758);
#9130=VERTEX_POINT('',#74759);
#9131=VERTEX_POINT('',#74806);
#9132=VERTEX_POINT('',#74807);
#9133=VERTEX_POINT('',#74857);
#9134=VERTEX_POINT('',#74858);
#9135=VERTEX_POINT('',#74860);
#9136=VERTEX_POINT('',#74874);
#9137=VERTEX_POINT('',#74896);
#9138=VERTEX_POINT('',#74897);
#9139=VERTEX_POINT('',#74899);
#9140=VERTEX_POINT('',#74904);
#9141=VERTEX_POINT('',#74917);
#9142=VERTEX_POINT('',#74918);
#9143=VERTEX_POINT('',#74968);
#9144=VERTEX_POINT('',#74969);
#9145=VERTEX_POINT('',#75019);
#9146=VERTEX_POINT('',#75020);
#9147=VERTEX_POINT('',#75067);
#9148=VERTEX_POINT('',#75068);
#9149=VERTEX_POINT('',#75115);
#9150=VERTEX_POINT('',#75116);
#9151=VERTEX_POINT('',#75166);
#9152=VERTEX_POINT('',#75167);
#9153=VERTEX_POINT('',#75217);
#9154=VERTEX_POINT('',#75218);
#9155=VERTEX_POINT('',#75265);
#9156=VERTEX_POINT('',#75266);
#9157=VERTEX_POINT('',#75316);
#9158=VERTEX_POINT('',#75317);
#9159=VERTEX_POINT('',#75367);
#9160=VERTEX_POINT('',#75368);
#9161=VERTEX_POINT('',#75415);
#9162=VERTEX_POINT('',#75416);
#9163=VERTEX_POINT('',#75463);
#9164=VERTEX_POINT('',#75464);
#9165=VERTEX_POINT('',#75517);
#9166=VERTEX_POINT('',#75518);
#9167=VERTEX_POINT('',#75565);
#9168=VERTEX_POINT('',#75566);
#9169=VERTEX_POINT('',#75613);
#9170=VERTEX_POINT('',#75614);
#9171=VERTEX_POINT('',#75664);
#9172=VERTEX_POINT('',#75665);
#9173=VERTEX_POINT('',#75715);
#9174=VERTEX_POINT('',#75716);
#9175=VERTEX_POINT('',#75763);
#9176=VERTEX_POINT('',#75764);
#9177=VERTEX_POINT('',#75814);
#9178=VERTEX_POINT('',#75815);
#9179=VERTEX_POINT('',#75817);
#9180=VERTEX_POINT('',#75831);
#9181=VERTEX_POINT('',#75853);
#9182=VERTEX_POINT('',#75854);
#9183=VERTEX_POINT('',#75856);
#9184=VERTEX_POINT('',#75861);
#9185=VERTEX_POINT('',#75874);
#9186=VERTEX_POINT('',#75875);
#9187=VERTEX_POINT('',#75925);
#9188=VERTEX_POINT('',#75926);
#9189=VERTEX_POINT('',#75976);
#9190=VERTEX_POINT('',#75977);
#9191=VERTEX_POINT('',#76024);
#9192=VERTEX_POINT('',#76025);
#9193=VERTEX_POINT('',#76072);
#9194=VERTEX_POINT('',#76073);
#9195=VERTEX_POINT('',#76123);
#9196=VERTEX_POINT('',#76124);
#9197=VERTEX_POINT('',#76174);
#9198=VERTEX_POINT('',#76175);
#9199=VERTEX_POINT('',#76222);
#9200=VERTEX_POINT('',#76223);
#9201=VERTEX_POINT('',#76273);
#9202=VERTEX_POINT('',#76274);
#9203=VERTEX_POINT('',#76324);
#9204=VERTEX_POINT('',#76325);
#9205=VERTEX_POINT('',#76372);
#9206=VERTEX_POINT('',#76373);
#9207=VERTEX_POINT('',#76420);
#9208=VERTEX_POINT('',#76421);
#9209=VERTEX_POINT('',#76474);
#9210=VERTEX_POINT('',#76475);
#9211=VERTEX_POINT('',#76522);
#9212=VERTEX_POINT('',#76523);
#9213=VERTEX_POINT('',#76570);
#9214=VERTEX_POINT('',#76571);
#9215=VERTEX_POINT('',#76621);
#9216=VERTEX_POINT('',#76622);
#9217=VERTEX_POINT('',#76672);
#9218=VERTEX_POINT('',#76673);
#9219=VERTEX_POINT('',#76720);
#9220=VERTEX_POINT('',#76721);
#9221=VERTEX_POINT('',#76771);
#9222=VERTEX_POINT('',#76772);
#9223=VERTEX_POINT('',#76774);
#9224=VERTEX_POINT('',#76788);
#9225=VERTEX_POINT('',#76810);
#9226=VERTEX_POINT('',#76811);
#9227=VERTEX_POINT('',#76813);
#9228=VERTEX_POINT('',#76818);
#9229=VERTEX_POINT('',#76831);
#9230=VERTEX_POINT('',#76832);
#9231=VERTEX_POINT('',#76882);
#9232=VERTEX_POINT('',#76883);
#9233=VERTEX_POINT('',#76933);
#9234=VERTEX_POINT('',#76934);
#9235=VERTEX_POINT('',#76981);
#9236=VERTEX_POINT('',#76982);
#9237=VERTEX_POINT('',#77029);
#9238=VERTEX_POINT('',#77030);
#9239=VERTEX_POINT('',#77080);
#9240=VERTEX_POINT('',#77081);
#9241=VERTEX_POINT('',#77131);
#9242=VERTEX_POINT('',#77132);
#9243=VERTEX_POINT('',#77179);
#9244=VERTEX_POINT('',#77180);
#9245=VERTEX_POINT('',#77230);
#9246=VERTEX_POINT('',#77231);
#9247=VERTEX_POINT('',#77281);
#9248=VERTEX_POINT('',#77282);
#9249=VERTEX_POINT('',#77329);
#9250=VERTEX_POINT('',#77330);
#9251=VERTEX_POINT('',#77377);
#9252=VERTEX_POINT('',#77378);
#9253=VERTEX_POINT('',#77431);
#9254=VERTEX_POINT('',#77432);
#9255=VERTEX_POINT('',#77479);
#9256=VERTEX_POINT('',#77480);
#9257=VERTEX_POINT('',#77527);
#9258=VERTEX_POINT('',#77528);
#9259=VERTEX_POINT('',#77578);
#9260=VERTEX_POINT('',#77579);
#9261=VERTEX_POINT('',#77629);
#9262=VERTEX_POINT('',#77630);
#9263=VERTEX_POINT('',#77677);
#9264=VERTEX_POINT('',#77678);
#9265=VERTEX_POINT('',#77728);
#9266=VERTEX_POINT('',#77729);
#9267=VERTEX_POINT('',#77731);
#9268=VERTEX_POINT('',#77745);
#9269=VERTEX_POINT('',#77767);
#9270=VERTEX_POINT('',#77768);
#9271=VERTEX_POINT('',#77770);
#9272=VERTEX_POINT('',#77775);
#9273=VERTEX_POINT('',#77788);
#9274=VERTEX_POINT('',#77789);
#9275=VERTEX_POINT('',#77839);
#9276=VERTEX_POINT('',#77840);
#9277=VERTEX_POINT('',#77890);
#9278=VERTEX_POINT('',#77891);
#9279=VERTEX_POINT('',#77938);
#9280=VERTEX_POINT('',#77939);
#9281=VERTEX_POINT('',#77986);
#9282=VERTEX_POINT('',#77987);
#9283=VERTEX_POINT('',#78037);
#9284=VERTEX_POINT('',#78038);
#9285=VERTEX_POINT('',#78088);
#9286=VERTEX_POINT('',#78089);
#9287=VERTEX_POINT('',#78136);
#9288=VERTEX_POINT('',#78137);
#9289=VERTEX_POINT('',#78187);
#9290=VERTEX_POINT('',#78188);
#9291=VERTEX_POINT('',#78238);
#9292=VERTEX_POINT('',#78239);
#9293=VERTEX_POINT('',#78286);
#9294=VERTEX_POINT('',#78287);
#9295=VERTEX_POINT('',#78334);
#9296=VERTEX_POINT('',#78335);
#9297=VERTEX_POINT('',#78388);
#9298=VERTEX_POINT('',#78389);
#9299=VERTEX_POINT('',#78436);
#9300=VERTEX_POINT('',#78437);
#9301=VERTEX_POINT('',#78484);
#9302=VERTEX_POINT('',#78485);
#9303=VERTEX_POINT('',#78535);
#9304=VERTEX_POINT('',#78536);
#9305=VERTEX_POINT('',#78586);
#9306=VERTEX_POINT('',#78587);
#9307=VERTEX_POINT('',#78634);
#9308=VERTEX_POINT('',#78635);
#9309=VERTEX_POINT('',#78685);
#9310=VERTEX_POINT('',#78686);
#9311=VERTEX_POINT('',#78688);
#9312=VERTEX_POINT('',#78702);
#9313=VERTEX_POINT('',#78724);
#9314=VERTEX_POINT('',#78725);
#9315=VERTEX_POINT('',#78727);
#9316=VERTEX_POINT('',#78736);
#9317=VERTEX_POINT('',#78748);
#9318=VERTEX_POINT('',#78749);
#9319=VERTEX_POINT('',#78772);
#9320=VERTEX_POINT('',#78773);
#9321=VERTEX_POINT('',#78797);
#9322=VERTEX_POINT('',#78798);
#9323=VERTEX_POINT('',#78821);
#9324=VERTEX_POINT('',#78822);
#9325=VERTEX_POINT('',#78846);
#9326=VERTEX_POINT('',#78847);
#9327=VERTEX_POINT('',#78870);
#9328=VERTEX_POINT('',#78871);
#9329=VERTEX_POINT('',#78895);
#9330=VERTEX_POINT('',#78896);
#9331=VERTEX_POINT('',#78920);
#9332=VERTEX_POINT('',#78921);
#9333=VERTEX_POINT('',#78944);
#9334=VERTEX_POINT('',#78945);
#9335=VERTEX_POINT('',#78969);
#9336=VERTEX_POINT('',#78970);
#9337=VERTEX_POINT('',#78993);
#9338=VERTEX_POINT('',#78994);
#9339=VERTEX_POINT('',#79018);
#9340=VERTEX_POINT('',#79019);
#9341=VERTEX_POINT('',#79043);
#9342=VERTEX_POINT('',#79044);
#9343=VERTEX_POINT('',#79067);
#9344=VERTEX_POINT('',#79068);
#9345=VERTEX_POINT('',#79092);
#9346=VERTEX_POINT('',#79093);
#9347=VERTEX_POINT('',#79116);
#9348=VERTEX_POINT('',#79117);
#9349=VERTEX_POINT('',#79141);
#9350=VERTEX_POINT('',#79142);
#9351=VERTEX_POINT('',#79166);
#9352=VERTEX_POINT('',#79167);
#9353=VERTEX_POINT('',#79190);
#9354=VERTEX_POINT('',#79191);
#9355=VERTEX_POINT('',#79193);
#9356=VERTEX_POINT('',#79199);
#9357=VERTEX_POINT('',#79207);
#9358=VERTEX_POINT('',#79208);
#9359=VERTEX_POINT('',#79210);
#9360=VERTEX_POINT('',#79219);
#9361=VERTEX_POINT('',#79231);
#9362=VERTEX_POINT('',#79232);
#9363=VERTEX_POINT('',#79255);
#9364=VERTEX_POINT('',#79256);
#9365=VERTEX_POINT('',#79280);
#9366=VERTEX_POINT('',#79281);
#9367=VERTEX_POINT('',#79304);
#9368=VERTEX_POINT('',#79305);
#9369=VERTEX_POINT('',#79329);
#9370=VERTEX_POINT('',#79330);
#9371=VERTEX_POINT('',#79353);
#9372=VERTEX_POINT('',#79354);
#9373=VERTEX_POINT('',#79378);
#9374=VERTEX_POINT('',#79379);
#9375=VERTEX_POINT('',#79403);
#9376=VERTEX_POINT('',#79404);
#9377=VERTEX_POINT('',#79427);
#9378=VERTEX_POINT('',#79428);
#9379=VERTEX_POINT('',#79452);
#9380=VERTEX_POINT('',#79453);
#9381=VERTEX_POINT('',#79476);
#9382=VERTEX_POINT('',#79477);
#9383=VERTEX_POINT('',#79501);
#9384=VERTEX_POINT('',#79502);
#9385=VERTEX_POINT('',#79526);
#9386=VERTEX_POINT('',#79527);
#9387=VERTEX_POINT('',#79550);
#9388=VERTEX_POINT('',#79551);
#9389=VERTEX_POINT('',#79575);
#9390=VERTEX_POINT('',#79576);
#9391=VERTEX_POINT('',#79599);
#9392=VERTEX_POINT('',#79600);
#9393=VERTEX_POINT('',#79624);
#9394=VERTEX_POINT('',#79625);
#9395=VERTEX_POINT('',#79649);
#9396=VERTEX_POINT('',#79650);
#9397=VERTEX_POINT('',#79673);
#9398=VERTEX_POINT('',#79674);
#9399=VERTEX_POINT('',#79676);
#9400=VERTEX_POINT('',#79682);
#9401=VERTEX_POINT('',#79690);
#9402=VERTEX_POINT('',#79691);
#9403=VERTEX_POINT('',#79693);
#9404=VERTEX_POINT('',#79702);
#9405=VERTEX_POINT('',#79714);
#9406=VERTEX_POINT('',#79715);
#9407=VERTEX_POINT('',#79738);
#9408=VERTEX_POINT('',#79739);
#9409=VERTEX_POINT('',#79763);
#9410=VERTEX_POINT('',#79764);
#9411=VERTEX_POINT('',#79787);
#9412=VERTEX_POINT('',#79788);
#9413=VERTEX_POINT('',#79812);
#9414=VERTEX_POINT('',#79813);
#9415=VERTEX_POINT('',#79836);
#9416=VERTEX_POINT('',#79837);
#9417=VERTEX_POINT('',#79861);
#9418=VERTEX_POINT('',#79862);
#9419=VERTEX_POINT('',#79886);
#9420=VERTEX_POINT('',#79887);
#9421=VERTEX_POINT('',#79910);
#9422=VERTEX_POINT('',#79911);
#9423=VERTEX_POINT('',#79935);
#9424=VERTEX_POINT('',#79936);
#9425=VERTEX_POINT('',#79959);
#9426=VERTEX_POINT('',#79960);
#9427=VERTEX_POINT('',#79984);
#9428=VERTEX_POINT('',#79985);
#9429=VERTEX_POINT('',#80009);
#9430=VERTEX_POINT('',#80010);
#9431=VERTEX_POINT('',#80033);
#9432=VERTEX_POINT('',#80034);
#9433=VERTEX_POINT('',#80058);
#9434=VERTEX_POINT('',#80059);
#9435=VERTEX_POINT('',#80082);
#9436=VERTEX_POINT('',#80083);
#9437=VERTEX_POINT('',#80107);
#9438=VERTEX_POINT('',#80108);
#9439=VERTEX_POINT('',#80132);
#9440=VERTEX_POINT('',#80133);
#9441=VERTEX_POINT('',#80156);
#9442=VERTEX_POINT('',#80157);
#9443=VERTEX_POINT('',#80159);
#9444=VERTEX_POINT('',#80165);
#9445=VERTEX_POINT('',#80173);
#9446=VERTEX_POINT('',#80174);
#9447=VERTEX_POINT('',#80176);
#9448=VERTEX_POINT('',#80185);
#9449=VERTEX_POINT('',#80197);
#9450=VERTEX_POINT('',#80198);
#9451=VERTEX_POINT('',#80221);
#9452=VERTEX_POINT('',#80222);
#9453=VERTEX_POINT('',#80246);
#9454=VERTEX_POINT('',#80247);
#9455=VERTEX_POINT('',#80270);
#9456=VERTEX_POINT('',#80271);
#9457=VERTEX_POINT('',#80295);
#9458=VERTEX_POINT('',#80296);
#9459=VERTEX_POINT('',#80319);
#9460=VERTEX_POINT('',#80320);
#9461=VERTEX_POINT('',#80344);
#9462=VERTEX_POINT('',#80345);
#9463=VERTEX_POINT('',#80369);
#9464=VERTEX_POINT('',#80370);
#9465=VERTEX_POINT('',#80393);
#9466=VERTEX_POINT('',#80394);
#9467=VERTEX_POINT('',#80418);
#9468=VERTEX_POINT('',#80419);
#9469=VERTEX_POINT('',#80442);
#9470=VERTEX_POINT('',#80443);
#9471=VERTEX_POINT('',#80467);
#9472=VERTEX_POINT('',#80468);
#9473=VERTEX_POINT('',#80492);
#9474=VERTEX_POINT('',#80493);
#9475=VERTEX_POINT('',#80516);
#9476=VERTEX_POINT('',#80517);
#9477=VERTEX_POINT('',#80541);
#9478=VERTEX_POINT('',#80542);
#9479=VERTEX_POINT('',#80565);
#9480=VERTEX_POINT('',#80566);
#9481=VERTEX_POINT('',#80590);
#9482=VERTEX_POINT('',#80591);
#9483=VERTEX_POINT('',#80615);
#9484=VERTEX_POINT('',#80616);
#9485=VERTEX_POINT('',#80639);
#9486=VERTEX_POINT('',#80640);
#9487=VERTEX_POINT('',#80642);
#9488=VERTEX_POINT('',#80648);
#9489=VERTEX_POINT('',#80656);
#9490=VERTEX_POINT('',#80657);
#9491=VERTEX_POINT('',#80659);
#9492=VERTEX_POINT('',#80668);
#9493=VERTEX_POINT('',#80680);
#9494=VERTEX_POINT('',#80681);
#9495=VERTEX_POINT('',#80704);
#9496=VERTEX_POINT('',#80705);
#9497=VERTEX_POINT('',#80729);
#9498=VERTEX_POINT('',#80730);
#9499=VERTEX_POINT('',#80753);
#9500=VERTEX_POINT('',#80754);
#9501=VERTEX_POINT('',#80778);
#9502=VERTEX_POINT('',#80779);
#9503=VERTEX_POINT('',#80802);
#9504=VERTEX_POINT('',#80803);
#9505=VERTEX_POINT('',#80827);
#9506=VERTEX_POINT('',#80828);
#9507=VERTEX_POINT('',#80852);
#9508=VERTEX_POINT('',#80853);
#9509=VERTEX_POINT('',#80876);
#9510=VERTEX_POINT('',#80877);
#9511=VERTEX_POINT('',#80901);
#9512=VERTEX_POINT('',#80902);
#9513=VERTEX_POINT('',#80925);
#9514=VERTEX_POINT('',#80926);
#9515=VERTEX_POINT('',#80950);
#9516=VERTEX_POINT('',#80951);
#9517=VERTEX_POINT('',#80975);
#9518=VERTEX_POINT('',#80976);
#9519=VERTEX_POINT('',#80999);
#9520=VERTEX_POINT('',#81000);
#9521=VERTEX_POINT('',#81024);
#9522=VERTEX_POINT('',#81025);
#9523=VERTEX_POINT('',#81048);
#9524=VERTEX_POINT('',#81049);
#9525=VERTEX_POINT('',#81073);
#9526=VERTEX_POINT('',#81074);
#9527=VERTEX_POINT('',#81098);
#9528=VERTEX_POINT('',#81099);
#9529=VERTEX_POINT('',#81122);
#9530=VERTEX_POINT('',#81123);
#9531=VERTEX_POINT('',#81125);
#9532=VERTEX_POINT('',#81131);
#9533=VERTEX_POINT('',#81139);
#9534=VERTEX_POINT('',#81140);
#9535=VERTEX_POINT('',#81142);
#9536=VERTEX_POINT('',#81151);
#9537=VERTEX_POINT('',#81163);
#9538=VERTEX_POINT('',#81164);
#9539=VERTEX_POINT('',#81187);
#9540=VERTEX_POINT('',#81188);
#9541=VERTEX_POINT('',#81212);
#9542=VERTEX_POINT('',#81213);
#9543=VERTEX_POINT('',#81236);
#9544=VERTEX_POINT('',#81237);
#9545=VERTEX_POINT('',#81261);
#9546=VERTEX_POINT('',#81262);
#9547=VERTEX_POINT('',#81285);
#9548=VERTEX_POINT('',#81286);
#9549=VERTEX_POINT('',#81310);
#9550=VERTEX_POINT('',#81311);
#9551=VERTEX_POINT('',#81335);
#9552=VERTEX_POINT('',#81336);
#9553=VERTEX_POINT('',#81359);
#9554=VERTEX_POINT('',#81360);
#9555=VERTEX_POINT('',#81384);
#9556=VERTEX_POINT('',#81385);
#9557=VERTEX_POINT('',#81408);
#9558=VERTEX_POINT('',#81409);
#9559=VERTEX_POINT('',#81433);
#9560=VERTEX_POINT('',#81434);
#9561=VERTEX_POINT('',#81458);
#9562=VERTEX_POINT('',#81459);
#9563=VERTEX_POINT('',#81482);
#9564=VERTEX_POINT('',#81483);
#9565=VERTEX_POINT('',#81507);
#9566=VERTEX_POINT('',#81508);
#9567=VERTEX_POINT('',#81531);
#9568=VERTEX_POINT('',#81532);
#9569=VERTEX_POINT('',#81556);
#9570=VERTEX_POINT('',#81557);
#9571=VERTEX_POINT('',#81581);
#9572=VERTEX_POINT('',#81582);
#9573=VERTEX_POINT('',#81605);
#9574=VERTEX_POINT('',#81606);
#9575=VERTEX_POINT('',#81608);
#9576=VERTEX_POINT('',#81614);
#9577=VERTEX_POINT('',#83115);
#9578=VERTEX_POINT('',#83116);
#9579=VERTEX_POINT('',#83118);
#9580=VERTEX_POINT('',#83120);
#9581=VERTEX_POINT('',#90595);
#9582=VERTEX_POINT('',#90596);
#9583=VERTEX_POINT('',#90601);
#9584=VERTEX_POINT('',#90605);
#11966=EDGE_CURVE('',#9049,#9050,#5776,.T.);
#11967=EDGE_CURVE('',#9050,#9051,#1479,.T.);
#11968=EDGE_CURVE('',#9052,#9051,#7574,.F.);
#11969=EDGE_CURVE('',#9052,#9049,#1480,.T.);
#11970=EDGE_CURVE('',#9053,#9054,#5777,.T.);
#11971=EDGE_CURVE('',#9054,#9050,#1481,.T.);
#11972=EDGE_CURVE('',#9049,#9053,#1482,.T.);
#11973=EDGE_CURVE('',#9055,#9056,#5778,.T.);
#11974=EDGE_CURVE('',#9056,#9054,#1483,.T.);
#11975=EDGE_CURVE('',#9053,#9055,#1484,.T.);
#11976=EDGE_CURVE('',#9057,#9058,#5779,.T.);
#11977=EDGE_CURVE('',#9058,#9056,#1485,.T.);
#11978=EDGE_CURVE('',#9055,#9057,#1486,.T.);
#11979=EDGE_CURVE('',#9059,#9060,#5780,.T.);
#11980=EDGE_CURVE('',#9060,#9058,#1487,.T.);
#11981=EDGE_CURVE('',#9057,#9059,#1488,.T.);
#11982=EDGE_CURVE('',#9061,#9062,#5781,.T.);
#11983=EDGE_CURVE('',#9062,#9060,#1489,.T.);
#11984=EDGE_CURVE('',#9059,#9061,#1490,.T.);
#11985=EDGE_CURVE('',#9063,#9064,#5782,.T.);
#11986=EDGE_CURVE('',#9064,#9062,#1491,.T.);
#11987=EDGE_CURVE('',#9061,#9063,#1492,.T.);
#11988=EDGE_CURVE('',#9065,#9066,#5783,.T.);
#11989=EDGE_CURVE('',#9066,#9064,#1493,.T.);
#11990=EDGE_CURVE('',#9063,#9065,#1494,.T.);
#11991=EDGE_CURVE('',#9067,#9068,#5784,.T.);
#11992=EDGE_CURVE('',#9068,#9066,#1495,.T.);
#11993=EDGE_CURVE('',#9065,#9067,#1496,.T.);
#11994=EDGE_CURVE('',#9069,#9070,#5785,.T.);
#11995=EDGE_CURVE('',#9070,#9068,#1497,.T.);
#11996=EDGE_CURVE('',#9067,#9069,#1498,.T.);
#11997=EDGE_CURVE('',#9071,#9072,#5786,.T.);
#11998=EDGE_CURVE('',#9072,#9070,#1499,.T.);
#11999=EDGE_CURVE('',#9069,#9071,#1500,.T.);
#12000=EDGE_CURVE('',#9073,#9074,#5787,.T.);
#12001=EDGE_CURVE('',#9074,#9072,#1501,.T.);
#12002=EDGE_CURVE('',#9071,#9073,#1502,.T.);
#12003=EDGE_CURVE('',#9075,#9076,#5788,.T.);
#12004=EDGE_CURVE('',#9076,#9074,#1503,.T.);
#12005=EDGE_CURVE('',#9073,#9075,#1504,.T.);
#12006=EDGE_CURVE('',#9077,#9078,#5789,.T.);
#12007=EDGE_CURVE('',#9078,#9076,#1505,.T.);
#12008=EDGE_CURVE('',#9075,#9077,#1506,.T.);
#12009=EDGE_CURVE('',#9079,#9080,#5790,.T.);
#12010=EDGE_CURVE('',#9080,#9078,#1507,.T.);
#12011=EDGE_CURVE('',#9077,#9079,#1508,.T.);
#12012=EDGE_CURVE('',#9081,#9082,#5791,.T.);
#12013=EDGE_CURVE('',#9082,#9080,#1509,.T.);
#12014=EDGE_CURVE('',#9079,#9081,#1510,.T.);
#12015=EDGE_CURVE('',#9083,#9084,#5792,.T.);
#12016=EDGE_CURVE('',#9084,#9082,#1511,.T.);
#12017=EDGE_CURVE('',#9081,#9083,#1512,.T.);
#12018=EDGE_CURVE('',#9085,#9086,#5793,.T.);
#12019=EDGE_CURVE('',#9086,#9084,#1513,.T.);
#12020=EDGE_CURVE('',#9083,#9085,#1514,.T.);
#12021=EDGE_CURVE('',#9087,#9088,#5794,.T.);
#12022=EDGE_CURVE('',#9088,#9086,#1515,.T.);
#12023=EDGE_CURVE('',#9085,#9087,#1516,.T.);
#12024=EDGE_CURVE('',#9089,#9090,#5795,.T.);
#12025=EDGE_CURVE('',#9089,#9091,#1517,.T.);
#12026=EDGE_CURVE('',#9092,#9091,#7575,.T.);
#12027=EDGE_CURVE('',#9092,#9090,#1518,.T.);
#12028=EDGE_CURVE('',#9093,#9094,#5796,.T.);
#12029=EDGE_CURVE('',#9094,#9095,#1519,.T.);
#12030=EDGE_CURVE('',#9096,#9095,#7576,.F.);
#12031=EDGE_CURVE('',#9096,#9093,#1520,.T.);
#12032=EDGE_CURVE('',#9097,#9098,#5797,.T.);
#12033=EDGE_CURVE('',#9098,#9094,#1521,.T.);
#12034=EDGE_CURVE('',#9093,#9097,#1522,.T.);
#12035=EDGE_CURVE('',#9099,#9100,#5798,.T.);
#12036=EDGE_CURVE('',#9100,#9098,#1523,.T.);
#12037=EDGE_CURVE('',#9097,#9099,#1524,.T.);
#12038=EDGE_CURVE('',#9101,#9102,#5799,.T.);
#12039=EDGE_CURVE('',#9102,#9100,#1525,.T.);
#12040=EDGE_CURVE('',#9099,#9101,#1526,.T.);
#12041=EDGE_CURVE('',#9103,#9104,#5800,.T.);
#12042=EDGE_CURVE('',#9104,#9102,#1527,.T.);
#12043=EDGE_CURVE('',#9101,#9103,#1528,.T.);
#12044=EDGE_CURVE('',#9105,#9106,#5801,.T.);
#12045=EDGE_CURVE('',#9106,#9104,#1529,.T.);
#12046=EDGE_CURVE('',#9103,#9105,#1530,.T.);
#12047=EDGE_CURVE('',#9107,#9108,#5802,.T.);
#12048=EDGE_CURVE('',#9108,#9106,#1531,.T.);
#12049=EDGE_CURVE('',#9105,#9107,#1532,.T.);
#12050=EDGE_CURVE('',#9109,#9110,#5803,.T.);
#12051=EDGE_CURVE('',#9110,#9108,#1533,.T.);
#12052=EDGE_CURVE('',#9107,#9109,#1534,.T.);
#12053=EDGE_CURVE('',#9111,#9112,#5804,.T.);
#12054=EDGE_CURVE('',#9112,#9110,#1535,.T.);
#12055=EDGE_CURVE('',#9109,#9111,#1536,.T.);
#12056=EDGE_CURVE('',#9113,#9114,#5805,.T.);
#12057=EDGE_CURVE('',#9114,#9112,#1537,.T.);
#12058=EDGE_CURVE('',#9111,#9113,#1538,.T.);
#12059=EDGE_CURVE('',#9115,#9116,#5806,.T.);
#12060=EDGE_CURVE('',#9116,#9114,#1539,.T.);
#12061=EDGE_CURVE('',#9113,#9115,#1540,.T.);
#12062=EDGE_CURVE('',#9117,#9118,#5807,.T.);
#12063=EDGE_CURVE('',#9118,#9116,#1541,.T.);
#12064=EDGE_CURVE('',#9115,#9117,#1542,.T.);
#12065=EDGE_CURVE('',#9119,#9120,#5808,.T.);
#12066=EDGE_CURVE('',#9120,#9118,#1543,.T.);
#12067=EDGE_CURVE('',#9117,#9119,#1544,.T.);
#12068=EDGE_CURVE('',#9121,#9122,#5809,.T.);
#12069=EDGE_CURVE('',#9122,#9120,#1545,.T.);
#12070=EDGE_CURVE('',#9119,#9121,#1546,.T.);
#12071=EDGE_CURVE('',#9123,#9124,#5810,.T.);
#12072=EDGE_CURVE('',#9124,#9122,#1547,.T.);
#12073=EDGE_CURVE('',#9121,#9123,#1548,.T.);
#12074=EDGE_CURVE('',#9125,#9126,#5811,.T.);
#12075=EDGE_CURVE('',#9126,#9124,#1549,.T.);
#12076=EDGE_CURVE('',#9123,#9125,#1550,.T.);
#12077=EDGE_CURVE('',#9127,#9128,#5812,.T.);
#12078=EDGE_CURVE('',#9128,#9126,#1551,.T.);
#12079=EDGE_CURVE('',#9125,#9127,#1552,.T.);
#12080=EDGE_CURVE('',#9129,#9130,#5813,.T.);
#12081=EDGE_CURVE('',#9130,#9128,#1553,.T.);
#12082=EDGE_CURVE('',#9127,#9129,#1554,.T.);
#12083=EDGE_CURVE('',#9131,#9132,#5814,.T.);
#12084=EDGE_CURVE('',#9132,#9130,#1555,.T.);
#12085=EDGE_CURVE('',#9129,#9131,#1556,.T.);
#12086=EDGE_CURVE('',#9133,#9134,#5815,.T.);
#12087=EDGE_CURVE('',#9133,#9135,#1557,.T.);
#12088=EDGE_CURVE('',#9136,#9135,#7577,.T.);
#12089=EDGE_CURVE('',#9136,#9134,#1558,.T.);
#12090=EDGE_CURVE('',#9137,#9138,#5816,.T.);
#12091=EDGE_CURVE('',#9138,#9139,#1559,.T.);
#12092=EDGE_CURVE('',#9140,#9139,#7578,.F.);
#12093=EDGE_CURVE('',#9140,#9137,#1560,.T.);
#12094=EDGE_CURVE('',#9141,#9142,#5817,.T.);
#12095=EDGE_CURVE('',#9142,#9138,#1561,.T.);
#12096=EDGE_CURVE('',#9137,#9141,#1562,.T.);
#12097=EDGE_CURVE('',#9143,#9144,#5818,.T.);
#12098=EDGE_CURVE('',#9144,#9142,#1563,.T.);
#12099=EDGE_CURVE('',#9141,#9143,#1564,.T.);
#12100=EDGE_CURVE('',#9145,#9146,#5819,.T.);
#12101=EDGE_CURVE('',#9146,#9144,#1565,.T.);
#12102=EDGE_CURVE('',#9143,#9145,#1566,.T.);
#12103=EDGE_CURVE('',#9147,#9148,#5820,.T.);
#12104=EDGE_CURVE('',#9148,#9146,#1567,.T.);
#12105=EDGE_CURVE('',#9145,#9147,#1568,.T.);
#12106=EDGE_CURVE('',#9149,#9150,#5821,.T.);
#12107=EDGE_CURVE('',#9150,#9148,#1569,.T.);
#12108=EDGE_CURVE('',#9147,#9149,#1570,.T.);
#12109=EDGE_CURVE('',#9151,#9152,#5822,.T.);
#12110=EDGE_CURVE('',#9152,#9150,#1571,.T.);
#12111=EDGE_CURVE('',#9149,#9151,#1572,.T.);
#12112=EDGE_CURVE('',#9153,#9154,#5823,.T.);
#12113=EDGE_CURVE('',#9154,#9152,#1573,.T.);
#12114=EDGE_CURVE('',#9151,#9153,#1574,.T.);
#12115=EDGE_CURVE('',#9155,#9156,#5824,.T.);
#12116=EDGE_CURVE('',#9156,#9154,#1575,.T.);
#12117=EDGE_CURVE('',#9153,#9155,#1576,.T.);
#12118=EDGE_CURVE('',#9157,#9158,#5825,.T.);
#12119=EDGE_CURVE('',#9158,#9156,#1577,.T.);
#12120=EDGE_CURVE('',#9155,#9157,#1578,.T.);
#12121=EDGE_CURVE('',#9159,#9160,#5826,.T.);
#12122=EDGE_CURVE('',#9160,#9158,#1579,.T.);
#12123=EDGE_CURVE('',#9157,#9159,#1580,.T.);
#12124=EDGE_CURVE('',#9161,#9162,#5827,.T.);
#12125=EDGE_CURVE('',#9162,#9160,#1581,.T.);
#12126=EDGE_CURVE('',#9159,#9161,#1582,.T.);
#12127=EDGE_CURVE('',#9163,#9164,#5828,.T.);
#12128=EDGE_CURVE('',#9164,#9162,#1583,.T.);
#12129=EDGE_CURVE('',#9161,#9163,#1584,.T.);
#12130=EDGE_CURVE('',#9165,#9166,#5829,.T.);
#12131=EDGE_CURVE('',#9166,#9164,#1585,.T.);
#12132=EDGE_CURVE('',#9163,#9165,#1586,.T.);
#12133=EDGE_CURVE('',#9167,#9168,#5830,.T.);
#12134=EDGE_CURVE('',#9168,#9166,#1587,.T.);
#12135=EDGE_CURVE('',#9165,#9167,#1588,.T.);
#12136=EDGE_CURVE('',#9169,#9170,#5831,.T.);
#12137=EDGE_CURVE('',#9170,#9168,#1589,.T.);
#12138=EDGE_CURVE('',#9167,#9169,#1590,.T.);
#12139=EDGE_CURVE('',#9171,#9172,#5832,.T.);
#12140=EDGE_CURVE('',#9172,#9170,#1591,.T.);
#12141=EDGE_CURVE('',#9169,#9171,#1592,.T.);
#12142=EDGE_CURVE('',#9173,#9174,#5833,.T.);
#12143=EDGE_CURVE('',#9174,#9172,#1593,.T.);
#12144=EDGE_CURVE('',#9171,#9173,#1594,.T.);
#12145=EDGE_CURVE('',#9175,#9176,#5834,.T.);
#12146=EDGE_CURVE('',#9176,#9174,#1595,.T.);
#12147=EDGE_CURVE('',#9173,#9175,#1596,.T.);
#12148=EDGE_CURVE('',#9177,#9178,#5835,.T.);
#12149=EDGE_CURVE('',#9177,#9179,#1597,.T.);
#12150=EDGE_CURVE('',#9180,#9179,#7579,.T.);
#12151=EDGE_CURVE('',#9180,#9178,#1598,.T.);
#12152=EDGE_CURVE('',#9181,#9182,#5836,.T.);
#12153=EDGE_CURVE('',#9182,#9183,#1599,.T.);
#12154=EDGE_CURVE('',#9184,#9183,#7580,.F.);
#12155=EDGE_CURVE('',#9184,#9181,#1600,.T.);
#12156=EDGE_CURVE('',#9185,#9186,#5837,.T.);
#12157=EDGE_CURVE('',#9186,#9182,#1601,.T.);
#12158=EDGE_CURVE('',#9181,#9185,#1602,.T.);
#12159=EDGE_CURVE('',#9187,#9188,#5838,.T.);
#12160=EDGE_CURVE('',#9188,#9186,#1603,.T.);
#12161=EDGE_CURVE('',#9185,#9187,#1604,.T.);
#12162=EDGE_CURVE('',#9189,#9190,#5839,.T.);
#12163=EDGE_CURVE('',#9190,#9188,#1605,.T.);
#12164=EDGE_CURVE('',#9187,#9189,#1606,.T.);
#12165=EDGE_CURVE('',#9191,#9192,#5840,.T.);
#12166=EDGE_CURVE('',#9192,#9190,#1607,.T.);
#12167=EDGE_CURVE('',#9189,#9191,#1608,.T.);
#12168=EDGE_CURVE('',#9193,#9194,#5841,.T.);
#12169=EDGE_CURVE('',#9194,#9192,#1609,.T.);
#12170=EDGE_CURVE('',#9191,#9193,#1610,.T.);
#12171=EDGE_CURVE('',#9195,#9196,#5842,.T.);
#12172=EDGE_CURVE('',#9196,#9194,#1611,.T.);
#12173=EDGE_CURVE('',#9193,#9195,#1612,.T.);
#12174=EDGE_CURVE('',#9197,#9198,#5843,.T.);
#12175=EDGE_CURVE('',#9198,#9196,#1613,.T.);
#12176=EDGE_CURVE('',#9195,#9197,#1614,.T.);
#12177=EDGE_CURVE('',#9199,#9200,#5844,.T.);
#12178=EDGE_CURVE('',#9200,#9198,#1615,.T.);
#12179=EDGE_CURVE('',#9197,#9199,#1616,.T.);
#12180=EDGE_CURVE('',#9201,#9202,#5845,.T.);
#12181=EDGE_CURVE('',#9202,#9200,#1617,.T.);
#12182=EDGE_CURVE('',#9199,#9201,#1618,.T.);
#12183=EDGE_CURVE('',#9203,#9204,#5846,.T.);
#12184=EDGE_CURVE('',#9204,#9202,#1619,.T.);
#12185=EDGE_CURVE('',#9201,#9203,#1620,.T.);
#12186=EDGE_CURVE('',#9205,#9206,#5847,.T.);
#12187=EDGE_CURVE('',#9206,#9204,#1621,.T.);
#12188=EDGE_CURVE('',#9203,#9205,#1622,.T.);
#12189=EDGE_CURVE('',#9207,#9208,#5848,.T.);
#12190=EDGE_CURVE('',#9208,#9206,#1623,.T.);
#12191=EDGE_CURVE('',#9205,#9207,#1624,.T.);
#12192=EDGE_CURVE('',#9209,#9210,#5849,.T.);
#12193=EDGE_CURVE('',#9210,#9208,#1625,.T.);
#12194=EDGE_CURVE('',#9207,#9209,#1626,.T.);
#12195=EDGE_CURVE('',#9211,#9212,#5850,.T.);
#12196=EDGE_CURVE('',#9212,#9210,#1627,.T.);
#12197=EDGE_CURVE('',#9209,#9211,#1628,.T.);
#12198=EDGE_CURVE('',#9213,#9214,#5851,.T.);
#12199=EDGE_CURVE('',#9214,#9212,#1629,.T.);
#12200=EDGE_CURVE('',#9211,#9213,#1630,.T.);
#12201=EDGE_CURVE('',#9215,#9216,#5852,.T.);
#12202=EDGE_CURVE('',#9216,#9214,#1631,.T.);
#12203=EDGE_CURVE('',#9213,#9215,#1632,.T.);
#12204=EDGE_CURVE('',#9217,#9218,#5853,.T.);
#12205=EDGE_CURVE('',#9218,#9216,#1633,.T.);
#12206=EDGE_CURVE('',#9215,#9217,#1634,.T.);
#12207=EDGE_CURVE('',#9219,#9220,#5854,.T.);
#12208=EDGE_CURVE('',#9220,#9218,#1635,.T.);
#12209=EDGE_CURVE('',#9217,#9219,#1636,.T.);
#12210=EDGE_CURVE('',#9221,#9222,#5855,.T.);
#12211=EDGE_CURVE('',#9221,#9223,#1637,.T.);
#12212=EDGE_CURVE('',#9224,#9223,#7581,.T.);
#12213=EDGE_CURVE('',#9224,#9222,#1638,.T.);
#12214=EDGE_CURVE('',#9225,#9226,#5856,.T.);
#12215=EDGE_CURVE('',#9226,#9227,#1639,.T.);
#12216=EDGE_CURVE('',#9228,#9227,#7582,.F.);
#12217=EDGE_CURVE('',#9228,#9225,#1640,.T.);
#12218=EDGE_CURVE('',#9229,#9230,#5857,.T.);
#12219=EDGE_CURVE('',#9230,#9226,#1641,.T.);
#12220=EDGE_CURVE('',#9225,#9229,#1642,.T.);
#12221=EDGE_CURVE('',#9231,#9232,#5858,.T.);
#12222=EDGE_CURVE('',#9232,#9230,#1643,.T.);
#12223=EDGE_CURVE('',#9229,#9231,#1644,.T.);
#12224=EDGE_CURVE('',#9233,#9234,#5859,.T.);
#12225=EDGE_CURVE('',#9234,#9232,#1645,.T.);
#12226=EDGE_CURVE('',#9231,#9233,#1646,.T.);
#12227=EDGE_CURVE('',#9235,#9236,#5860,.T.);
#12228=EDGE_CURVE('',#9236,#9234,#1647,.T.);
#12229=EDGE_CURVE('',#9233,#9235,#1648,.T.);
#12230=EDGE_CURVE('',#9237,#9238,#5861,.T.);
#12231=EDGE_CURVE('',#9238,#9236,#1649,.T.);
#12232=EDGE_CURVE('',#9235,#9237,#1650,.T.);
#12233=EDGE_CURVE('',#9239,#9240,#5862,.T.);
#12234=EDGE_CURVE('',#9240,#9238,#1651,.T.);
#12235=EDGE_CURVE('',#9237,#9239,#1652,.T.);
#12236=EDGE_CURVE('',#9241,#9242,#5863,.T.);
#12237=EDGE_CURVE('',#9242,#9240,#1653,.T.);
#12238=EDGE_CURVE('',#9239,#9241,#1654,.T.);
#12239=EDGE_CURVE('',#9243,#9244,#5864,.T.);
#12240=EDGE_CURVE('',#9244,#9242,#1655,.T.);
#12241=EDGE_CURVE('',#9241,#9243,#1656,.T.);
#12242=EDGE_CURVE('',#9245,#9246,#5865,.T.);
#12243=EDGE_CURVE('',#9246,#9244,#1657,.T.);
#12244=EDGE_CURVE('',#9243,#9245,#1658,.T.);
#12245=EDGE_CURVE('',#9247,#9248,#5866,.T.);
#12246=EDGE_CURVE('',#9248,#9246,#1659,.T.);
#12247=EDGE_CURVE('',#9245,#9247,#1660,.T.);
#12248=EDGE_CURVE('',#9249,#9250,#5867,.T.);
#12249=EDGE_CURVE('',#9250,#9248,#1661,.T.);
#12250=EDGE_CURVE('',#9247,#9249,#1662,.T.);
#12251=EDGE_CURVE('',#9251,#9252,#5868,.T.);
#12252=EDGE_CURVE('',#9252,#9250,#1663,.T.);
#12253=EDGE_CURVE('',#9249,#9251,#1664,.T.);
#12254=EDGE_CURVE('',#9253,#9254,#5869,.T.);
#12255=EDGE_CURVE('',#9254,#9252,#1665,.T.);
#12256=EDGE_CURVE('',#9251,#9253,#1666,.T.);
#12257=EDGE_CURVE('',#9255,#9256,#5870,.T.);
#12258=EDGE_CURVE('',#9256,#9254,#1667,.T.);
#12259=EDGE_CURVE('',#9253,#9255,#1668,.T.);
#12260=EDGE_CURVE('',#9257,#9258,#5871,.T.);
#12261=EDGE_CURVE('',#9258,#9256,#1669,.T.);
#12262=EDGE_CURVE('',#9255,#9257,#1670,.T.);
#12263=EDGE_CURVE('',#9259,#9260,#5872,.T.);
#12264=EDGE_CURVE('',#9260,#9258,#1671,.T.);
#12265=EDGE_CURVE('',#9257,#9259,#1672,.T.);
#12266=EDGE_CURVE('',#9261,#9262,#5873,.T.);
#12267=EDGE_CURVE('',#9262,#9260,#1673,.T.);
#12268=EDGE_CURVE('',#9259,#9261,#1674,.T.);
#12269=EDGE_CURVE('',#9263,#9264,#5874,.T.);
#12270=EDGE_CURVE('',#9264,#9262,#1675,.T.);
#12271=EDGE_CURVE('',#9261,#9263,#1676,.T.);
#12272=EDGE_CURVE('',#9265,#9266,#5875,.T.);
#12273=EDGE_CURVE('',#9265,#9267,#1677,.T.);
#12274=EDGE_CURVE('',#9268,#9267,#7583,.T.);
#12275=EDGE_CURVE('',#9268,#9266,#1678,.T.);
#12276=EDGE_CURVE('',#9269,#9270,#5876,.T.);
#12277=EDGE_CURVE('',#9270,#9271,#1679,.T.);
#12278=EDGE_CURVE('',#9272,#9271,#7584,.F.);
#12279=EDGE_CURVE('',#9272,#9269,#1680,.T.);
#12280=EDGE_CURVE('',#9273,#9274,#5877,.T.);
#12281=EDGE_CURVE('',#9274,#9270,#1681,.T.);
#12282=EDGE_CURVE('',#9269,#9273,#1682,.T.);
#12283=EDGE_CURVE('',#9275,#9276,#5878,.T.);
#12284=EDGE_CURVE('',#9276,#9274,#1683,.T.);
#12285=EDGE_CURVE('',#9273,#9275,#1684,.T.);
#12286=EDGE_CURVE('',#9277,#9278,#5879,.T.);
#12287=EDGE_CURVE('',#9278,#9276,#1685,.T.);
#12288=EDGE_CURVE('',#9275,#9277,#1686,.T.);
#12289=EDGE_CURVE('',#9279,#9280,#5880,.T.);
#12290=EDGE_CURVE('',#9280,#9278,#1687,.T.);
#12291=EDGE_CURVE('',#9277,#9279,#1688,.T.);
#12292=EDGE_CURVE('',#9281,#9282,#5881,.T.);
#12293=EDGE_CURVE('',#9282,#9280,#1689,.T.);
#12294=EDGE_CURVE('',#9279,#9281,#1690,.T.);
#12295=EDGE_CURVE('',#9283,#9284,#5882,.T.);
#12296=EDGE_CURVE('',#9284,#9282,#1691,.T.);
#12297=EDGE_CURVE('',#9281,#9283,#1692,.T.);
#12298=EDGE_CURVE('',#9285,#9286,#5883,.T.);
#12299=EDGE_CURVE('',#9286,#9284,#1693,.T.);
#12300=EDGE_CURVE('',#9283,#9285,#1694,.T.);
#12301=EDGE_CURVE('',#9287,#9288,#5884,.T.);
#12302=EDGE_CURVE('',#9288,#9286,#1695,.T.);
#12303=EDGE_CURVE('',#9285,#9287,#1696,.T.);
#12304=EDGE_CURVE('',#9289,#9290,#5885,.T.);
#12305=EDGE_CURVE('',#9290,#9288,#1697,.T.);
#12306=EDGE_CURVE('',#9287,#9289,#1698,.T.);
#12307=EDGE_CURVE('',#9291,#9292,#5886,.T.);
#12308=EDGE_CURVE('',#9292,#9290,#1699,.T.);
#12309=EDGE_CURVE('',#9289,#9291,#1700,.T.);
#12310=EDGE_CURVE('',#9293,#9294,#5887,.T.);
#12311=EDGE_CURVE('',#9294,#9292,#1701,.T.);
#12312=EDGE_CURVE('',#9291,#9293,#1702,.T.);
#12313=EDGE_CURVE('',#9295,#9296,#5888,.T.);
#12314=EDGE_CURVE('',#9296,#9294,#1703,.T.);
#12315=EDGE_CURVE('',#9293,#9295,#1704,.T.);
#12316=EDGE_CURVE('',#9297,#9298,#5889,.T.);
#12317=EDGE_CURVE('',#9298,#9296,#1705,.T.);
#12318=EDGE_CURVE('',#9295,#9297,#1706,.T.);
#12319=EDGE_CURVE('',#9299,#9300,#5890,.T.);
#12320=EDGE_CURVE('',#9300,#9298,#1707,.T.);
#12321=EDGE_CURVE('',#9297,#9299,#1708,.T.);
#12322=EDGE_CURVE('',#9301,#9302,#5891,.T.);
#12323=EDGE_CURVE('',#9302,#9300,#1709,.T.);
#12324=EDGE_CURVE('',#9299,#9301,#1710,.T.);
#12325=EDGE_CURVE('',#9303,#9304,#5892,.T.);
#12326=EDGE_CURVE('',#9304,#9302,#1711,.T.);
#12327=EDGE_CURVE('',#9301,#9303,#1712,.T.);
#12328=EDGE_CURVE('',#9305,#9306,#5893,.T.);
#12329=EDGE_CURVE('',#9306,#9304,#1713,.T.);
#12330=EDGE_CURVE('',#9303,#9305,#1714,.T.);
#12331=EDGE_CURVE('',#9307,#9308,#5894,.T.);
#12332=EDGE_CURVE('',#9308,#9306,#1715,.T.);
#12333=EDGE_CURVE('',#9305,#9307,#1716,.T.);
#12334=EDGE_CURVE('',#9309,#9310,#5895,.T.);
#12335=EDGE_CURVE('',#9309,#9311,#1717,.T.);
#12336=EDGE_CURVE('',#9312,#9311,#7585,.T.);
#12337=EDGE_CURVE('',#9312,#9310,#1718,.T.);
#12338=EDGE_CURVE('',#9313,#9314,#5896,.T.);
#12339=EDGE_CURVE('',#9314,#9315,#1719,.T.);
#12340=EDGE_CURVE('',#9316,#9315,#7586,.T.);
#12341=EDGE_CURVE('',#9313,#9316,#1720,.T.);
#12342=EDGE_CURVE('',#9317,#9318,#5897,.T.);
#12343=EDGE_CURVE('',#9318,#9314,#1721,.T.);
#12344=EDGE_CURVE('',#9317,#9313,#1722,.T.);
#12345=EDGE_CURVE('',#9319,#9320,#5898,.T.);
#12346=EDGE_CURVE('',#9320,#9318,#1723,.T.);
#12347=EDGE_CURVE('',#9319,#9317,#1724,.T.);
#12348=EDGE_CURVE('',#9321,#9322,#5899,.T.);
#12349=EDGE_CURVE('',#9322,#9320,#1725,.T.);
#12350=EDGE_CURVE('',#9321,#9319,#1726,.T.);
#12351=EDGE_CURVE('',#9323,#9324,#5900,.T.);
#12352=EDGE_CURVE('',#9324,#9322,#1727,.T.);
#12353=EDGE_CURVE('',#9323,#9321,#1728,.T.);
#12354=EDGE_CURVE('',#9325,#9326,#5901,.T.);
#12355=EDGE_CURVE('',#9326,#9324,#1729,.T.);
#12356=EDGE_CURVE('',#9325,#9323,#1730,.T.);
#12357=EDGE_CURVE('',#9327,#9328,#5902,.T.);
#12358=EDGE_CURVE('',#9328,#9326,#1731,.T.);
#12359=EDGE_CURVE('',#9327,#9325,#1732,.T.);
#12360=EDGE_CURVE('',#9329,#9330,#5903,.T.);
#12361=EDGE_CURVE('',#9330,#9328,#1733,.T.);
#12362=EDGE_CURVE('',#9329,#9327,#1734,.T.);
#12363=EDGE_CURVE('',#9331,#9332,#5904,.T.);
#12364=EDGE_CURVE('',#9332,#9330,#1735,.T.);
#12365=EDGE_CURVE('',#9331,#9329,#1736,.T.);
#12366=EDGE_CURVE('',#9333,#9334,#5905,.T.);
#12367=EDGE_CURVE('',#9334,#9332,#1737,.T.);
#12368=EDGE_CURVE('',#9333,#9331,#1738,.T.);
#12369=EDGE_CURVE('',#9335,#9336,#5906,.T.);
#12370=EDGE_CURVE('',#9336,#9334,#1739,.T.);
#12371=EDGE_CURVE('',#9335,#9333,#1740,.T.);
#12372=EDGE_CURVE('',#9337,#9338,#5907,.T.);
#12373=EDGE_CURVE('',#9338,#9336,#1741,.T.);
#12374=EDGE_CURVE('',#9337,#9335,#1742,.T.);
#12375=EDGE_CURVE('',#9339,#9340,#5908,.T.);
#12376=EDGE_CURVE('',#9340,#9338,#1743,.T.);
#12377=EDGE_CURVE('',#9339,#9337,#1744,.T.);
#12378=EDGE_CURVE('',#9341,#9342,#5909,.T.);
#12379=EDGE_CURVE('',#9342,#9340,#1745,.T.);
#12380=EDGE_CURVE('',#9341,#9339,#1746,.T.);
#12381=EDGE_CURVE('',#9343,#9344,#5910,.T.);
#12382=EDGE_CURVE('',#9344,#9342,#1747,.T.);
#12383=EDGE_CURVE('',#9343,#9341,#1748,.T.);
#12384=EDGE_CURVE('',#9345,#9346,#5911,.T.);
#12385=EDGE_CURVE('',#9346,#9344,#1749,.T.);
#12386=EDGE_CURVE('',#9345,#9343,#1750,.T.);
#12387=EDGE_CURVE('',#9347,#9348,#5912,.T.);
#12388=EDGE_CURVE('',#9348,#9346,#1751,.T.);
#12389=EDGE_CURVE('',#9347,#9345,#1752,.T.);
#12390=EDGE_CURVE('',#9349,#9350,#5913,.T.);
#12391=EDGE_CURVE('',#9350,#9348,#1753,.T.);
#12392=EDGE_CURVE('',#9349,#9347,#1754,.T.);
#12393=EDGE_CURVE('',#9351,#9352,#5914,.T.);
#12394=EDGE_CURVE('',#9352,#9350,#1755,.T.);
#12395=EDGE_CURVE('',#9351,#9349,#1756,.T.);
#12396=EDGE_CURVE('',#9353,#9354,#5915,.T.);
#12397=EDGE_CURVE('',#9355,#9353,#1757,.T.);
#12398=EDGE_CURVE('',#9356,#9355,#7587,.T.);
#12399=EDGE_CURVE('',#9356,#9354,#1758,.T.);
#12400=EDGE_CURVE('',#9357,#9358,#5916,.T.);
#12401=EDGE_CURVE('',#9358,#9359,#1759,.T.);
#12402=EDGE_CURVE('',#9360,#9359,#7588,.T.);
#12403=EDGE_CURVE('',#9357,#9360,#1760,.T.);
#12404=EDGE_CURVE('',#9361,#9362,#5917,.T.);
#12405=EDGE_CURVE('',#9362,#9358,#1761,.T.);
#12406=EDGE_CURVE('',#9361,#9357,#1762,.T.);
#12407=EDGE_CURVE('',#9363,#9364,#5918,.T.);
#12408=EDGE_CURVE('',#9364,#9362,#1763,.T.);
#12409=EDGE_CURVE('',#9363,#9361,#1764,.T.);
#12410=EDGE_CURVE('',#9365,#9366,#5919,.T.);
#12411=EDGE_CURVE('',#9366,#9364,#1765,.T.);
#12412=EDGE_CURVE('',#9365,#9363,#1766,.T.);
#12413=EDGE_CURVE('',#9367,#9368,#5920,.T.);
#12414=EDGE_CURVE('',#9368,#9366,#1767,.T.);
#12415=EDGE_CURVE('',#9367,#9365,#1768,.T.);
#12416=EDGE_CURVE('',#9369,#9370,#5921,.T.);
#12417=EDGE_CURVE('',#9370,#9368,#1769,.T.);
#12418=EDGE_CURVE('',#9369,#9367,#1770,.T.);
#12419=EDGE_CURVE('',#9371,#9372,#5922,.T.);
#12420=EDGE_CURVE('',#9372,#9370,#1771,.T.);
#12421=EDGE_CURVE('',#9371,#9369,#1772,.T.);
#12422=EDGE_CURVE('',#9373,#9374,#5923,.T.);
#12423=EDGE_CURVE('',#9374,#9372,#1773,.T.);
#12424=EDGE_CURVE('',#9373,#9371,#1774,.T.);
#12425=EDGE_CURVE('',#9375,#9376,#5924,.T.);
#12426=EDGE_CURVE('',#9376,#9374,#1775,.T.);
#12427=EDGE_CURVE('',#9375,#9373,#1776,.T.);
#12428=EDGE_CURVE('',#9377,#9378,#5925,.T.);
#12429=EDGE_CURVE('',#9378,#9376,#1777,.T.);
#12430=EDGE_CURVE('',#9377,#9375,#1778,.T.);
#12431=EDGE_CURVE('',#9379,#9380,#5926,.T.);
#12432=EDGE_CURVE('',#9380,#9378,#1779,.T.);
#12433=EDGE_CURVE('',#9379,#9377,#1780,.T.);
#12434=EDGE_CURVE('',#9381,#9382,#5927,.T.);
#12435=EDGE_CURVE('',#9382,#9380,#1781,.T.);
#12436=EDGE_CURVE('',#9381,#9379,#1782,.T.);
#12437=EDGE_CURVE('',#9383,#9384,#5928,.T.);
#12438=EDGE_CURVE('',#9384,#9382,#1783,.T.);
#12439=EDGE_CURVE('',#9383,#9381,#1784,.T.);
#12440=EDGE_CURVE('',#9385,#9386,#5929,.T.);
#12441=EDGE_CURVE('',#9386,#9384,#1785,.T.);
#12442=EDGE_CURVE('',#9385,#9383,#1786,.T.);
#12443=EDGE_CURVE('',#9387,#9388,#5930,.T.);
#12444=EDGE_CURVE('',#9388,#9386,#1787,.T.);
#12445=EDGE_CURVE('',#9387,#9385,#1788,.T.);
#12446=EDGE_CURVE('',#9389,#9390,#5931,.T.);
#12447=EDGE_CURVE('',#9390,#9388,#1789,.T.);
#12448=EDGE_CURVE('',#9389,#9387,#1790,.T.);
#12449=EDGE_CURVE('',#9391,#9392,#5932,.T.);
#12450=EDGE_CURVE('',#9392,#9390,#1791,.T.);
#12451=EDGE_CURVE('',#9391,#9389,#1792,.T.);
#12452=EDGE_CURVE('',#9393,#9394,#5933,.T.);
#12453=EDGE_CURVE('',#9394,#9392,#1793,.T.);
#12454=EDGE_CURVE('',#9393,#9391,#1794,.T.);
#12455=EDGE_CURVE('',#9395,#9396,#5934,.T.);
#12456=EDGE_CURVE('',#9396,#9394,#1795,.T.);
#12457=EDGE_CURVE('',#9395,#9393,#1796,.T.);
#12458=EDGE_CURVE('',#9397,#9398,#5935,.T.);
#12459=EDGE_CURVE('',#9399,#9397,#1797,.T.);
#12460=EDGE_CURVE('',#9400,#9399,#7589,.T.);
#12461=EDGE_CURVE('',#9400,#9398,#1798,.T.);
#12462=EDGE_CURVE('',#9401,#9402,#5936,.T.);
#12463=EDGE_CURVE('',#9402,#9403,#1799,.T.);
#12464=EDGE_CURVE('',#9404,#9403,#7590,.T.);
#12465=EDGE_CURVE('',#9401,#9404,#1800,.T.);
#12466=EDGE_CURVE('',#9405,#9406,#5937,.T.);
#12467=EDGE_CURVE('',#9406,#9402,#1801,.T.);
#12468=EDGE_CURVE('',#9405,#9401,#1802,.T.);
#12469=EDGE_CURVE('',#9407,#9408,#5938,.T.);
#12470=EDGE_CURVE('',#9408,#9406,#1803,.T.);
#12471=EDGE_CURVE('',#9407,#9405,#1804,.T.);
#12472=EDGE_CURVE('',#9409,#9410,#5939,.T.);
#12473=EDGE_CURVE('',#9410,#9408,#1805,.T.);
#12474=EDGE_CURVE('',#9409,#9407,#1806,.T.);
#12475=EDGE_CURVE('',#9411,#9412,#5940,.T.);
#12476=EDGE_CURVE('',#9412,#9410,#1807,.T.);
#12477=EDGE_CURVE('',#9411,#9409,#1808,.T.);
#12478=EDGE_CURVE('',#9413,#9414,#5941,.T.);
#12479=EDGE_CURVE('',#9414,#9412,#1809,.T.);
#12480=EDGE_CURVE('',#9413,#9411,#1810,.T.);
#12481=EDGE_CURVE('',#9415,#9416,#5942,.T.);
#12482=EDGE_CURVE('',#9416,#9414,#1811,.T.);
#12483=EDGE_CURVE('',#9415,#9413,#1812,.T.);
#12484=EDGE_CURVE('',#9417,#9418,#5943,.T.);
#12485=EDGE_CURVE('',#9418,#9416,#1813,.T.);
#12486=EDGE_CURVE('',#9417,#9415,#1814,.T.);
#12487=EDGE_CURVE('',#9419,#9420,#5944,.T.);
#12488=EDGE_CURVE('',#9420,#9418,#1815,.T.);
#12489=EDGE_CURVE('',#9419,#9417,#1816,.T.);
#12490=EDGE_CURVE('',#9421,#9422,#5945,.T.);
#12491=EDGE_CURVE('',#9422,#9420,#1817,.T.);
#12492=EDGE_CURVE('',#9421,#9419,#1818,.T.);
#12493=EDGE_CURVE('',#9423,#9424,#5946,.T.);
#12494=EDGE_CURVE('',#9424,#9422,#1819,.T.);
#12495=EDGE_CURVE('',#9423,#9421,#1820,.T.);
#12496=EDGE_CURVE('',#9425,#9426,#5947,.T.);
#12497=EDGE_CURVE('',#9426,#9424,#1821,.T.);
#12498=EDGE_CURVE('',#9425,#9423,#1822,.T.);
#12499=EDGE_CURVE('',#9427,#9428,#5948,.T.);
#12500=EDGE_CURVE('',#9428,#9426,#1823,.T.);
#12501=EDGE_CURVE('',#9427,#9425,#1824,.T.);
#12502=EDGE_CURVE('',#9429,#9430,#5949,.T.);
#12503=EDGE_CURVE('',#9430,#9428,#1825,.T.);
#12504=EDGE_CURVE('',#9429,#9427,#1826,.T.);
#12505=EDGE_CURVE('',#9431,#9432,#5950,.T.);
#12506=EDGE_CURVE('',#9432,#9430,#1827,.T.);
#12507=EDGE_CURVE('',#9431,#9429,#1828,.T.);
#12508=EDGE_CURVE('',#9433,#9434,#5951,.T.);
#12509=EDGE_CURVE('',#9434,#9432,#1829,.T.);
#12510=EDGE_CURVE('',#9433,#9431,#1830,.T.);
#12511=EDGE_CURVE('',#9435,#9436,#5952,.T.);
#12512=EDGE_CURVE('',#9436,#9434,#1831,.T.);
#12513=EDGE_CURVE('',#9435,#9433,#1832,.T.);
#12514=EDGE_CURVE('',#9437,#9438,#5953,.T.);
#12515=EDGE_CURVE('',#9438,#9436,#1833,.T.);
#12516=EDGE_CURVE('',#9437,#9435,#1834,.T.);
#12517=EDGE_CURVE('',#9439,#9440,#5954,.T.);
#12518=EDGE_CURVE('',#9440,#9438,#1835,.T.);
#12519=EDGE_CURVE('',#9439,#9437,#1836,.T.);
#12520=EDGE_CURVE('',#9441,#9442,#5955,.T.);
#12521=EDGE_CURVE('',#9443,#9441,#1837,.T.);
#12522=EDGE_CURVE('',#9444,#9443,#7591,.T.);
#12523=EDGE_CURVE('',#9444,#9442,#1838,.T.);
#12524=EDGE_CURVE('',#9445,#9446,#5956,.T.);
#12525=EDGE_CURVE('',#9446,#9447,#1839,.T.);
#12526=EDGE_CURVE('',#9448,#9447,#7592,.T.);
#12527=EDGE_CURVE('',#9445,#9448,#1840,.T.);
#12528=EDGE_CURVE('',#9449,#9450,#5957,.T.);
#12529=EDGE_CURVE('',#9450,#9446,#1841,.T.);
#12530=EDGE_CURVE('',#9449,#9445,#1842,.T.);
#12531=EDGE_CURVE('',#9451,#9452,#5958,.T.);
#12532=EDGE_CURVE('',#9452,#9450,#1843,.T.);
#12533=EDGE_CURVE('',#9451,#9449,#1844,.T.);
#12534=EDGE_CURVE('',#9453,#9454,#5959,.T.);
#12535=EDGE_CURVE('',#9454,#9452,#1845,.T.);
#12536=EDGE_CURVE('',#9453,#9451,#1846,.T.);
#12537=EDGE_CURVE('',#9455,#9456,#5960,.T.);
#12538=EDGE_CURVE('',#9456,#9454,#1847,.T.);
#12539=EDGE_CURVE('',#9455,#9453,#1848,.T.);
#12540=EDGE_CURVE('',#9457,#9458,#5961,.T.);
#12541=EDGE_CURVE('',#9458,#9456,#1849,.T.);
#12542=EDGE_CURVE('',#9457,#9455,#1850,.T.);
#12543=EDGE_CURVE('',#9459,#9460,#5962,.T.);
#12544=EDGE_CURVE('',#9460,#9458,#1851,.T.);
#12545=EDGE_CURVE('',#9459,#9457,#1852,.T.);
#12546=EDGE_CURVE('',#9461,#9462,#5963,.T.);
#12547=EDGE_CURVE('',#9462,#9460,#1853,.T.);
#12548=EDGE_CURVE('',#9461,#9459,#1854,.T.);
#12549=EDGE_CURVE('',#9463,#9464,#5964,.T.);
#12550=EDGE_CURVE('',#9464,#9462,#1855,.T.);
#12551=EDGE_CURVE('',#9463,#9461,#1856,.T.);
#12552=EDGE_CURVE('',#9465,#9466,#5965,.T.);
#12553=EDGE_CURVE('',#9466,#9464,#1857,.T.);
#12554=EDGE_CURVE('',#9465,#9463,#1858,.T.);
#12555=EDGE_CURVE('',#9467,#9468,#5966,.T.);
#12556=EDGE_CURVE('',#9468,#9466,#1859,.T.);
#12557=EDGE_CURVE('',#9467,#9465,#1860,.T.);
#12558=EDGE_CURVE('',#9469,#9470,#5967,.T.);
#12559=EDGE_CURVE('',#9470,#9468,#1861,.T.);
#12560=EDGE_CURVE('',#9469,#9467,#1862,.T.);
#12561=EDGE_CURVE('',#9471,#9472,#5968,.T.);
#12562=EDGE_CURVE('',#9472,#9470,#1863,.T.);
#12563=EDGE_CURVE('',#9471,#9469,#1864,.T.);
#12564=EDGE_CURVE('',#9473,#9474,#5969,.T.);
#12565=EDGE_CURVE('',#9474,#9472,#1865,.T.);
#12566=EDGE_CURVE('',#9473,#9471,#1866,.T.);
#12567=EDGE_CURVE('',#9475,#9476,#5970,.T.);
#12568=EDGE_CURVE('',#9476,#9474,#1867,.T.);
#12569=EDGE_CURVE('',#9475,#9473,#1868,.T.);
#12570=EDGE_CURVE('',#9477,#9478,#5971,.T.);
#12571=EDGE_CURVE('',#9478,#9476,#1869,.T.);
#12572=EDGE_CURVE('',#9477,#9475,#1870,.T.);
#12573=EDGE_CURVE('',#9479,#9480,#5972,.T.);
#12574=EDGE_CURVE('',#9480,#9478,#1871,.T.);
#12575=EDGE_CURVE('',#9479,#9477,#1872,.T.);
#12576=EDGE_CURVE('',#9481,#9482,#5973,.T.);
#12577=EDGE_CURVE('',#9482,#9480,#1873,.T.);
#12578=EDGE_CURVE('',#9481,#9479,#1874,.T.);
#12579=EDGE_CURVE('',#9483,#9484,#5974,.T.);
#12580=EDGE_CURVE('',#9484,#9482,#1875,.T.);
#12581=EDGE_CURVE('',#9483,#9481,#1876,.T.);
#12582=EDGE_CURVE('',#9485,#9486,#5975,.T.);
#12583=EDGE_CURVE('',#9487,#9485,#1877,.T.);
#12584=EDGE_CURVE('',#9488,#9487,#7593,.T.);
#12585=EDGE_CURVE('',#9488,#9486,#1878,.T.);
#12586=EDGE_CURVE('',#9489,#9490,#5976,.T.);
#12587=EDGE_CURVE('',#9490,#9491,#1879,.T.);
#12588=EDGE_CURVE('',#9492,#9491,#7594,.T.);
#12589=EDGE_CURVE('',#9489,#9492,#1880,.T.);
#12590=EDGE_CURVE('',#9493,#9494,#5977,.T.);
#12591=EDGE_CURVE('',#9494,#9490,#1881,.T.);
#12592=EDGE_CURVE('',#9493,#9489,#1882,.T.);
#12593=EDGE_CURVE('',#9495,#9496,#5978,.T.);
#12594=EDGE_CURVE('',#9496,#9494,#1883,.T.);
#12595=EDGE_CURVE('',#9495,#9493,#1884,.T.);
#12596=EDGE_CURVE('',#9497,#9498,#5979,.T.);
#12597=EDGE_CURVE('',#9498,#9496,#1885,.T.);
#12598=EDGE_CURVE('',#9497,#9495,#1886,.T.);
#12599=EDGE_CURVE('',#9499,#9500,#5980,.T.);
#12600=EDGE_CURVE('',#9500,#9498,#1887,.T.);
#12601=EDGE_CURVE('',#9499,#9497,#1888,.T.);
#12602=EDGE_CURVE('',#9501,#9502,#5981,.T.);
#12603=EDGE_CURVE('',#9502,#9500,#1889,.T.);
#12604=EDGE_CURVE('',#9501,#9499,#1890,.T.);
#12605=EDGE_CURVE('',#9503,#9504,#5982,.T.);
#12606=EDGE_CURVE('',#9504,#9502,#1891,.T.);
#12607=EDGE_CURVE('',#9503,#9501,#1892,.T.);
#12608=EDGE_CURVE('',#9505,#9506,#5983,.T.);
#12609=EDGE_CURVE('',#9506,#9504,#1893,.T.);
#12610=EDGE_CURVE('',#9505,#9503,#1894,.T.);
#12611=EDGE_CURVE('',#9507,#9508,#5984,.T.);
#12612=EDGE_CURVE('',#9508,#9506,#1895,.T.);
#12613=EDGE_CURVE('',#9507,#9505,#1896,.T.);
#12614=EDGE_CURVE('',#9509,#9510,#5985,.T.);
#12615=EDGE_CURVE('',#9510,#9508,#1897,.T.);
#12616=EDGE_CURVE('',#9509,#9507,#1898,.T.);
#12617=EDGE_CURVE('',#9511,#9512,#5986,.T.);
#12618=EDGE_CURVE('',#9512,#9510,#1899,.T.);
#12619=EDGE_CURVE('',#9511,#9509,#1900,.T.);
#12620=EDGE_CURVE('',#9513,#9514,#5987,.T.);
#12621=EDGE_CURVE('',#9514,#9512,#1901,.T.);
#12622=EDGE_CURVE('',#9513,#9511,#1902,.T.);
#12623=EDGE_CURVE('',#9515,#9516,#5988,.T.);
#12624=EDGE_CURVE('',#9516,#9514,#1903,.T.);
#12625=EDGE_CURVE('',#9515,#9513,#1904,.T.);
#12626=EDGE_CURVE('',#9517,#9518,#5989,.T.);
#12627=EDGE_CURVE('',#9518,#9516,#1905,.T.);
#12628=EDGE_CURVE('',#9517,#9515,#1906,.T.);
#12629=EDGE_CURVE('',#9519,#9520,#5990,.T.);
#12630=EDGE_CURVE('',#9520,#9518,#1907,.T.);
#12631=EDGE_CURVE('',#9519,#9517,#1908,.T.);
#12632=EDGE_CURVE('',#9521,#9522,#5991,.T.);
#12633=EDGE_CURVE('',#9522,#9520,#1909,.T.);
#12634=EDGE_CURVE('',#9521,#9519,#1910,.T.);
#12635=EDGE_CURVE('',#9523,#9524,#5992,.T.);
#12636=EDGE_CURVE('',#9524,#9522,#1911,.T.);
#12637=EDGE_CURVE('',#9523,#9521,#1912,.T.);
#12638=EDGE_CURVE('',#9525,#9526,#5993,.T.);
#12639=EDGE_CURVE('',#9526,#9524,#1913,.T.);
#12640=EDGE_CURVE('',#9525,#9523,#1914,.T.);
#12641=EDGE_CURVE('',#9527,#9528,#5994,.T.);
#12642=EDGE_CURVE('',#9528,#9526,#1915,.T.);
#12643=EDGE_CURVE('',#9527,#9525,#1916,.T.);
#12644=EDGE_CURVE('',#9529,#9530,#5995,.T.);
#12645=EDGE_CURVE('',#9531,#9529,#1917,.T.);
#12646=EDGE_CURVE('',#9532,#9531,#7595,.T.);
#12647=EDGE_CURVE('',#9532,#9530,#1918,.T.);
#12648=EDGE_CURVE('',#9533,#9534,#5996,.T.);
#12649=EDGE_CURVE('',#9534,#9535,#1919,.T.);
#12650=EDGE_CURVE('',#9536,#9535,#7596,.T.);
#12651=EDGE_CURVE('',#9533,#9536,#1920,.T.);
#12652=EDGE_CURVE('',#9537,#9538,#5997,.T.);
#12653=EDGE_CURVE('',#9538,#9534,#1921,.T.);
#12654=EDGE_CURVE('',#9537,#9533,#1922,.T.);
#12655=EDGE_CURVE('',#9539,#9540,#5998,.T.);
#12656=EDGE_CURVE('',#9540,#9538,#1923,.T.);
#12657=EDGE_CURVE('',#9539,#9537,#1924,.T.);
#12658=EDGE_CURVE('',#9541,#9542,#5999,.T.);
#12659=EDGE_CURVE('',#9542,#9540,#1925,.T.);
#12660=EDGE_CURVE('',#9541,#9539,#1926,.T.);
#12661=EDGE_CURVE('',#9543,#9544,#6000,.T.);
#12662=EDGE_CURVE('',#9544,#9542,#1927,.T.);
#12663=EDGE_CURVE('',#9543,#9541,#1928,.T.);
#12664=EDGE_CURVE('',#9545,#9546,#6001,.T.);
#12665=EDGE_CURVE('',#9546,#9544,#1929,.T.);
#12666=EDGE_CURVE('',#9545,#9543,#1930,.T.);
#12667=EDGE_CURVE('',#9547,#9548,#6002,.T.);
#12668=EDGE_CURVE('',#9548,#9546,#1931,.T.);
#12669=EDGE_CURVE('',#9547,#9545,#1932,.T.);
#12670=EDGE_CURVE('',#9549,#9550,#6003,.T.);
#12671=EDGE_CURVE('',#9550,#9548,#1933,.T.);
#12672=EDGE_CURVE('',#9549,#9547,#1934,.T.);
#12673=EDGE_CURVE('',#9551,#9552,#6004,.T.);
#12674=EDGE_CURVE('',#9552,#9550,#1935,.T.);
#12675=EDGE_CURVE('',#9551,#9549,#1936,.T.);
#12676=EDGE_CURVE('',#9553,#9554,#6005,.T.);
#12677=EDGE_CURVE('',#9554,#9552,#1937,.T.);
#12678=EDGE_CURVE('',#9553,#9551,#1938,.T.);
#12679=EDGE_CURVE('',#9555,#9556,#6006,.T.);
#12680=EDGE_CURVE('',#9556,#9554,#1939,.T.);
#12681=EDGE_CURVE('',#9555,#9553,#1940,.T.);
#12682=EDGE_CURVE('',#9557,#9558,#6007,.T.);
#12683=EDGE_CURVE('',#9558,#9556,#1941,.T.);
#12684=EDGE_CURVE('',#9557,#9555,#1942,.T.);
#12685=EDGE_CURVE('',#9559,#9560,#6008,.T.);
#12686=EDGE_CURVE('',#9560,#9558,#1943,.T.);
#12687=EDGE_CURVE('',#9559,#9557,#1944,.T.);
#12688=EDGE_CURVE('',#9561,#9562,#6009,.T.);
#12689=EDGE_CURVE('',#9562,#9560,#1945,.T.);
#12690=EDGE_CURVE('',#9561,#9559,#1946,.T.);
#12691=EDGE_CURVE('',#9563,#9564,#6010,.T.);
#12692=EDGE_CURVE('',#9564,#9562,#1947,.T.);
#12693=EDGE_CURVE('',#9563,#9561,#1948,.T.);
#12694=EDGE_CURVE('',#9565,#9566,#6011,.T.);
#12695=EDGE_CURVE('',#9566,#9564,#1949,.T.);
#12696=EDGE_CURVE('',#9565,#9563,#1950,.T.);
#12697=EDGE_CURVE('',#9567,#9568,#6012,.T.);
#12698=EDGE_CURVE('',#9568,#9566,#1951,.T.);
#12699=EDGE_CURVE('',#9567,#9565,#1952,.T.);
#12700=EDGE_CURVE('',#9569,#9570,#6013,.T.);
#12701=EDGE_CURVE('',#9570,#9568,#1953,.T.);
#12702=EDGE_CURVE('',#9569,#9567,#1954,.T.);
#12703=EDGE_CURVE('',#9571,#9572,#6014,.T.);
#12704=EDGE_CURVE('',#9572,#9570,#1955,.T.);
#12705=EDGE_CURVE('',#9571,#9569,#1956,.T.);
#12706=EDGE_CURVE('',#9573,#9574,#6015,.T.);
#12707=EDGE_CURVE('',#9575,#9573,#1957,.T.);
#12708=EDGE_CURVE('',#9576,#9575,#7597,.T.);
#12709=EDGE_CURVE('',#9576,#9574,#1958,.T.);
#12710=EDGE_CURVE('',#9574,#9572,#1959,.T.);
#12711=EDGE_CURVE('',#9573,#9571,#1960,.T.);
#12712=EDGE_CURVE('',#9535,#9140,#1961,.T.);
#12713=EDGE_CURVE('',#9179,#9576,#1962,.T.);
#12714=EDGE_CURVE('',#9175,#9177,#1963,.T.);
#12715=EDGE_CURVE('',#9139,#9536,#1964,.T.);
#12716=EDGE_CURVE('',#9178,#9176,#1965,.T.);
#12717=EDGE_CURVE('',#9575,#9180,#1966,.T.);
#12718=EDGE_CURVE('',#9577,#9578,#6016,.T.);
#12719=EDGE_CURVE('',#9578,#9579,#6017,.T.);
#12720=EDGE_CURVE('',#9579,#9580,#6018,.T.);
#12721=EDGE_CURVE('',#9580,#9577,#6019,.T.);
#12722=EDGE_CURVE('',#9091,#9400,#1967,.T.);
#12723=EDGE_CURVE('',#9399,#9092,#1968,.T.);
#12724=EDGE_CURVE('',#9135,#9444,#1969,.T.);
#12725=EDGE_CURVE('',#9443,#9136,#1970,.T.);
#12726=EDGE_CURVE('',#9223,#9488,#1971,.T.);
#12727=EDGE_CURVE('',#9487,#9224,#1972,.T.);
#12728=EDGE_CURVE('',#9267,#9532,#1973,.T.);
#12729=EDGE_CURVE('',#9531,#9268,#1974,.T.);
#12730=EDGE_CURVE('',#9311,#9356,#1975,.T.);
#12731=EDGE_CURVE('',#9355,#9312,#1976,.T.);
#12732=EDGE_CURVE('',#9530,#9528,#1977,.T.);
#12733=EDGE_CURVE('',#9529,#9527,#1978,.T.);
#12734=EDGE_CURVE('',#9491,#9228,#1979,.T.);
#12735=EDGE_CURVE('',#9263,#9265,#1980,.T.);
#12736=EDGE_CURVE('',#9227,#9492,#1981,.T.);
#12737=EDGE_CURVE('',#9266,#9264,#1982,.T.);
#12738=EDGE_CURVE('',#9486,#9484,#1983,.T.);
#12739=EDGE_CURVE('',#9485,#9483,#1984,.T.);
#12740=EDGE_CURVE('',#9447,#9184,#1985,.T.);
#12741=EDGE_CURVE('',#9219,#9221,#1986,.T.);
#12742=EDGE_CURVE('',#9183,#9448,#1987,.T.);
#12743=EDGE_CURVE('',#9222,#9220,#1988,.T.);
#12744=EDGE_CURVE('',#9442,#9440,#1989,.T.);
#12745=EDGE_CURVE('',#9441,#9439,#1990,.T.);
#12746=EDGE_CURVE('',#9403,#9096,#1991,.T.);
#12747=EDGE_CURVE('',#9131,#9133,#1992,.T.);
#12748=EDGE_CURVE('',#9095,#9404,#1993,.T.);
#12749=EDGE_CURVE('',#9134,#9132,#1994,.T.);
#12750=EDGE_CURVE('',#9398,#9396,#1995,.T.);
#12751=EDGE_CURVE('',#9397,#9395,#1996,.T.);
#12752=EDGE_CURVE('',#9359,#9052,#1997,.T.);
#12753=EDGE_CURVE('',#9087,#9089,#1998,.T.);
#12754=EDGE_CURVE('',#9051,#9360,#1999,.T.);
#12755=EDGE_CURVE('',#9090,#9088,#2000,.T.);
#12756=EDGE_CURVE('',#9354,#9352,#2001,.T.);
#12757=EDGE_CURVE('',#9353,#9351,#2002,.T.);
#12758=EDGE_CURVE('',#9315,#9272,#2003,.T.);
#12759=EDGE_CURVE('',#9307,#9309,#2004,.T.);
#12760=EDGE_CURVE('',#9271,#9316,#2005,.T.);
#12761=EDGE_CURVE('',#9310,#9308,#2006,.T.);
#12762=EDGE_CURVE('',#9581,#9582,#6020,.T.);
#12763=EDGE_CURVE('',#9582,#9577,#6021,.T.);
#12764=EDGE_CURVE('',#9581,#9580,#6022,.T.);
#12765=EDGE_CURVE('',#9583,#9581,#6023,.T.);
#12766=EDGE_CURVE('',#9583,#9579,#6024,.T.);
#12767=EDGE_CURVE('',#9584,#9583,#6025,.T.);
#12768=EDGE_CURVE('',#9584,#9578,#6026,.T.);
#12769=EDGE_CURVE('',#9582,#9584,#6027,.T.);
#17418=ORIENTED_EDGE('',*,*,#11966,.T.);
#17419=ORIENTED_EDGE('',*,*,#11967,.T.);
#17420=ORIENTED_EDGE('',*,*,#11968,.F.);
#17421=ORIENTED_EDGE('',*,*,#11969,.T.);
#17422=ORIENTED_EDGE('',*,*,#11970,.T.);
#17423=ORIENTED_EDGE('',*,*,#11971,.T.);
#17424=ORIENTED_EDGE('',*,*,#11966,.F.);
#17425=ORIENTED_EDGE('',*,*,#11972,.T.);
#17426=ORIENTED_EDGE('',*,*,#11973,.T.);
#17427=ORIENTED_EDGE('',*,*,#11974,.T.);
#17428=ORIENTED_EDGE('',*,*,#11970,.F.);
#17429=ORIENTED_EDGE('',*,*,#11975,.T.);
#17430=ORIENTED_EDGE('',*,*,#11976,.T.);
#17431=ORIENTED_EDGE('',*,*,#11977,.T.);
#17432=ORIENTED_EDGE('',*,*,#11973,.F.);
#17433=ORIENTED_EDGE('',*,*,#11978,.T.);
#17434=ORIENTED_EDGE('',*,*,#11979,.T.);
#17435=ORIENTED_EDGE('',*,*,#11980,.T.);
#17436=ORIENTED_EDGE('',*,*,#11976,.F.);
#17437=ORIENTED_EDGE('',*,*,#11981,.T.);
#17438=ORIENTED_EDGE('',*,*,#11982,.T.);
#17439=ORIENTED_EDGE('',*,*,#11983,.T.);
#17440=ORIENTED_EDGE('',*,*,#11979,.F.);
#17441=ORIENTED_EDGE('',*,*,#11984,.T.);
#17442=ORIENTED_EDGE('',*,*,#11985,.T.);
#17443=ORIENTED_EDGE('',*,*,#11986,.T.);
#17444=ORIENTED_EDGE('',*,*,#11982,.F.);
#17445=ORIENTED_EDGE('',*,*,#11987,.T.);
#17446=ORIENTED_EDGE('',*,*,#11988,.T.);
#17447=ORIENTED_EDGE('',*,*,#11989,.T.);
#17448=ORIENTED_EDGE('',*,*,#11985,.F.);
#17449=ORIENTED_EDGE('',*,*,#11990,.T.);
#17450=ORIENTED_EDGE('',*,*,#11991,.T.);
#17451=ORIENTED_EDGE('',*,*,#11992,.T.);
#17452=ORIENTED_EDGE('',*,*,#11988,.F.);
#17453=ORIENTED_EDGE('',*,*,#11993,.T.);
#17454=ORIENTED_EDGE('',*,*,#11994,.T.);
#17455=ORIENTED_EDGE('',*,*,#11995,.T.);
#17456=ORIENTED_EDGE('',*,*,#11991,.F.);
#17457=ORIENTED_EDGE('',*,*,#11996,.T.);
#17458=ORIENTED_EDGE('',*,*,#11997,.T.);
#17459=ORIENTED_EDGE('',*,*,#11998,.T.);
#17460=ORIENTED_EDGE('',*,*,#11994,.F.);
#17461=ORIENTED_EDGE('',*,*,#11999,.T.);
#17462=ORIENTED_EDGE('',*,*,#12000,.T.);
#17463=ORIENTED_EDGE('',*,*,#12001,.T.);
#17464=ORIENTED_EDGE('',*,*,#11997,.F.);
#17465=ORIENTED_EDGE('',*,*,#12002,.T.);
#17466=ORIENTED_EDGE('',*,*,#12003,.T.);
#17467=ORIENTED_EDGE('',*,*,#12004,.T.);
#17468=ORIENTED_EDGE('',*,*,#12000,.F.);
#17469=ORIENTED_EDGE('',*,*,#12005,.T.);
#17470=ORIENTED_EDGE('',*,*,#12006,.T.);
#17471=ORIENTED_EDGE('',*,*,#12007,.T.);
#17472=ORIENTED_EDGE('',*,*,#12003,.F.);
#17473=ORIENTED_EDGE('',*,*,#12008,.T.);
#17474=ORIENTED_EDGE('',*,*,#12009,.T.);
#17475=ORIENTED_EDGE('',*,*,#12010,.T.);
#17476=ORIENTED_EDGE('',*,*,#12006,.F.);
#17477=ORIENTED_EDGE('',*,*,#12011,.T.);
#17478=ORIENTED_EDGE('',*,*,#12012,.T.);
#17479=ORIENTED_EDGE('',*,*,#12013,.T.);
#17480=ORIENTED_EDGE('',*,*,#12009,.F.);
#17481=ORIENTED_EDGE('',*,*,#12014,.T.);
#17482=ORIENTED_EDGE('',*,*,#12015,.T.);
#17483=ORIENTED_EDGE('',*,*,#12016,.T.);
#17484=ORIENTED_EDGE('',*,*,#12012,.F.);
#17485=ORIENTED_EDGE('',*,*,#12017,.T.);
#17486=ORIENTED_EDGE('',*,*,#12018,.T.);
#17487=ORIENTED_EDGE('',*,*,#12019,.T.);
#17488=ORIENTED_EDGE('',*,*,#12015,.F.);
#17489=ORIENTED_EDGE('',*,*,#12020,.T.);
#17490=ORIENTED_EDGE('',*,*,#12021,.T.);
#17491=ORIENTED_EDGE('',*,*,#12022,.T.);
#17492=ORIENTED_EDGE('',*,*,#12018,.F.);
#17493=ORIENTED_EDGE('',*,*,#12023,.T.);
#17494=ORIENTED_EDGE('',*,*,#12024,.F.);
#17495=ORIENTED_EDGE('',*,*,#12025,.T.);
#17496=ORIENTED_EDGE('',*,*,#12026,.F.);
#17497=ORIENTED_EDGE('',*,*,#12027,.T.);
#17498=ORIENTED_EDGE('',*,*,#12028,.T.);
#17499=ORIENTED_EDGE('',*,*,#12029,.T.);
#17500=ORIENTED_EDGE('',*,*,#12030,.F.);
#17501=ORIENTED_EDGE('',*,*,#12031,.T.);
#17502=ORIENTED_EDGE('',*,*,#12032,.T.);
#17503=ORIENTED_EDGE('',*,*,#12033,.T.);
#17504=ORIENTED_EDGE('',*,*,#12028,.F.);
#17505=ORIENTED_EDGE('',*,*,#12034,.T.);
#17506=ORIENTED_EDGE('',*,*,#12035,.T.);
#17507=ORIENTED_EDGE('',*,*,#12036,.T.);
#17508=ORIENTED_EDGE('',*,*,#12032,.F.);
#17509=ORIENTED_EDGE('',*,*,#12037,.T.);
#17510=ORIENTED_EDGE('',*,*,#12038,.T.);
#17511=ORIENTED_EDGE('',*,*,#12039,.T.);
#17512=ORIENTED_EDGE('',*,*,#12035,.F.);
#17513=ORIENTED_EDGE('',*,*,#12040,.T.);
#17514=ORIENTED_EDGE('',*,*,#12041,.T.);
#17515=ORIENTED_EDGE('',*,*,#12042,.T.);
#17516=ORIENTED_EDGE('',*,*,#12038,.F.);
#17517=ORIENTED_EDGE('',*,*,#12043,.T.);
#17518=ORIENTED_EDGE('',*,*,#12044,.T.);
#17519=ORIENTED_EDGE('',*,*,#12045,.T.);
#17520=ORIENTED_EDGE('',*,*,#12041,.F.);
#17521=ORIENTED_EDGE('',*,*,#12046,.T.);
#17522=ORIENTED_EDGE('',*,*,#12047,.T.);
#17523=ORIENTED_EDGE('',*,*,#12048,.T.);
#17524=ORIENTED_EDGE('',*,*,#12044,.F.);
#17525=ORIENTED_EDGE('',*,*,#12049,.T.);
#17526=ORIENTED_EDGE('',*,*,#12050,.T.);
#17527=ORIENTED_EDGE('',*,*,#12051,.T.);
#17528=ORIENTED_EDGE('',*,*,#12047,.F.);
#17529=ORIENTED_EDGE('',*,*,#12052,.T.);
#17530=ORIENTED_EDGE('',*,*,#12053,.T.);
#17531=ORIENTED_EDGE('',*,*,#12054,.T.);
#17532=ORIENTED_EDGE('',*,*,#12050,.F.);
#17533=ORIENTED_EDGE('',*,*,#12055,.T.);
#17534=ORIENTED_EDGE('',*,*,#12056,.T.);
#17535=ORIENTED_EDGE('',*,*,#12057,.T.);
#17536=ORIENTED_EDGE('',*,*,#12053,.F.);
#17537=ORIENTED_EDGE('',*,*,#12058,.T.);
#17538=ORIENTED_EDGE('',*,*,#12059,.T.);
#17539=ORIENTED_EDGE('',*,*,#12060,.T.);
#17540=ORIENTED_EDGE('',*,*,#12056,.F.);
#17541=ORIENTED_EDGE('',*,*,#12061,.T.);
#17542=ORIENTED_EDGE('',*,*,#12062,.T.);
#17543=ORIENTED_EDGE('',*,*,#12063,.T.);
#17544=ORIENTED_EDGE('',*,*,#12059,.F.);
#17545=ORIENTED_EDGE('',*,*,#12064,.T.);
#17546=ORIENTED_EDGE('',*,*,#12065,.T.);
#17547=ORIENTED_EDGE('',*,*,#12066,.T.);
#17548=ORIENTED_EDGE('',*,*,#12062,.F.);
#17549=ORIENTED_EDGE('',*,*,#12067,.T.);
#17550=ORIENTED_EDGE('',*,*,#12068,.T.);
#17551=ORIENTED_EDGE('',*,*,#12069,.T.);
#17552=ORIENTED_EDGE('',*,*,#12065,.F.);
#17553=ORIENTED_EDGE('',*,*,#12070,.T.);
#17554=ORIENTED_EDGE('',*,*,#12071,.T.);
#17555=ORIENTED_EDGE('',*,*,#12072,.T.);
#17556=ORIENTED_EDGE('',*,*,#12068,.F.);
#17557=ORIENTED_EDGE('',*,*,#12073,.T.);
#17558=ORIENTED_EDGE('',*,*,#12074,.T.);
#17559=ORIENTED_EDGE('',*,*,#12075,.T.);
#17560=ORIENTED_EDGE('',*,*,#12071,.F.);
#17561=ORIENTED_EDGE('',*,*,#12076,.T.);
#17562=ORIENTED_EDGE('',*,*,#12077,.T.);
#17563=ORIENTED_EDGE('',*,*,#12078,.T.);
#17564=ORIENTED_EDGE('',*,*,#12074,.F.);
#17565=ORIENTED_EDGE('',*,*,#12079,.T.);
#17566=ORIENTED_EDGE('',*,*,#12080,.T.);
#17567=ORIENTED_EDGE('',*,*,#12081,.T.);
#17568=ORIENTED_EDGE('',*,*,#12077,.F.);
#17569=ORIENTED_EDGE('',*,*,#12082,.T.);
#17570=ORIENTED_EDGE('',*,*,#12083,.T.);
#17571=ORIENTED_EDGE('',*,*,#12084,.T.);
#17572=ORIENTED_EDGE('',*,*,#12080,.F.);
#17573=ORIENTED_EDGE('',*,*,#12085,.T.);
#17574=ORIENTED_EDGE('',*,*,#12086,.F.);
#17575=ORIENTED_EDGE('',*,*,#12087,.T.);
#17576=ORIENTED_EDGE('',*,*,#12088,.F.);
#17577=ORIENTED_EDGE('',*,*,#12089,.T.);
#17578=ORIENTED_EDGE('',*,*,#12090,.T.);
#17579=ORIENTED_EDGE('',*,*,#12091,.T.);
#17580=ORIENTED_EDGE('',*,*,#12092,.F.);
#17581=ORIENTED_EDGE('',*,*,#12093,.T.);
#17582=ORIENTED_EDGE('',*,*,#12094,.T.);
#17583=ORIENTED_EDGE('',*,*,#12095,.T.);
#17584=ORIENTED_EDGE('',*,*,#12090,.F.);
#17585=ORIENTED_EDGE('',*,*,#12096,.T.);
#17586=ORIENTED_EDGE('',*,*,#12097,.T.);
#17587=ORIENTED_EDGE('',*,*,#12098,.T.);
#17588=ORIENTED_EDGE('',*,*,#12094,.F.);
#17589=ORIENTED_EDGE('',*,*,#12099,.T.);
#17590=ORIENTED_EDGE('',*,*,#12100,.T.);
#17591=ORIENTED_EDGE('',*,*,#12101,.T.);
#17592=ORIENTED_EDGE('',*,*,#12097,.F.);
#17593=ORIENTED_EDGE('',*,*,#12102,.T.);
#17594=ORIENTED_EDGE('',*,*,#12103,.T.);
#17595=ORIENTED_EDGE('',*,*,#12104,.T.);
#17596=ORIENTED_EDGE('',*,*,#12100,.F.);
#17597=ORIENTED_EDGE('',*,*,#12105,.T.);
#17598=ORIENTED_EDGE('',*,*,#12106,.T.);
#17599=ORIENTED_EDGE('',*,*,#12107,.T.);
#17600=ORIENTED_EDGE('',*,*,#12103,.F.);
#17601=ORIENTED_EDGE('',*,*,#12108,.T.);
#17602=ORIENTED_EDGE('',*,*,#12109,.T.);
#17603=ORIENTED_EDGE('',*,*,#12110,.T.);
#17604=ORIENTED_EDGE('',*,*,#12106,.F.);
#17605=ORIENTED_EDGE('',*,*,#12111,.T.);
#17606=ORIENTED_EDGE('',*,*,#12112,.T.);
#17607=ORIENTED_EDGE('',*,*,#12113,.T.);
#17608=ORIENTED_EDGE('',*,*,#12109,.F.);
#17609=ORIENTED_EDGE('',*,*,#12114,.T.);
#17610=ORIENTED_EDGE('',*,*,#12115,.T.);
#17611=ORIENTED_EDGE('',*,*,#12116,.T.);
#17612=ORIENTED_EDGE('',*,*,#12112,.F.);
#17613=ORIENTED_EDGE('',*,*,#12117,.T.);
#17614=ORIENTED_EDGE('',*,*,#12118,.T.);
#17615=ORIENTED_EDGE('',*,*,#12119,.T.);
#17616=ORIENTED_EDGE('',*,*,#12115,.F.);
#17617=ORIENTED_EDGE('',*,*,#12120,.T.);
#17618=ORIENTED_EDGE('',*,*,#12121,.T.);
#17619=ORIENTED_EDGE('',*,*,#12122,.T.);
#17620=ORIENTED_EDGE('',*,*,#12118,.F.);
#17621=ORIENTED_EDGE('',*,*,#12123,.T.);
#17622=ORIENTED_EDGE('',*,*,#12124,.T.);
#17623=ORIENTED_EDGE('',*,*,#12125,.T.);
#17624=ORIENTED_EDGE('',*,*,#12121,.F.);
#17625=ORIENTED_EDGE('',*,*,#12126,.T.);
#17626=ORIENTED_EDGE('',*,*,#12127,.T.);
#17627=ORIENTED_EDGE('',*,*,#12128,.T.);
#17628=ORIENTED_EDGE('',*,*,#12124,.F.);
#17629=ORIENTED_EDGE('',*,*,#12129,.T.);
#17630=ORIENTED_EDGE('',*,*,#12130,.T.);
#17631=ORIENTED_EDGE('',*,*,#12131,.T.);
#17632=ORIENTED_EDGE('',*,*,#12127,.F.);
#17633=ORIENTED_EDGE('',*,*,#12132,.T.);
#17634=ORIENTED_EDGE('',*,*,#12133,.T.);
#17635=ORIENTED_EDGE('',*,*,#12134,.T.);
#17636=ORIENTED_EDGE('',*,*,#12130,.F.);
#17637=ORIENTED_EDGE('',*,*,#12135,.T.);
#17638=ORIENTED_EDGE('',*,*,#12136,.T.);
#17639=ORIENTED_EDGE('',*,*,#12137,.T.);
#17640=ORIENTED_EDGE('',*,*,#12133,.F.);
#17641=ORIENTED_EDGE('',*,*,#12138,.T.);
#17642=ORIENTED_EDGE('',*,*,#12139,.T.);
#17643=ORIENTED_EDGE('',*,*,#12140,.T.);
#17644=ORIENTED_EDGE('',*,*,#12136,.F.);
#17645=ORIENTED_EDGE('',*,*,#12141,.T.);
#17646=ORIENTED_EDGE('',*,*,#12142,.T.);
#17647=ORIENTED_EDGE('',*,*,#12143,.T.);
#17648=ORIENTED_EDGE('',*,*,#12139,.F.);
#17649=ORIENTED_EDGE('',*,*,#12144,.T.);
#17650=ORIENTED_EDGE('',*,*,#12145,.T.);
#17651=ORIENTED_EDGE('',*,*,#12146,.T.);
#17652=ORIENTED_EDGE('',*,*,#12142,.F.);
#17653=ORIENTED_EDGE('',*,*,#12147,.T.);
#17654=ORIENTED_EDGE('',*,*,#12148,.F.);
#17655=ORIENTED_EDGE('',*,*,#12149,.T.);
#17656=ORIENTED_EDGE('',*,*,#12150,.F.);
#17657=ORIENTED_EDGE('',*,*,#12151,.T.);
#17658=ORIENTED_EDGE('',*,*,#12152,.T.);
#17659=ORIENTED_EDGE('',*,*,#12153,.T.);
#17660=ORIENTED_EDGE('',*,*,#12154,.F.);
#17661=ORIENTED_EDGE('',*,*,#12155,.T.);
#17662=ORIENTED_EDGE('',*,*,#12156,.T.);
#17663=ORIENTED_EDGE('',*,*,#12157,.T.);
#17664=ORIENTED_EDGE('',*,*,#12152,.F.);
#17665=ORIENTED_EDGE('',*,*,#12158,.T.);
#17666=ORIENTED_EDGE('',*,*,#12159,.T.);
#17667=ORIENTED_EDGE('',*,*,#12160,.T.);
#17668=ORIENTED_EDGE('',*,*,#12156,.F.);
#17669=ORIENTED_EDGE('',*,*,#12161,.T.);
#17670=ORIENTED_EDGE('',*,*,#12162,.T.);
#17671=ORIENTED_EDGE('',*,*,#12163,.T.);
#17672=ORIENTED_EDGE('',*,*,#12159,.F.);
#17673=ORIENTED_EDGE('',*,*,#12164,.T.);
#17674=ORIENTED_EDGE('',*,*,#12165,.T.);
#17675=ORIENTED_EDGE('',*,*,#12166,.T.);
#17676=ORIENTED_EDGE('',*,*,#12162,.F.);
#17677=ORIENTED_EDGE('',*,*,#12167,.T.);
#17678=ORIENTED_EDGE('',*,*,#12168,.T.);
#17679=ORIENTED_EDGE('',*,*,#12169,.T.);
#17680=ORIENTED_EDGE('',*,*,#12165,.F.);
#17681=ORIENTED_EDGE('',*,*,#12170,.T.);
#17682=ORIENTED_EDGE('',*,*,#12171,.T.);
#17683=ORIENTED_EDGE('',*,*,#12172,.T.);
#17684=ORIENTED_EDGE('',*,*,#12168,.F.);
#17685=ORIENTED_EDGE('',*,*,#12173,.T.);
#17686=ORIENTED_EDGE('',*,*,#12174,.T.);
#17687=ORIENTED_EDGE('',*,*,#12175,.T.);
#17688=ORIENTED_EDGE('',*,*,#12171,.F.);
#17689=ORIENTED_EDGE('',*,*,#12176,.T.);
#17690=ORIENTED_EDGE('',*,*,#12177,.T.);
#17691=ORIENTED_EDGE('',*,*,#12178,.T.);
#17692=ORIENTED_EDGE('',*,*,#12174,.F.);
#17693=ORIENTED_EDGE('',*,*,#12179,.T.);
#17694=ORIENTED_EDGE('',*,*,#12180,.T.);
#17695=ORIENTED_EDGE('',*,*,#12181,.T.);
#17696=ORIENTED_EDGE('',*,*,#12177,.F.);
#17697=ORIENTED_EDGE('',*,*,#12182,.T.);
#17698=ORIENTED_EDGE('',*,*,#12183,.T.);
#17699=ORIENTED_EDGE('',*,*,#12184,.T.);
#17700=ORIENTED_EDGE('',*,*,#12180,.F.);
#17701=ORIENTED_EDGE('',*,*,#12185,.T.);
#17702=ORIENTED_EDGE('',*,*,#12186,.T.);
#17703=ORIENTED_EDGE('',*,*,#12187,.T.);
#17704=ORIENTED_EDGE('',*,*,#12183,.F.);
#17705=ORIENTED_EDGE('',*,*,#12188,.T.);
#17706=ORIENTED_EDGE('',*,*,#12189,.T.);
#17707=ORIENTED_EDGE('',*,*,#12190,.T.);
#17708=ORIENTED_EDGE('',*,*,#12186,.F.);
#17709=ORIENTED_EDGE('',*,*,#12191,.T.);
#17710=ORIENTED_EDGE('',*,*,#12192,.T.);
#17711=ORIENTED_EDGE('',*,*,#12193,.T.);
#17712=ORIENTED_EDGE('',*,*,#12189,.F.);
#17713=ORIENTED_EDGE('',*,*,#12194,.T.);
#17714=ORIENTED_EDGE('',*,*,#12195,.T.);
#17715=ORIENTED_EDGE('',*,*,#12196,.T.);
#17716=ORIENTED_EDGE('',*,*,#12192,.F.);
#17717=ORIENTED_EDGE('',*,*,#12197,.T.);
#17718=ORIENTED_EDGE('',*,*,#12198,.T.);
#17719=ORIENTED_EDGE('',*,*,#12199,.T.);
#17720=ORIENTED_EDGE('',*,*,#12195,.F.);
#17721=ORIENTED_EDGE('',*,*,#12200,.T.);
#17722=ORIENTED_EDGE('',*,*,#12201,.T.);
#17723=ORIENTED_EDGE('',*,*,#12202,.T.);
#17724=ORIENTED_EDGE('',*,*,#12198,.F.);
#17725=ORIENTED_EDGE('',*,*,#12203,.T.);
#17726=ORIENTED_EDGE('',*,*,#12204,.T.);
#17727=ORIENTED_EDGE('',*,*,#12205,.T.);
#17728=ORIENTED_EDGE('',*,*,#12201,.F.);
#17729=ORIENTED_EDGE('',*,*,#12206,.T.);
#17730=ORIENTED_EDGE('',*,*,#12207,.T.);
#17731=ORIENTED_EDGE('',*,*,#12208,.T.);
#17732=ORIENTED_EDGE('',*,*,#12204,.F.);
#17733=ORIENTED_EDGE('',*,*,#12209,.T.);
#17734=ORIENTED_EDGE('',*,*,#12210,.F.);
#17735=ORIENTED_EDGE('',*,*,#12211,.T.);
#17736=ORIENTED_EDGE('',*,*,#12212,.F.);
#17737=ORIENTED_EDGE('',*,*,#12213,.T.);
#17738=ORIENTED_EDGE('',*,*,#12214,.T.);
#17739=ORIENTED_EDGE('',*,*,#12215,.T.);
#17740=ORIENTED_EDGE('',*,*,#12216,.F.);
#17741=ORIENTED_EDGE('',*,*,#12217,.T.);
#17742=ORIENTED_EDGE('',*,*,#12218,.T.);
#17743=ORIENTED_EDGE('',*,*,#12219,.T.);
#17744=ORIENTED_EDGE('',*,*,#12214,.F.);
#17745=ORIENTED_EDGE('',*,*,#12220,.T.);
#17746=ORIENTED_EDGE('',*,*,#12221,.T.);
#17747=ORIENTED_EDGE('',*,*,#12222,.T.);
#17748=ORIENTED_EDGE('',*,*,#12218,.F.);
#17749=ORIENTED_EDGE('',*,*,#12223,.T.);
#17750=ORIENTED_EDGE('',*,*,#12224,.T.);
#17751=ORIENTED_EDGE('',*,*,#12225,.T.);
#17752=ORIENTED_EDGE('',*,*,#12221,.F.);
#17753=ORIENTED_EDGE('',*,*,#12226,.T.);
#17754=ORIENTED_EDGE('',*,*,#12227,.T.);
#17755=ORIENTED_EDGE('',*,*,#12228,.T.);
#17756=ORIENTED_EDGE('',*,*,#12224,.F.);
#17757=ORIENTED_EDGE('',*,*,#12229,.T.);
#17758=ORIENTED_EDGE('',*,*,#12230,.T.);
#17759=ORIENTED_EDGE('',*,*,#12231,.T.);
#17760=ORIENTED_EDGE('',*,*,#12227,.F.);
#17761=ORIENTED_EDGE('',*,*,#12232,.T.);
#17762=ORIENTED_EDGE('',*,*,#12233,.T.);
#17763=ORIENTED_EDGE('',*,*,#12234,.T.);
#17764=ORIENTED_EDGE('',*,*,#12230,.F.);
#17765=ORIENTED_EDGE('',*,*,#12235,.T.);
#17766=ORIENTED_EDGE('',*,*,#12236,.T.);
#17767=ORIENTED_EDGE('',*,*,#12237,.T.);
#17768=ORIENTED_EDGE('',*,*,#12233,.F.);
#17769=ORIENTED_EDGE('',*,*,#12238,.T.);
#17770=ORIENTED_EDGE('',*,*,#12239,.T.);
#17771=ORIENTED_EDGE('',*,*,#12240,.T.);
#17772=ORIENTED_EDGE('',*,*,#12236,.F.);
#17773=ORIENTED_EDGE('',*,*,#12241,.T.);
#17774=ORIENTED_EDGE('',*,*,#12242,.T.);
#17775=ORIENTED_EDGE('',*,*,#12243,.T.);
#17776=ORIENTED_EDGE('',*,*,#12239,.F.);
#17777=ORIENTED_EDGE('',*,*,#12244,.T.);
#17778=ORIENTED_EDGE('',*,*,#12245,.T.);
#17779=ORIENTED_EDGE('',*,*,#12246,.T.);
#17780=ORIENTED_EDGE('',*,*,#12242,.F.);
#17781=ORIENTED_EDGE('',*,*,#12247,.T.);
#17782=ORIENTED_EDGE('',*,*,#12248,.T.);
#17783=ORIENTED_EDGE('',*,*,#12249,.T.);
#17784=ORIENTED_EDGE('',*,*,#12245,.F.);
#17785=ORIENTED_EDGE('',*,*,#12250,.T.);
#17786=ORIENTED_EDGE('',*,*,#12251,.T.);
#17787=ORIENTED_EDGE('',*,*,#12252,.T.);
#17788=ORIENTED_EDGE('',*,*,#12248,.F.);
#17789=ORIENTED_EDGE('',*,*,#12253,.T.);
#17790=ORIENTED_EDGE('',*,*,#12254,.T.);
#17791=ORIENTED_EDGE('',*,*,#12255,.T.);
#17792=ORIENTED_EDGE('',*,*,#12251,.F.);
#17793=ORIENTED_EDGE('',*,*,#12256,.T.);
#17794=ORIENTED_EDGE('',*,*,#12257,.T.);
#17795=ORIENTED_EDGE('',*,*,#12258,.T.);
#17796=ORIENTED_EDGE('',*,*,#12254,.F.);
#17797=ORIENTED_EDGE('',*,*,#12259,.T.);
#17798=ORIENTED_EDGE('',*,*,#12260,.T.);
#17799=ORIENTED_EDGE('',*,*,#12261,.T.);
#17800=ORIENTED_EDGE('',*,*,#12257,.F.);
#17801=ORIENTED_EDGE('',*,*,#12262,.T.);
#17802=ORIENTED_EDGE('',*,*,#12263,.T.);
#17803=ORIENTED_EDGE('',*,*,#12264,.T.);
#17804=ORIENTED_EDGE('',*,*,#12260,.F.);
#17805=ORIENTED_EDGE('',*,*,#12265,.T.);
#17806=ORIENTED_EDGE('',*,*,#12266,.T.);
#17807=ORIENTED_EDGE('',*,*,#12267,.T.);
#17808=ORIENTED_EDGE('',*,*,#12263,.F.);
#17809=ORIENTED_EDGE('',*,*,#12268,.T.);
#17810=ORIENTED_EDGE('',*,*,#12269,.T.);
#17811=ORIENTED_EDGE('',*,*,#12270,.T.);
#17812=ORIENTED_EDGE('',*,*,#12266,.F.);
#17813=ORIENTED_EDGE('',*,*,#12271,.T.);
#17814=ORIENTED_EDGE('',*,*,#12272,.F.);
#17815=ORIENTED_EDGE('',*,*,#12273,.T.);
#17816=ORIENTED_EDGE('',*,*,#12274,.F.);
#17817=ORIENTED_EDGE('',*,*,#12275,.T.);
#17818=ORIENTED_EDGE('',*,*,#12276,.T.);
#17819=ORIENTED_EDGE('',*,*,#12277,.T.);
#17820=ORIENTED_EDGE('',*,*,#12278,.F.);
#17821=ORIENTED_EDGE('',*,*,#12279,.T.);
#17822=ORIENTED_EDGE('',*,*,#12280,.T.);
#17823=ORIENTED_EDGE('',*,*,#12281,.T.);
#17824=ORIENTED_EDGE('',*,*,#12276,.F.);
#17825=ORIENTED_EDGE('',*,*,#12282,.T.);
#17826=ORIENTED_EDGE('',*,*,#12283,.T.);
#17827=ORIENTED_EDGE('',*,*,#12284,.T.);
#17828=ORIENTED_EDGE('',*,*,#12280,.F.);
#17829=ORIENTED_EDGE('',*,*,#12285,.T.);
#17830=ORIENTED_EDGE('',*,*,#12286,.T.);
#17831=ORIENTED_EDGE('',*,*,#12287,.T.);
#17832=ORIENTED_EDGE('',*,*,#12283,.F.);
#17833=ORIENTED_EDGE('',*,*,#12288,.T.);
#17834=ORIENTED_EDGE('',*,*,#12289,.T.);
#17835=ORIENTED_EDGE('',*,*,#12290,.T.);
#17836=ORIENTED_EDGE('',*,*,#12286,.F.);
#17837=ORIENTED_EDGE('',*,*,#12291,.T.);
#17838=ORIENTED_EDGE('',*,*,#12292,.T.);
#17839=ORIENTED_EDGE('',*,*,#12293,.T.);
#17840=ORIENTED_EDGE('',*,*,#12289,.F.);
#17841=ORIENTED_EDGE('',*,*,#12294,.T.);
#17842=ORIENTED_EDGE('',*,*,#12295,.T.);
#17843=ORIENTED_EDGE('',*,*,#12296,.T.);
#17844=ORIENTED_EDGE('',*,*,#12292,.F.);
#17845=ORIENTED_EDGE('',*,*,#12297,.T.);
#17846=ORIENTED_EDGE('',*,*,#12298,.T.);
#17847=ORIENTED_EDGE('',*,*,#12299,.T.);
#17848=ORIENTED_EDGE('',*,*,#12295,.F.);
#17849=ORIENTED_EDGE('',*,*,#12300,.T.);
#17850=ORIENTED_EDGE('',*,*,#12301,.T.);
#17851=ORIENTED_EDGE('',*,*,#12302,.T.);
#17852=ORIENTED_EDGE('',*,*,#12298,.F.);
#17853=ORIENTED_EDGE('',*,*,#12303,.T.);
#17854=ORIENTED_EDGE('',*,*,#12304,.T.);
#17855=ORIENTED_EDGE('',*,*,#12305,.T.);
#17856=ORIENTED_EDGE('',*,*,#12301,.F.);
#17857=ORIENTED_EDGE('',*,*,#12306,.T.);
#17858=ORIENTED_EDGE('',*,*,#12307,.T.);
#17859=ORIENTED_EDGE('',*,*,#12308,.T.);
#17860=ORIENTED_EDGE('',*,*,#12304,.F.);
#17861=ORIENTED_EDGE('',*,*,#12309,.T.);
#17862=ORIENTED_EDGE('',*,*,#12310,.T.);
#17863=ORIENTED_EDGE('',*,*,#12311,.T.);
#17864=ORIENTED_EDGE('',*,*,#12307,.F.);
#17865=ORIENTED_EDGE('',*,*,#12312,.T.);
#17866=ORIENTED_EDGE('',*,*,#12313,.T.);
#17867=ORIENTED_EDGE('',*,*,#12314,.T.);
#17868=ORIENTED_EDGE('',*,*,#12310,.F.);
#17869=ORIENTED_EDGE('',*,*,#12315,.T.);
#17870=ORIENTED_EDGE('',*,*,#12316,.T.);
#17871=ORIENTED_EDGE('',*,*,#12317,.T.);
#17872=ORIENTED_EDGE('',*,*,#12313,.F.);
#17873=ORIENTED_EDGE('',*,*,#12318,.T.);
#17874=ORIENTED_EDGE('',*,*,#12319,.T.);
#17875=ORIENTED_EDGE('',*,*,#12320,.T.);
#17876=ORIENTED_EDGE('',*,*,#12316,.F.);
#17877=ORIENTED_EDGE('',*,*,#12321,.T.);
#17878=ORIENTED_EDGE('',*,*,#12322,.T.);
#17879=ORIENTED_EDGE('',*,*,#12323,.T.);
#17880=ORIENTED_EDGE('',*,*,#12319,.F.);
#17881=ORIENTED_EDGE('',*,*,#12324,.T.);
#17882=ORIENTED_EDGE('',*,*,#12325,.T.);
#17883=ORIENTED_EDGE('',*,*,#12326,.T.);
#17884=ORIENTED_EDGE('',*,*,#12322,.F.);
#17885=ORIENTED_EDGE('',*,*,#12327,.T.);
#17886=ORIENTED_EDGE('',*,*,#12328,.T.);
#17887=ORIENTED_EDGE('',*,*,#12329,.T.);
#17888=ORIENTED_EDGE('',*,*,#12325,.F.);
#17889=ORIENTED_EDGE('',*,*,#12330,.T.);
#17890=ORIENTED_EDGE('',*,*,#12331,.T.);
#17891=ORIENTED_EDGE('',*,*,#12332,.T.);
#17892=ORIENTED_EDGE('',*,*,#12328,.F.);
#17893=ORIENTED_EDGE('',*,*,#12333,.T.);
#17894=ORIENTED_EDGE('',*,*,#12334,.F.);
#17895=ORIENTED_EDGE('',*,*,#12335,.T.);
#17896=ORIENTED_EDGE('',*,*,#12336,.F.);
#17897=ORIENTED_EDGE('',*,*,#12337,.T.);
#17898=ORIENTED_EDGE('',*,*,#12338,.T.);
#17899=ORIENTED_EDGE('',*,*,#12339,.T.);
#17900=ORIENTED_EDGE('',*,*,#12340,.F.);
#17901=ORIENTED_EDGE('',*,*,#12341,.F.);
#17902=ORIENTED_EDGE('',*,*,#12342,.T.);
#17903=ORIENTED_EDGE('',*,*,#12343,.T.);
#17904=ORIENTED_EDGE('',*,*,#12338,.F.);
#17905=ORIENTED_EDGE('',*,*,#12344,.F.);
#17906=ORIENTED_EDGE('',*,*,#12345,.T.);
#17907=ORIENTED_EDGE('',*,*,#12346,.T.);
#17908=ORIENTED_EDGE('',*,*,#12342,.F.);
#17909=ORIENTED_EDGE('',*,*,#12347,.F.);
#17910=ORIENTED_EDGE('',*,*,#12348,.T.);
#17911=ORIENTED_EDGE('',*,*,#12349,.T.);
#17912=ORIENTED_EDGE('',*,*,#12345,.F.);
#17913=ORIENTED_EDGE('',*,*,#12350,.F.);
#17914=ORIENTED_EDGE('',*,*,#12351,.T.);
#17915=ORIENTED_EDGE('',*,*,#12352,.T.);
#17916=ORIENTED_EDGE('',*,*,#12348,.F.);
#17917=ORIENTED_EDGE('',*,*,#12353,.F.);
#17918=ORIENTED_EDGE('',*,*,#12354,.T.);
#17919=ORIENTED_EDGE('',*,*,#12355,.T.);
#17920=ORIENTED_EDGE('',*,*,#12351,.F.);
#17921=ORIENTED_EDGE('',*,*,#12356,.F.);
#17922=ORIENTED_EDGE('',*,*,#12357,.T.);
#17923=ORIENTED_EDGE('',*,*,#12358,.T.);
#17924=ORIENTED_EDGE('',*,*,#12354,.F.);
#17925=ORIENTED_EDGE('',*,*,#12359,.F.);
#17926=ORIENTED_EDGE('',*,*,#12360,.T.);
#17927=ORIENTED_EDGE('',*,*,#12361,.T.);
#17928=ORIENTED_EDGE('',*,*,#12357,.F.);
#17929=ORIENTED_EDGE('',*,*,#12362,.F.);
#17930=ORIENTED_EDGE('',*,*,#12363,.T.);
#17931=ORIENTED_EDGE('',*,*,#12364,.T.);
#17932=ORIENTED_EDGE('',*,*,#12360,.F.);
#17933=ORIENTED_EDGE('',*,*,#12365,.F.);
#17934=ORIENTED_EDGE('',*,*,#12366,.T.);
#17935=ORIENTED_EDGE('',*,*,#12367,.T.);
#17936=ORIENTED_EDGE('',*,*,#12363,.F.);
#17937=ORIENTED_EDGE('',*,*,#12368,.F.);
#17938=ORIENTED_EDGE('',*,*,#12369,.T.);
#17939=ORIENTED_EDGE('',*,*,#12370,.T.);
#17940=ORIENTED_EDGE('',*,*,#12366,.F.);
#17941=ORIENTED_EDGE('',*,*,#12371,.F.);
#17942=ORIENTED_EDGE('',*,*,#12372,.T.);
#17943=ORIENTED_EDGE('',*,*,#12373,.T.);
#17944=ORIENTED_EDGE('',*,*,#12369,.F.);
#17945=ORIENTED_EDGE('',*,*,#12374,.F.);
#17946=ORIENTED_EDGE('',*,*,#12375,.T.);
#17947=ORIENTED_EDGE('',*,*,#12376,.T.);
#17948=ORIENTED_EDGE('',*,*,#12372,.F.);
#17949=ORIENTED_EDGE('',*,*,#12377,.F.);
#17950=ORIENTED_EDGE('',*,*,#12378,.T.);
#17951=ORIENTED_EDGE('',*,*,#12379,.T.);
#17952=ORIENTED_EDGE('',*,*,#12375,.F.);
#17953=ORIENTED_EDGE('',*,*,#12380,.F.);
#17954=ORIENTED_EDGE('',*,*,#12381,.T.);
#17955=ORIENTED_EDGE('',*,*,#12382,.T.);
#17956=ORIENTED_EDGE('',*,*,#12378,.F.);
#17957=ORIENTED_EDGE('',*,*,#12383,.F.);
#17958=ORIENTED_EDGE('',*,*,#12384,.T.);
#17959=ORIENTED_EDGE('',*,*,#12385,.T.);
#17960=ORIENTED_EDGE('',*,*,#12381,.F.);
#17961=ORIENTED_EDGE('',*,*,#12386,.F.);
#17962=ORIENTED_EDGE('',*,*,#12387,.T.);
#17963=ORIENTED_EDGE('',*,*,#12388,.T.);
#17964=ORIENTED_EDGE('',*,*,#12384,.F.);
#17965=ORIENTED_EDGE('',*,*,#12389,.F.);
#17966=ORIENTED_EDGE('',*,*,#12390,.T.);
#17967=ORIENTED_EDGE('',*,*,#12391,.T.);
#17968=ORIENTED_EDGE('',*,*,#12387,.F.);
#17969=ORIENTED_EDGE('',*,*,#12392,.F.);
#17970=ORIENTED_EDGE('',*,*,#12393,.T.);
#17971=ORIENTED_EDGE('',*,*,#12394,.T.);
#17972=ORIENTED_EDGE('',*,*,#12390,.F.);
#17973=ORIENTED_EDGE('',*,*,#12395,.F.);
#17974=ORIENTED_EDGE('',*,*,#12396,.F.);
#17975=ORIENTED_EDGE('',*,*,#12397,.F.);
#17976=ORIENTED_EDGE('',*,*,#12398,.F.);
#17977=ORIENTED_EDGE('',*,*,#12399,.T.);
#17978=ORIENTED_EDGE('',*,*,#12400,.T.);
#17979=ORIENTED_EDGE('',*,*,#12401,.T.);
#17980=ORIENTED_EDGE('',*,*,#12402,.F.);
#17981=ORIENTED_EDGE('',*,*,#12403,.F.);
#17982=ORIENTED_EDGE('',*,*,#12404,.T.);
#17983=ORIENTED_EDGE('',*,*,#12405,.T.);
#17984=ORIENTED_EDGE('',*,*,#12400,.F.);
#17985=ORIENTED_EDGE('',*,*,#12406,.F.);
#17986=ORIENTED_EDGE('',*,*,#12407,.T.);
#17987=ORIENTED_EDGE('',*,*,#12408,.T.);
#17988=ORIENTED_EDGE('',*,*,#12404,.F.);
#17989=ORIENTED_EDGE('',*,*,#12409,.F.);
#17990=ORIENTED_EDGE('',*,*,#12410,.T.);
#17991=ORIENTED_EDGE('',*,*,#12411,.T.);
#17992=ORIENTED_EDGE('',*,*,#12407,.F.);
#17993=ORIENTED_EDGE('',*,*,#12412,.F.);
#17994=ORIENTED_EDGE('',*,*,#12413,.T.);
#17995=ORIENTED_EDGE('',*,*,#12414,.T.);
#17996=ORIENTED_EDGE('',*,*,#12410,.F.);
#17997=ORIENTED_EDGE('',*,*,#12415,.F.);
#17998=ORIENTED_EDGE('',*,*,#12416,.T.);
#17999=ORIENTED_EDGE('',*,*,#12417,.T.);
#18000=ORIENTED_EDGE('',*,*,#12413,.F.);
#18001=ORIENTED_EDGE('',*,*,#12418,.F.);
#18002=ORIENTED_EDGE('',*,*,#12419,.T.);
#18003=ORIENTED_EDGE('',*,*,#12420,.T.);
#18004=ORIENTED_EDGE('',*,*,#12416,.F.);
#18005=ORIENTED_EDGE('',*,*,#12421,.F.);
#18006=ORIENTED_EDGE('',*,*,#12422,.T.);
#18007=ORIENTED_EDGE('',*,*,#12423,.T.);
#18008=ORIENTED_EDGE('',*,*,#12419,.F.);
#18009=ORIENTED_EDGE('',*,*,#12424,.F.);
#18010=ORIENTED_EDGE('',*,*,#12425,.T.);
#18011=ORIENTED_EDGE('',*,*,#12426,.T.);
#18012=ORIENTED_EDGE('',*,*,#12422,.F.);
#18013=ORIENTED_EDGE('',*,*,#12427,.F.);
#18014=ORIENTED_EDGE('',*,*,#12428,.T.);
#18015=ORIENTED_EDGE('',*,*,#12429,.T.);
#18016=ORIENTED_EDGE('',*,*,#12425,.F.);
#18017=ORIENTED_EDGE('',*,*,#12430,.F.);
#18018=ORIENTED_EDGE('',*,*,#12431,.T.);
#18019=ORIENTED_EDGE('',*,*,#12432,.T.);
#18020=ORIENTED_EDGE('',*,*,#12428,.F.);
#18021=ORIENTED_EDGE('',*,*,#12433,.F.);
#18022=ORIENTED_EDGE('',*,*,#12434,.T.);
#18023=ORIENTED_EDGE('',*,*,#12435,.T.);
#18024=ORIENTED_EDGE('',*,*,#12431,.F.);
#18025=ORIENTED_EDGE('',*,*,#12436,.F.);
#18026=ORIENTED_EDGE('',*,*,#12437,.T.);
#18027=ORIENTED_EDGE('',*,*,#12438,.T.);
#18028=ORIENTED_EDGE('',*,*,#12434,.F.);
#18029=ORIENTED_EDGE('',*,*,#12439,.F.);
#18030=ORIENTED_EDGE('',*,*,#12440,.T.);
#18031=ORIENTED_EDGE('',*,*,#12441,.T.);
#18032=ORIENTED_EDGE('',*,*,#12437,.F.);
#18033=ORIENTED_EDGE('',*,*,#12442,.F.);
#18034=ORIENTED_EDGE('',*,*,#12443,.T.);
#18035=ORIENTED_EDGE('',*,*,#12444,.T.);
#18036=ORIENTED_EDGE('',*,*,#12440,.F.);
#18037=ORIENTED_EDGE('',*,*,#12445,.F.);
#18038=ORIENTED_EDGE('',*,*,#12446,.T.);
#18039=ORIENTED_EDGE('',*,*,#12447,.T.);
#18040=ORIENTED_EDGE('',*,*,#12443,.F.);
#18041=ORIENTED_EDGE('',*,*,#12448,.F.);
#18042=ORIENTED_EDGE('',*,*,#12449,.T.);
#18043=ORIENTED_EDGE('',*,*,#12450,.T.);
#18044=ORIENTED_EDGE('',*,*,#12446,.F.);
#18045=ORIENTED_EDGE('',*,*,#12451,.F.);
#18046=ORIENTED_EDGE('',*,*,#12452,.T.);
#18047=ORIENTED_EDGE('',*,*,#12453,.T.);
#18048=ORIENTED_EDGE('',*,*,#12449,.F.);
#18049=ORIENTED_EDGE('',*,*,#12454,.F.);
#18050=ORIENTED_EDGE('',*,*,#12455,.T.);
#18051=ORIENTED_EDGE('',*,*,#12456,.T.);
#18052=ORIENTED_EDGE('',*,*,#12452,.F.);
#18053=ORIENTED_EDGE('',*,*,#12457,.F.);
#18054=ORIENTED_EDGE('',*,*,#12458,.F.);
#18055=ORIENTED_EDGE('',*,*,#12459,.F.);
#18056=ORIENTED_EDGE('',*,*,#12460,.F.);
#18057=ORIENTED_EDGE('',*,*,#12461,.T.);
#18058=ORIENTED_EDGE('',*,*,#12462,.T.);
#18059=ORIENTED_EDGE('',*,*,#12463,.T.);
#18060=ORIENTED_EDGE('',*,*,#12464,.F.);
#18061=ORIENTED_EDGE('',*,*,#12465,.F.);
#18062=ORIENTED_EDGE('',*,*,#12466,.T.);
#18063=ORIENTED_EDGE('',*,*,#12467,.T.);
#18064=ORIENTED_EDGE('',*,*,#12462,.F.);
#18065=ORIENTED_EDGE('',*,*,#12468,.F.);
#18066=ORIENTED_EDGE('',*,*,#12469,.T.);
#18067=ORIENTED_EDGE('',*,*,#12470,.T.);
#18068=ORIENTED_EDGE('',*,*,#12466,.F.);
#18069=ORIENTED_EDGE('',*,*,#12471,.F.);
#18070=ORIENTED_EDGE('',*,*,#12472,.T.);
#18071=ORIENTED_EDGE('',*,*,#12473,.T.);
#18072=ORIENTED_EDGE('',*,*,#12469,.F.);
#18073=ORIENTED_EDGE('',*,*,#12474,.F.);
#18074=ORIENTED_EDGE('',*,*,#12475,.T.);
#18075=ORIENTED_EDGE('',*,*,#12476,.T.);
#18076=ORIENTED_EDGE('',*,*,#12472,.F.);
#18077=ORIENTED_EDGE('',*,*,#12477,.F.);
#18078=ORIENTED_EDGE('',*,*,#12478,.T.);
#18079=ORIENTED_EDGE('',*,*,#12479,.T.);
#18080=ORIENTED_EDGE('',*,*,#12475,.F.);
#18081=ORIENTED_EDGE('',*,*,#12480,.F.);
#18082=ORIENTED_EDGE('',*,*,#12481,.T.);
#18083=ORIENTED_EDGE('',*,*,#12482,.T.);
#18084=ORIENTED_EDGE('',*,*,#12478,.F.);
#18085=ORIENTED_EDGE('',*,*,#12483,.F.);
#18086=ORIENTED_EDGE('',*,*,#12484,.T.);
#18087=ORIENTED_EDGE('',*,*,#12485,.T.);
#18088=ORIENTED_EDGE('',*,*,#12481,.F.);
#18089=ORIENTED_EDGE('',*,*,#12486,.F.);
#18090=ORIENTED_EDGE('',*,*,#12487,.T.);
#18091=ORIENTED_EDGE('',*,*,#12488,.T.);
#18092=ORIENTED_EDGE('',*,*,#12484,.F.);
#18093=ORIENTED_EDGE('',*,*,#12489,.F.);
#18094=ORIENTED_EDGE('',*,*,#12490,.T.);
#18095=ORIENTED_EDGE('',*,*,#12491,.T.);
#18096=ORIENTED_EDGE('',*,*,#12487,.F.);
#18097=ORIENTED_EDGE('',*,*,#12492,.F.);
#18098=ORIENTED_EDGE('',*,*,#12493,.T.);
#18099=ORIENTED_EDGE('',*,*,#12494,.T.);
#18100=ORIENTED_EDGE('',*,*,#12490,.F.);
#18101=ORIENTED_EDGE('',*,*,#12495,.F.);
#18102=ORIENTED_EDGE('',*,*,#12496,.T.);
#18103=ORIENTED_EDGE('',*,*,#12497,.T.);
#18104=ORIENTED_EDGE('',*,*,#12493,.F.);
#18105=ORIENTED_EDGE('',*,*,#12498,.F.);
#18106=ORIENTED_EDGE('',*,*,#12499,.T.);
#18107=ORIENTED_EDGE('',*,*,#12500,.T.);
#18108=ORIENTED_EDGE('',*,*,#12496,.F.);
#18109=ORIENTED_EDGE('',*,*,#12501,.F.);
#18110=ORIENTED_EDGE('',*,*,#12502,.T.);
#18111=ORIENTED_EDGE('',*,*,#12503,.T.);
#18112=ORIENTED_EDGE('',*,*,#12499,.F.);
#18113=ORIENTED_EDGE('',*,*,#12504,.F.);
#18114=ORIENTED_EDGE('',*,*,#12505,.T.);
#18115=ORIENTED_EDGE('',*,*,#12506,.T.);
#18116=ORIENTED_EDGE('',*,*,#12502,.F.);
#18117=ORIENTED_EDGE('',*,*,#12507,.F.);
#18118=ORIENTED_EDGE('',*,*,#12508,.T.);
#18119=ORIENTED_EDGE('',*,*,#12509,.T.);
#18120=ORIENTED_EDGE('',*,*,#12505,.F.);
#18121=ORIENTED_EDGE('',*,*,#12510,.F.);
#18122=ORIENTED_EDGE('',*,*,#12511,.T.);
#18123=ORIENTED_EDGE('',*,*,#12512,.T.);
#18124=ORIENTED_EDGE('',*,*,#12508,.F.);
#18125=ORIENTED_EDGE('',*,*,#12513,.F.);
#18126=ORIENTED_EDGE('',*,*,#12514,.T.);
#18127=ORIENTED_EDGE('',*,*,#12515,.T.);
#18128=ORIENTED_EDGE('',*,*,#12511,.F.);
#18129=ORIENTED_EDGE('',*,*,#12516,.F.);
#18130=ORIENTED_EDGE('',*,*,#12517,.T.);
#18131=ORIENTED_EDGE('',*,*,#12518,.T.);
#18132=ORIENTED_EDGE('',*,*,#12514,.F.);
#18133=ORIENTED_EDGE('',*,*,#12519,.F.);
#18134=ORIENTED_EDGE('',*,*,#12520,.F.);
#18135=ORIENTED_EDGE('',*,*,#12521,.F.);
#18136=ORIENTED_EDGE('',*,*,#12522,.F.);
#18137=ORIENTED_EDGE('',*,*,#12523,.T.);
#18138=ORIENTED_EDGE('',*,*,#12524,.T.);
#18139=ORIENTED_EDGE('',*,*,#12525,.T.);
#18140=ORIENTED_EDGE('',*,*,#12526,.F.);
#18141=ORIENTED_EDGE('',*,*,#12527,.F.);
#18142=ORIENTED_EDGE('',*,*,#12528,.T.);
#18143=ORIENTED_EDGE('',*,*,#12529,.T.);
#18144=ORIENTED_EDGE('',*,*,#12524,.F.);
#18145=ORIENTED_EDGE('',*,*,#12530,.F.);
#18146=ORIENTED_EDGE('',*,*,#12531,.T.);
#18147=ORIENTED_EDGE('',*,*,#12532,.T.);
#18148=ORIENTED_EDGE('',*,*,#12528,.F.);
#18149=ORIENTED_EDGE('',*,*,#12533,.F.);
#18150=ORIENTED_EDGE('',*,*,#12534,.T.);
#18151=ORIENTED_EDGE('',*,*,#12535,.T.);
#18152=ORIENTED_EDGE('',*,*,#12531,.F.);
#18153=ORIENTED_EDGE('',*,*,#12536,.F.);
#18154=ORIENTED_EDGE('',*,*,#12537,.T.);
#18155=ORIENTED_EDGE('',*,*,#12538,.T.);
#18156=ORIENTED_EDGE('',*,*,#12534,.F.);
#18157=ORIENTED_EDGE('',*,*,#12539,.F.);
#18158=ORIENTED_EDGE('',*,*,#12540,.T.);
#18159=ORIENTED_EDGE('',*,*,#12541,.T.);
#18160=ORIENTED_EDGE('',*,*,#12537,.F.);
#18161=ORIENTED_EDGE('',*,*,#12542,.F.);
#18162=ORIENTED_EDGE('',*,*,#12543,.T.);
#18163=ORIENTED_EDGE('',*,*,#12544,.T.);
#18164=ORIENTED_EDGE('',*,*,#12540,.F.);
#18165=ORIENTED_EDGE('',*,*,#12545,.F.);
#18166=ORIENTED_EDGE('',*,*,#12546,.T.);
#18167=ORIENTED_EDGE('',*,*,#12547,.T.);
#18168=ORIENTED_EDGE('',*,*,#12543,.F.);
#18169=ORIENTED_EDGE('',*,*,#12548,.F.);
#18170=ORIENTED_EDGE('',*,*,#12549,.T.);
#18171=ORIENTED_EDGE('',*,*,#12550,.T.);
#18172=ORIENTED_EDGE('',*,*,#12546,.F.);
#18173=ORIENTED_EDGE('',*,*,#12551,.F.);
#18174=ORIENTED_EDGE('',*,*,#12552,.T.);
#18175=ORIENTED_EDGE('',*,*,#12553,.T.);
#18176=ORIENTED_EDGE('',*,*,#12549,.F.);
#18177=ORIENTED_EDGE('',*,*,#12554,.F.);
#18178=ORIENTED_EDGE('',*,*,#12555,.T.);
#18179=ORIENTED_EDGE('',*,*,#12556,.T.);
#18180=ORIENTED_EDGE('',*,*,#12552,.F.);
#18181=ORIENTED_EDGE('',*,*,#12557,.F.);
#18182=ORIENTED_EDGE('',*,*,#12558,.T.);
#18183=ORIENTED_EDGE('',*,*,#12559,.T.);
#18184=ORIENTED_EDGE('',*,*,#12555,.F.);
#18185=ORIENTED_EDGE('',*,*,#12560,.F.);
#18186=ORIENTED_EDGE('',*,*,#12561,.T.);
#18187=ORIENTED_EDGE('',*,*,#12562,.T.);
#18188=ORIENTED_EDGE('',*,*,#12558,.F.);
#18189=ORIENTED_EDGE('',*,*,#12563,.F.);
#18190=ORIENTED_EDGE('',*,*,#12564,.T.);
#18191=ORIENTED_EDGE('',*,*,#12565,.T.);
#18192=ORIENTED_EDGE('',*,*,#12561,.F.);
#18193=ORIENTED_EDGE('',*,*,#12566,.F.);
#18194=ORIENTED_EDGE('',*,*,#12567,.T.);
#18195=ORIENTED_EDGE('',*,*,#12568,.T.);
#18196=ORIENTED_EDGE('',*,*,#12564,.F.);
#18197=ORIENTED_EDGE('',*,*,#12569,.F.);
#18198=ORIENTED_EDGE('',*,*,#12570,.T.);
#18199=ORIENTED_EDGE('',*,*,#12571,.T.);
#18200=ORIENTED_EDGE('',*,*,#12567,.F.);
#18201=ORIENTED_EDGE('',*,*,#12572,.F.);
#18202=ORIENTED_EDGE('',*,*,#12573,.T.);
#18203=ORIENTED_EDGE('',*,*,#12574,.T.);
#18204=ORIENTED_EDGE('',*,*,#12570,.F.);
#18205=ORIENTED_EDGE('',*,*,#12575,.F.);
#18206=ORIENTED_EDGE('',*,*,#12576,.T.);
#18207=ORIENTED_EDGE('',*,*,#12577,.T.);
#18208=ORIENTED_EDGE('',*,*,#12573,.F.);
#18209=ORIENTED_EDGE('',*,*,#12578,.F.);
#18210=ORIENTED_EDGE('',*,*,#12579,.T.);
#18211=ORIENTED_EDGE('',*,*,#12580,.T.);
#18212=ORIENTED_EDGE('',*,*,#12576,.F.);
#18213=ORIENTED_EDGE('',*,*,#12581,.F.);
#18214=ORIENTED_EDGE('',*,*,#12582,.F.);
#18215=ORIENTED_EDGE('',*,*,#12583,.F.);
#18216=ORIENTED_EDGE('',*,*,#12584,.F.);
#18217=ORIENTED_EDGE('',*,*,#12585,.T.);
#18218=ORIENTED_EDGE('',*,*,#12586,.T.);
#18219=ORIENTED_EDGE('',*,*,#12587,.T.);
#18220=ORIENTED_EDGE('',*,*,#12588,.F.);
#18221=ORIENTED_EDGE('',*,*,#12589,.F.);
#18222=ORIENTED_EDGE('',*,*,#12590,.T.);
#18223=ORIENTED_EDGE('',*,*,#12591,.T.);
#18224=ORIENTED_EDGE('',*,*,#12586,.F.);
#18225=ORIENTED_EDGE('',*,*,#12592,.F.);
#18226=ORIENTED_EDGE('',*,*,#12593,.T.);
#18227=ORIENTED_EDGE('',*,*,#12594,.T.);
#18228=ORIENTED_EDGE('',*,*,#12590,.F.);
#18229=ORIENTED_EDGE('',*,*,#12595,.F.);
#18230=ORIENTED_EDGE('',*,*,#12596,.T.);
#18231=ORIENTED_EDGE('',*,*,#12597,.T.);
#18232=ORIENTED_EDGE('',*,*,#12593,.F.);
#18233=ORIENTED_EDGE('',*,*,#12598,.F.);
#18234=ORIENTED_EDGE('',*,*,#12599,.T.);
#18235=ORIENTED_EDGE('',*,*,#12600,.T.);
#18236=ORIENTED_EDGE('',*,*,#12596,.F.);
#18237=ORIENTED_EDGE('',*,*,#12601,.F.);
#18238=ORIENTED_EDGE('',*,*,#12602,.T.);
#18239=ORIENTED_EDGE('',*,*,#12603,.T.);
#18240=ORIENTED_EDGE('',*,*,#12599,.F.);
#18241=ORIENTED_EDGE('',*,*,#12604,.F.);
#18242=ORIENTED_EDGE('',*,*,#12605,.T.);
#18243=ORIENTED_EDGE('',*,*,#12606,.T.);
#18244=ORIENTED_EDGE('',*,*,#12602,.F.);
#18245=ORIENTED_EDGE('',*,*,#12607,.F.);
#18246=ORIENTED_EDGE('',*,*,#12608,.T.);
#18247=ORIENTED_EDGE('',*,*,#12609,.T.);
#18248=ORIENTED_EDGE('',*,*,#12605,.F.);
#18249=ORIENTED_EDGE('',*,*,#12610,.F.);
#18250=ORIENTED_EDGE('',*,*,#12611,.T.);
#18251=ORIENTED_EDGE('',*,*,#12612,.T.);
#18252=ORIENTED_EDGE('',*,*,#12608,.F.);
#18253=ORIENTED_EDGE('',*,*,#12613,.F.);
#18254=ORIENTED_EDGE('',*,*,#12614,.T.);
#18255=ORIENTED_EDGE('',*,*,#12615,.T.);
#18256=ORIENTED_EDGE('',*,*,#12611,.F.);
#18257=ORIENTED_EDGE('',*,*,#12616,.F.);
#18258=ORIENTED_EDGE('',*,*,#12617,.T.);
#18259=ORIENTED_EDGE('',*,*,#12618,.T.);
#18260=ORIENTED_EDGE('',*,*,#12614,.F.);
#18261=ORIENTED_EDGE('',*,*,#12619,.F.);
#18262=ORIENTED_EDGE('',*,*,#12620,.T.);
#18263=ORIENTED_EDGE('',*,*,#12621,.T.);
#18264=ORIENTED_EDGE('',*,*,#12617,.F.);
#18265=ORIENTED_EDGE('',*,*,#12622,.F.);
#18266=ORIENTED_EDGE('',*,*,#12623,.T.);
#18267=ORIENTED_EDGE('',*,*,#12624,.T.);
#18268=ORIENTED_EDGE('',*,*,#12620,.F.);
#18269=ORIENTED_EDGE('',*,*,#12625,.F.);
#18270=ORIENTED_EDGE('',*,*,#12626,.T.);
#18271=ORIENTED_EDGE('',*,*,#12627,.T.);
#18272=ORIENTED_EDGE('',*,*,#12623,.F.);
#18273=ORIENTED_EDGE('',*,*,#12628,.F.);
#18274=ORIENTED_EDGE('',*,*,#12629,.T.);
#18275=ORIENTED_EDGE('',*,*,#12630,.T.);
#18276=ORIENTED_EDGE('',*,*,#12626,.F.);
#18277=ORIENTED_EDGE('',*,*,#12631,.F.);
#18278=ORIENTED_EDGE('',*,*,#12632,.T.);
#18279=ORIENTED_EDGE('',*,*,#12633,.T.);
#18280=ORIENTED_EDGE('',*,*,#12629,.F.);
#18281=ORIENTED_EDGE('',*,*,#12634,.F.);
#18282=ORIENTED_EDGE('',*,*,#12635,.T.);
#18283=ORIENTED_EDGE('',*,*,#12636,.T.);
#18284=ORIENTED_EDGE('',*,*,#12632,.F.);
#18285=ORIENTED_EDGE('',*,*,#12637,.F.);
#18286=ORIENTED_EDGE('',*,*,#12638,.T.);
#18287=ORIENTED_EDGE('',*,*,#12639,.T.);
#18288=ORIENTED_EDGE('',*,*,#12635,.F.);
#18289=ORIENTED_EDGE('',*,*,#12640,.F.);
#18290=ORIENTED_EDGE('',*,*,#12641,.T.);
#18291=ORIENTED_EDGE('',*,*,#12642,.T.);
#18292=ORIENTED_EDGE('',*,*,#12638,.F.);
#18293=ORIENTED_EDGE('',*,*,#12643,.F.);
#18294=ORIENTED_EDGE('',*,*,#12644,.F.);
#18295=ORIENTED_EDGE('',*,*,#12645,.F.);
#18296=ORIENTED_EDGE('',*,*,#12646,.F.);
#18297=ORIENTED_EDGE('',*,*,#12647,.T.);
#18298=ORIENTED_EDGE('',*,*,#12648,.T.);
#18299=ORIENTED_EDGE('',*,*,#12649,.T.);
#18300=ORIENTED_EDGE('',*,*,#12650,.F.);
#18301=ORIENTED_EDGE('',*,*,#12651,.F.);
#18302=ORIENTED_EDGE('',*,*,#12652,.T.);
#18303=ORIENTED_EDGE('',*,*,#12653,.T.);
#18304=ORIENTED_EDGE('',*,*,#12648,.F.);
#18305=ORIENTED_EDGE('',*,*,#12654,.F.);
#18306=ORIENTED_EDGE('',*,*,#12655,.T.);
#18307=ORIENTED_EDGE('',*,*,#12656,.T.);
#18308=ORIENTED_EDGE('',*,*,#12652,.F.);
#18309=ORIENTED_EDGE('',*,*,#12657,.F.);
#18310=ORIENTED_EDGE('',*,*,#12658,.T.);
#18311=ORIENTED_EDGE('',*,*,#12659,.T.);
#18312=ORIENTED_EDGE('',*,*,#12655,.F.);
#18313=ORIENTED_EDGE('',*,*,#12660,.F.);
#18314=ORIENTED_EDGE('',*,*,#12661,.T.);
#18315=ORIENTED_EDGE('',*,*,#12662,.T.);
#18316=ORIENTED_EDGE('',*,*,#12658,.F.);
#18317=ORIENTED_EDGE('',*,*,#12663,.F.);
#18318=ORIENTED_EDGE('',*,*,#12664,.T.);
#18319=ORIENTED_EDGE('',*,*,#12665,.T.);
#18320=ORIENTED_EDGE('',*,*,#12661,.F.);
#18321=ORIENTED_EDGE('',*,*,#12666,.F.);
#18322=ORIENTED_EDGE('',*,*,#12667,.T.);
#18323=ORIENTED_EDGE('',*,*,#12668,.T.);
#18324=ORIENTED_EDGE('',*,*,#12664,.F.);
#18325=ORIENTED_EDGE('',*,*,#12669,.F.);
#18326=ORIENTED_EDGE('',*,*,#12670,.T.);
#18327=ORIENTED_EDGE('',*,*,#12671,.T.);
#18328=ORIENTED_EDGE('',*,*,#12667,.F.);
#18329=ORIENTED_EDGE('',*,*,#12672,.F.);
#18330=ORIENTED_EDGE('',*,*,#12673,.T.);
#18331=ORIENTED_EDGE('',*,*,#12674,.T.);
#18332=ORIENTED_EDGE('',*,*,#12670,.F.);
#18333=ORIENTED_EDGE('',*,*,#12675,.F.);
#18334=ORIENTED_EDGE('',*,*,#12676,.T.);
#18335=ORIENTED_EDGE('',*,*,#12677,.T.);
#18336=ORIENTED_EDGE('',*,*,#12673,.F.);
#18337=ORIENTED_EDGE('',*,*,#12678,.F.);
#18338=ORIENTED_EDGE('',*,*,#12679,.T.);
#18339=ORIENTED_EDGE('',*,*,#12680,.T.);
#18340=ORIENTED_EDGE('',*,*,#12676,.F.);
#18341=ORIENTED_EDGE('',*,*,#12681,.F.);
#18342=ORIENTED_EDGE('',*,*,#12682,.T.);
#18343=ORIENTED_EDGE('',*,*,#12683,.T.);
#18344=ORIENTED_EDGE('',*,*,#12679,.F.);
#18345=ORIENTED_EDGE('',*,*,#12684,.F.);
#18346=ORIENTED_EDGE('',*,*,#12685,.T.);
#18347=ORIENTED_EDGE('',*,*,#12686,.T.);
#18348=ORIENTED_EDGE('',*,*,#12682,.F.);
#18349=ORIENTED_EDGE('',*,*,#12687,.F.);
#18350=ORIENTED_EDGE('',*,*,#12688,.T.);
#18351=ORIENTED_EDGE('',*,*,#12689,.T.);
#18352=ORIENTED_EDGE('',*,*,#12685,.F.);
#18353=ORIENTED_EDGE('',*,*,#12690,.F.);
#18354=ORIENTED_EDGE('',*,*,#12691,.T.);
#18355=ORIENTED_EDGE('',*,*,#12692,.T.);
#18356=ORIENTED_EDGE('',*,*,#12688,.F.);
#18357=ORIENTED_EDGE('',*,*,#12693,.F.);
#18358=ORIENTED_EDGE('',*,*,#12694,.T.);
#18359=ORIENTED_EDGE('',*,*,#12695,.T.);
#18360=ORIENTED_EDGE('',*,*,#12691,.F.);
#18361=ORIENTED_EDGE('',*,*,#12696,.F.);
#18362=ORIENTED_EDGE('',*,*,#12697,.T.);
#18363=ORIENTED_EDGE('',*,*,#12698,.T.);
#18364=ORIENTED_EDGE('',*,*,#12694,.F.);
#18365=ORIENTED_EDGE('',*,*,#12699,.F.);
#18366=ORIENTED_EDGE('',*,*,#12700,.T.);
#18367=ORIENTED_EDGE('',*,*,#12701,.T.);
#18368=ORIENTED_EDGE('',*,*,#12697,.F.);
#18369=ORIENTED_EDGE('',*,*,#12702,.F.);
#18370=ORIENTED_EDGE('',*,*,#12703,.T.);
#18371=ORIENTED_EDGE('',*,*,#12704,.T.);
#18372=ORIENTED_EDGE('',*,*,#12700,.F.);
#18373=ORIENTED_EDGE('',*,*,#12705,.F.);
#18374=ORIENTED_EDGE('',*,*,#12706,.F.);
#18375=ORIENTED_EDGE('',*,*,#12707,.F.);
#18376=ORIENTED_EDGE('',*,*,#12708,.F.);
#18377=ORIENTED_EDGE('',*,*,#12709,.T.);
#18378=ORIENTED_EDGE('',*,*,#12706,.T.);
#18379=ORIENTED_EDGE('',*,*,#12710,.T.);
#18380=ORIENTED_EDGE('',*,*,#12703,.F.);
#18381=ORIENTED_EDGE('',*,*,#12711,.F.);
#18382=ORIENTED_EDGE('',*,*,#12712,.F.);
#18383=ORIENTED_EDGE('',*,*,#12649,.F.);
#18384=ORIENTED_EDGE('',*,*,#12653,.F.);
#18385=ORIENTED_EDGE('',*,*,#12656,.F.);
#18386=ORIENTED_EDGE('',*,*,#12659,.F.);
#18387=ORIENTED_EDGE('',*,*,#12662,.F.);
#18388=ORIENTED_EDGE('',*,*,#12665,.F.);
#18389=ORIENTED_EDGE('',*,*,#12668,.F.);
#18390=ORIENTED_EDGE('',*,*,#12671,.F.);
#18391=ORIENTED_EDGE('',*,*,#12674,.F.);
#18392=ORIENTED_EDGE('',*,*,#12677,.F.);
#18393=ORIENTED_EDGE('',*,*,#12680,.F.);
#18394=ORIENTED_EDGE('',*,*,#12683,.F.);
#18395=ORIENTED_EDGE('',*,*,#12686,.F.);
#18396=ORIENTED_EDGE('',*,*,#12689,.F.);
#18397=ORIENTED_EDGE('',*,*,#12692,.F.);
#18398=ORIENTED_EDGE('',*,*,#12695,.F.);
#18399=ORIENTED_EDGE('',*,*,#12698,.F.);
#18400=ORIENTED_EDGE('',*,*,#12701,.F.);
#18401=ORIENTED_EDGE('',*,*,#12704,.F.);
#18402=ORIENTED_EDGE('',*,*,#12710,.F.);
#18403=ORIENTED_EDGE('',*,*,#12709,.F.);
#18404=ORIENTED_EDGE('',*,*,#12713,.F.);
#18405=ORIENTED_EDGE('',*,*,#12149,.F.);
#18406=ORIENTED_EDGE('',*,*,#12714,.F.);
#18407=ORIENTED_EDGE('',*,*,#12147,.F.);
#18408=ORIENTED_EDGE('',*,*,#12144,.F.);
#18409=ORIENTED_EDGE('',*,*,#12141,.F.);
#18410=ORIENTED_EDGE('',*,*,#12138,.F.);
#18411=ORIENTED_EDGE('',*,*,#12135,.F.);
#18412=ORIENTED_EDGE('',*,*,#12132,.F.);
#18413=ORIENTED_EDGE('',*,*,#12129,.F.);
#18414=ORIENTED_EDGE('',*,*,#12126,.F.);
#18415=ORIENTED_EDGE('',*,*,#12123,.F.);
#18416=ORIENTED_EDGE('',*,*,#12120,.F.);
#18417=ORIENTED_EDGE('',*,*,#12117,.F.);
#18418=ORIENTED_EDGE('',*,*,#12114,.F.);
#18419=ORIENTED_EDGE('',*,*,#12111,.F.);
#18420=ORIENTED_EDGE('',*,*,#12108,.F.);
#18421=ORIENTED_EDGE('',*,*,#12105,.F.);
#18422=ORIENTED_EDGE('',*,*,#12102,.F.);
#18423=ORIENTED_EDGE('',*,*,#12099,.F.);
#18424=ORIENTED_EDGE('',*,*,#12096,.F.);
#18425=ORIENTED_EDGE('',*,*,#12093,.F.);
#18426=ORIENTED_EDGE('',*,*,#12715,.F.);
#18427=ORIENTED_EDGE('',*,*,#12091,.F.);
#18428=ORIENTED_EDGE('',*,*,#12095,.F.);
#18429=ORIENTED_EDGE('',*,*,#12098,.F.);
#18430=ORIENTED_EDGE('',*,*,#12101,.F.);
#18431=ORIENTED_EDGE('',*,*,#12104,.F.);
#18432=ORIENTED_EDGE('',*,*,#12107,.F.);
#18433=ORIENTED_EDGE('',*,*,#12110,.F.);
#18434=ORIENTED_EDGE('',*,*,#12113,.F.);
#18435=ORIENTED_EDGE('',*,*,#12116,.F.);
#18436=ORIENTED_EDGE('',*,*,#12119,.F.);
#18437=ORIENTED_EDGE('',*,*,#12122,.F.);
#18438=ORIENTED_EDGE('',*,*,#12125,.F.);
#18439=ORIENTED_EDGE('',*,*,#12128,.F.);
#18440=ORIENTED_EDGE('',*,*,#12131,.F.);
#18441=ORIENTED_EDGE('',*,*,#12134,.F.);
#18442=ORIENTED_EDGE('',*,*,#12137,.F.);
#18443=ORIENTED_EDGE('',*,*,#12140,.F.);
#18444=ORIENTED_EDGE('',*,*,#12143,.F.);
#18445=ORIENTED_EDGE('',*,*,#12146,.F.);
#18446=ORIENTED_EDGE('',*,*,#12716,.F.);
#18447=ORIENTED_EDGE('',*,*,#12151,.F.);
#18448=ORIENTED_EDGE('',*,*,#12717,.F.);
#18449=ORIENTED_EDGE('',*,*,#12707,.T.);
#18450=ORIENTED_EDGE('',*,*,#12711,.T.);
#18451=ORIENTED_EDGE('',*,*,#12705,.T.);
#18452=ORIENTED_EDGE('',*,*,#12702,.T.);
#18453=ORIENTED_EDGE('',*,*,#12699,.T.);
#18454=ORIENTED_EDGE('',*,*,#12696,.T.);
#18455=ORIENTED_EDGE('',*,*,#12693,.T.);
#18456=ORIENTED_EDGE('',*,*,#12690,.T.);
#18457=ORIENTED_EDGE('',*,*,#12687,.T.);
#18458=ORIENTED_EDGE('',*,*,#12684,.T.);
#18459=ORIENTED_EDGE('',*,*,#12681,.T.);
#18460=ORIENTED_EDGE('',*,*,#12678,.T.);
#18461=ORIENTED_EDGE('',*,*,#12675,.T.);
#18462=ORIENTED_EDGE('',*,*,#12672,.T.);
#18463=ORIENTED_EDGE('',*,*,#12669,.T.);
#18464=ORIENTED_EDGE('',*,*,#12666,.T.);
#18465=ORIENTED_EDGE('',*,*,#12663,.T.);
#18466=ORIENTED_EDGE('',*,*,#12660,.T.);
#18467=ORIENTED_EDGE('',*,*,#12657,.T.);
#18468=ORIENTED_EDGE('',*,*,#12654,.T.);
#18469=ORIENTED_EDGE('',*,*,#12651,.T.);
#18470=ORIENTED_EDGE('',*,*,#12718,.T.);
#18471=ORIENTED_EDGE('',*,*,#12719,.T.);
#18472=ORIENTED_EDGE('',*,*,#12720,.T.);
#18473=ORIENTED_EDGE('',*,*,#12721,.T.);
#18474=ORIENTED_EDGE('',*,*,#12722,.T.);
#18475=ORIENTED_EDGE('',*,*,#12460,.T.);
#18476=ORIENTED_EDGE('',*,*,#12723,.T.);
#18477=ORIENTED_EDGE('',*,*,#12026,.T.);
#18478=ORIENTED_EDGE('',*,*,#12724,.T.);
#18479=ORIENTED_EDGE('',*,*,#12522,.T.);
#18480=ORIENTED_EDGE('',*,*,#12725,.T.);
#18481=ORIENTED_EDGE('',*,*,#12088,.T.);
#18482=ORIENTED_EDGE('',*,*,#12713,.T.);
#18483=ORIENTED_EDGE('',*,*,#12708,.T.);
#18484=ORIENTED_EDGE('',*,*,#12717,.T.);
#18485=ORIENTED_EDGE('',*,*,#12150,.T.);
#18486=ORIENTED_EDGE('',*,*,#12726,.T.);
#18487=ORIENTED_EDGE('',*,*,#12584,.T.);
#18488=ORIENTED_EDGE('',*,*,#12727,.T.);
#18489=ORIENTED_EDGE('',*,*,#12212,.T.);
#18490=ORIENTED_EDGE('',*,*,#12728,.T.);
#18491=ORIENTED_EDGE('',*,*,#12646,.T.);
#18492=ORIENTED_EDGE('',*,*,#12729,.T.);
#18493=ORIENTED_EDGE('',*,*,#12274,.T.);
#18494=ORIENTED_EDGE('',*,*,#12730,.T.);
#18495=ORIENTED_EDGE('',*,*,#12398,.T.);
#18496=ORIENTED_EDGE('',*,*,#12731,.T.);
#18497=ORIENTED_EDGE('',*,*,#12336,.T.);
#18498=ORIENTED_EDGE('',*,*,#12644,.T.);
#18499=ORIENTED_EDGE('',*,*,#12732,.T.);
#18500=ORIENTED_EDGE('',*,*,#12641,.F.);
#18501=ORIENTED_EDGE('',*,*,#12733,.F.);
#18502=ORIENTED_EDGE('',*,*,#12734,.F.);
#18503=ORIENTED_EDGE('',*,*,#12587,.F.);
#18504=ORIENTED_EDGE('',*,*,#12591,.F.);
#18505=ORIENTED_EDGE('',*,*,#12594,.F.);
#18506=ORIENTED_EDGE('',*,*,#12597,.F.);
#18507=ORIENTED_EDGE('',*,*,#12600,.F.);
#18508=ORIENTED_EDGE('',*,*,#12603,.F.);
#18509=ORIENTED_EDGE('',*,*,#12606,.F.);
#18510=ORIENTED_EDGE('',*,*,#12609,.F.);
#18511=ORIENTED_EDGE('',*,*,#12612,.F.);
#18512=ORIENTED_EDGE('',*,*,#12615,.F.);
#18513=ORIENTED_EDGE('',*,*,#12618,.F.);
#18514=ORIENTED_EDGE('',*,*,#12621,.F.);
#18515=ORIENTED_EDGE('',*,*,#12624,.F.);
#18516=ORIENTED_EDGE('',*,*,#12627,.F.);
#18517=ORIENTED_EDGE('',*,*,#12630,.F.);
#18518=ORIENTED_EDGE('',*,*,#12633,.F.);
#18519=ORIENTED_EDGE('',*,*,#12636,.F.);
#18520=ORIENTED_EDGE('',*,*,#12639,.F.);
#18521=ORIENTED_EDGE('',*,*,#12642,.F.);
#18522=ORIENTED_EDGE('',*,*,#12732,.F.);
#18523=ORIENTED_EDGE('',*,*,#12647,.F.);
#18524=ORIENTED_EDGE('',*,*,#12728,.F.);
#18525=ORIENTED_EDGE('',*,*,#12273,.F.);
#18526=ORIENTED_EDGE('',*,*,#12735,.F.);
#18527=ORIENTED_EDGE('',*,*,#12271,.F.);
#18528=ORIENTED_EDGE('',*,*,#12268,.F.);
#18529=ORIENTED_EDGE('',*,*,#12265,.F.);
#18530=ORIENTED_EDGE('',*,*,#12262,.F.);
#18531=ORIENTED_EDGE('',*,*,#12259,.F.);
#18532=ORIENTED_EDGE('',*,*,#12256,.F.);
#18533=ORIENTED_EDGE('',*,*,#12253,.F.);
#18534=ORIENTED_EDGE('',*,*,#12250,.F.);
#18535=ORIENTED_EDGE('',*,*,#12247,.F.);
#18536=ORIENTED_EDGE('',*,*,#12244,.F.);
#18537=ORIENTED_EDGE('',*,*,#12241,.F.);
#18538=ORIENTED_EDGE('',*,*,#12238,.F.);
#18539=ORIENTED_EDGE('',*,*,#12235,.F.);
#18540=ORIENTED_EDGE('',*,*,#12232,.F.);
#18541=ORIENTED_EDGE('',*,*,#12229,.F.);
#18542=ORIENTED_EDGE('',*,*,#12226,.F.);
#18543=ORIENTED_EDGE('',*,*,#12223,.F.);
#18544=ORIENTED_EDGE('',*,*,#12220,.F.);
#18545=ORIENTED_EDGE('',*,*,#12217,.F.);
#18546=ORIENTED_EDGE('',*,*,#12736,.F.);
#18547=ORIENTED_EDGE('',*,*,#12215,.F.);
#18548=ORIENTED_EDGE('',*,*,#12219,.F.);
#18549=ORIENTED_EDGE('',*,*,#12222,.F.);
#18550=ORIENTED_EDGE('',*,*,#12225,.F.);
#18551=ORIENTED_EDGE('',*,*,#12228,.F.);
#18552=ORIENTED_EDGE('',*,*,#12231,.F.);
#18553=ORIENTED_EDGE('',*,*,#12234,.F.);
#18554=ORIENTED_EDGE('',*,*,#12237,.F.);
#18555=ORIENTED_EDGE('',*,*,#12240,.F.);
#18556=ORIENTED_EDGE('',*,*,#12243,.F.);
#18557=ORIENTED_EDGE('',*,*,#12246,.F.);
#18558=ORIENTED_EDGE('',*,*,#12249,.F.);
#18559=ORIENTED_EDGE('',*,*,#12252,.F.);
#18560=ORIENTED_EDGE('',*,*,#12255,.F.);
#18561=ORIENTED_EDGE('',*,*,#12258,.F.);
#18562=ORIENTED_EDGE('',*,*,#12261,.F.);
#18563=ORIENTED_EDGE('',*,*,#12264,.F.);
#18564=ORIENTED_EDGE('',*,*,#12267,.F.);
#18565=ORIENTED_EDGE('',*,*,#12270,.F.);
#18566=ORIENTED_EDGE('',*,*,#12737,.F.);
#18567=ORIENTED_EDGE('',*,*,#12275,.F.);
#18568=ORIENTED_EDGE('',*,*,#12729,.F.);
#18569=ORIENTED_EDGE('',*,*,#12645,.T.);
#18570=ORIENTED_EDGE('',*,*,#12733,.T.);
#18571=ORIENTED_EDGE('',*,*,#12643,.T.);
#18572=ORIENTED_EDGE('',*,*,#12640,.T.);
#18573=ORIENTED_EDGE('',*,*,#12637,.T.);
#18574=ORIENTED_EDGE('',*,*,#12634,.T.);
#18575=ORIENTED_EDGE('',*,*,#12631,.T.);
#18576=ORIENTED_EDGE('',*,*,#12628,.T.);
#18577=ORIENTED_EDGE('',*,*,#12625,.T.);
#18578=ORIENTED_EDGE('',*,*,#12622,.T.);
#18579=ORIENTED_EDGE('',*,*,#12619,.T.);
#18580=ORIENTED_EDGE('',*,*,#12616,.T.);
#18581=ORIENTED_EDGE('',*,*,#12613,.T.);
#18582=ORIENTED_EDGE('',*,*,#12610,.T.);
#18583=ORIENTED_EDGE('',*,*,#12607,.T.);
#18584=ORIENTED_EDGE('',*,*,#12604,.T.);
#18585=ORIENTED_EDGE('',*,*,#12601,.T.);
#18586=ORIENTED_EDGE('',*,*,#12598,.T.);
#18587=ORIENTED_EDGE('',*,*,#12595,.T.);
#18588=ORIENTED_EDGE('',*,*,#12592,.T.);
#18589=ORIENTED_EDGE('',*,*,#12589,.T.);
#18590=ORIENTED_EDGE('',*,*,#12582,.T.);
#18591=ORIENTED_EDGE('',*,*,#12738,.T.);
#18592=ORIENTED_EDGE('',*,*,#12579,.F.);
#18593=ORIENTED_EDGE('',*,*,#12739,.F.);
#18594=ORIENTED_EDGE('',*,*,#12740,.F.);
#18595=ORIENTED_EDGE('',*,*,#12525,.F.);
#18596=ORIENTED_EDGE('',*,*,#12529,.F.);
#18597=ORIENTED_EDGE('',*,*,#12532,.F.);
#18598=ORIENTED_EDGE('',*,*,#12535,.F.);
#18599=ORIENTED_EDGE('',*,*,#12538,.F.);
#18600=ORIENTED_EDGE('',*,*,#12541,.F.);
#18601=ORIENTED_EDGE('',*,*,#12544,.F.);
#18602=ORIENTED_EDGE('',*,*,#12547,.F.);
#18603=ORIENTED_EDGE('',*,*,#12550,.F.);
#18604=ORIENTED_EDGE('',*,*,#12553,.F.);
#18605=ORIENTED_EDGE('',*,*,#12556,.F.);
#18606=ORIENTED_EDGE('',*,*,#12559,.F.);
#18607=ORIENTED_EDGE('',*,*,#12562,.F.);
#18608=ORIENTED_EDGE('',*,*,#12565,.F.);
#18609=ORIENTED_EDGE('',*,*,#12568,.F.);
#18610=ORIENTED_EDGE('',*,*,#12571,.F.);
#18611=ORIENTED_EDGE('',*,*,#12574,.F.);
#18612=ORIENTED_EDGE('',*,*,#12577,.F.);
#18613=ORIENTED_EDGE('',*,*,#12580,.F.);
#18614=ORIENTED_EDGE('',*,*,#12738,.F.);
#18615=ORIENTED_EDGE('',*,*,#12585,.F.);
#18616=ORIENTED_EDGE('',*,*,#12726,.F.);
#18617=ORIENTED_EDGE('',*,*,#12211,.F.);
#18618=ORIENTED_EDGE('',*,*,#12741,.F.);
#18619=ORIENTED_EDGE('',*,*,#12209,.F.);
#18620=ORIENTED_EDGE('',*,*,#12206,.F.);
#18621=ORIENTED_EDGE('',*,*,#12203,.F.);
#18622=ORIENTED_EDGE('',*,*,#12200,.F.);
#18623=ORIENTED_EDGE('',*,*,#12197,.F.);
#18624=ORIENTED_EDGE('',*,*,#12194,.F.);
#18625=ORIENTED_EDGE('',*,*,#12191,.F.);
#18626=ORIENTED_EDGE('',*,*,#12188,.F.);
#18627=ORIENTED_EDGE('',*,*,#12185,.F.);
#18628=ORIENTED_EDGE('',*,*,#12182,.F.);
#18629=ORIENTED_EDGE('',*,*,#12179,.F.);
#18630=ORIENTED_EDGE('',*,*,#12176,.F.);
#18631=ORIENTED_EDGE('',*,*,#12173,.F.);
#18632=ORIENTED_EDGE('',*,*,#12170,.F.);
#18633=ORIENTED_EDGE('',*,*,#12167,.F.);
#18634=ORIENTED_EDGE('',*,*,#12164,.F.);
#18635=ORIENTED_EDGE('',*,*,#12161,.F.);
#18636=ORIENTED_EDGE('',*,*,#12158,.F.);
#18637=ORIENTED_EDGE('',*,*,#12155,.F.);
#18638=ORIENTED_EDGE('',*,*,#12742,.F.);
#18639=ORIENTED_EDGE('',*,*,#12153,.F.);
#18640=ORIENTED_EDGE('',*,*,#12157,.F.);
#18641=ORIENTED_EDGE('',*,*,#12160,.F.);
#18642=ORIENTED_EDGE('',*,*,#12163,.F.);
#18643=ORIENTED_EDGE('',*,*,#12166,.F.);
#18644=ORIENTED_EDGE('',*,*,#12169,.F.);
#18645=ORIENTED_EDGE('',*,*,#12172,.F.);
#18646=ORIENTED_EDGE('',*,*,#12175,.F.);
#18647=ORIENTED_EDGE('',*,*,#12178,.F.);
#18648=ORIENTED_EDGE('',*,*,#12181,.F.);
#18649=ORIENTED_EDGE('',*,*,#12184,.F.);
#18650=ORIENTED_EDGE('',*,*,#12187,.F.);
#18651=ORIENTED_EDGE('',*,*,#12190,.F.);
#18652=ORIENTED_EDGE('',*,*,#12193,.F.);
#18653=ORIENTED_EDGE('',*,*,#12196,.F.);
#18654=ORIENTED_EDGE('',*,*,#12199,.F.);
#18655=ORIENTED_EDGE('',*,*,#12202,.F.);
#18656=ORIENTED_EDGE('',*,*,#12205,.F.);
#18657=ORIENTED_EDGE('',*,*,#12208,.F.);
#18658=ORIENTED_EDGE('',*,*,#12743,.F.);
#18659=ORIENTED_EDGE('',*,*,#12213,.F.);
#18660=ORIENTED_EDGE('',*,*,#12727,.F.);
#18661=ORIENTED_EDGE('',*,*,#12583,.T.);
#18662=ORIENTED_EDGE('',*,*,#12739,.T.);
#18663=ORIENTED_EDGE('',*,*,#12581,.T.);
#18664=ORIENTED_EDGE('',*,*,#12578,.T.);
#18665=ORIENTED_EDGE('',*,*,#12575,.T.);
#18666=ORIENTED_EDGE('',*,*,#12572,.T.);
#18667=ORIENTED_EDGE('',*,*,#12569,.T.);
#18668=ORIENTED_EDGE('',*,*,#12566,.T.);
#18669=ORIENTED_EDGE('',*,*,#12563,.T.);
#18670=ORIENTED_EDGE('',*,*,#12560,.T.);
#18671=ORIENTED_EDGE('',*,*,#12557,.T.);
#18672=ORIENTED_EDGE('',*,*,#12554,.T.);
#18673=ORIENTED_EDGE('',*,*,#12551,.T.);
#18674=ORIENTED_EDGE('',*,*,#12548,.T.);
#18675=ORIENTED_EDGE('',*,*,#12545,.T.);
#18676=ORIENTED_EDGE('',*,*,#12542,.T.);
#18677=ORIENTED_EDGE('',*,*,#12539,.T.);
#18678=ORIENTED_EDGE('',*,*,#12536,.T.);
#18679=ORIENTED_EDGE('',*,*,#12533,.T.);
#18680=ORIENTED_EDGE('',*,*,#12530,.T.);
#18681=ORIENTED_EDGE('',*,*,#12527,.T.);
#18682=ORIENTED_EDGE('',*,*,#12520,.T.);
#18683=ORIENTED_EDGE('',*,*,#12744,.T.);
#18684=ORIENTED_EDGE('',*,*,#12517,.F.);
#18685=ORIENTED_EDGE('',*,*,#12745,.F.);
#18686=ORIENTED_EDGE('',*,*,#12746,.F.);
#18687=ORIENTED_EDGE('',*,*,#12463,.F.);
#18688=ORIENTED_EDGE('',*,*,#12467,.F.);
#18689=ORIENTED_EDGE('',*,*,#12470,.F.);
#18690=ORIENTED_EDGE('',*,*,#12473,.F.);
#18691=ORIENTED_EDGE('',*,*,#12476,.F.);
#18692=ORIENTED_EDGE('',*,*,#12479,.F.);
#18693=ORIENTED_EDGE('',*,*,#12482,.F.);
#18694=ORIENTED_EDGE('',*,*,#12485,.F.);
#18695=ORIENTED_EDGE('',*,*,#12488,.F.);
#18696=ORIENTED_EDGE('',*,*,#12491,.F.);
#18697=ORIENTED_EDGE('',*,*,#12494,.F.);
#18698=ORIENTED_EDGE('',*,*,#12497,.F.);
#18699=ORIENTED_EDGE('',*,*,#12500,.F.);
#18700=ORIENTED_EDGE('',*,*,#12503,.F.);
#18701=ORIENTED_EDGE('',*,*,#12506,.F.);
#18702=ORIENTED_EDGE('',*,*,#12509,.F.);
#18703=ORIENTED_EDGE('',*,*,#12512,.F.);
#18704=ORIENTED_EDGE('',*,*,#12515,.F.);
#18705=ORIENTED_EDGE('',*,*,#12518,.F.);
#18706=ORIENTED_EDGE('',*,*,#12744,.F.);
#18707=ORIENTED_EDGE('',*,*,#12523,.F.);
#18708=ORIENTED_EDGE('',*,*,#12724,.F.);
#18709=ORIENTED_EDGE('',*,*,#12087,.F.);
#18710=ORIENTED_EDGE('',*,*,#12747,.F.);
#18711=ORIENTED_EDGE('',*,*,#12085,.F.);
#18712=ORIENTED_EDGE('',*,*,#12082,.F.);
#18713=ORIENTED_EDGE('',*,*,#12079,.F.);
#18714=ORIENTED_EDGE('',*,*,#12076,.F.);
#18715=ORIENTED_EDGE('',*,*,#12073,.F.);
#18716=ORIENTED_EDGE('',*,*,#12070,.F.);
#18717=ORIENTED_EDGE('',*,*,#12067,.F.);
#18718=ORIENTED_EDGE('',*,*,#12064,.F.);
#18719=ORIENTED_EDGE('',*,*,#12061,.F.);
#18720=ORIENTED_EDGE('',*,*,#12058,.F.);
#18721=ORIENTED_EDGE('',*,*,#12055,.F.);
#18722=ORIENTED_EDGE('',*,*,#12052,.F.);
#18723=ORIENTED_EDGE('',*,*,#12049,.F.);
#18724=ORIENTED_EDGE('',*,*,#12046,.F.);
#18725=ORIENTED_EDGE('',*,*,#12043,.F.);
#18726=ORIENTED_EDGE('',*,*,#12040,.F.);
#18727=ORIENTED_EDGE('',*,*,#12037,.F.);
#18728=ORIENTED_EDGE('',*,*,#12034,.F.);
#18729=ORIENTED_EDGE('',*,*,#12031,.F.);
#18730=ORIENTED_EDGE('',*,*,#12748,.F.);
#18731=ORIENTED_EDGE('',*,*,#12029,.F.);
#18732=ORIENTED_EDGE('',*,*,#12033,.F.);
#18733=ORIENTED_EDGE('',*,*,#12036,.F.);
#18734=ORIENTED_EDGE('',*,*,#12039,.F.);
#18735=ORIENTED_EDGE('',*,*,#12042,.F.);
#18736=ORIENTED_EDGE('',*,*,#12045,.F.);
#18737=ORIENTED_EDGE('',*,*,#12048,.F.);
#18738=ORIENTED_EDGE('',*,*,#12051,.F.);
#18739=ORIENTED_EDGE('',*,*,#12054,.F.);
#18740=ORIENTED_EDGE('',*,*,#12057,.F.);
#18741=ORIENTED_EDGE('',*,*,#12060,.F.);
#18742=ORIENTED_EDGE('',*,*,#12063,.F.);
#18743=ORIENTED_EDGE('',*,*,#12066,.F.);
#18744=ORIENTED_EDGE('',*,*,#12069,.F.);
#18745=ORIENTED_EDGE('',*,*,#12072,.F.);
#18746=ORIENTED_EDGE('',*,*,#12075,.F.);
#18747=ORIENTED_EDGE('',*,*,#12078,.F.);
#18748=ORIENTED_EDGE('',*,*,#12081,.F.);
#18749=ORIENTED_EDGE('',*,*,#12084,.F.);
#18750=ORIENTED_EDGE('',*,*,#12749,.F.);
#18751=ORIENTED_EDGE('',*,*,#12089,.F.);
#18752=ORIENTED_EDGE('',*,*,#12725,.F.);
#18753=ORIENTED_EDGE('',*,*,#12521,.T.);
#18754=ORIENTED_EDGE('',*,*,#12745,.T.);
#18755=ORIENTED_EDGE('',*,*,#12519,.T.);
#18756=ORIENTED_EDGE('',*,*,#12516,.T.);
#18757=ORIENTED_EDGE('',*,*,#12513,.T.);
#18758=ORIENTED_EDGE('',*,*,#12510,.T.);
#18759=ORIENTED_EDGE('',*,*,#12507,.T.);
#18760=ORIENTED_EDGE('',*,*,#12504,.T.);
#18761=ORIENTED_EDGE('',*,*,#12501,.T.);
#18762=ORIENTED_EDGE('',*,*,#12498,.T.);
#18763=ORIENTED_EDGE('',*,*,#12495,.T.);
#18764=ORIENTED_EDGE('',*,*,#12492,.T.);
#18765=ORIENTED_EDGE('',*,*,#12489,.T.);
#18766=ORIENTED_EDGE('',*,*,#12486,.T.);
#18767=ORIENTED_EDGE('',*,*,#12483,.T.);
#18768=ORIENTED_EDGE('',*,*,#12480,.T.);
#18769=ORIENTED_EDGE('',*,*,#12477,.T.);
#18770=ORIENTED_EDGE('',*,*,#12474,.T.);
#18771=ORIENTED_EDGE('',*,*,#12471,.T.);
#18772=ORIENTED_EDGE('',*,*,#12468,.T.);
#18773=ORIENTED_EDGE('',*,*,#12465,.T.);
#18774=ORIENTED_EDGE('',*,*,#12458,.T.);
#18775=ORIENTED_EDGE('',*,*,#12750,.T.);
#18776=ORIENTED_EDGE('',*,*,#12455,.F.);
#18777=ORIENTED_EDGE('',*,*,#12751,.F.);
#18778=ORIENTED_EDGE('',*,*,#12752,.F.);
#18779=ORIENTED_EDGE('',*,*,#12401,.F.);
#18780=ORIENTED_EDGE('',*,*,#12405,.F.);
#18781=ORIENTED_EDGE('',*,*,#12408,.F.);
#18782=ORIENTED_EDGE('',*,*,#12411,.F.);
#18783=ORIENTED_EDGE('',*,*,#12414,.F.);
#18784=ORIENTED_EDGE('',*,*,#12417,.F.);
#18785=ORIENTED_EDGE('',*,*,#12420,.F.);
#18786=ORIENTED_EDGE('',*,*,#12423,.F.);
#18787=ORIENTED_EDGE('',*,*,#12426,.F.);
#18788=ORIENTED_EDGE('',*,*,#12429,.F.);
#18789=ORIENTED_EDGE('',*,*,#12432,.F.);
#18790=ORIENTED_EDGE('',*,*,#12435,.F.);
#18791=ORIENTED_EDGE('',*,*,#12438,.F.);
#18792=ORIENTED_EDGE('',*,*,#12441,.F.);
#18793=ORIENTED_EDGE('',*,*,#12444,.F.);
#18794=ORIENTED_EDGE('',*,*,#12447,.F.);
#18795=ORIENTED_EDGE('',*,*,#12450,.F.);
#18796=ORIENTED_EDGE('',*,*,#12453,.F.);
#18797=ORIENTED_EDGE('',*,*,#12456,.F.);
#18798=ORIENTED_EDGE('',*,*,#12750,.F.);
#18799=ORIENTED_EDGE('',*,*,#12461,.F.);
#18800=ORIENTED_EDGE('',*,*,#12722,.F.);
#18801=ORIENTED_EDGE('',*,*,#12025,.F.);
#18802=ORIENTED_EDGE('',*,*,#12753,.F.);
#18803=ORIENTED_EDGE('',*,*,#12023,.F.);
#18804=ORIENTED_EDGE('',*,*,#12020,.F.);
#18805=ORIENTED_EDGE('',*,*,#12017,.F.);
#18806=ORIENTED_EDGE('',*,*,#12014,.F.);
#18807=ORIENTED_EDGE('',*,*,#12011,.F.);
#18808=ORIENTED_EDGE('',*,*,#12008,.F.);
#18809=ORIENTED_EDGE('',*,*,#12005,.F.);
#18810=ORIENTED_EDGE('',*,*,#12002,.F.);
#18811=ORIENTED_EDGE('',*,*,#11999,.F.);
#18812=ORIENTED_EDGE('',*,*,#11996,.F.);
#18813=ORIENTED_EDGE('',*,*,#11993,.F.);
#18814=ORIENTED_EDGE('',*,*,#11990,.F.);
#18815=ORIENTED_EDGE('',*,*,#11987,.F.);
#18816=ORIENTED_EDGE('',*,*,#11984,.F.);
#18817=ORIENTED_EDGE('',*,*,#11981,.F.);
#18818=ORIENTED_EDGE('',*,*,#11978,.F.);
#18819=ORIENTED_EDGE('',*,*,#11975,.F.);
#18820=ORIENTED_EDGE('',*,*,#11972,.F.);
#18821=ORIENTED_EDGE('',*,*,#11969,.F.);
#18822=ORIENTED_EDGE('',*,*,#12754,.F.);
#18823=ORIENTED_EDGE('',*,*,#11967,.F.);
#18824=ORIENTED_EDGE('',*,*,#11971,.F.);
#18825=ORIENTED_EDGE('',*,*,#11974,.F.);
#18826=ORIENTED_EDGE('',*,*,#11977,.F.);
#18827=ORIENTED_EDGE('',*,*,#11980,.F.);
#18828=ORIENTED_EDGE('',*,*,#11983,.F.);
#18829=ORIENTED_EDGE('',*,*,#11986,.F.);
#18830=ORIENTED_EDGE('',*,*,#11989,.F.);
#18831=ORIENTED_EDGE('',*,*,#11992,.F.);
#18832=ORIENTED_EDGE('',*,*,#11995,.F.);
#18833=ORIENTED_EDGE('',*,*,#11998,.F.);
#18834=ORIENTED_EDGE('',*,*,#12001,.F.);
#18835=ORIENTED_EDGE('',*,*,#12004,.F.);
#18836=ORIENTED_EDGE('',*,*,#12007,.F.);
#18837=ORIENTED_EDGE('',*,*,#12010,.F.);
#18838=ORIENTED_EDGE('',*,*,#12013,.F.);
#18839=ORIENTED_EDGE('',*,*,#12016,.F.);
#18840=ORIENTED_EDGE('',*,*,#12019,.F.);
#18841=ORIENTED_EDGE('',*,*,#12022,.F.);
#18842=ORIENTED_EDGE('',*,*,#12755,.F.);
#18843=ORIENTED_EDGE('',*,*,#12027,.F.);
#18844=ORIENTED_EDGE('',*,*,#12723,.F.);
#18845=ORIENTED_EDGE('',*,*,#12459,.T.);
#18846=ORIENTED_EDGE('',*,*,#12751,.T.);
#18847=ORIENTED_EDGE('',*,*,#12457,.T.);
#18848=ORIENTED_EDGE('',*,*,#12454,.T.);
#18849=ORIENTED_EDGE('',*,*,#12451,.T.);
#18850=ORIENTED_EDGE('',*,*,#12448,.T.);
#18851=ORIENTED_EDGE('',*,*,#12445,.T.);
#18852=ORIENTED_EDGE('',*,*,#12442,.T.);
#18853=ORIENTED_EDGE('',*,*,#12439,.T.);
#18854=ORIENTED_EDGE('',*,*,#12436,.T.);
#18855=ORIENTED_EDGE('',*,*,#12433,.T.);
#18856=ORIENTED_EDGE('',*,*,#12430,.T.);
#18857=ORIENTED_EDGE('',*,*,#12427,.T.);
#18858=ORIENTED_EDGE('',*,*,#12424,.T.);
#18859=ORIENTED_EDGE('',*,*,#12421,.T.);
#18860=ORIENTED_EDGE('',*,*,#12418,.T.);
#18861=ORIENTED_EDGE('',*,*,#12415,.T.);
#18862=ORIENTED_EDGE('',*,*,#12412,.T.);
#18863=ORIENTED_EDGE('',*,*,#12409,.T.);
#18864=ORIENTED_EDGE('',*,*,#12406,.T.);
#18865=ORIENTED_EDGE('',*,*,#12403,.T.);
#18866=ORIENTED_EDGE('',*,*,#12396,.T.);
#18867=ORIENTED_EDGE('',*,*,#12756,.T.);
#18868=ORIENTED_EDGE('',*,*,#12393,.F.);
#18869=ORIENTED_EDGE('',*,*,#12757,.F.);
#18870=ORIENTED_EDGE('',*,*,#12758,.F.);
#18871=ORIENTED_EDGE('',*,*,#12339,.F.);
#18872=ORIENTED_EDGE('',*,*,#12343,.F.);
#18873=ORIENTED_EDGE('',*,*,#12346,.F.);
#18874=ORIENTED_EDGE('',*,*,#12349,.F.);
#18875=ORIENTED_EDGE('',*,*,#12352,.F.);
#18876=ORIENTED_EDGE('',*,*,#12355,.F.);
#18877=ORIENTED_EDGE('',*,*,#12358,.F.);
#18878=ORIENTED_EDGE('',*,*,#12361,.F.);
#18879=ORIENTED_EDGE('',*,*,#12364,.F.);
#18880=ORIENTED_EDGE('',*,*,#12367,.F.);
#18881=ORIENTED_EDGE('',*,*,#12370,.F.);
#18882=ORIENTED_EDGE('',*,*,#12373,.F.);
#18883=ORIENTED_EDGE('',*,*,#12376,.F.);
#18884=ORIENTED_EDGE('',*,*,#12379,.F.);
#18885=ORIENTED_EDGE('',*,*,#12382,.F.);
#18886=ORIENTED_EDGE('',*,*,#12385,.F.);
#18887=ORIENTED_EDGE('',*,*,#12388,.F.);
#18888=ORIENTED_EDGE('',*,*,#12391,.F.);
#18889=ORIENTED_EDGE('',*,*,#12394,.F.);
#18890=ORIENTED_EDGE('',*,*,#12756,.F.);
#18891=ORIENTED_EDGE('',*,*,#12399,.F.);
#18892=ORIENTED_EDGE('',*,*,#12730,.F.);
#18893=ORIENTED_EDGE('',*,*,#12335,.F.);
#18894=ORIENTED_EDGE('',*,*,#12759,.F.);
#18895=ORIENTED_EDGE('',*,*,#12333,.F.);
#18896=ORIENTED_EDGE('',*,*,#12330,.F.);
#18897=ORIENTED_EDGE('',*,*,#12327,.F.);
#18898=ORIENTED_EDGE('',*,*,#12324,.F.);
#18899=ORIENTED_EDGE('',*,*,#12321,.F.);
#18900=ORIENTED_EDGE('',*,*,#12318,.F.);
#18901=ORIENTED_EDGE('',*,*,#12315,.F.);
#18902=ORIENTED_EDGE('',*,*,#12312,.F.);
#18903=ORIENTED_EDGE('',*,*,#12309,.F.);
#18904=ORIENTED_EDGE('',*,*,#12306,.F.);
#18905=ORIENTED_EDGE('',*,*,#12303,.F.);
#18906=ORIENTED_EDGE('',*,*,#12300,.F.);
#18907=ORIENTED_EDGE('',*,*,#12297,.F.);
#18908=ORIENTED_EDGE('',*,*,#12294,.F.);
#18909=ORIENTED_EDGE('',*,*,#12291,.F.);
#18910=ORIENTED_EDGE('',*,*,#12288,.F.);
#18911=ORIENTED_EDGE('',*,*,#12285,.F.);
#18912=ORIENTED_EDGE('',*,*,#12282,.F.);
#18913=ORIENTED_EDGE('',*,*,#12279,.F.);
#18914=ORIENTED_EDGE('',*,*,#12760,.F.);
#18915=ORIENTED_EDGE('',*,*,#12277,.F.);
#18916=ORIENTED_EDGE('',*,*,#12281,.F.);
#18917=ORIENTED_EDGE('',*,*,#12284,.F.);
#18918=ORIENTED_EDGE('',*,*,#12287,.F.);
#18919=ORIENTED_EDGE('',*,*,#12290,.F.);
#18920=ORIENTED_EDGE('',*,*,#12293,.F.);
#18921=ORIENTED_EDGE('',*,*,#12296,.F.);
#18922=ORIENTED_EDGE('',*,*,#12299,.F.);
#18923=ORIENTED_EDGE('',*,*,#12302,.F.);
#18924=ORIENTED_EDGE('',*,*,#12305,.F.);
#18925=ORIENTED_EDGE('',*,*,#12308,.F.);
#18926=ORIENTED_EDGE('',*,*,#12311,.F.);
#18927=ORIENTED_EDGE('',*,*,#12314,.F.);
#18928=ORIENTED_EDGE('',*,*,#12317,.F.);
#18929=ORIENTED_EDGE('',*,*,#12320,.F.);
#18930=ORIENTED_EDGE('',*,*,#12323,.F.);
#18931=ORIENTED_EDGE('',*,*,#12326,.F.);
#18932=ORIENTED_EDGE('',*,*,#12329,.F.);
#18933=ORIENTED_EDGE('',*,*,#12332,.F.);
#18934=ORIENTED_EDGE('',*,*,#12761,.F.);
#18935=ORIENTED_EDGE('',*,*,#12337,.F.);
#18936=ORIENTED_EDGE('',*,*,#12731,.F.);
#18937=ORIENTED_EDGE('',*,*,#12397,.T.);
#18938=ORIENTED_EDGE('',*,*,#12757,.T.);
#18939=ORIENTED_EDGE('',*,*,#12395,.T.);
#18940=ORIENTED_EDGE('',*,*,#12392,.T.);
#18941=ORIENTED_EDGE('',*,*,#12389,.T.);
#18942=ORIENTED_EDGE('',*,*,#12386,.T.);
#18943=ORIENTED_EDGE('',*,*,#12383,.T.);
#18944=ORIENTED_EDGE('',*,*,#12380,.T.);
#18945=ORIENTED_EDGE('',*,*,#12377,.T.);
#18946=ORIENTED_EDGE('',*,*,#12374,.T.);
#18947=ORIENTED_EDGE('',*,*,#12371,.T.);
#18948=ORIENTED_EDGE('',*,*,#12368,.T.);
#18949=ORIENTED_EDGE('',*,*,#12365,.T.);
#18950=ORIENTED_EDGE('',*,*,#12362,.T.);
#18951=ORIENTED_EDGE('',*,*,#12359,.T.);
#18952=ORIENTED_EDGE('',*,*,#12356,.T.);
#18953=ORIENTED_EDGE('',*,*,#12353,.T.);
#18954=ORIENTED_EDGE('',*,*,#12350,.T.);
#18955=ORIENTED_EDGE('',*,*,#12347,.T.);
#18956=ORIENTED_EDGE('',*,*,#12344,.T.);
#18957=ORIENTED_EDGE('',*,*,#12341,.T.);
#18958=ORIENTED_EDGE('',*,*,#12334,.T.);
#18959=ORIENTED_EDGE('',*,*,#12761,.T.);
#18960=ORIENTED_EDGE('',*,*,#12331,.F.);
#18961=ORIENTED_EDGE('',*,*,#12759,.T.);
#18962=ORIENTED_EDGE('',*,*,#12272,.T.);
#18963=ORIENTED_EDGE('',*,*,#12737,.T.);
#18964=ORIENTED_EDGE('',*,*,#12269,.F.);
#18965=ORIENTED_EDGE('',*,*,#12735,.T.);
#18966=ORIENTED_EDGE('',*,*,#12210,.T.);
#18967=ORIENTED_EDGE('',*,*,#12743,.T.);
#18968=ORIENTED_EDGE('',*,*,#12207,.F.);
#18969=ORIENTED_EDGE('',*,*,#12741,.T.);
#18970=ORIENTED_EDGE('',*,*,#12148,.T.);
#18971=ORIENTED_EDGE('',*,*,#12716,.T.);
#18972=ORIENTED_EDGE('',*,*,#12145,.F.);
#18973=ORIENTED_EDGE('',*,*,#12714,.T.);
#18974=ORIENTED_EDGE('',*,*,#12086,.T.);
#18975=ORIENTED_EDGE('',*,*,#12749,.T.);
#18976=ORIENTED_EDGE('',*,*,#12083,.F.);
#18977=ORIENTED_EDGE('',*,*,#12747,.T.);
#18978=ORIENTED_EDGE('',*,*,#12024,.T.);
#18979=ORIENTED_EDGE('',*,*,#12755,.T.);
#18980=ORIENTED_EDGE('',*,*,#12021,.F.);
#18981=ORIENTED_EDGE('',*,*,#12753,.T.);
#18982=ORIENTED_EDGE('',*,*,#12762,.T.);
#18983=ORIENTED_EDGE('',*,*,#12763,.T.);
#18984=ORIENTED_EDGE('',*,*,#12721,.F.);
#18985=ORIENTED_EDGE('',*,*,#12764,.F.);
#18986=ORIENTED_EDGE('',*,*,#12765,.T.);
#18987=ORIENTED_EDGE('',*,*,#12764,.T.);
#18988=ORIENTED_EDGE('',*,*,#12720,.F.);
#18989=ORIENTED_EDGE('',*,*,#12766,.F.);
#18990=ORIENTED_EDGE('',*,*,#12767,.T.);
#18991=ORIENTED_EDGE('',*,*,#12766,.T.);
#18992=ORIENTED_EDGE('',*,*,#12719,.F.);
#18993=ORIENTED_EDGE('',*,*,#12768,.F.);
#18994=ORIENTED_EDGE('',*,*,#12769,.T.);
#18995=ORIENTED_EDGE('',*,*,#12768,.T.);
#18996=ORIENTED_EDGE('',*,*,#12718,.F.);
#18997=ORIENTED_EDGE('',*,*,#12763,.F.);
#18998=ORIENTED_EDGE('',*,*,#12769,.F.);
#18999=ORIENTED_EDGE('',*,*,#12762,.F.);
#19000=ORIENTED_EDGE('',*,*,#12765,.F.);
#19001=ORIENTED_EDGE('',*,*,#12767,.F.);
#19002=ORIENTED_EDGE('',*,*,#12712,.T.);
#19003=ORIENTED_EDGE('',*,*,#12092,.T.);
#19004=ORIENTED_EDGE('',*,*,#12715,.T.);
#19005=ORIENTED_EDGE('',*,*,#12650,.T.);
#19006=ORIENTED_EDGE('',*,*,#12734,.T.);
#19007=ORIENTED_EDGE('',*,*,#12216,.T.);
#19008=ORIENTED_EDGE('',*,*,#12736,.T.);
#19009=ORIENTED_EDGE('',*,*,#12588,.T.);
#19010=ORIENTED_EDGE('',*,*,#12740,.T.);
#19011=ORIENTED_EDGE('',*,*,#12154,.T.);
#19012=ORIENTED_EDGE('',*,*,#12742,.T.);
#19013=ORIENTED_EDGE('',*,*,#12526,.T.);
#19014=ORIENTED_EDGE('',*,*,#12746,.T.);
#19015=ORIENTED_EDGE('',*,*,#12030,.T.);
#19016=ORIENTED_EDGE('',*,*,#12748,.T.);
#19017=ORIENTED_EDGE('',*,*,#12464,.T.);
#19018=ORIENTED_EDGE('',*,*,#12752,.T.);
#19019=ORIENTED_EDGE('',*,*,#11968,.T.);
#19020=ORIENTED_EDGE('',*,*,#12754,.T.);
#19021=ORIENTED_EDGE('',*,*,#12402,.T.);
#19022=ORIENTED_EDGE('',*,*,#12758,.T.);
#19023=ORIENTED_EDGE('',*,*,#12278,.T.);
#19024=ORIENTED_EDGE('',*,*,#12760,.T.);
#19025=ORIENTED_EDGE('',*,*,#12340,.T.);
#20300=CYLINDRICAL_SURFACE('',#23043,2.5175);
#20301=CYLINDRICAL_SURFACE('',#23045,2.5175);
#20302=CYLINDRICAL_SURFACE('',#23046,2.5175);
#20303=CYLINDRICAL_SURFACE('',#23047,2.5175);
#20304=CYLINDRICAL_SURFACE('',#23048,2.5175);
#20305=CYLINDRICAL_SURFACE('',#23049,2.5175);
#20306=CYLINDRICAL_SURFACE('',#23050,2.5175);
#20307=CYLINDRICAL_SURFACE('',#23051,2.5175);
#20308=CYLINDRICAL_SURFACE('',#23052,2.5175);
#20309=CYLINDRICAL_SURFACE('',#23053,2.5175);
#20310=CYLINDRICAL_SURFACE('',#23054,2.5175);
#20311=CYLINDRICAL_SURFACE('',#23055,2.5175);
#20312=CYLINDRICAL_SURFACE('',#23056,2.5175);
#20313=CYLINDRICAL_SURFACE('',#23057,2.5175);
#20314=CYLINDRICAL_SURFACE('',#23058,2.5175);
#20315=CYLINDRICAL_SURFACE('',#23059,2.5175);
#20316=CYLINDRICAL_SURFACE('',#23060,2.5175);
#20317=CYLINDRICAL_SURFACE('',#23061,2.5175);
#20318=CYLINDRICAL_SURFACE('',#23062,2.5175);
#20319=CYLINDRICAL_SURFACE('',#23063,2.5175);
#20320=CYLINDRICAL_SURFACE('',#23065,2.5175);
#20321=CYLINDRICAL_SURFACE('',#23067,2.5175);
#20322=CYLINDRICAL_SURFACE('',#23068,2.5175);
#20323=CYLINDRICAL_SURFACE('',#23069,2.5175);
#20324=CYLINDRICAL_SURFACE('',#23070,2.5175);
#20325=CYLINDRICAL_SURFACE('',#23071,2.5175);
#20326=CYLINDRICAL_SURFACE('',#23072,2.5175);
#20327=CYLINDRICAL_SURFACE('',#23073,2.5175);
#20328=CYLINDRICAL_SURFACE('',#23074,2.5175);
#20329=CYLINDRICAL_SURFACE('',#23075,2.5175);
#20330=CYLINDRICAL_SURFACE('',#23076,2.5175);
#20331=CYLINDRICAL_SURFACE('',#23077,2.5175);
#20332=CYLINDRICAL_SURFACE('',#23078,2.5175);
#20333=CYLINDRICAL_SURFACE('',#23079,2.5175);
#20334=CYLINDRICAL_SURFACE('',#23080,2.5175);
#20335=CYLINDRICAL_SURFACE('',#23081,2.5175);
#20336=CYLINDRICAL_SURFACE('',#23082,2.5175);
#20337=CYLINDRICAL_SURFACE('',#23083,2.5175);
#20338=CYLINDRICAL_SURFACE('',#23084,2.5175);
#20339=CYLINDRICAL_SURFACE('',#23085,2.5175);
#20340=CYLINDRICAL_SURFACE('',#23087,2.5175);
#20341=CYLINDRICAL_SURFACE('',#23089,2.5175);
#20342=CYLINDRICAL_SURFACE('',#23090,2.5175);
#20343=CYLINDRICAL_SURFACE('',#23091,2.5175);
#20344=CYLINDRICAL_SURFACE('',#23092,2.5175);
#20345=CYLINDRICAL_SURFACE('',#23093,2.5175);
#20346=CYLINDRICAL_SURFACE('',#23094,2.5175);
#20347=CYLINDRICAL_SURFACE('',#23095,2.5175);
#20348=CYLINDRICAL_SURFACE('',#23096,2.5175);
#20349=CYLINDRICAL_SURFACE('',#23097,2.5175);
#20350=CYLINDRICAL_SURFACE('',#23098,2.5175);
#20351=CYLINDRICAL_SURFACE('',#23099,2.5175);
#20352=CYLINDRICAL_SURFACE('',#23100,2.5175);
#20353=CYLINDRICAL_SURFACE('',#23101,2.5175);
#20354=CYLINDRICAL_SURFACE('',#23102,2.5175);
#20355=CYLINDRICAL_SURFACE('',#23103,2.5175);
#20356=CYLINDRICAL_SURFACE('',#23104,2.5175);
#20357=CYLINDRICAL_SURFACE('',#23105,2.5175);
#20358=CYLINDRICAL_SURFACE('',#23106,2.5175);
#20359=CYLINDRICAL_SURFACE('',#23107,2.5175);
#20360=CYLINDRICAL_SURFACE('',#23109,2.5175);
#20361=CYLINDRICAL_SURFACE('',#23111,2.5175);
#20362=CYLINDRICAL_SURFACE('',#23112,2.5175);
#20363=CYLINDRICAL_SURFACE('',#23113,2.5175);
#20364=CYLINDRICAL_SURFACE('',#23114,2.5175);
#20365=CYLINDRICAL_SURFACE('',#23115,2.5175);
#20366=CYLINDRICAL_SURFACE('',#23116,2.5175);
#20367=CYLINDRICAL_SURFACE('',#23117,2.5175);
#20368=CYLINDRICAL_SURFACE('',#23118,2.5175);
#20369=CYLINDRICAL_SURFACE('',#23119,2.5175);
#20370=CYLINDRICAL_SURFACE('',#23120,2.5175);
#20371=CYLINDRICAL_SURFACE('',#23121,2.5175);
#20372=CYLINDRICAL_SURFACE('',#23122,2.5175);
#20373=CYLINDRICAL_SURFACE('',#23123,2.5175);
#20374=CYLINDRICAL_SURFACE('',#23124,2.5175);
#20375=CYLINDRICAL_SURFACE('',#23125,2.5175);
#20376=CYLINDRICAL_SURFACE('',#23126,2.5175);
#20377=CYLINDRICAL_SURFACE('',#23127,2.5175);
#20378=CYLINDRICAL_SURFACE('',#23128,2.5175);
#20379=CYLINDRICAL_SURFACE('',#23129,2.5175);
#20380=CYLINDRICAL_SURFACE('',#23131,2.5175);
#20381=CYLINDRICAL_SURFACE('',#23133,2.5175);
#20382=CYLINDRICAL_SURFACE('',#23134,2.5175);
#20383=CYLINDRICAL_SURFACE('',#23135,2.5175);
#20384=CYLINDRICAL_SURFACE('',#23136,2.5175);
#20385=CYLINDRICAL_SURFACE('',#23137,2.5175);
#20386=CYLINDRICAL_SURFACE('',#23138,2.5175);
#20387=CYLINDRICAL_SURFACE('',#23139,2.5175);
#20388=CYLINDRICAL_SURFACE('',#23140,2.5175);
#20389=CYLINDRICAL_SURFACE('',#23141,2.5175);
#20390=CYLINDRICAL_SURFACE('',#23142,2.5175);
#20391=CYLINDRICAL_SURFACE('',#23143,2.5175);
#20392=CYLINDRICAL_SURFACE('',#23144,2.5175);
#20393=CYLINDRICAL_SURFACE('',#23145,2.5175);
#20394=CYLINDRICAL_SURFACE('',#23146,2.5175);
#20395=CYLINDRICAL_SURFACE('',#23147,2.5175);
#20396=CYLINDRICAL_SURFACE('',#23148,2.5175);
#20397=CYLINDRICAL_SURFACE('',#23149,2.5175);
#20398=CYLINDRICAL_SURFACE('',#23150,2.5175);
#20399=CYLINDRICAL_SURFACE('',#23151,2.5175);
#20400=CYLINDRICAL_SURFACE('',#23153,2.5175);
#20401=CYLINDRICAL_SURFACE('',#23155,2.5175);
#20402=CYLINDRICAL_SURFACE('',#23156,2.5175);
#20403=CYLINDRICAL_SURFACE('',#23157,2.5175);
#20404=CYLINDRICAL_SURFACE('',#23158,2.5175);
#20405=CYLINDRICAL_SURFACE('',#23159,2.5175);
#20406=CYLINDRICAL_SURFACE('',#23160,2.5175);
#20407=CYLINDRICAL_SURFACE('',#23161,2.5175);
#20408=CYLINDRICAL_SURFACE('',#23162,2.5175);
#20409=CYLINDRICAL_SURFACE('',#23163,2.5175);
#20410=CYLINDRICAL_SURFACE('',#23164,2.5175);
#20411=CYLINDRICAL_SURFACE('',#23165,2.5175);
#20412=CYLINDRICAL_SURFACE('',#23166,2.5175);
#20413=CYLINDRICAL_SURFACE('',#23167,2.5175);
#20414=CYLINDRICAL_SURFACE('',#23168,2.5175);
#20415=CYLINDRICAL_SURFACE('',#23169,2.5175);
#20416=CYLINDRICAL_SURFACE('',#23170,2.5175);
#20417=CYLINDRICAL_SURFACE('',#23171,2.5175);
#20418=CYLINDRICAL_SURFACE('',#23172,2.5175);
#20419=CYLINDRICAL_SURFACE('',#23173,2.5175);
#20420=CYLINDRICAL_SURFACE('',#23175,3.0735);
#20421=CYLINDRICAL_SURFACE('',#23177,3.0735);
#20422=CYLINDRICAL_SURFACE('',#23178,3.0735);
#20423=CYLINDRICAL_SURFACE('',#23179,3.0735);
#20424=CYLINDRICAL_SURFACE('',#23180,3.0735);
#20425=CYLINDRICAL_SURFACE('',#23181,3.0735);
#20426=CYLINDRICAL_SURFACE('',#23182,3.0735);
#20427=CYLINDRICAL_SURFACE('',#23183,3.0735);
#20428=CYLINDRICAL_SURFACE('',#23184,3.0735);
#20429=CYLINDRICAL_SURFACE('',#23185,3.0735);
#20430=CYLINDRICAL_SURFACE('',#23186,3.0735);
#20431=CYLINDRICAL_SURFACE('',#23187,3.0735);
#20432=CYLINDRICAL_SURFACE('',#23188,3.0735);
#20433=CYLINDRICAL_SURFACE('',#23189,3.0735);
#20434=CYLINDRICAL_SURFACE('',#23190,3.0735);
#20435=CYLINDRICAL_SURFACE('',#23191,3.0735);
#20436=CYLINDRICAL_SURFACE('',#23192,3.0735);
#20437=CYLINDRICAL_SURFACE('',#23193,3.0735);
#20438=CYLINDRICAL_SURFACE('',#23194,3.0735);
#20439=CYLINDRICAL_SURFACE('',#23195,3.0735);
#20440=CYLINDRICAL_SURFACE('',#23197,3.0735);
#20441=CYLINDRICAL_SURFACE('',#23199,3.0735);
#20442=CYLINDRICAL_SURFACE('',#23200,3.0735);
#20443=CYLINDRICAL_SURFACE('',#23201,3.0735);
#20444=CYLINDRICAL_SURFACE('',#23202,3.0735);
#20445=CYLINDRICAL_SURFACE('',#23203,3.0735);
#20446=CYLINDRICAL_SURFACE('',#23204,3.0735);
#20447=CYLINDRICAL_SURFACE('',#23205,3.0735);
#20448=CYLINDRICAL_SURFACE('',#23206,3.0735);
#20449=CYLINDRICAL_SURFACE('',#23207,3.0735);
#20450=CYLINDRICAL_SURFACE('',#23208,3.0735);
#20451=CYLINDRICAL_SURFACE('',#23209,3.0735);
#20452=CYLINDRICAL_SURFACE('',#23210,3.0735);
#20453=CYLINDRICAL_SURFACE('',#23211,3.0735);
#20454=CYLINDRICAL_SURFACE('',#23212,3.0735);
#20455=CYLINDRICAL_SURFACE('',#23213,3.0735);
#20456=CYLINDRICAL_SURFACE('',#23214,3.0735);
#20457=CYLINDRICAL_SURFACE('',#23215,3.0735);
#20458=CYLINDRICAL_SURFACE('',#23216,3.0735);
#20459=CYLINDRICAL_SURFACE('',#23217,3.0735);
#20460=CYLINDRICAL_SURFACE('',#23219,3.07349999999996);
#20461=CYLINDRICAL_SURFACE('',#23221,3.07349999999996);
#20462=CYLINDRICAL_SURFACE('',#23222,3.07349999999996);
#20463=CYLINDRICAL_SURFACE('',#23223,3.07349999999996);
#20464=CYLINDRICAL_SURFACE('',#23224,3.07349999999996);
#20465=CYLINDRICAL_SURFACE('',#23225,3.07349999999996);
#20466=CYLINDRICAL_SURFACE('',#23226,3.07349999999996);
#20467=CYLINDRICAL_SURFACE('',#23227,3.07349999999996);
#20468=CYLINDRICAL_SURFACE('',#23228,3.07349999999996);
#20469=CYLINDRICAL_SURFACE('',#23229,3.07349999999996);
#20470=CYLINDRICAL_SURFACE('',#23230,3.07349999999996);
#20471=CYLINDRICAL_SURFACE('',#23231,3.07349999999996);
#20472=CYLINDRICAL_SURFACE('',#23232,3.07349999999996);
#20473=CYLINDRICAL_SURFACE('',#23233,3.07349999999996);
#20474=CYLINDRICAL_SURFACE('',#23234,3.07349999999996);
#20475=CYLINDRICAL_SURFACE('',#23235,3.07349999999996);
#20476=CYLINDRICAL_SURFACE('',#23236,3.07349999999996);
#20477=CYLINDRICAL_SURFACE('',#23237,3.07349999999996);
#20478=CYLINDRICAL_SURFACE('',#23238,3.07349999999996);
#20479=CYLINDRICAL_SURFACE('',#23239,3.07349999999996);
#20480=CYLINDRICAL_SURFACE('',#23241,3.07349999999996);
#20481=CYLINDRICAL_SURFACE('',#23243,3.07349999999996);
#20482=CYLINDRICAL_SURFACE('',#23244,3.07349999999996);
#20483=CYLINDRICAL_SURFACE('',#23245,3.07349999999996);
#20484=CYLINDRICAL_SURFACE('',#23246,3.07349999999996);
#20485=CYLINDRICAL_SURFACE('',#23247,3.07349999999996);
#20486=CYLINDRICAL_SURFACE('',#23248,3.07349999999996);
#20487=CYLINDRICAL_SURFACE('',#23249,3.07349999999996);
#20488=CYLINDRICAL_SURFACE('',#23250,3.07349999999996);
#20489=CYLINDRICAL_SURFACE('',#23251,3.07349999999996);
#20490=CYLINDRICAL_SURFACE('',#23252,3.07349999999996);
#20491=CYLINDRICAL_SURFACE('',#23253,3.07349999999996);
#20492=CYLINDRICAL_SURFACE('',#23254,3.07349999999996);
#20493=CYLINDRICAL_SURFACE('',#23255,3.07349999999996);
#20494=CYLINDRICAL_SURFACE('',#23256,3.07349999999996);
#20495=CYLINDRICAL_SURFACE('',#23257,3.07349999999996);
#20496=CYLINDRICAL_SURFACE('',#23258,3.07349999999996);
#20497=CYLINDRICAL_SURFACE('',#23259,3.07349999999996);
#20498=CYLINDRICAL_SURFACE('',#23260,3.07349999999996);
#20499=CYLINDRICAL_SURFACE('',#23261,3.07349999999996);
#20500=CYLINDRICAL_SURFACE('',#23263,3.0735);
#20501=CYLINDRICAL_SURFACE('',#23265,3.0735);
#20502=CYLINDRICAL_SURFACE('',#23266,3.0735);
#20503=CYLINDRICAL_SURFACE('',#23267,3.0735);
#20504=CYLINDRICAL_SURFACE('',#23268,3.0735);
#20505=CYLINDRICAL_SURFACE('',#23269,3.0735);
#20506=CYLINDRICAL_SURFACE('',#23270,3.0735);
#20507=CYLINDRICAL_SURFACE('',#23271,3.0735);
#20508=CYLINDRICAL_SURFACE('',#23272,3.0735);
#20509=CYLINDRICAL_SURFACE('',#23273,3.0735);
#20510=CYLINDRICAL_SURFACE('',#23274,3.0735);
#20511=CYLINDRICAL_SURFACE('',#23275,3.0735);
#20512=CYLINDRICAL_SURFACE('',#23276,3.0735);
#20513=CYLINDRICAL_SURFACE('',#23277,3.0735);
#20514=CYLINDRICAL_SURFACE('',#23278,3.0735);
#20515=CYLINDRICAL_SURFACE('',#23279,3.0735);
#20516=CYLINDRICAL_SURFACE('',#23280,3.0735);
#20517=CYLINDRICAL_SURFACE('',#23281,3.0735);
#20518=CYLINDRICAL_SURFACE('',#23282,3.0735);
#20519=CYLINDRICAL_SURFACE('',#23283,3.0735);
#20520=CYLINDRICAL_SURFACE('',#23285,3.0735);
#20521=CYLINDRICAL_SURFACE('',#23287,3.0735);
#20522=CYLINDRICAL_SURFACE('',#23288,3.0735);
#20523=CYLINDRICAL_SURFACE('',#23289,3.0735);
#20524=CYLINDRICAL_SURFACE('',#23290,3.0735);
#20525=CYLINDRICAL_SURFACE('',#23291,3.0735);
#20526=CYLINDRICAL_SURFACE('',#23292,3.0735);
#20527=CYLINDRICAL_SURFACE('',#23293,3.0735);
#20528=CYLINDRICAL_SURFACE('',#23294,3.0735);
#20529=CYLINDRICAL_SURFACE('',#23295,3.0735);
#20530=CYLINDRICAL_SURFACE('',#23296,3.0735);
#20531=CYLINDRICAL_SURFACE('',#23297,3.0735);
#20532=CYLINDRICAL_SURFACE('',#23298,3.0735);
#20533=CYLINDRICAL_SURFACE('',#23299,3.0735);
#20534=CYLINDRICAL_SURFACE('',#23300,3.0735);
#20535=CYLINDRICAL_SURFACE('',#23301,3.0735);
#20536=CYLINDRICAL_SURFACE('',#23302,3.0735);
#20537=CYLINDRICAL_SURFACE('',#23303,3.0735);
#20538=CYLINDRICAL_SURFACE('',#23304,3.0735);
#20539=CYLINDRICAL_SURFACE('',#23305,3.0735);
#20540=CYLINDRICAL_SURFACE('',#23307,3.0735);
#20541=CYLINDRICAL_SURFACE('',#23309,3.0735);
#20542=CYLINDRICAL_SURFACE('',#23310,3.07349999999996);
#20543=CYLINDRICAL_SURFACE('',#23311,3.07349999999996);
#20544=CYLINDRICAL_SURFACE('',#23312,3.0735);
#20545=CYLINDRICAL_SURFACE('',#23313,3.0735);
#20546=CYLINDRICAL_SURFACE('',#23314,2.5175);
#20547=CYLINDRICAL_SURFACE('',#23315,2.5175);
#20548=CYLINDRICAL_SURFACE('',#23316,2.5175);
#20549=CYLINDRICAL_SURFACE('',#23317,2.5175);
#20550=CYLINDRICAL_SURFACE('',#23318,2.5175);
#20551=CYLINDRICAL_SURFACE('',#23319,2.5175);
#21419=ADVANCED_FACE('',(#3299),#20300,.F.);
#21420=ADVANCED_FACE('',(#3300),#20301,.F.);
#21421=ADVANCED_FACE('',(#3301),#20302,.F.);
#21422=ADVANCED_FACE('',(#3302),#20303,.F.);
#21423=ADVANCED_FACE('',(#3303),#20304,.F.);
#21424=ADVANCED_FACE('',(#3304),#20305,.F.);
#21425=ADVANCED_FACE('',(#3305),#20306,.F.);
#21426=ADVANCED_FACE('',(#3306),#20307,.F.);
#21427=ADVANCED_FACE('',(#3307),#20308,.F.);
#21428=ADVANCED_FACE('',(#3308),#20309,.F.);
#21429=ADVANCED_FACE('',(#3309),#20310,.F.);
#21430=ADVANCED_FACE('',(#3310),#20311,.F.);
#21431=ADVANCED_FACE('',(#3311),#20312,.F.);
#21432=ADVANCED_FACE('',(#3312),#20313,.F.);
#21433=ADVANCED_FACE('',(#3313),#20314,.F.);
#21434=ADVANCED_FACE('',(#3314),#20315,.F.);
#21435=ADVANCED_FACE('',(#3315),#20316,.F.);
#21436=ADVANCED_FACE('',(#3316),#20317,.F.);
#21437=ADVANCED_FACE('',(#3317),#20318,.F.);
#21438=ADVANCED_FACE('',(#3318),#20319,.F.);
#21439=ADVANCED_FACE('',(#3319),#20320,.F.);
#21440=ADVANCED_FACE('',(#3320),#20321,.F.);
#21441=ADVANCED_FACE('',(#3321),#20322,.F.);
#21442=ADVANCED_FACE('',(#3322),#20323,.F.);
#21443=ADVANCED_FACE('',(#3323),#20324,.F.);
#21444=ADVANCED_FACE('',(#3324),#20325,.F.);
#21445=ADVANCED_FACE('',(#3325),#20326,.F.);
#21446=ADVANCED_FACE('',(#3326),#20327,.F.);
#21447=ADVANCED_FACE('',(#3327),#20328,.F.);
#21448=ADVANCED_FACE('',(#3328),#20329,.F.);
#21449=ADVANCED_FACE('',(#3329),#20330,.F.);
#21450=ADVANCED_FACE('',(#3330),#20331,.F.);
#21451=ADVANCED_FACE('',(#3331),#20332,.F.);
#21452=ADVANCED_FACE('',(#3332),#20333,.F.);
#21453=ADVANCED_FACE('',(#3333),#20334,.F.);
#21454=ADVANCED_FACE('',(#3334),#20335,.F.);
#21455=ADVANCED_FACE('',(#3335),#20336,.F.);
#21456=ADVANCED_FACE('',(#3336),#20337,.F.);
#21457=ADVANCED_FACE('',(#3337),#20338,.F.);
#21458=ADVANCED_FACE('',(#3338),#20339,.F.);
#21459=ADVANCED_FACE('',(#3339),#20340,.F.);
#21460=ADVANCED_FACE('',(#3340),#20341,.F.);
#21461=ADVANCED_FACE('',(#3341),#20342,.F.);
#21462=ADVANCED_FACE('',(#3342),#20343,.F.);
#21463=ADVANCED_FACE('',(#3343),#20344,.F.);
#21464=ADVANCED_FACE('',(#3344),#20345,.F.);
#21465=ADVANCED_FACE('',(#3345),#20346,.F.);
#21466=ADVANCED_FACE('',(#3346),#20347,.F.);
#21467=ADVANCED_FACE('',(#3347),#20348,.F.);
#21468=ADVANCED_FACE('',(#3348),#20349,.F.);
#21469=ADVANCED_FACE('',(#3349),#20350,.F.);
#21470=ADVANCED_FACE('',(#3350),#20351,.F.);
#21471=ADVANCED_FACE('',(#3351),#20352,.F.);
#21472=ADVANCED_FACE('',(#3352),#20353,.F.);
#21473=ADVANCED_FACE('',(#3353),#20354,.F.);
#21474=ADVANCED_FACE('',(#3354),#20355,.F.);
#21475=ADVANCED_FACE('',(#3355),#20356,.F.);
#21476=ADVANCED_FACE('',(#3356),#20357,.F.);
#21477=ADVANCED_FACE('',(#3357),#20358,.F.);
#21478=ADVANCED_FACE('',(#3358),#20359,.F.);
#21479=ADVANCED_FACE('',(#3359),#20360,.F.);
#21480=ADVANCED_FACE('',(#3360),#20361,.F.);
#21481=ADVANCED_FACE('',(#3361),#20362,.F.);
#21482=ADVANCED_FACE('',(#3362),#20363,.F.);
#21483=ADVANCED_FACE('',(#3363),#20364,.F.);
#21484=ADVANCED_FACE('',(#3364),#20365,.F.);
#21485=ADVANCED_FACE('',(#3365),#20366,.F.);
#21486=ADVANCED_FACE('',(#3366),#20367,.F.);
#21487=ADVANCED_FACE('',(#3367),#20368,.F.);
#21488=ADVANCED_FACE('',(#3368),#20369,.F.);
#21489=ADVANCED_FACE('',(#3369),#20370,.F.);
#21490=ADVANCED_FACE('',(#3370),#20371,.F.);
#21491=ADVANCED_FACE('',(#3371),#20372,.F.);
#21492=ADVANCED_FACE('',(#3372),#20373,.F.);
#21493=ADVANCED_FACE('',(#3373),#20374,.F.);
#21494=ADVANCED_FACE('',(#3374),#20375,.F.);
#21495=ADVANCED_FACE('',(#3375),#20376,.F.);
#21496=ADVANCED_FACE('',(#3376),#20377,.F.);
#21497=ADVANCED_FACE('',(#3377),#20378,.F.);
#21498=ADVANCED_FACE('',(#3378),#20379,.F.);
#21499=ADVANCED_FACE('',(#3379),#20380,.F.);
#21500=ADVANCED_FACE('',(#3380),#20381,.F.);
#21501=ADVANCED_FACE('',(#3381),#20382,.F.);
#21502=ADVANCED_FACE('',(#3382),#20383,.F.);
#21503=ADVANCED_FACE('',(#3383),#20384,.F.);
#21504=ADVANCED_FACE('',(#3384),#20385,.F.);
#21505=ADVANCED_FACE('',(#3385),#20386,.F.);
#21506=ADVANCED_FACE('',(#3386),#20387,.F.);
#21507=ADVANCED_FACE('',(#3387),#20388,.F.);
#21508=ADVANCED_FACE('',(#3388),#20389,.F.);
#21509=ADVANCED_FACE('',(#3389),#20390,.F.);
#21510=ADVANCED_FACE('',(#3390),#20391,.F.);
#21511=ADVANCED_FACE('',(#3391),#20392,.F.);
#21512=ADVANCED_FACE('',(#3392),#20393,.F.);
#21513=ADVANCED_FACE('',(#3393),#20394,.F.);
#21514=ADVANCED_FACE('',(#3394),#20395,.F.);
#21515=ADVANCED_FACE('',(#3395),#20396,.F.);
#21516=ADVANCED_FACE('',(#3396),#20397,.F.);
#21517=ADVANCED_FACE('',(#3397),#20398,.F.);
#21518=ADVANCED_FACE('',(#3398),#20399,.F.);
#21519=ADVANCED_FACE('',(#3399),#20400,.F.);
#21520=ADVANCED_FACE('',(#3400),#20401,.F.);
#21521=ADVANCED_FACE('',(#3401),#20402,.F.);
#21522=ADVANCED_FACE('',(#3402),#20403,.F.);
#21523=ADVANCED_FACE('',(#3403),#20404,.F.);
#21524=ADVANCED_FACE('',(#3404),#20405,.F.);
#21525=ADVANCED_FACE('',(#3405),#20406,.F.);
#21526=ADVANCED_FACE('',(#3406),#20407,.F.);
#21527=ADVANCED_FACE('',(#3407),#20408,.F.);
#21528=ADVANCED_FACE('',(#3408),#20409,.F.);
#21529=ADVANCED_FACE('',(#3409),#20410,.F.);
#21530=ADVANCED_FACE('',(#3410),#20411,.F.);
#21531=ADVANCED_FACE('',(#3411),#20412,.F.);
#21532=ADVANCED_FACE('',(#3412),#20413,.F.);
#21533=ADVANCED_FACE('',(#3413),#20414,.F.);
#21534=ADVANCED_FACE('',(#3414),#20415,.F.);
#21535=ADVANCED_FACE('',(#3415),#20416,.F.);
#21536=ADVANCED_FACE('',(#3416),#20417,.F.);
#21537=ADVANCED_FACE('',(#3417),#20418,.F.);
#21538=ADVANCED_FACE('',(#3418),#20419,.F.);
#21539=ADVANCED_FACE('',(#3419),#20420,.F.);
#21540=ADVANCED_FACE('',(#3420),#20421,.F.);
#21541=ADVANCED_FACE('',(#3421),#20422,.F.);
#21542=ADVANCED_FACE('',(#3422),#20423,.F.);
#21543=ADVANCED_FACE('',(#3423),#20424,.F.);
#21544=ADVANCED_FACE('',(#3424),#20425,.F.);
#21545=ADVANCED_FACE('',(#3425),#20426,.F.);
#21546=ADVANCED_FACE('',(#3426),#20427,.F.);
#21547=ADVANCED_FACE('',(#3427),#20428,.F.);
#21548=ADVANCED_FACE('',(#3428),#20429,.F.);
#21549=ADVANCED_FACE('',(#3429),#20430,.F.);
#21550=ADVANCED_FACE('',(#3430),#20431,.F.);
#21551=ADVANCED_FACE('',(#3431),#20432,.F.);
#21552=ADVANCED_FACE('',(#3432),#20433,.F.);
#21553=ADVANCED_FACE('',(#3433),#20434,.F.);
#21554=ADVANCED_FACE('',(#3434),#20435,.F.);
#21555=ADVANCED_FACE('',(#3435),#20436,.F.);
#21556=ADVANCED_FACE('',(#3436),#20437,.F.);
#21557=ADVANCED_FACE('',(#3437),#20438,.F.);
#21558=ADVANCED_FACE('',(#3438),#20439,.F.);
#21559=ADVANCED_FACE('',(#3439),#20440,.F.);
#21560=ADVANCED_FACE('',(#3440),#20441,.F.);
#21561=ADVANCED_FACE('',(#3441),#20442,.F.);
#21562=ADVANCED_FACE('',(#3442),#20443,.F.);
#21563=ADVANCED_FACE('',(#3443),#20444,.F.);
#21564=ADVANCED_FACE('',(#3444),#20445,.F.);
#21565=ADVANCED_FACE('',(#3445),#20446,.F.);
#21566=ADVANCED_FACE('',(#3446),#20447,.F.);
#21567=ADVANCED_FACE('',(#3447),#20448,.F.);
#21568=ADVANCED_FACE('',(#3448),#20449,.F.);
#21569=ADVANCED_FACE('',(#3449),#20450,.F.);
#21570=ADVANCED_FACE('',(#3450),#20451,.F.);
#21571=ADVANCED_FACE('',(#3451),#20452,.F.);
#21572=ADVANCED_FACE('',(#3452),#20453,.F.);
#21573=ADVANCED_FACE('',(#3453),#20454,.F.);
#21574=ADVANCED_FACE('',(#3454),#20455,.F.);
#21575=ADVANCED_FACE('',(#3455),#20456,.F.);
#21576=ADVANCED_FACE('',(#3456),#20457,.F.);
#21577=ADVANCED_FACE('',(#3457),#20458,.F.);
#21578=ADVANCED_FACE('',(#3458),#20459,.F.);
#21579=ADVANCED_FACE('',(#3459),#20460,.F.);
#21580=ADVANCED_FACE('',(#3460),#20461,.F.);
#21581=ADVANCED_FACE('',(#3461),#20462,.F.);
#21582=ADVANCED_FACE('',(#3462),#20463,.F.);
#21583=ADVANCED_FACE('',(#3463),#20464,.F.);
#21584=ADVANCED_FACE('',(#3464),#20465,.F.);
#21585=ADVANCED_FACE('',(#3465),#20466,.F.);
#21586=ADVANCED_FACE('',(#3466),#20467,.F.);
#21587=ADVANCED_FACE('',(#3467),#20468,.F.);
#21588=ADVANCED_FACE('',(#3468),#20469,.F.);
#21589=ADVANCED_FACE('',(#3469),#20470,.F.);
#21590=ADVANCED_FACE('',(#3470),#20471,.F.);
#21591=ADVANCED_FACE('',(#3471),#20472,.F.);
#21592=ADVANCED_FACE('',(#3472),#20473,.F.);
#21593=ADVANCED_FACE('',(#3473),#20474,.F.);
#21594=ADVANCED_FACE('',(#3474),#20475,.F.);
#21595=ADVANCED_FACE('',(#3475),#20476,.F.);
#21596=ADVANCED_FACE('',(#3476),#20477,.F.);
#21597=ADVANCED_FACE('',(#3477),#20478,.F.);
#21598=ADVANCED_FACE('',(#3478),#20479,.F.);
#21599=ADVANCED_FACE('',(#3479),#20480,.F.);
#21600=ADVANCED_FACE('',(#3480),#20481,.F.);
#21601=ADVANCED_FACE('',(#3481),#20482,.F.);
#21602=ADVANCED_FACE('',(#3482),#20483,.F.);
#21603=ADVANCED_FACE('',(#3483),#20484,.F.);
#21604=ADVANCED_FACE('',(#3484),#20485,.F.);
#21605=ADVANCED_FACE('',(#3485),#20486,.F.);
#21606=ADVANCED_FACE('',(#3486),#20487,.F.);
#21607=ADVANCED_FACE('',(#3487),#20488,.F.);
#21608=ADVANCED_FACE('',(#3488),#20489,.F.);
#21609=ADVANCED_FACE('',(#3489),#20490,.F.);
#21610=ADVANCED_FACE('',(#3490),#20491,.F.);
#21611=ADVANCED_FACE('',(#3491),#20492,.F.);
#21612=ADVANCED_FACE('',(#3492),#20493,.F.);
#21613=ADVANCED_FACE('',(#3493),#20494,.F.);
#21614=ADVANCED_FACE('',(#3494),#20495,.F.);
#21615=ADVANCED_FACE('',(#3495),#20496,.F.);
#21616=ADVANCED_FACE('',(#3496),#20497,.F.);
#21617=ADVANCED_FACE('',(#3497),#20498,.F.);
#21618=ADVANCED_FACE('',(#3498),#20499,.F.);
#21619=ADVANCED_FACE('',(#3499),#20500,.F.);
#21620=ADVANCED_FACE('',(#3500),#20501,.F.);
#21621=ADVANCED_FACE('',(#3501),#20502,.F.);
#21622=ADVANCED_FACE('',(#3502),#20503,.F.);
#21623=ADVANCED_FACE('',(#3503),#20504,.F.);
#21624=ADVANCED_FACE('',(#3504),#20505,.F.);
#21625=ADVANCED_FACE('',(#3505),#20506,.F.);
#21626=ADVANCED_FACE('',(#3506),#20507,.F.);
#21627=ADVANCED_FACE('',(#3507),#20508,.F.);
#21628=ADVANCED_FACE('',(#3508),#20509,.F.);
#21629=ADVANCED_FACE('',(#3509),#20510,.F.);
#21630=ADVANCED_FACE('',(#3510),#20511,.F.);
#21631=ADVANCED_FACE('',(#3511),#20512,.F.);
#21632=ADVANCED_FACE('',(#3512),#20513,.F.);
#21633=ADVANCED_FACE('',(#3513),#20514,.F.);
#21634=ADVANCED_FACE('',(#3514),#20515,.F.);
#21635=ADVANCED_FACE('',(#3515),#20516,.F.);
#21636=ADVANCED_FACE('',(#3516),#20517,.F.);
#21637=ADVANCED_FACE('',(#3517),#20518,.F.);
#21638=ADVANCED_FACE('',(#3518),#20519,.F.);
#21639=ADVANCED_FACE('',(#3519),#20520,.F.);
#21640=ADVANCED_FACE('',(#3520),#20521,.F.);
#21641=ADVANCED_FACE('',(#3521),#20522,.F.);
#21642=ADVANCED_FACE('',(#3522),#20523,.F.);
#21643=ADVANCED_FACE('',(#3523),#20524,.F.);
#21644=ADVANCED_FACE('',(#3524),#20525,.F.);
#21645=ADVANCED_FACE('',(#3525),#20526,.F.);
#21646=ADVANCED_FACE('',(#3526),#20527,.F.);
#21647=ADVANCED_FACE('',(#3527),#20528,.F.);
#21648=ADVANCED_FACE('',(#3528),#20529,.F.);
#21649=ADVANCED_FACE('',(#3529),#20530,.F.);
#21650=ADVANCED_FACE('',(#3530),#20531,.F.);
#21651=ADVANCED_FACE('',(#3531),#20532,.F.);
#21652=ADVANCED_FACE('',(#3532),#20533,.F.);
#21653=ADVANCED_FACE('',(#3533),#20534,.F.);
#21654=ADVANCED_FACE('',(#3534),#20535,.F.);
#21655=ADVANCED_FACE('',(#3535),#20536,.F.);
#21656=ADVANCED_FACE('',(#3536),#20537,.F.);
#21657=ADVANCED_FACE('',(#3537),#20538,.F.);
#21658=ADVANCED_FACE('',(#3538),#20539,.F.);
#21659=ADVANCED_FACE('',(#3539),#20540,.F.);
#21660=ADVANCED_FACE('',(#3540),#362,.F.);
#21661=ADVANCED_FACE('',(#3541),#363,.F.);
#21662=ADVANCED_FACE('',(#3542,#2361,#2362,#2363,#2364,#2365,#2366),#2517,
 .T.);
#21663=ADVANCED_FACE('',(#3543),#20541,.F.);
#21664=ADVANCED_FACE('',(#3544),#364,.F.);
#21665=ADVANCED_FACE('',(#3545),#365,.F.);
#21666=ADVANCED_FACE('',(#3546),#20542,.F.);
#21667=ADVANCED_FACE('',(#3547),#366,.F.);
#21668=ADVANCED_FACE('',(#3548),#367,.F.);
#21669=ADVANCED_FACE('',(#3549),#20543,.F.);
#21670=ADVANCED_FACE('',(#3550),#368,.F.);
#21671=ADVANCED_FACE('',(#3551),#369,.F.);
#21672=ADVANCED_FACE('',(#3552),#20544,.F.);
#21673=ADVANCED_FACE('',(#3553),#370,.F.);
#21674=ADVANCED_FACE('',(#3554),#371,.F.);
#21675=ADVANCED_FACE('',(#3555),#20545,.F.);
#21676=ADVANCED_FACE('',(#3556),#372,.F.);
#21677=ADVANCED_FACE('',(#3557),#373,.F.);
#21678=ADVANCED_FACE('',(#3558),#20546,.F.);
#21679=ADVANCED_FACE('',(#3559),#20547,.F.);
#21680=ADVANCED_FACE('',(#3560),#20548,.F.);
#21681=ADVANCED_FACE('',(#3561),#20549,.F.);
#21682=ADVANCED_FACE('',(#3562),#20550,.F.);
#21683=ADVANCED_FACE('',(#3563),#20551,.F.);
#21684=ADVANCED_FACE('',(#3564),#2518,.T.);
#21685=ADVANCED_FACE('',(#3565),#2519,.T.);
#21686=ADVANCED_FACE('',(#3566),#2520,.T.);
#21687=ADVANCED_FACE('',(#3567),#2521,.T.);
#21688=ADVANCED_FACE('',(#3568,#2367,#2368,#2369,#2370,#2371,#2372),#2522,
 .F.);
#21826=CLOSED_SHELL('',(#21419,#21420,#21421,#21422,#21423,#21424,#21425,
#21426,#21427,#21428,#21429,#21430,#21431,#21432,#21433,#21434,#21435,#21436,
#21437,#21438,#21439,#21440,#21441,#21442,#21443,#21444,#21445,#21446,#21447,
#21448,#21449,#21450,#21451,#21452,#21453,#21454,#21455,#21456,#21457,#21458,
#21459,#21460,#21461,#21462,#21463,#21464,#21465,#21466,#21467,#21468,#21469,
#21470,#21471,#21472,#21473,#21474,#21475,#21476,#21477,#21478,#21479,#21480,
#21481,#21482,#21483,#21484,#21485,#21486,#21487,#21488,#21489,#21490,#21491,
#21492,#21493,#21494,#21495,#21496,#21497,#21498,#21499,#21500,#21501,#21502,
#21503,#21504,#21505,#21506,#21507,#21508,#21509,#21510,#21511,#21512,#21513,
#21514,#21515,#21516,#21517,#21518,#21519,#21520,#21521,#21522,#21523,#21524,
#21525,#21526,#21527,#21528,#21529,#21530,#21531,#21532,#21533,#21534,#21535,
#21536,#21537,#21538,#21539,#21540,#21541,#21542,#21543,#21544,#21545,#21546,
#21547,#21548,#21549,#21550,#21551,#21552,#21553,#21554,#21555,#21556,#21557,
#21558,#21559,#21560,#21561,#21562,#21563,#21564,#21565,#21566,#21567,#21568,
#21569,#21570,#21571,#21572,#21573,#21574,#21575,#21576,#21577,#21578,#21579,
#21580,#21581,#21582,#21583,#21584,#21585,#21586,#21587,#21588,#21589,#21590,
#21591,#21592,#21593,#21594,#21595,#21596,#21597,#21598,#21599,#21600,#21601,
#21602,#21603,#21604,#21605,#21606,#21607,#21608,#21609,#21610,#21611,#21612,
#21613,#21614,#21615,#21616,#21617,#21618,#21619,#21620,#21621,#21622,#21623,
#21624,#21625,#21626,#21627,#21628,#21629,#21630,#21631,#21632,#21633,#21634,
#21635,#21636,#21637,#21638,#21639,#21640,#21641,#21642,#21643,#21644,#21645,
#21646,#21647,#21648,#21649,#21650,#21651,#21652,#21653,#21654,#21655,#21656,
#21657,#21658,#21659,#21660,#21661,#21662,#21663,#21664,#21665,#21666,#21667,
#21668,#21669,#21670,#21671,#21672,#21673,#21674,#21675,#21676,#21677,#21678,
#21679,#21680,#21681,#21682,#21683,#21684,#21685,#21686,#21687,#21688));
#23042=AXIS2_PLACEMENT_3D('',#72980,#26346,#26347);
#23043=AXIS2_PLACEMENT_3D('',#72981,#26348,#26349);
#23044=AXIS2_PLACEMENT_3D('',#72991,#26351,#26352);
#23045=AXIS2_PLACEMENT_3D('',#73002,#26353,#26354);
#23046=AXIS2_PLACEMENT_3D('',#73053,#26356,#26357);
#23047=AXIS2_PLACEMENT_3D('',#73104,#26359,#26360);
#23048=AXIS2_PLACEMENT_3D('',#73152,#26362,#26363);
#23049=AXIS2_PLACEMENT_3D('',#73200,#26365,#26366);
#23050=AXIS2_PLACEMENT_3D('',#73251,#26368,#26369);
#23051=AXIS2_PLACEMENT_3D('',#73302,#26371,#26372);
#23052=AXIS2_PLACEMENT_3D('',#73350,#26374,#26375);
#23053=AXIS2_PLACEMENT_3D('',#73401,#26377,#26378);
#23054=AXIS2_PLACEMENT_3D('',#73452,#26380,#26381);
#23055=AXIS2_PLACEMENT_3D('',#73500,#26383,#26384);
#23056=AXIS2_PLACEMENT_3D('',#73548,#26386,#26387);
#23057=AXIS2_PLACEMENT_3D('',#73602,#26389,#26390);
#23058=AXIS2_PLACEMENT_3D('',#73650,#26392,#26393);
#23059=AXIS2_PLACEMENT_3D('',#73698,#26395,#26396);
#23060=AXIS2_PLACEMENT_3D('',#73749,#26398,#26399);
#23061=AXIS2_PLACEMENT_3D('',#73800,#26401,#26402);
#23062=AXIS2_PLACEMENT_3D('',#73848,#26404,#26405);
#23063=AXIS2_PLACEMENT_3D('',#73899,#26407,#26408);
#23064=AXIS2_PLACEMENT_3D('',#73918,#26410,#26411);
#23065=AXIS2_PLACEMENT_3D('',#73938,#26412,#26413);
#23066=AXIS2_PLACEMENT_3D('',#73948,#26415,#26416);
#23067=AXIS2_PLACEMENT_3D('',#73959,#26417,#26418);
#23068=AXIS2_PLACEMENT_3D('',#74010,#26420,#26421);
#23069=AXIS2_PLACEMENT_3D('',#74061,#26423,#26424);
#23070=AXIS2_PLACEMENT_3D('',#74109,#26426,#26427);
#23071=AXIS2_PLACEMENT_3D('',#74157,#26429,#26430);
#23072=AXIS2_PLACEMENT_3D('',#74208,#26432,#26433);
#23073=AXIS2_PLACEMENT_3D('',#74259,#26435,#26436);
#23074=AXIS2_PLACEMENT_3D('',#74307,#26438,#26439);
#23075=AXIS2_PLACEMENT_3D('',#74358,#26441,#26442);
#23076=AXIS2_PLACEMENT_3D('',#74409,#26444,#26445);
#23077=AXIS2_PLACEMENT_3D('',#74457,#26447,#26448);
#23078=AXIS2_PLACEMENT_3D('',#74505,#26450,#26451);
#23079=AXIS2_PLACEMENT_3D('',#74559,#26453,#26454);
#23080=AXIS2_PLACEMENT_3D('',#74607,#26456,#26457);
#23081=AXIS2_PLACEMENT_3D('',#74655,#26459,#26460);
#23082=AXIS2_PLACEMENT_3D('',#74706,#26462,#26463);
#23083=AXIS2_PLACEMENT_3D('',#74757,#26465,#26466);
#23084=AXIS2_PLACEMENT_3D('',#74805,#26468,#26469);
#23085=AXIS2_PLACEMENT_3D('',#74856,#26471,#26472);
#23086=AXIS2_PLACEMENT_3D('',#74875,#26474,#26475);
#23087=AXIS2_PLACEMENT_3D('',#74895,#26476,#26477);
#23088=AXIS2_PLACEMENT_3D('',#74905,#26479,#26480);
#23089=AXIS2_PLACEMENT_3D('',#74916,#26481,#26482);
#23090=AXIS2_PLACEMENT_3D('',#74967,#26484,#26485);
#23091=AXIS2_PLACEMENT_3D('',#75018,#26487,#26488);
#23092=AXIS2_PLACEMENT_3D('',#75066,#26490,#26491);
#23093=AXIS2_PLACEMENT_3D('',#75114,#26493,#26494);
#23094=AXIS2_PLACEMENT_3D('',#75165,#26496,#26497);
#23095=AXIS2_PLACEMENT_3D('',#75216,#26499,#26500);
#23096=AXIS2_PLACEMENT_3D('',#75264,#26502,#26503);
#23097=AXIS2_PLACEMENT_3D('',#75315,#26505,#26506);
#23098=AXIS2_PLACEMENT_3D('',#75366,#26508,#26509);
#23099=AXIS2_PLACEMENT_3D('',#75414,#26511,#26512);
#23100=AXIS2_PLACEMENT_3D('',#75462,#26514,#26515);
#23101=AXIS2_PLACEMENT_3D('',#75516,#26517,#26518);
#23102=AXIS2_PLACEMENT_3D('',#75564,#26520,#26521);
#23103=AXIS2_PLACEMENT_3D('',#75612,#26523,#26524);
#23104=AXIS2_PLACEMENT_3D('',#75663,#26526,#26527);
#23105=AXIS2_PLACEMENT_3D('',#75714,#26529,#26530);
#23106=AXIS2_PLACEMENT_3D('',#75762,#26532,#26533);
#23107=AXIS2_PLACEMENT_3D('',#75813,#26535,#26536);
#23108=AXIS2_PLACEMENT_3D('',#75832,#26538,#26539);
#23109=AXIS2_PLACEMENT_3D('',#75852,#26540,#26541);
#23110=AXIS2_PLACEMENT_3D('',#75862,#26543,#26544);
#23111=AXIS2_PLACEMENT_3D('',#75873,#26545,#26546);
#23112=AXIS2_PLACEMENT_3D('',#75924,#26548,#26549);
#23113=AXIS2_PLACEMENT_3D('',#75975,#26551,#26552);
#23114=AXIS2_PLACEMENT_3D('',#76023,#26554,#26555);
#23115=AXIS2_PLACEMENT_3D('',#76071,#26557,#26558);
#23116=AXIS2_PLACEMENT_3D('',#76122,#26560,#26561);
#23117=AXIS2_PLACEMENT_3D('',#76173,#26563,#26564);
#23118=AXIS2_PLACEMENT_3D('',#76221,#26566,#26567);
#23119=AXIS2_PLACEMENT_3D('',#76272,#26569,#26570);
#23120=AXIS2_PLACEMENT_3D('',#76323,#26572,#26573);
#23121=AXIS2_PLACEMENT_3D('',#76371,#26575,#26576);
#23122=AXIS2_PLACEMENT_3D('',#76419,#26578,#26579);
#23123=AXIS2_PLACEMENT_3D('',#76473,#26581,#26582);
#23124=AXIS2_PLACEMENT_3D('',#76521,#26584,#26585);
#23125=AXIS2_PLACEMENT_3D('',#76569,#26587,#26588);
#23126=AXIS2_PLACEMENT_3D('',#76620,#26590,#26591);
#23127=AXIS2_PLACEMENT_3D('',#76671,#26593,#26594);
#23128=AXIS2_PLACEMENT_3D('',#76719,#26596,#26597);
#23129=AXIS2_PLACEMENT_3D('',#76770,#26599,#26600);
#23130=AXIS2_PLACEMENT_3D('',#76789,#26602,#26603);
#23131=AXIS2_PLACEMENT_3D('',#76809,#26604,#26605);
#23132=AXIS2_PLACEMENT_3D('',#76819,#26607,#26608);
#23133=AXIS2_PLACEMENT_3D('',#76830,#26609,#26610);
#23134=AXIS2_PLACEMENT_3D('',#76881,#26612,#26613);
#23135=AXIS2_PLACEMENT_3D('',#76932,#26615,#26616);
#23136=AXIS2_PLACEMENT_3D('',#76980,#26618,#26619);
#23137=AXIS2_PLACEMENT_3D('',#77028,#26621,#26622);
#23138=AXIS2_PLACEMENT_3D('',#77079,#26624,#26625);
#23139=AXIS2_PLACEMENT_3D('',#77130,#26627,#26628);
#23140=AXIS2_PLACEMENT_3D('',#77178,#26630,#26631);
#23141=AXIS2_PLACEMENT_3D('',#77229,#26633,#26634);
#23142=AXIS2_PLACEMENT_3D('',#77280,#26636,#26637);
#23143=AXIS2_PLACEMENT_3D('',#77328,#26639,#26640);
#23144=AXIS2_PLACEMENT_3D('',#77376,#26642,#26643);
#23145=AXIS2_PLACEMENT_3D('',#77430,#26645,#26646);
#23146=AXIS2_PLACEMENT_3D('',#77478,#26648,#26649);
#23147=AXIS2_PLACEMENT_3D('',#77526,#26651,#26652);
#23148=AXIS2_PLACEMENT_3D('',#77577,#26654,#26655);
#23149=AXIS2_PLACEMENT_3D('',#77628,#26657,#26658);
#23150=AXIS2_PLACEMENT_3D('',#77676,#26660,#26661);
#23151=AXIS2_PLACEMENT_3D('',#77727,#26663,#26664);
#23152=AXIS2_PLACEMENT_3D('',#77746,#26666,#26667);
#23153=AXIS2_PLACEMENT_3D('',#77766,#26668,#26669);
#23154=AXIS2_PLACEMENT_3D('',#77776,#26671,#26672);
#23155=AXIS2_PLACEMENT_3D('',#77787,#26673,#26674);
#23156=AXIS2_PLACEMENT_3D('',#77838,#26676,#26677);
#23157=AXIS2_PLACEMENT_3D('',#77889,#26679,#26680);
#23158=AXIS2_PLACEMENT_3D('',#77937,#26682,#26683);
#23159=AXIS2_PLACEMENT_3D('',#77985,#26685,#26686);
#23160=AXIS2_PLACEMENT_3D('',#78036,#26688,#26689);
#23161=AXIS2_PLACEMENT_3D('',#78087,#26691,#26692);
#23162=AXIS2_PLACEMENT_3D('',#78135,#26694,#26695);
#23163=AXIS2_PLACEMENT_3D('',#78186,#26697,#26698);
#23164=AXIS2_PLACEMENT_3D('',#78237,#26700,#26701);
#23165=AXIS2_PLACEMENT_3D('',#78285,#26703,#26704);
#23166=AXIS2_PLACEMENT_3D('',#78333,#26706,#26707);
#23167=AXIS2_PLACEMENT_3D('',#78387,#26709,#26710);
#23168=AXIS2_PLACEMENT_3D('',#78435,#26712,#26713);
#23169=AXIS2_PLACEMENT_3D('',#78483,#26715,#26716);
#23170=AXIS2_PLACEMENT_3D('',#78534,#26718,#26719);
#23171=AXIS2_PLACEMENT_3D('',#78585,#26721,#26722);
#23172=AXIS2_PLACEMENT_3D('',#78633,#26724,#26725);
#23173=AXIS2_PLACEMENT_3D('',#78684,#26727,#26728);
#23174=AXIS2_PLACEMENT_3D('',#78703,#26730,#26731);
#23175=AXIS2_PLACEMENT_3D('',#78723,#26732,#26733);
#23176=AXIS2_PLACEMENT_3D('',#78737,#26735,#26736);
#23177=AXIS2_PLACEMENT_3D('',#78747,#26737,#26738);
#23178=AXIS2_PLACEMENT_3D('',#78771,#26740,#26741);
#23179=AXIS2_PLACEMENT_3D('',#78796,#26743,#26744);
#23180=AXIS2_PLACEMENT_3D('',#78820,#26746,#26747);
#23181=AXIS2_PLACEMENT_3D('',#78845,#26749,#26750);
#23182=AXIS2_PLACEMENT_3D('',#78869,#26752,#26753);
#23183=AXIS2_PLACEMENT_3D('',#78894,#26755,#26756);
#23184=AXIS2_PLACEMENT_3D('',#78919,#26758,#26759);
#23185=AXIS2_PLACEMENT_3D('',#78943,#26761,#26762);
#23186=AXIS2_PLACEMENT_3D('',#78968,#26764,#26765);
#23187=AXIS2_PLACEMENT_3D('',#78992,#26767,#26768);
#23188=AXIS2_PLACEMENT_3D('',#79017,#26770,#26771);
#23189=AXIS2_PLACEMENT_3D('',#79042,#26773,#26774);
#23190=AXIS2_PLACEMENT_3D('',#79066,#26776,#26777);
#23191=AXIS2_PLACEMENT_3D('',#79091,#26779,#26780);
#23192=AXIS2_PLACEMENT_3D('',#79115,#26782,#26783);
#23193=AXIS2_PLACEMENT_3D('',#79140,#26785,#26786);
#23194=AXIS2_PLACEMENT_3D('',#79165,#26788,#26789);
#23195=AXIS2_PLACEMENT_3D('',#79189,#26791,#26792);
#23196=AXIS2_PLACEMENT_3D('',#79200,#26794,#26795);
#23197=AXIS2_PLACEMENT_3D('',#79206,#26796,#26797);
#23198=AXIS2_PLACEMENT_3D('',#79220,#26799,#26800);
#23199=AXIS2_PLACEMENT_3D('',#79230,#26801,#26802);
#23200=AXIS2_PLACEMENT_3D('',#79254,#26804,#26805);
#23201=AXIS2_PLACEMENT_3D('',#79279,#26807,#26808);
#23202=AXIS2_PLACEMENT_3D('',#79303,#26810,#26811);
#23203=AXIS2_PLACEMENT_3D('',#79328,#26813,#26814);
#23204=AXIS2_PLACEMENT_3D('',#79352,#26816,#26817);
#23205=AXIS2_PLACEMENT_3D('',#79377,#26819,#26820);
#23206=AXIS2_PLACEMENT_3D('',#79402,#26822,#26823);
#23207=AXIS2_PLACEMENT_3D('',#79426,#26825,#26826);
#23208=AXIS2_PLACEMENT_3D('',#79451,#26828,#26829);
#23209=AXIS2_PLACEMENT_3D('',#79475,#26831,#26832);
#23210=AXIS2_PLACEMENT_3D('',#79500,#26834,#26835);
#23211=AXIS2_PLACEMENT_3D('',#79525,#26837,#26838);
#23212=AXIS2_PLACEMENT_3D('',#79549,#26840,#26841);
#23213=AXIS2_PLACEMENT_3D('',#79574,#26843,#26844);
#23214=AXIS2_PLACEMENT_3D('',#79598,#26846,#26847);
#23215=AXIS2_PLACEMENT_3D('',#79623,#26849,#26850);
#23216=AXIS2_PLACEMENT_3D('',#79648,#26852,#26853);
#23217=AXIS2_PLACEMENT_3D('',#79672,#26855,#26856);
#23218=AXIS2_PLACEMENT_3D('',#79683,#26858,#26859);
#23219=AXIS2_PLACEMENT_3D('',#79689,#26860,#26861);
#23220=AXIS2_PLACEMENT_3D('',#79703,#26863,#26864);
#23221=AXIS2_PLACEMENT_3D('',#79713,#26865,#26866);
#23222=AXIS2_PLACEMENT_3D('',#79737,#26868,#26869);
#23223=AXIS2_PLACEMENT_3D('',#79762,#26871,#26872);
#23224=AXIS2_PLACEMENT_3D('',#79786,#26874,#26875);
#23225=AXIS2_PLACEMENT_3D('',#79811,#26877,#26878);
#23226=AXIS2_PLACEMENT_3D('',#79835,#26880,#26881);
#23227=AXIS2_PLACEMENT_3D('',#79860,#26883,#26884);
#23228=AXIS2_PLACEMENT_3D('',#79885,#26886,#26887);
#23229=AXIS2_PLACEMENT_3D('',#79909,#26889,#26890);
#23230=AXIS2_PLACEMENT_3D('',#79934,#26892,#26893);
#23231=AXIS2_PLACEMENT_3D('',#79958,#26895,#26896);
#23232=AXIS2_PLACEMENT_3D('',#79983,#26898,#26899);
#23233=AXIS2_PLACEMENT_3D('',#80008,#26901,#26902);
#23234=AXIS2_PLACEMENT_3D('',#80032,#26904,#26905);
#23235=AXIS2_PLACEMENT_3D('',#80057,#26907,#26908);
#23236=AXIS2_PLACEMENT_3D('',#80081,#26910,#26911);
#23237=AXIS2_PLACEMENT_3D('',#80106,#26913,#26914);
#23238=AXIS2_PLACEMENT_3D('',#80131,#26916,#26917);
#23239=AXIS2_PLACEMENT_3D('',#80155,#26919,#26920);
#23240=AXIS2_PLACEMENT_3D('',#80166,#26922,#26923);
#23241=AXIS2_PLACEMENT_3D('',#80172,#26924,#26925);
#23242=AXIS2_PLACEMENT_3D('',#80186,#26927,#26928);
#23243=AXIS2_PLACEMENT_3D('',#80196,#26929,#26930);
#23244=AXIS2_PLACEMENT_3D('',#80220,#26932,#26933);
#23245=AXIS2_PLACEMENT_3D('',#80245,#26935,#26936);
#23246=AXIS2_PLACEMENT_3D('',#80269,#26938,#26939);
#23247=AXIS2_PLACEMENT_3D('',#80294,#26941,#26942);
#23248=AXIS2_PLACEMENT_3D('',#80318,#26944,#26945);
#23249=AXIS2_PLACEMENT_3D('',#80343,#26947,#26948);
#23250=AXIS2_PLACEMENT_3D('',#80368,#26950,#26951);
#23251=AXIS2_PLACEMENT_3D('',#80392,#26953,#26954);
#23252=AXIS2_PLACEMENT_3D('',#80417,#26956,#26957);
#23253=AXIS2_PLACEMENT_3D('',#80441,#26959,#26960);
#23254=AXIS2_PLACEMENT_3D('',#80466,#26962,#26963);
#23255=AXIS2_PLACEMENT_3D('',#80491,#26965,#26966);
#23256=AXIS2_PLACEMENT_3D('',#80515,#26968,#26969);
#23257=AXIS2_PLACEMENT_3D('',#80540,#26971,#26972);
#23258=AXIS2_PLACEMENT_3D('',#80564,#26974,#26975);
#23259=AXIS2_PLACEMENT_3D('',#80589,#26977,#26978);
#23260=AXIS2_PLACEMENT_3D('',#80614,#26980,#26981);
#23261=AXIS2_PLACEMENT_3D('',#80638,#26983,#26984);
#23262=AXIS2_PLACEMENT_3D('',#80649,#26986,#26987);
#23263=AXIS2_PLACEMENT_3D('',#80655,#26988,#26989);
#23264=AXIS2_PLACEMENT_3D('',#80669,#26991,#26992);
#23265=AXIS2_PLACEMENT_3D('',#80679,#26993,#26994);
#23266=AXIS2_PLACEMENT_3D('',#80703,#26996,#26997);
#23267=AXIS2_PLACEMENT_3D('',#80728,#26999,#27000);
#23268=AXIS2_PLACEMENT_3D('',#80752,#27002,#27003);
#23269=AXIS2_PLACEMENT_3D('',#80777,#27005,#27006);
#23270=AXIS2_PLACEMENT_3D('',#80801,#27008,#27009);
#23271=AXIS2_PLACEMENT_3D('',#80826,#27011,#27012);
#23272=AXIS2_PLACEMENT_3D('',#80851,#27014,#27015);
#23273=AXIS2_PLACEMENT_3D('',#80875,#27017,#27018);
#23274=AXIS2_PLACEMENT_3D('',#80900,#27020,#27021);
#23275=AXIS2_PLACEMENT_3D('',#80924,#27023,#27024);
#23276=AXIS2_PLACEMENT_3D('',#80949,#27026,#27027);
#23277=AXIS2_PLACEMENT_3D('',#80974,#27029,#27030);
#23278=AXIS2_PLACEMENT_3D('',#80998,#27032,#27033);
#23279=AXIS2_PLACEMENT_3D('',#81023,#27035,#27036);
#23280=AXIS2_PLACEMENT_3D('',#81047,#27038,#27039);
#23281=AXIS2_PLACEMENT_3D('',#81072,#27041,#27042);
#23282=AXIS2_PLACEMENT_3D('',#81097,#27044,#27045);
#23283=AXIS2_PLACEMENT_3D('',#81121,#27047,#27048);
#23284=AXIS2_PLACEMENT_3D('',#81132,#27050,#27051);
#23285=AXIS2_PLACEMENT_3D('',#81138,#27052,#27053);
#23286=AXIS2_PLACEMENT_3D('',#81152,#27055,#27056);
#23287=AXIS2_PLACEMENT_3D('',#81162,#27057,#27058);
#23288=AXIS2_PLACEMENT_3D('',#81186,#27060,#27061);
#23289=AXIS2_PLACEMENT_3D('',#81211,#27063,#27064);
#23290=AXIS2_PLACEMENT_3D('',#81235,#27066,#27067);
#23291=AXIS2_PLACEMENT_3D('',#81260,#27069,#27070);
#23292=AXIS2_PLACEMENT_3D('',#81284,#27072,#27073);
#23293=AXIS2_PLACEMENT_3D('',#81309,#27075,#27076);
#23294=AXIS2_PLACEMENT_3D('',#81334,#27078,#27079);
#23295=AXIS2_PLACEMENT_3D('',#81358,#27081,#27082);
#23296=AXIS2_PLACEMENT_3D('',#81383,#27084,#27085);
#23297=AXIS2_PLACEMENT_3D('',#81407,#27087,#27088);
#23298=AXIS2_PLACEMENT_3D('',#81432,#27090,#27091);
#23299=AXIS2_PLACEMENT_3D('',#81457,#27093,#27094);
#23300=AXIS2_PLACEMENT_3D('',#81481,#27096,#27097);
#23301=AXIS2_PLACEMENT_3D('',#81506,#27099,#27100);
#23302=AXIS2_PLACEMENT_3D('',#81530,#27102,#27103);
#23303=AXIS2_PLACEMENT_3D('',#81555,#27105,#27106);
#23304=AXIS2_PLACEMENT_3D('',#81580,#27108,#27109);
#23305=AXIS2_PLACEMENT_3D('',#81604,#27111,#27112);
#23306=AXIS2_PLACEMENT_3D('',#81615,#27114,#27115);
#23307=AXIS2_PLACEMENT_3D('',#81621,#27116,#27117);
#23308=AXIS2_PLACEMENT_3D('',#83114,#27118,#27119);
#23309=AXIS2_PLACEMENT_3D('',#84063,#27124,#27125);
#23310=AXIS2_PLACEMENT_3D('',#85368,#27126,#27127);
#23311=AXIS2_PLACEMENT_3D('',#86673,#27128,#27129);
#23312=AXIS2_PLACEMENT_3D('',#87978,#27130,#27131);
#23313=AXIS2_PLACEMENT_3D('',#89283,#27132,#27133);
#23314=AXIS2_PLACEMENT_3D('',#90588,#27134,#27135);
#23315=AXIS2_PLACEMENT_3D('',#90589,#27136,#27137);
#23316=AXIS2_PLACEMENT_3D('',#90590,#27138,#27139);
#23317=AXIS2_PLACEMENT_3D('',#90591,#27140,#27141);
#23318=AXIS2_PLACEMENT_3D('',#90592,#27142,#27143);
#23319=AXIS2_PLACEMENT_3D('',#90593,#27144,#27145);
#23320=AXIS2_PLACEMENT_3D('',#90594,#27146,#27147);
#23321=AXIS2_PLACEMENT_3D('',#90600,#27151,#27152);
#23322=AXIS2_PLACEMENT_3D('',#90604,#27155,#27156);
#23323=AXIS2_PLACEMENT_3D('',#90608,#27159,#27160);
#23324=AXIS2_PLACEMENT_3D('',#90610,#27162,#27163);
#26346=DIRECTION('axis',(0.,0.,1.));
#26347=DIRECTION('refdir',(1.,0.,0.));
#26348=DIRECTION('center_axis',(0.,0.,-1.));
#26349=DIRECTION('ref_axis',(-0.347005528821294,0.937863083273595,0.));
#26350=DIRECTION('',(0.,0.,-1.));
#26351=DIRECTION('center_axis',(0.,0.,-1.));
#26352=DIRECTION('ref_axis',(1.,0.,0.));
#26353=DIRECTION('center_axis',(0.,0.,-1.));
#26354=DIRECTION('ref_axis',(1.,0.,0.));
#26355=DIRECTION('',(0.,0.,-1.));
#26356=DIRECTION('center_axis',(0.,0.,-1.));
#26357=DIRECTION('ref_axis',(1.,0.,0.));
#26358=DIRECTION('',(0.,0.,-1.));
#26359=DIRECTION('center_axis',(0.,0.,-1.));
#26360=DIRECTION('ref_axis',(1.,0.,0.));
#26361=DIRECTION('',(0.,0.,-1.));
#26362=DIRECTION('center_axis',(0.,0.,-1.));
#26363=DIRECTION('ref_axis',(1.,0.,0.));
#26364=DIRECTION('',(0.,0.,-1.));
#26365=DIRECTION('center_axis',(0.,0.,-1.));
#26366=DIRECTION('ref_axis',(1.,0.,0.));
#26367=DIRECTION('',(0.,0.,-1.));
#26368=DIRECTION('center_axis',(0.,0.,-1.));
#26369=DIRECTION('ref_axis',(1.,0.,0.));
#26370=DIRECTION('',(0.,0.,-1.));
#26371=DIRECTION('center_axis',(0.,0.,-1.));
#26372=DIRECTION('ref_axis',(1.,0.,0.));
#26373=DIRECTION('',(0.,0.,-1.));
#26374=DIRECTION('center_axis',(0.,0.,-1.));
#26375=DIRECTION('ref_axis',(1.,0.,0.));
#26376=DIRECTION('',(0.,0.,-1.));
#26377=DIRECTION('center_axis',(0.,0.,-1.));
#26378=DIRECTION('ref_axis',(1.,0.,0.));
#26379=DIRECTION('',(0.,0.,-1.));
#26380=DIRECTION('center_axis',(0.,0.,-1.));
#26381=DIRECTION('ref_axis',(1.,0.,0.));
#26382=DIRECTION('',(0.,0.,-1.));
#26383=DIRECTION('center_axis',(0.,0.,-1.));
#26384=DIRECTION('ref_axis',(1.,0.,0.));
#26385=DIRECTION('',(0.,0.,-1.));
#26386=DIRECTION('center_axis',(0.,0.,-1.));
#26387=DIRECTION('ref_axis',(1.,0.,0.));
#26388=DIRECTION('',(0.,0.,-1.));
#26389=DIRECTION('center_axis',(0.,0.,-1.));
#26390=DIRECTION('ref_axis',(1.,0.,0.));
#26391=DIRECTION('',(0.,0.,-1.));
#26392=DIRECTION('center_axis',(0.,0.,-1.));
#26393=DIRECTION('ref_axis',(1.,0.,0.));
#26394=DIRECTION('',(0.,0.,-1.));
#26395=DIRECTION('center_axis',(0.,0.,-1.));
#26396=DIRECTION('ref_axis',(1.,0.,0.));
#26397=DIRECTION('',(0.,0.,-1.));
#26398=DIRECTION('center_axis',(0.,0.,-1.));
#26399=DIRECTION('ref_axis',(1.,0.,0.));
#26400=DIRECTION('',(0.,0.,-1.));
#26401=DIRECTION('center_axis',(0.,0.,-1.));
#26402=DIRECTION('ref_axis',(1.,0.,0.));
#26403=DIRECTION('',(0.,0.,-1.));
#26404=DIRECTION('center_axis',(0.,0.,-1.));
#26405=DIRECTION('ref_axis',(1.,0.,0.));
#26406=DIRECTION('',(0.,0.,-1.));
#26407=DIRECTION('center_axis',(0.,0.,-1.));
#26408=DIRECTION('ref_axis',(0.937995430874257,-0.346647618856695,0.));
#26409=DIRECTION('',(0.,0.,-1.));
#26410=DIRECTION('center_axis',(0.,0.,-1.));
#26411=DIRECTION('ref_axis',(1.,0.,0.));
#26412=DIRECTION('center_axis',(0.,0.,-1.));
#26413=DIRECTION('ref_axis',(-0.347005563593634,0.93786307040797,0.));
#26414=DIRECTION('',(0.,0.,-1.));
#26415=DIRECTION('center_axis',(0.,0.,-1.));
#26416=DIRECTION('ref_axis',(1.,0.,0.));
#26417=DIRECTION('center_axis',(0.,0.,-1.));
#26418=DIRECTION('ref_axis',(1.,0.,0.));
#26419=DIRECTION('',(0.,0.,-1.));
#26420=DIRECTION('center_axis',(0.,0.,-1.));
#26421=DIRECTION('ref_axis',(1.,0.,0.));
#26422=DIRECTION('',(0.,0.,-1.));
#26423=DIRECTION('center_axis',(0.,0.,-1.));
#26424=DIRECTION('ref_axis',(1.,0.,0.));
#26425=DIRECTION('',(0.,0.,-1.));
#26426=DIRECTION('center_axis',(0.,0.,-1.));
#26427=DIRECTION('ref_axis',(1.,0.,0.));
#26428=DIRECTION('',(0.,0.,-1.));
#26429=DIRECTION('center_axis',(0.,0.,-1.));
#26430=DIRECTION('ref_axis',(1.,0.,0.));
#26431=DIRECTION('',(0.,0.,-1.));
#26432=DIRECTION('center_axis',(0.,0.,-1.));
#26433=DIRECTION('ref_axis',(1.,0.,0.));
#26434=DIRECTION('',(0.,0.,-1.));
#26435=DIRECTION('center_axis',(0.,0.,-1.));
#26436=DIRECTION('ref_axis',(1.,0.,0.));
#26437=DIRECTION('',(0.,0.,-1.));
#26438=DIRECTION('center_axis',(0.,0.,-1.));
#26439=DIRECTION('ref_axis',(1.,0.,0.));
#26440=DIRECTION('',(0.,0.,-1.));
#26441=DIRECTION('center_axis',(0.,0.,-1.));
#26442=DIRECTION('ref_axis',(1.,0.,0.));
#26443=DIRECTION('',(0.,0.,-1.));
#26444=DIRECTION('center_axis',(0.,0.,-1.));
#26445=DIRECTION('ref_axis',(1.,0.,0.));
#26446=DIRECTION('',(0.,0.,-1.));
#26447=DIRECTION('center_axis',(0.,0.,-1.));
#26448=DIRECTION('ref_axis',(1.,0.,0.));
#26449=DIRECTION('',(0.,0.,-1.));
#26450=DIRECTION('center_axis',(0.,0.,-1.));
#26451=DIRECTION('ref_axis',(1.,0.,0.));
#26452=DIRECTION('',(0.,0.,-1.));
#26453=DIRECTION('center_axis',(0.,0.,-1.));
#26454=DIRECTION('ref_axis',(1.,0.,0.));
#26455=DIRECTION('',(0.,0.,-1.));
#26456=DIRECTION('center_axis',(0.,0.,-1.));
#26457=DIRECTION('ref_axis',(1.,0.,0.));
#26458=DIRECTION('',(0.,0.,-1.));
#26459=DIRECTION('center_axis',(0.,0.,-1.));
#26460=DIRECTION('ref_axis',(1.,0.,0.));
#26461=DIRECTION('',(0.,0.,-1.));
#26462=DIRECTION('center_axis',(0.,0.,-1.));
#26463=DIRECTION('ref_axis',(1.,0.,0.));
#26464=DIRECTION('',(0.,0.,-1.));
#26465=DIRECTION('center_axis',(0.,0.,-1.));
#26466=DIRECTION('ref_axis',(1.,0.,0.));
#26467=DIRECTION('',(0.,0.,-1.));
#26468=DIRECTION('center_axis',(0.,0.,-1.));
#26469=DIRECTION('ref_axis',(1.,0.,0.));
#26470=DIRECTION('',(0.,0.,-1.));
#26471=DIRECTION('center_axis',(0.,0.,-1.));
#26472=DIRECTION('ref_axis',(0.93799543155111,-0.346647617025196,0.));
#26473=DIRECTION('',(0.,0.,-1.));
#26474=DIRECTION('center_axis',(0.,0.,-1.));
#26475=DIRECTION('ref_axis',(1.,0.,0.));
#26476=DIRECTION('center_axis',(0.,0.,-1.));
#26477=DIRECTION('ref_axis',(-0.346979519569086,0.937872706181178,0.));
#26478=DIRECTION('',(0.,0.,-1.));
#26479=DIRECTION('center_axis',(0.,0.,-1.));
#26480=DIRECTION('ref_axis',(1.,0.,0.));
#26481=DIRECTION('center_axis',(0.,0.,-1.));
#26482=DIRECTION('ref_axis',(1.,0.,0.));
#26483=DIRECTION('',(0.,0.,-1.));
#26484=DIRECTION('center_axis',(0.,0.,-1.));
#26485=DIRECTION('ref_axis',(1.,0.,0.));
#26486=DIRECTION('',(0.,0.,-1.));
#26487=DIRECTION('center_axis',(0.,0.,-1.));
#26488=DIRECTION('ref_axis',(1.,0.,0.));
#26489=DIRECTION('',(0.,0.,-1.));
#26490=DIRECTION('center_axis',(0.,0.,-1.));
#26491=DIRECTION('ref_axis',(1.,0.,0.));
#26492=DIRECTION('',(0.,0.,-1.));
#26493=DIRECTION('center_axis',(0.,0.,-1.));
#26494=DIRECTION('ref_axis',(1.,0.,0.));
#26495=DIRECTION('',(0.,0.,-1.));
#26496=DIRECTION('center_axis',(0.,0.,-1.));
#26497=DIRECTION('ref_axis',(1.,0.,0.));
#26498=DIRECTION('',(0.,0.,-1.));
#26499=DIRECTION('center_axis',(0.,0.,-1.));
#26500=DIRECTION('ref_axis',(1.,0.,0.));
#26501=DIRECTION('',(0.,0.,-1.));
#26502=DIRECTION('center_axis',(0.,0.,-1.));
#26503=DIRECTION('ref_axis',(1.,0.,0.));
#26504=DIRECTION('',(0.,0.,-1.));
#26505=DIRECTION('center_axis',(0.,0.,-1.));
#26506=DIRECTION('ref_axis',(1.,0.,0.));
#26507=DIRECTION('',(0.,0.,-1.));
#26508=DIRECTION('center_axis',(0.,0.,-1.));
#26509=DIRECTION('ref_axis',(1.,0.,0.));
#26510=DIRECTION('',(0.,0.,-1.));
#26511=DIRECTION('center_axis',(0.,0.,-1.));
#26512=DIRECTION('ref_axis',(1.,0.,0.));
#26513=DIRECTION('',(0.,0.,-1.));
#26514=DIRECTION('center_axis',(0.,0.,-1.));
#26515=DIRECTION('ref_axis',(1.,0.,0.));
#26516=DIRECTION('',(0.,0.,-1.));
#26517=DIRECTION('center_axis',(0.,0.,-1.));
#26518=DIRECTION('ref_axis',(1.,0.,0.));
#26519=DIRECTION('',(0.,0.,-1.));
#26520=DIRECTION('center_axis',(0.,0.,-1.));
#26521=DIRECTION('ref_axis',(1.,0.,0.));
#26522=DIRECTION('',(0.,0.,-1.));
#26523=DIRECTION('center_axis',(0.,0.,-1.));
#26524=DIRECTION('ref_axis',(1.,0.,0.));
#26525=DIRECTION('',(0.,0.,-1.));
#26526=DIRECTION('center_axis',(0.,0.,-1.));
#26527=DIRECTION('ref_axis',(1.,0.,0.));
#26528=DIRECTION('',(0.,0.,-1.));
#26529=DIRECTION('center_axis',(0.,0.,-1.));
#26530=DIRECTION('ref_axis',(1.,0.,0.));
#26531=DIRECTION('',(0.,0.,-1.));
#26532=DIRECTION('center_axis',(0.,0.,-1.));
#26533=DIRECTION('ref_axis',(1.,0.,0.));
#26534=DIRECTION('',(0.,0.,-1.));
#26535=DIRECTION('center_axis',(0.,0.,-1.));
#26536=DIRECTION('ref_axis',(0.93799553354803,-0.346647341031121,0.));
#26537=DIRECTION('',(0.,0.,-1.));
#26538=DIRECTION('center_axis',(0.,0.,-1.));
#26539=DIRECTION('ref_axis',(1.,0.,0.));
#26540=DIRECTION('center_axis',(0.,0.,-1.));
#26541=DIRECTION('ref_axis',(-0.347005604905985,0.937863055122565,0.));
#26542=DIRECTION('',(0.,0.,-1.));
#26543=DIRECTION('center_axis',(0.,0.,-1.));
#26544=DIRECTION('ref_axis',(1.,0.,0.));
#26545=DIRECTION('center_axis',(0.,0.,-1.));
#26546=DIRECTION('ref_axis',(1.,0.,0.));
#26547=DIRECTION('',(0.,0.,-1.));
#26548=DIRECTION('center_axis',(0.,0.,-1.));
#26549=DIRECTION('ref_axis',(1.,0.,0.));
#26550=DIRECTION('',(0.,0.,-1.));
#26551=DIRECTION('center_axis',(0.,0.,-1.));
#26552=DIRECTION('ref_axis',(1.,0.,0.));
#26553=DIRECTION('',(0.,0.,-1.));
#26554=DIRECTION('center_axis',(0.,0.,-1.));
#26555=DIRECTION('ref_axis',(1.,0.,0.));
#26556=DIRECTION('',(0.,0.,-1.));
#26557=DIRECTION('center_axis',(0.,0.,-1.));
#26558=DIRECTION('ref_axis',(1.,0.,0.));
#26559=DIRECTION('',(0.,0.,-1.));
#26560=DIRECTION('center_axis',(0.,0.,-1.));
#26561=DIRECTION('ref_axis',(1.,0.,0.));
#26562=DIRECTION('',(0.,0.,-1.));
#26563=DIRECTION('center_axis',(0.,0.,-1.));
#26564=DIRECTION('ref_axis',(1.,0.,0.));
#26565=DIRECTION('',(0.,0.,-1.));
#26566=DIRECTION('center_axis',(0.,0.,-1.));
#26567=DIRECTION('ref_axis',(1.,0.,0.));
#26568=DIRECTION('',(0.,0.,-1.));
#26569=DIRECTION('center_axis',(0.,0.,-1.));
#26570=DIRECTION('ref_axis',(1.,0.,0.));
#26571=DIRECTION('',(0.,0.,-1.));
#26572=DIRECTION('center_axis',(0.,0.,-1.));
#26573=DIRECTION('ref_axis',(1.,0.,0.));
#26574=DIRECTION('',(0.,0.,-1.));
#26575=DIRECTION('center_axis',(0.,0.,-1.));
#26576=DIRECTION('ref_axis',(1.,0.,0.));
#26577=DIRECTION('',(0.,0.,-1.));
#26578=DIRECTION('center_axis',(0.,0.,-1.));
#26579=DIRECTION('ref_axis',(1.,0.,0.));
#26580=DIRECTION('',(0.,0.,-1.));
#26581=DIRECTION('center_axis',(0.,0.,-1.));
#26582=DIRECTION('ref_axis',(1.,0.,0.));
#26583=DIRECTION('',(0.,0.,-1.));
#26584=DIRECTION('center_axis',(0.,0.,-1.));
#26585=DIRECTION('ref_axis',(1.,0.,0.));
#26586=DIRECTION('',(0.,0.,-1.));
#26587=DIRECTION('center_axis',(0.,0.,-1.));
#26588=DIRECTION('ref_axis',(1.,0.,0.));
#26589=DIRECTION('',(0.,0.,-1.));
#26590=DIRECTION('center_axis',(0.,0.,-1.));
#26591=DIRECTION('ref_axis',(1.,0.,0.));
#26592=DIRECTION('',(0.,0.,-1.));
#26593=DIRECTION('center_axis',(0.,0.,-1.));
#26594=DIRECTION('ref_axis',(1.,0.,0.));
#26595=DIRECTION('',(0.,0.,-1.));
#26596=DIRECTION('center_axis',(0.,0.,-1.));
#26597=DIRECTION('ref_axis',(1.,0.,0.));
#26598=DIRECTION('',(0.,0.,-1.));
#26599=DIRECTION('center_axis',(0.,0.,-1.));
#26600=DIRECTION('ref_axis',(0.937995429977383,-0.34664762128355,0.));
#26601=DIRECTION('',(0.,0.,-1.));
#26602=DIRECTION('center_axis',(0.,0.,-1.));
#26603=DIRECTION('ref_axis',(1.,0.,0.));
#26604=DIRECTION('center_axis',(0.,0.,-1.));
#26605=DIRECTION('ref_axis',(-0.34700548079112,0.937863101044563,0.));
#26606=DIRECTION('',(0.,0.,-1.));
#26607=DIRECTION('center_axis',(0.,0.,-1.));
#26608=DIRECTION('ref_axis',(1.,0.,0.));
#26609=DIRECTION('center_axis',(0.,0.,-1.));
#26610=DIRECTION('ref_axis',(1.,0.,0.));
#26611=DIRECTION('',(0.,0.,-1.));
#26612=DIRECTION('center_axis',(0.,0.,-1.));
#26613=DIRECTION('ref_axis',(1.,0.,0.));
#26614=DIRECTION('',(0.,0.,-1.));
#26615=DIRECTION('center_axis',(0.,0.,-1.));
#26616=DIRECTION('ref_axis',(1.,0.,0.));
#26617=DIRECTION('',(0.,0.,-1.));
#26618=DIRECTION('center_axis',(0.,0.,-1.));
#26619=DIRECTION('ref_axis',(1.,0.,0.));
#26620=DIRECTION('',(0.,0.,-1.));
#26621=DIRECTION('center_axis',(0.,0.,-1.));
#26622=DIRECTION('ref_axis',(1.,0.,0.));
#26623=DIRECTION('',(0.,0.,-1.));
#26624=DIRECTION('center_axis',(0.,0.,-1.));
#26625=DIRECTION('ref_axis',(1.,0.,0.));
#26626=DIRECTION('',(0.,0.,-1.));
#26627=DIRECTION('center_axis',(0.,0.,-1.));
#26628=DIRECTION('ref_axis',(1.,0.,0.));
#26629=DIRECTION('',(0.,0.,-1.));
#26630=DIRECTION('center_axis',(0.,0.,-1.));
#26631=DIRECTION('ref_axis',(1.,0.,0.));
#26632=DIRECTION('',(0.,0.,-1.));
#26633=DIRECTION('center_axis',(0.,0.,-1.));
#26634=DIRECTION('ref_axis',(1.,0.,0.));
#26635=DIRECTION('',(0.,0.,-1.));
#26636=DIRECTION('center_axis',(0.,0.,-1.));
#26637=DIRECTION('ref_axis',(1.,0.,0.));
#26638=DIRECTION('',(0.,0.,-1.));
#26639=DIRECTION('center_axis',(0.,0.,-1.));
#26640=DIRECTION('ref_axis',(1.,0.,0.));
#26641=DIRECTION('',(0.,0.,-1.));
#26642=DIRECTION('center_axis',(0.,0.,-1.));
#26643=DIRECTION('ref_axis',(1.,0.,0.));
#26644=DIRECTION('',(0.,0.,-1.));
#26645=DIRECTION('center_axis',(0.,0.,-1.));
#26646=DIRECTION('ref_axis',(1.,0.,0.));
#26647=DIRECTION('',(0.,0.,-1.));
#26648=DIRECTION('center_axis',(0.,0.,-1.));
#26649=DIRECTION('ref_axis',(1.,0.,0.));
#26650=DIRECTION('',(0.,0.,-1.));
#26651=DIRECTION('center_axis',(0.,0.,-1.));
#26652=DIRECTION('ref_axis',(1.,0.,0.));
#26653=DIRECTION('',(0.,0.,-1.));
#26654=DIRECTION('center_axis',(0.,0.,-1.));
#26655=DIRECTION('ref_axis',(1.,0.,0.));
#26656=DIRECTION('',(0.,0.,-1.));
#26657=DIRECTION('center_axis',(0.,0.,-1.));
#26658=DIRECTION('ref_axis',(1.,0.,0.));
#26659=DIRECTION('',(0.,0.,-1.));
#26660=DIRECTION('center_axis',(0.,0.,-1.));
#26661=DIRECTION('ref_axis',(1.,0.,0.));
#26662=DIRECTION('',(0.,0.,-1.));
#26663=DIRECTION('center_axis',(0.,0.,-1.));
#26664=DIRECTION('ref_axis',(0.937995432501147,-0.346647614454486,0.));
#26665=DIRECTION('',(0.,0.,-1.));
#26666=DIRECTION('center_axis',(0.,0.,-1.));
#26667=DIRECTION('ref_axis',(1.,0.,0.));
#26668=DIRECTION('center_axis',(0.,0.,-1.));
#26669=DIRECTION('ref_axis',(-0.346979462678664,0.937872727228607,0.));
#26670=DIRECTION('',(0.,0.,-1.));
#26671=DIRECTION('center_axis',(0.,0.,-1.));
#26672=DIRECTION('ref_axis',(1.,0.,0.));
#26673=DIRECTION('center_axis',(0.,0.,-1.));
#26674=DIRECTION('ref_axis',(1.,0.,0.));
#26675=DIRECTION('',(0.,0.,-1.));
#26676=DIRECTION('center_axis',(0.,0.,-1.));
#26677=DIRECTION('ref_axis',(1.,0.,0.));
#26678=DIRECTION('',(0.,0.,-1.));
#26679=DIRECTION('center_axis',(0.,0.,-1.));
#26680=DIRECTION('ref_axis',(1.,0.,0.));
#26681=DIRECTION('',(0.,0.,-1.));
#26682=DIRECTION('center_axis',(0.,0.,-1.));
#26683=DIRECTION('ref_axis',(1.,0.,0.));
#26684=DIRECTION('',(0.,0.,-1.));
#26685=DIRECTION('center_axis',(0.,0.,-1.));
#26686=DIRECTION('ref_axis',(1.,0.,0.));
#26687=DIRECTION('',(0.,0.,-1.));
#26688=DIRECTION('center_axis',(0.,0.,-1.));
#26689=DIRECTION('ref_axis',(1.,0.,0.));
#26690=DIRECTION('',(0.,0.,-1.));
#26691=DIRECTION('center_axis',(0.,0.,-1.));
#26692=DIRECTION('ref_axis',(1.,0.,0.));
#26693=DIRECTION('',(0.,0.,-1.));
#26694=DIRECTION('center_axis',(0.,0.,-1.));
#26695=DIRECTION('ref_axis',(1.,0.,0.));
#26696=DIRECTION('',(0.,0.,-1.));
#26697=DIRECTION('center_axis',(0.,0.,-1.));
#26698=DIRECTION('ref_axis',(1.,0.,0.));
#26699=DIRECTION('',(0.,0.,-1.));
#26700=DIRECTION('center_axis',(0.,0.,-1.));
#26701=DIRECTION('ref_axis',(1.,0.,0.));
#26702=DIRECTION('',(0.,0.,-1.));
#26703=DIRECTION('center_axis',(0.,0.,-1.));
#26704=DIRECTION('ref_axis',(1.,0.,0.));
#26705=DIRECTION('',(0.,0.,-1.));
#26706=DIRECTION('center_axis',(0.,0.,-1.));
#26707=DIRECTION('ref_axis',(1.,0.,0.));
#26708=DIRECTION('',(0.,0.,-1.));
#26709=DIRECTION('center_axis',(0.,0.,-1.));
#26710=DIRECTION('ref_axis',(1.,0.,0.));
#26711=DIRECTION('',(0.,0.,-1.));
#26712=DIRECTION('center_axis',(0.,0.,-1.));
#26713=DIRECTION('ref_axis',(1.,0.,0.));
#26714=DIRECTION('',(0.,0.,-1.));
#26715=DIRECTION('center_axis',(0.,0.,-1.));
#26716=DIRECTION('ref_axis',(1.,0.,0.));
#26717=DIRECTION('',(0.,0.,-1.));
#26718=DIRECTION('center_axis',(0.,0.,-1.));
#26719=DIRECTION('ref_axis',(1.,0.,0.));
#26720=DIRECTION('',(0.,0.,-1.));
#26721=DIRECTION('center_axis',(0.,0.,-1.));
#26722=DIRECTION('ref_axis',(1.,0.,0.));
#26723=DIRECTION('',(0.,0.,-1.));
#26724=DIRECTION('center_axis',(0.,0.,-1.));
#26725=DIRECTION('ref_axis',(1.,0.,0.));
#26726=DIRECTION('',(0.,0.,-1.));
#26727=DIRECTION('center_axis',(0.,0.,-1.));
#26728=DIRECTION('ref_axis',(0.937995529739744,-0.346647351335988,0.));
#26729=DIRECTION('',(0.,0.,-1.));
#26730=DIRECTION('center_axis',(0.,0.,-1.));
#26731=DIRECTION('ref_axis',(1.,0.,0.));
#26732=DIRECTION('center_axis',(0.,0.,-1.));
#26733=DIRECTION('ref_axis',(1.,-9.24734323422938E-14,0.));
#26734=DIRECTION('',(1.22464679914735E-16,-1.13397268902426E-29,-1.));
#26735=DIRECTION('center_axis',(0.,0.,1.));
#26736=DIRECTION('ref_axis',(1.,-9.24734323422938E-14,0.));
#26737=DIRECTION('center_axis',(0.,0.,-1.));
#26738=DIRECTION('ref_axis',(1.,-9.24734323422938E-14,0.));
#26739=DIRECTION('',(1.22464679914735E-16,-1.13397268902426E-29,-1.));
#26740=DIRECTION('center_axis',(0.,0.,-1.));
#26741=DIRECTION('ref_axis',(1.,-9.24734323422938E-14,0.));
#26742=DIRECTION('',(1.22464679914735E-16,-1.13397268902426E-29,-1.));
#26743=DIRECTION('center_axis',(0.,0.,-1.));
#26744=DIRECTION('ref_axis',(1.,-9.24734323422938E-14,0.));
#26745=DIRECTION('',(1.22464679914735E-16,-1.13397268902426E-29,-1.));
#26746=DIRECTION('center_axis',(0.,0.,-1.));
#26747=DIRECTION('ref_axis',(1.,-9.24734323422938E-14,0.));
#26748=DIRECTION('',(1.22464679914735E-16,-1.13397268902426E-29,-1.));
#26749=DIRECTION('center_axis',(0.,0.,-1.));
#26750=DIRECTION('ref_axis',(1.,-9.24734323422938E-14,0.));
#26751=DIRECTION('',(1.22464679914735E-16,-1.13397268902426E-29,-1.));
#26752=DIRECTION('center_axis',(0.,0.,-1.));
#26753=DIRECTION('ref_axis',(1.,-9.24734323422938E-14,0.));
#26754=DIRECTION('',(1.22464679914735E-16,-1.13397268902426E-29,-1.));
#26755=DIRECTION('center_axis',(0.,0.,-1.));
#26756=DIRECTION('ref_axis',(1.,-9.24734323422938E-14,0.));
#26757=DIRECTION('',(1.22464679914735E-16,-1.13397268902426E-29,-1.));
#26758=DIRECTION('center_axis',(0.,0.,-1.));
#26759=DIRECTION('ref_axis',(1.,-9.24734323422938E-14,0.));
#26760=DIRECTION('',(1.22464679914735E-16,-1.13397268902426E-29,-1.));
#26761=DIRECTION('center_axis',(0.,0.,-1.));
#26762=DIRECTION('ref_axis',(1.,-9.24734323422938E-14,0.));
#26763=DIRECTION('',(1.22464679914735E-16,-1.13397268902426E-29,-1.));
#26764=DIRECTION('center_axis',(0.,0.,-1.));
#26765=DIRECTION('ref_axis',(1.,-9.24734323422938E-14,0.));
#26766=DIRECTION('',(1.22464679914735E-16,-1.13397268902426E-29,-1.));
#26767=DIRECTION('center_axis',(0.,0.,-1.));
#26768=DIRECTION('ref_axis',(1.,-9.24734323422938E-14,0.));
#26769=DIRECTION('',(1.22464679914735E-16,-1.13397268902426E-29,-1.));
#26770=DIRECTION('center_axis',(0.,0.,-1.));
#26771=DIRECTION('ref_axis',(1.,-9.24734323422938E-14,0.));
#26772=DIRECTION('',(1.22464679914735E-16,-1.13397268902426E-29,-1.));
#26773=DIRECTION('center_axis',(0.,0.,-1.));
#26774=DIRECTION('ref_axis',(1.,-9.24734323422938E-14,0.));
#26775=DIRECTION('',(1.22464679914735E-16,-1.13397268902426E-29,-1.));
#26776=DIRECTION('center_axis',(0.,0.,-1.));
#26777=DIRECTION('ref_axis',(1.,-9.24734323422938E-14,0.));
#26778=DIRECTION('',(1.22464679914735E-16,-1.13397268902426E-29,-1.));
#26779=DIRECTION('center_axis',(0.,0.,-1.));
#26780=DIRECTION('ref_axis',(1.,-9.24734323422938E-14,0.));
#26781=DIRECTION('',(1.22464679914735E-16,-1.13397268902426E-29,-1.));
#26782=DIRECTION('center_axis',(0.,0.,-1.));
#26783=DIRECTION('ref_axis',(1.,-9.24734323422938E-14,0.));
#26784=DIRECTION('',(1.22464679914735E-16,-1.13397268902426E-29,-1.));
#26785=DIRECTION('center_axis',(0.,0.,-1.));
#26786=DIRECTION('ref_axis',(1.,-9.24734323422938E-14,0.));
#26787=DIRECTION('',(1.22464679914735E-16,-1.13397268902426E-29,-1.));
#26788=DIRECTION('center_axis',(0.,0.,-1.));
#26789=DIRECTION('ref_axis',(1.,-9.24734323422938E-14,0.));
#26790=DIRECTION('',(1.22464679914735E-16,-1.13397268902426E-29,-1.));
#26791=DIRECTION('center_axis',(0.,0.,-1.));
#26792=DIRECTION('ref_axis',(-0.609226759132665,-0.792996063014635,0.));
#26793=DIRECTION('',(1.22464679914735E-16,-1.13397268902426E-29,-1.));
#26794=DIRECTION('center_axis',(0.,0.,-1.));
#26795=DIRECTION('ref_axis',(1.,-9.24734323422938E-14,0.));
#26796=DIRECTION('center_axis',(0.,0.,-1.));
#26797=DIRECTION('ref_axis',(1.,-8.09142532995072E-14,0.));
#26798=DIRECTION('',(1.22464679914735E-16,-9.92413572869059E-30,-1.));
#26799=DIRECTION('center_axis',(0.,0.,1.));
#26800=DIRECTION('ref_axis',(1.,-8.09142532995072E-14,0.));
#26801=DIRECTION('center_axis',(0.,0.,-1.));
#26802=DIRECTION('ref_axis',(1.,-8.09142532995072E-14,0.));
#26803=DIRECTION('',(1.22464679914735E-16,-9.92413572869059E-30,-1.));
#26804=DIRECTION('center_axis',(0.,0.,-1.));
#26805=DIRECTION('ref_axis',(1.,-8.09142532995072E-14,0.));
#26806=DIRECTION('',(1.22464679914735E-16,-9.92413572869059E-30,-1.));
#26807=DIRECTION('center_axis',(0.,0.,-1.));
#26808=DIRECTION('ref_axis',(1.,-8.09142532995072E-14,0.));
#26809=DIRECTION('',(1.22464679914735E-16,-9.92413572869059E-30,-1.));
#26810=DIRECTION('center_axis',(0.,0.,-1.));
#26811=DIRECTION('ref_axis',(1.,-8.09142532995072E-14,0.));
#26812=DIRECTION('',(1.22464679914735E-16,-9.92413572869059E-30,-1.));
#26813=DIRECTION('center_axis',(0.,0.,-1.));
#26814=DIRECTION('ref_axis',(1.,-8.09142532995072E-14,0.));
#26815=DIRECTION('',(1.22464679914735E-16,-9.92413572869059E-30,-1.));
#26816=DIRECTION('center_axis',(0.,0.,-1.));
#26817=DIRECTION('ref_axis',(1.,-8.09142532995072E-14,0.));
#26818=DIRECTION('',(1.22464679914735E-16,-9.92413572869059E-30,-1.));
#26819=DIRECTION('center_axis',(0.,0.,-1.));
#26820=DIRECTION('ref_axis',(1.,-8.09142532995072E-14,0.));
#26821=DIRECTION('',(1.22464679914735E-16,-9.92413572869059E-30,-1.));
#26822=DIRECTION('center_axis',(0.,0.,-1.));
#26823=DIRECTION('ref_axis',(1.,-8.09142532995072E-14,0.));
#26824=DIRECTION('',(1.22464679914735E-16,-9.92413572869059E-30,-1.));
#26825=DIRECTION('center_axis',(0.,0.,-1.));
#26826=DIRECTION('ref_axis',(1.,-8.09142532995072E-14,0.));
#26827=DIRECTION('',(1.22464679914735E-16,-9.92413572869059E-30,-1.));
#26828=DIRECTION('center_axis',(0.,0.,-1.));
#26829=DIRECTION('ref_axis',(1.,-8.09142532995072E-14,0.));
#26830=DIRECTION('',(1.22464679914735E-16,-9.92413572869059E-30,-1.));
#26831=DIRECTION('center_axis',(0.,0.,-1.));
#26832=DIRECTION('ref_axis',(1.,-8.09142532995072E-14,0.));
#26833=DIRECTION('',(1.22464679914735E-16,-9.92413572869059E-30,-1.));
#26834=DIRECTION('center_axis',(0.,0.,-1.));
#26835=DIRECTION('ref_axis',(1.,-8.09142532995072E-14,0.));
#26836=DIRECTION('',(1.22464679914735E-16,-9.92413572869059E-30,-1.));
#26837=DIRECTION('center_axis',(0.,0.,-1.));
#26838=DIRECTION('ref_axis',(1.,-8.09142532995072E-14,0.));
#26839=DIRECTION('',(1.22464679914735E-16,-9.92413572869059E-30,-1.));
#26840=DIRECTION('center_axis',(0.,0.,-1.));
#26841=DIRECTION('ref_axis',(1.,-8.09142532995072E-14,0.));
#26842=DIRECTION('',(1.22464679914735E-16,-9.92413572869059E-30,-1.));
#26843=DIRECTION('center_axis',(0.,0.,-1.));
#26844=DIRECTION('ref_axis',(1.,-8.09142532995072E-14,0.));
#26845=DIRECTION('',(1.22464679914735E-16,-9.92413572869059E-30,-1.));
#26846=DIRECTION('center_axis',(0.,0.,-1.));
#26847=DIRECTION('ref_axis',(1.,-8.09142532995072E-14,0.));
#26848=DIRECTION('',(1.22464679914735E-16,-9.92413572869059E-30,-1.));
#26849=DIRECTION('center_axis',(0.,0.,-1.));
#26850=DIRECTION('ref_axis',(1.,-8.09142532995072E-14,0.));
#26851=DIRECTION('',(1.22464679914735E-16,-9.92413572869059E-30,-1.));
#26852=DIRECTION('center_axis',(0.,0.,-1.));
#26853=DIRECTION('ref_axis',(1.,-8.09142532995072E-14,0.));
#26854=DIRECTION('',(1.22464679914735E-16,-9.92413572869059E-30,-1.));
#26855=DIRECTION('center_axis',(0.,0.,-1.));
#26856=DIRECTION('ref_axis',(-0.60922700896484,-0.79299587107863,0.));
#26857=DIRECTION('',(1.22464679914735E-16,-9.92413572869059E-30,-1.));
#26858=DIRECTION('center_axis',(0.,0.,-1.));
#26859=DIRECTION('ref_axis',(1.,-8.09142532995072E-14,0.));
#26860=DIRECTION('center_axis',(0.,0.,-1.));
#26861=DIRECTION('ref_axis',(1.,-5.77958952139344E-14,0.));
#26862=DIRECTION('',(1.22464679914735E-16,-7.09295340558668E-30,-1.));
#26863=DIRECTION('center_axis',(0.,0.,1.));
#26864=DIRECTION('ref_axis',(1.,-5.77958952139344E-14,0.));
#26865=DIRECTION('center_axis',(0.,0.,-1.));
#26866=DIRECTION('ref_axis',(1.,-5.77958952139344E-14,0.));
#26867=DIRECTION('',(1.22464679914735E-16,-7.09295340558668E-30,-1.));
#26868=DIRECTION('center_axis',(0.,0.,-1.));
#26869=DIRECTION('ref_axis',(1.,-5.77958952139344E-14,0.));
#26870=DIRECTION('',(1.22464679914735E-16,-7.09295340558668E-30,-1.));
#26871=DIRECTION('center_axis',(0.,0.,-1.));
#26872=DIRECTION('ref_axis',(1.,-5.77958952139344E-14,0.));
#26873=DIRECTION('',(1.22464679914735E-16,-7.09295340558668E-30,-1.));
#26874=DIRECTION('center_axis',(0.,0.,-1.));
#26875=DIRECTION('ref_axis',(1.,-5.77958952139344E-14,0.));
#26876=DIRECTION('',(1.22464679914735E-16,-7.09295340558668E-30,-1.));
#26877=DIRECTION('center_axis',(0.,0.,-1.));
#26878=DIRECTION('ref_axis',(1.,-5.77958952139344E-14,0.));
#26879=DIRECTION('',(1.22464679914735E-16,-7.09295340558668E-30,-1.));
#26880=DIRECTION('center_axis',(0.,0.,-1.));
#26881=DIRECTION('ref_axis',(1.,-5.77958952139344E-14,0.));
#26882=DIRECTION('',(1.22464679914735E-16,-7.09295340558668E-30,-1.));
#26883=DIRECTION('center_axis',(0.,0.,-1.));
#26884=DIRECTION('ref_axis',(1.,-5.77958952139344E-14,0.));
#26885=DIRECTION('',(1.22464679914735E-16,-7.09295340558668E-30,-1.));
#26886=DIRECTION('center_axis',(0.,0.,-1.));
#26887=DIRECTION('ref_axis',(1.,-5.77958952139344E-14,0.));
#26888=DIRECTION('',(1.22464679914735E-16,-7.09295340558668E-30,-1.));
#26889=DIRECTION('center_axis',(0.,0.,-1.));
#26890=DIRECTION('ref_axis',(1.,-5.77958952139344E-14,0.));
#26891=DIRECTION('',(1.22464679914735E-16,-7.09295340558668E-30,-1.));
#26892=DIRECTION('center_axis',(0.,0.,-1.));
#26893=DIRECTION('ref_axis',(1.,-5.77958952139344E-14,0.));
#26894=DIRECTION('',(1.22464679914735E-16,-7.09295340558668E-30,-1.));
#26895=DIRECTION('center_axis',(0.,0.,-1.));
#26896=DIRECTION('ref_axis',(1.,-5.77958952139344E-14,0.));
#26897=DIRECTION('',(1.22464679914735E-16,-7.09295340558668E-30,-1.));
#26898=DIRECTION('center_axis',(0.,0.,-1.));
#26899=DIRECTION('ref_axis',(1.,-5.77958952139344E-14,0.));
#26900=DIRECTION('',(1.22464679914735E-16,-7.09295340558668E-30,-1.));
#26901=DIRECTION('center_axis',(0.,0.,-1.));
#26902=DIRECTION('ref_axis',(1.,-5.77958952139344E-14,0.));
#26903=DIRECTION('',(1.22464679914735E-16,-7.09295340558668E-30,-1.));
#26904=DIRECTION('center_axis',(0.,0.,-1.));
#26905=DIRECTION('ref_axis',(1.,-5.77958952139344E-14,0.));
#26906=DIRECTION('',(1.22464679914735E-16,-7.09295340558668E-30,-1.));
#26907=DIRECTION('center_axis',(0.,0.,-1.));
#26908=DIRECTION('ref_axis',(1.,-5.77958952139344E-14,0.));
#26909=DIRECTION('',(1.22464679914735E-16,-7.09295340558668E-30,-1.));
#26910=DIRECTION('center_axis',(0.,0.,-1.));
#26911=DIRECTION('ref_axis',(1.,-5.77958952139344E-14,0.));
#26912=DIRECTION('',(1.22464679914735E-16,-7.09295340558668E-30,-1.));
#26913=DIRECTION('center_axis',(0.,0.,-1.));
#26914=DIRECTION('ref_axis',(1.,-5.77958952139344E-14,0.));
#26915=DIRECTION('',(1.22464679914735E-16,-7.09295340558668E-30,-1.));
#26916=DIRECTION('center_axis',(0.,0.,-1.));
#26917=DIRECTION('ref_axis',(1.,-5.77958952139344E-14,0.));
#26918=DIRECTION('',(1.22464679914735E-16,-7.09295340558668E-30,-1.));
#26919=DIRECTION('center_axis',(0.,0.,-1.));
#26920=DIRECTION('ref_axis',(-0.609226998768103,-0.792995878912375,0.));
#26921=DIRECTION('',(1.22464679914735E-16,-7.09295340558668E-30,-1.));
#26922=DIRECTION('center_axis',(0.,0.,-1.));
#26923=DIRECTION('ref_axis',(1.,-5.77958952139344E-14,0.));
#26924=DIRECTION('center_axis',(0.,0.,-1.));
#26925=DIRECTION('ref_axis',(1.,-8.09142532995081E-14,0.));
#26926=DIRECTION('',(1.22464679914735E-16,-9.9241357286907E-30,-1.));
#26927=DIRECTION('center_axis',(0.,0.,1.));
#26928=DIRECTION('ref_axis',(1.,-8.09142532995081E-14,0.));
#26929=DIRECTION('center_axis',(0.,0.,-1.));
#26930=DIRECTION('ref_axis',(1.,-8.09142532995081E-14,0.));
#26931=DIRECTION('',(1.22464679914735E-16,-9.9241357286907E-30,-1.));
#26932=DIRECTION('center_axis',(0.,0.,-1.));
#26933=DIRECTION('ref_axis',(1.,-8.09142532995081E-14,0.));
#26934=DIRECTION('',(1.22464679914735E-16,-9.9241357286907E-30,-1.));
#26935=DIRECTION('center_axis',(0.,0.,-1.));
#26936=DIRECTION('ref_axis',(1.,-8.09142532995081E-14,0.));
#26937=DIRECTION('',(1.22464679914735E-16,-9.9241357286907E-30,-1.));
#26938=DIRECTION('center_axis',(0.,0.,-1.));
#26939=DIRECTION('ref_axis',(1.,-8.09142532995081E-14,0.));
#26940=DIRECTION('',(1.22464679914735E-16,-9.9241357286907E-30,-1.));
#26941=DIRECTION('center_axis',(0.,0.,-1.));
#26942=DIRECTION('ref_axis',(1.,-8.09142532995081E-14,0.));
#26943=DIRECTION('',(1.22464679914735E-16,-9.9241357286907E-30,-1.));
#26944=DIRECTION('center_axis',(0.,0.,-1.));
#26945=DIRECTION('ref_axis',(1.,-8.09142532995081E-14,0.));
#26946=DIRECTION('',(1.22464679914735E-16,-9.9241357286907E-30,-1.));
#26947=DIRECTION('center_axis',(0.,0.,-1.));
#26948=DIRECTION('ref_axis',(1.,-8.09142532995081E-14,0.));
#26949=DIRECTION('',(1.22464679914735E-16,-9.9241357286907E-30,-1.));
#26950=DIRECTION('center_axis',(0.,0.,-1.));
#26951=DIRECTION('ref_axis',(1.,-8.09142532995081E-14,0.));
#26952=DIRECTION('',(1.22464679914735E-16,-9.9241357286907E-30,-1.));
#26953=DIRECTION('center_axis',(0.,0.,-1.));
#26954=DIRECTION('ref_axis',(1.,-8.09142532995081E-14,0.));
#26955=DIRECTION('',(1.22464679914735E-16,-9.9241357286907E-30,-1.));
#26956=DIRECTION('center_axis',(0.,0.,-1.));
#26957=DIRECTION('ref_axis',(1.,-8.09142532995081E-14,0.));
#26958=DIRECTION('',(1.22464679914735E-16,-9.9241357286907E-30,-1.));
#26959=DIRECTION('center_axis',(0.,0.,-1.));
#26960=DIRECTION('ref_axis',(1.,-8.09142532995081E-14,0.));
#26961=DIRECTION('',(1.22464679914735E-16,-9.9241357286907E-30,-1.));
#26962=DIRECTION('center_axis',(0.,0.,-1.));
#26963=DIRECTION('ref_axis',(1.,-8.09142532995081E-14,0.));
#26964=DIRECTION('',(1.22464679914735E-16,-9.9241357286907E-30,-1.));
#26965=DIRECTION('center_axis',(0.,0.,-1.));
#26966=DIRECTION('ref_axis',(1.,-8.09142532995081E-14,0.));
#26967=DIRECTION('',(1.22464679914735E-16,-9.9241357286907E-30,-1.));
#26968=DIRECTION('center_axis',(0.,0.,-1.));
#26969=DIRECTION('ref_axis',(1.,-8.09142532995081E-14,0.));
#26970=DIRECTION('',(1.22464679914735E-16,-9.9241357286907E-30,-1.));
#26971=DIRECTION('center_axis',(0.,0.,-1.));
#26972=DIRECTION('ref_axis',(1.,-8.09142532995081E-14,0.));
#26973=DIRECTION('',(1.22464679914735E-16,-9.9241357286907E-30,-1.));
#26974=DIRECTION('center_axis',(0.,0.,-1.));
#26975=DIRECTION('ref_axis',(1.,-8.09142532995081E-14,0.));
#26976=DIRECTION('',(1.22464679914735E-16,-9.9241357286907E-30,-1.));
#26977=DIRECTION('center_axis',(0.,0.,-1.));
#26978=DIRECTION('ref_axis',(1.,-8.09142532995081E-14,0.));
#26979=DIRECTION('',(1.22464679914735E-16,-9.9241357286907E-30,-1.));
#26980=DIRECTION('center_axis',(0.,0.,-1.));
#26981=DIRECTION('ref_axis',(1.,-8.09142532995081E-14,0.));
#26982=DIRECTION('',(1.22464679914735E-16,-9.9241357286907E-30,-1.));
#26983=DIRECTION('center_axis',(0.,0.,-1.));
#26984=DIRECTION('ref_axis',(-0.609227002488276,-0.792995876054315,0.));
#26985=DIRECTION('',(1.22464679914735E-16,-9.9241357286907E-30,-1.));
#26986=DIRECTION('center_axis',(0.,0.,-1.));
#26987=DIRECTION('ref_axis',(1.,-8.09142532995081E-14,0.));
#26988=DIRECTION('center_axis',(0.,0.,-1.));
#26989=DIRECTION('ref_axis',(1.,-1.04032611385081E-13,0.));
#26990=DIRECTION('',(1.22464679914735E-16,-1.27553180517946E-29,-1.));
#26991=DIRECTION('center_axis',(0.,0.,1.));
#26992=DIRECTION('ref_axis',(1.,-1.04032611385081E-13,0.));
#26993=DIRECTION('center_axis',(0.,0.,-1.));
#26994=DIRECTION('ref_axis',(1.,-1.04032611385081E-13,0.));
#26995=DIRECTION('',(1.22464679914735E-16,-1.27553180517946E-29,-1.));
#26996=DIRECTION('center_axis',(0.,0.,-1.));
#26997=DIRECTION('ref_axis',(1.,-1.04032611385081E-13,0.));
#26998=DIRECTION('',(1.22464679914735E-16,-1.27553180517946E-29,-1.));
#26999=DIRECTION('center_axis',(0.,0.,-1.));
#27000=DIRECTION('ref_axis',(1.,-1.04032611385081E-13,0.));
#27001=DIRECTION('',(1.22464679914735E-16,-1.27553180517946E-29,-1.));
#27002=DIRECTION('center_axis',(0.,0.,-1.));
#27003=DIRECTION('ref_axis',(1.,-1.04032611385081E-13,0.));
#27004=DIRECTION('',(1.22464679914735E-16,-1.27553180517946E-29,-1.));
#27005=DIRECTION('center_axis',(0.,0.,-1.));
#27006=DIRECTION('ref_axis',(1.,-1.04032611385081E-13,0.));
#27007=DIRECTION('',(1.22464679914735E-16,-1.27553180517946E-29,-1.));
#27008=DIRECTION('center_axis',(0.,0.,-1.));
#27009=DIRECTION('ref_axis',(1.,-1.04032611385081E-13,0.));
#27010=DIRECTION('',(1.22464679914735E-16,-1.27553180517946E-29,-1.));
#27011=DIRECTION('center_axis',(0.,0.,-1.));
#27012=DIRECTION('ref_axis',(1.,-1.04032611385081E-13,0.));
#27013=DIRECTION('',(1.22464679914735E-16,-1.27553180517946E-29,-1.));
#27014=DIRECTION('center_axis',(0.,0.,-1.));
#27015=DIRECTION('ref_axis',(1.,-1.04032611385081E-13,0.));
#27016=DIRECTION('',(1.22464679914735E-16,-1.27553180517946E-29,-1.));
#27017=DIRECTION('center_axis',(0.,0.,-1.));
#27018=DIRECTION('ref_axis',(1.,-1.04032611385081E-13,0.));
#27019=DIRECTION('',(1.22464679914735E-16,-1.27553180517946E-29,-1.));
#27020=DIRECTION('center_axis',(0.,0.,-1.));
#27021=DIRECTION('ref_axis',(1.,-1.04032611385081E-13,0.));
#27022=DIRECTION('',(1.22464679914735E-16,-1.27553180517946E-29,-1.));
#27023=DIRECTION('center_axis',(0.,0.,-1.));
#27024=DIRECTION('ref_axis',(1.,-1.04032611385081E-13,0.));
#27025=DIRECTION('',(1.22464679914735E-16,-1.27553180517946E-29,-1.));
#27026=DIRECTION('center_axis',(0.,0.,-1.));
#27027=DIRECTION('ref_axis',(1.,-1.04032611385081E-13,0.));
#27028=DIRECTION('',(1.22464679914735E-16,-1.27553180517946E-29,-1.));
#27029=DIRECTION('center_axis',(0.,0.,-1.));
#27030=DIRECTION('ref_axis',(1.,-1.04032611385081E-13,0.));
#27031=DIRECTION('',(1.22464679914735E-16,-1.27553180517946E-29,-1.));
#27032=DIRECTION('center_axis',(0.,0.,-1.));
#27033=DIRECTION('ref_axis',(1.,-1.04032611385081E-13,0.));
#27034=DIRECTION('',(1.22464679914735E-16,-1.27553180517946E-29,-1.));
#27035=DIRECTION('center_axis',(0.,0.,-1.));
#27036=DIRECTION('ref_axis',(1.,-1.04032611385081E-13,0.));
#27037=DIRECTION('',(1.22464679914735E-16,-1.27553180517946E-29,-1.));
#27038=DIRECTION('center_axis',(0.,0.,-1.));
#27039=DIRECTION('ref_axis',(1.,-1.04032611385081E-13,0.));
#27040=DIRECTION('',(1.22464679914735E-16,-1.27553180517946E-29,-1.));
#27041=DIRECTION('center_axis',(0.,0.,-1.));
#27042=DIRECTION('ref_axis',(1.,-1.04032611385081E-13,0.));
#27043=DIRECTION('',(1.22464679914735E-16,-1.27553180517946E-29,-1.));
#27044=DIRECTION('center_axis',(0.,0.,-1.));
#27045=DIRECTION('ref_axis',(1.,-1.04032611385081E-13,0.));
#27046=DIRECTION('',(1.22464679914735E-16,-1.27553180517946E-29,-1.));
#27047=DIRECTION('center_axis',(0.,0.,-1.));
#27048=DIRECTION('ref_axis',(-0.60922700588817,-0.792995873442312,0.));
#27049=DIRECTION('',(1.22464679914735E-16,-1.27553180517946E-29,-1.));
#27050=DIRECTION('center_axis',(0.,0.,-1.));
#27051=DIRECTION('ref_axis',(1.,-1.04032611385081E-13,0.));
#27052=DIRECTION('center_axis',(0.,0.,-1.));
#27053=DIRECTION('ref_axis',(1.,-9.24734323422938E-14,0.));
#27054=DIRECTION('',(1.22464679914735E-16,-1.13397268902426E-29,-1.));
#27055=DIRECTION('center_axis',(0.,0.,1.));
#27056=DIRECTION('ref_axis',(1.,-9.24734323422938E-14,0.));
#27057=DIRECTION('center_axis',(0.,0.,-1.));
#27058=DIRECTION('ref_axis',(1.,-9.24734323422938E-14,0.));
#27059=DIRECTION('',(1.22464679914735E-16,-1.13397268902426E-29,-1.));
#27060=DIRECTION('center_axis',(0.,0.,-1.));
#27061=DIRECTION('ref_axis',(1.,-9.24734323422938E-14,0.));
#27062=DIRECTION('',(1.22464679914735E-16,-1.13397268902426E-29,-1.));
#27063=DIRECTION('center_axis',(0.,0.,-1.));
#27064=DIRECTION('ref_axis',(1.,-9.24734323422938E-14,0.));
#27065=DIRECTION('',(1.22464679914735E-16,-1.13397268902426E-29,-1.));
#27066=DIRECTION('center_axis',(0.,0.,-1.));
#27067=DIRECTION('ref_axis',(1.,-9.24734323422938E-14,0.));
#27068=DIRECTION('',(1.22464679914735E-16,-1.13397268902426E-29,-1.));
#27069=DIRECTION('center_axis',(0.,0.,-1.));
#27070=DIRECTION('ref_axis',(1.,-9.24734323422938E-14,0.));
#27071=DIRECTION('',(1.22464679914735E-16,-1.13397268902426E-29,-1.));
#27072=DIRECTION('center_axis',(0.,0.,-1.));
#27073=DIRECTION('ref_axis',(1.,-9.24734323422938E-14,0.));
#27074=DIRECTION('',(1.22464679914735E-16,-1.13397268902426E-29,-1.));
#27075=DIRECTION('center_axis',(0.,0.,-1.));
#27076=DIRECTION('ref_axis',(1.,-9.24734323422938E-14,0.));
#27077=DIRECTION('',(1.22464679914735E-16,-1.13397268902426E-29,-1.));
#27078=DIRECTION('center_axis',(0.,0.,-1.));
#27079=DIRECTION('ref_axis',(1.,-9.24734323422938E-14,0.));
#27080=DIRECTION('',(1.22464679914735E-16,-1.13397268902426E-29,-1.));
#27081=DIRECTION('center_axis',(0.,0.,-1.));
#27082=DIRECTION('ref_axis',(1.,-9.24734323422938E-14,0.));
#27083=DIRECTION('',(1.22464679914735E-16,-1.13397268902426E-29,-1.));
#27084=DIRECTION('center_axis',(0.,0.,-1.));
#27085=DIRECTION('ref_axis',(1.,-9.24734323422938E-14,0.));
#27086=DIRECTION('',(1.22464679914735E-16,-1.13397268902426E-29,-1.));
#27087=DIRECTION('center_axis',(0.,0.,-1.));
#27088=DIRECTION('ref_axis',(1.,-9.24734323422938E-14,0.));
#27089=DIRECTION('',(1.22464679914735E-16,-1.13397268902426E-29,-1.));
#27090=DIRECTION('center_axis',(0.,0.,-1.));
#27091=DIRECTION('ref_axis',(1.,-9.24734323422938E-14,0.));
#27092=DIRECTION('',(1.22464679914735E-16,-1.13397268902426E-29,-1.));
#27093=DIRECTION('center_axis',(0.,0.,-1.));
#27094=DIRECTION('ref_axis',(1.,-9.24734323422938E-14,0.));
#27095=DIRECTION('',(1.22464679914735E-16,-1.13397268902426E-29,-1.));
#27096=DIRECTION('center_axis',(0.,0.,-1.));
#27097=DIRECTION('ref_axis',(1.,-9.24734323422938E-14,0.));
#27098=DIRECTION('',(1.22464679914735E-16,-1.13397268902426E-29,-1.));
#27099=DIRECTION('center_axis',(0.,0.,-1.));
#27100=DIRECTION('ref_axis',(1.,-9.24734323422938E-14,0.));
#27101=DIRECTION('',(1.22464679914735E-16,-1.13397268902426E-29,-1.));
#27102=DIRECTION('center_axis',(0.,0.,-1.));
#27103=DIRECTION('ref_axis',(1.,-9.24734323422938E-14,0.));
#27104=DIRECTION('',(1.22464679914735E-16,-1.13397268902426E-29,-1.));
#27105=DIRECTION('center_axis',(0.,0.,-1.));
#27106=DIRECTION('ref_axis',(1.,-9.24734323422938E-14,0.));
#27107=DIRECTION('',(1.22464679914735E-16,-1.13397268902426E-29,-1.));
#27108=DIRECTION('center_axis',(0.,0.,-1.));
#27109=DIRECTION('ref_axis',(1.,-9.24734323422938E-14,0.));
#27110=DIRECTION('',(1.22464679914735E-16,-1.13397268902426E-29,-1.));
#27111=DIRECTION('center_axis',(0.,0.,-1.));
#27112=DIRECTION('ref_axis',(-0.609226762267633,-0.792996060606165,0.));
#27113=DIRECTION('',(1.22464679914735E-16,-1.13397268902426E-29,-1.));
#27114=DIRECTION('center_axis',(0.,0.,-1.));
#27115=DIRECTION('ref_axis',(1.,-9.24734323422938E-14,0.));
#27116=DIRECTION('center_axis',(0.,0.,-1.));
#27117=DIRECTION('ref_axis',(1.,-9.24734323422938E-14,0.));
#27118=DIRECTION('center_axis',(0.,0.,1.));
#27119=DIRECTION('ref_axis',(1.,0.,0.));
#27120=DIRECTION('',(0.,-1.,0.));
#27121=DIRECTION('',(1.,0.,0.));
#27122=DIRECTION('',(0.,1.,0.));
#27123=DIRECTION('',(-1.,0.,0.));
#27124=DIRECTION('center_axis',(0.,0.,-1.));
#27125=DIRECTION('ref_axis',(1.,-1.04032611385081E-13,0.));
#27126=DIRECTION('center_axis',(0.,0.,-1.));
#27127=DIRECTION('ref_axis',(1.,-8.09142532995081E-14,0.));
#27128=DIRECTION('center_axis',(0.,0.,-1.));
#27129=DIRECTION('ref_axis',(1.,-5.77958952139344E-14,0.));
#27130=DIRECTION('center_axis',(0.,0.,-1.));
#27131=DIRECTION('ref_axis',(1.,-8.09142532995072E-14,0.));
#27132=DIRECTION('center_axis',(0.,0.,-1.));
#27133=DIRECTION('ref_axis',(1.,-9.24734323422938E-14,0.));
#27134=DIRECTION('center_axis',(0.,0.,-1.));
#27135=DIRECTION('ref_axis',(1.,0.,0.));
#27136=DIRECTION('center_axis',(0.,0.,-1.));
#27137=DIRECTION('ref_axis',(1.,0.,0.));
#27138=DIRECTION('center_axis',(0.,0.,-1.));
#27139=DIRECTION('ref_axis',(1.,0.,0.));
#27140=DIRECTION('center_axis',(0.,0.,-1.));
#27141=DIRECTION('ref_axis',(1.,0.,0.));
#27142=DIRECTION('center_axis',(0.,0.,-1.));
#27143=DIRECTION('ref_axis',(1.,0.,0.));
#27144=DIRECTION('center_axis',(0.,0.,-1.));
#27145=DIRECTION('ref_axis',(1.,0.,0.));
#27146=DIRECTION('center_axis',(0.,1.,0.));
#27147=DIRECTION('ref_axis',(-1.,0.,0.));
#27148=DIRECTION('',(-1.,0.,0.));
#27149=DIRECTION('',(0.,0.,1.));
#27150=DIRECTION('',(0.,0.,1.));
#27151=DIRECTION('center_axis',(1.,0.,0.));
#27152=DIRECTION('ref_axis',(0.,1.,0.));
#27153=DIRECTION('',(0.,1.,0.));
#27154=DIRECTION('',(0.,0.,1.));
#27155=DIRECTION('center_axis',(0.,-1.,0.));
#27156=DIRECTION('ref_axis',(1.,0.,0.));
#27157=DIRECTION('',(1.,0.,0.));
#27158=DIRECTION('',(0.,0.,1.));
#27159=DIRECTION('center_axis',(-1.,0.,0.));
#27160=DIRECTION('ref_axis',(0.,-1.,0.));
#27161=DIRECTION('',(0.,-1.,0.));
#27162=DIRECTION('center_axis',(0.,0.,1.));
#27163=DIRECTION('ref_axis',(1.,0.,0.));
#72980=CARTESIAN_POINT('',(0.,0.,0.));
#72981=CARTESIAN_POINT('Origin',(160.,225.,10.));
#72982=CARTESIAN_POINT('',(157.486483939918,225.000575042283,0.387416697507991));
#72983=CARTESIAN_POINT('',(157.48459726363,224.996259956084,0.112583302491957));
#72984=CARTESIAN_POINT('',(157.4825,225.,10.));
#72985=CARTESIAN_POINT('',(158.086534003335,226.635987203375,0.));
#72986=CARTESIAN_POINT('Ctrl Pts',(157.48459726363,224.996259956084,0.112583302491957));
#72987=CARTESIAN_POINT('Ctrl Pts',(157.489762449105,225.588952407467,0.0750555349946362));
#72988=CARTESIAN_POINT('Ctrl Pts',(157.700778171916,226.184803560304,0.0375277674973158));
#72989=CARTESIAN_POINT('Ctrl Pts',(158.086534003335,226.635987203375,-4.09394740330526E-15));
#72990=CARTESIAN_POINT('',(161.917152715742,226.638755029745,8.50380292826545E-15));
#72991=CARTESIAN_POINT('Origin',(160.,225.,0.));
#72992=CARTESIAN_POINT('Ctrl Pts',(161.917156415839,226.638757807614,5.95993938154068E-15));
#72993=CARTESIAN_POINT('Ctrl Pts',(161.386618674923,227.257451018951,0.0517556153419846));
#72994=CARTESIAN_POINT('Ctrl Pts',(160.527623995925,227.597124544241,0.103511230683961));
#72995=CARTESIAN_POINT('Ctrl Pts',(159.717628701157,227.505772300943,0.15526684602594));
#72996=CARTESIAN_POINT('Ctrl Pts',(158.889421475104,227.412366094136,0.208186134436534));
#72997=CARTESIAN_POINT('Ctrl Pts',(158.112441807901,226.868333858592,0.261105422847131));
#72998=CARTESIAN_POINT('Ctrl Pts',(157.741727721422,226.12214743685,0.314024711257726));
#72999=CARTESIAN_POINT('Ctrl Pts',(157.570350743671,225.77719379613,0.338488706674481));
#73000=CARTESIAN_POINT('Ctrl Pts',(157.485797170545,225.389037591527,0.362952702091236));
#73001=CARTESIAN_POINT('Ctrl Pts',(157.486483939918,225.000575042283,0.387416697507991));
#73002=CARTESIAN_POINT('Origin',(160.,225.,10.));
#73003=CARTESIAN_POINT('',(157.482539767498,224.997698761652,1.38741669750799));
#73004=CARTESIAN_POINT('',(157.478271555719,225.000135319788,1.11258330249196));
#73005=CARTESIAN_POINT('',(157.4825,225.,10.));
#73006=CARTESIAN_POINT('Ctrl Pts',(157.478271555719,225.000135319788,1.11258330249196));
#73007=CARTESIAN_POINT('Ctrl Pts',(157.478266683081,225.006844587079,1.11215722053548));
#73008=CARTESIAN_POINT('Ctrl Pts',(157.478291126166,225.013553815972,1.11173113857901));
#73009=CARTESIAN_POINT('Ctrl Pts',(157.478344991774,225.020262806545,1.11130505662253));
#73010=CARTESIAN_POINT('Ctrl Pts',(157.485035088855,225.85351800941,1.05838576821194));
#73011=CARTESIAN_POINT('Ctrl Pts',(157.945584889413,226.683097001022,1.00546647980134));
#73012=CARTESIAN_POINT('Ctrl Pts',(158.649263586559,227.129460441397,0.952547191390747));
#73013=CARTESIAN_POINT('Ctrl Pts',(159.352942283705,227.575823881771,0.899627902980148));
#73014=CARTESIAN_POINT('Ctrl Pts',(160.299749877437,227.638971770909,0.84670861456955));
#73015=CARTESIAN_POINT('Ctrl Pts',(161.056392441986,227.289849947809,0.793789326158952));
#73016=CARTESIAN_POINT('Ctrl Pts',(161.813035006535,226.940728124708,0.740870037748355));
#73017=CARTESIAN_POINT('Ctrl Pts',(162.3795125419,226.179336589369,0.687950749337759));
#73018=CARTESIAN_POINT('Ctrl Pts',(162.496677259461,225.354415175787,0.635031460927162));
#73019=CARTESIAN_POINT('Ctrl Pts',(162.613841977023,224.529493762204,0.582112172516563));
#73020=CARTESIAN_POINT('Ctrl Pts',(162.281693876781,223.641042470379,0.529192884105964));
#73021=CARTESIAN_POINT('Ctrl Pts',(161.65207595311,223.09493528623,0.476273595695365));
#73022=CARTESIAN_POINT('Ctrl Pts',(161.022458029439,222.548828102082,0.423354307284768));
#73023=CARTESIAN_POINT('Ctrl Pts',(160.09537028234,222.34506502561,0.370435018874173));
#73024=CARTESIAN_POINT('Ctrl Pts',(159.295373479341,222.578292580861,0.317515730463577));
#73025=CARTESIAN_POINT('Ctrl Pts',(158.495376676342,222.811520136111,0.264596442052982));
#73026=CARTESIAN_POINT('Ctrl Pts',(157.822470817444,223.481738323085,0.211677153642386));
#73027=CARTESIAN_POINT('Ctrl Pts',(157.584268019495,224.278797417901,0.158757865231791));
#73028=CARTESIAN_POINT('Ctrl Pts',(157.514986979324,224.510621240471,0.143366344318513));
#73029=CARTESIAN_POINT('Ctrl Pts',(157.482478830652,224.753174932141,0.127974823405235));
#73030=CARTESIAN_POINT('Ctrl Pts',(157.48459726363,224.996259956084,0.112583302491957));
#73031=CARTESIAN_POINT('Ctrl Pts',(157.486483939918,225.000575042283,0.387416697507991));
#73032=CARTESIAN_POINT('Ctrl Pts',(157.487282755622,224.548734880137,0.415871990501833));
#73033=CARTESIAN_POINT('Ctrl Pts',(157.603404731867,224.096480258932,0.444327283495675));
#73034=CARTESIAN_POINT('Ctrl Pts',(157.832358689369,223.711314639842,0.472782576489517));
#73035=CARTESIAN_POINT('Ctrl Pts',(158.258152249548,222.995008872516,0.525701864900114));
#73036=CARTESIAN_POINT('Ctrl Pts',(159.07418787566,222.510737945805,0.578621153310711));
#73037=CARTESIAN_POINT('Ctrl Pts',(159.906929713407,222.479994087708,0.631540441721308));
#73038=CARTESIAN_POINT('Ctrl Pts',(160.739671551153,222.449250229612,0.684459730131907));
#73039=CARTESIAN_POINT('Ctrl Pts',(161.589119600533,222.872033440131,0.737379018542505));
#73040=CARTESIAN_POINT('Ctrl Pts',(162.066623300567,223.5549311968,0.790298306953104));
#73041=CARTESIAN_POINT('Ctrl Pts',(162.544127000601,224.237828953469,0.843217595363701));
#73042=CARTESIAN_POINT('Ctrl Pts',(162.649686351289,225.180841256288,0.896136883774297));
#73043=CARTESIAN_POINT('Ctrl Pts',(162.334970000144,225.952420120802,0.949056172184893));
#73044=CARTESIAN_POINT('Ctrl Pts',(162.020253649,226.723998985317,1.00197546059549));
#73045=CARTESIAN_POINT('Ctrl Pts',(161.285261596023,227.324144411527,1.05489474900609));
#73046=CARTESIAN_POINT('Ctrl Pts',(160.466339392169,227.478242187855,1.10781403741669));
#73047=CARTESIAN_POINT('Ctrl Pts',(159.647417188314,227.632339964183,1.16073332582729));
#73048=CARTESIAN_POINT('Ctrl Pts',(158.744564833583,227.34039009063,1.21365261423788));
#73049=CARTESIAN_POINT('Ctrl Pts',(158.170921185734,226.735982884831,1.26657190264848));
#73050=CARTESIAN_POINT('Ctrl Pts',(157.734269755296,226.275914561981,1.30685350093498));
#73051=CARTESIAN_POINT('Ctrl Pts',(157.488364882719,225.634805582068,1.34713509922148));
#73052=CARTESIAN_POINT('Ctrl Pts',(157.482539767498,224.997698761652,1.38741669750799));
#73053=CARTESIAN_POINT('Origin',(160.,225.,10.));
#73054=CARTESIAN_POINT('',(157.478659078657,225.000905528694,2.38741669750799));
#73055=CARTESIAN_POINT('',(157.484174776371,225.002114825273,2.11258330249196));
#73056=CARTESIAN_POINT('',(157.4825,225.,10.));
#73057=CARTESIAN_POINT('Ctrl Pts',(157.484174776371,225.002114825273,2.11258330249196));
#73058=CARTESIAN_POINT('Ctrl Pts',(157.48212567403,225.259454343706,2.09633961766574));
#73059=CARTESIAN_POINT('Ctrl Pts',(157.518448799924,225.516229216226,2.08009593283951));
#73060=CARTESIAN_POINT('Ctrl Pts',(157.59554743232,225.760113789415,2.06385224801329));
#73061=CARTESIAN_POINT('Ctrl Pts',(157.846722261643,226.554650140346,2.0109329596027));
#73062=CARTESIAN_POINT('Ctrl Pts',(158.530668186833,227.212375217892,1.9580136711921));
#73063=CARTESIAN_POINT('Ctrl Pts',(159.334411776144,227.432314991755,1.9050943827815));
#73064=CARTESIAN_POINT('Ctrl Pts',(160.138155365455,227.652254765619,1.8521750943709));
#73065=CARTESIAN_POINT('Ctrl Pts',(161.061696618887,227.4344092358,1.7992558059603));
#73066=CARTESIAN_POINT('Ctrl Pts',(161.682422640936,226.878462536606,1.74633651754971));
#73067=CARTESIAN_POINT('Ctrl Pts',(162.303148662985,226.322515837411,1.69341722913911));
#73068=CARTESIAN_POINT('Ctrl Pts',(162.621059453651,225.428467968842,1.64049794072851));
#73069=CARTESIAN_POINT('Ctrl Pts',(162.490679946232,224.605439317717,1.58757865231791));
#73070=CARTESIAN_POINT('Ctrl Pts',(162.360300438814,223.782410666591,1.53465936390732));
#73071=CARTESIAN_POINT('Ctrl Pts',(161.78163063331,223.03040123291,1.48174007549672));
#73072=CARTESIAN_POINT('Ctrl Pts',(161.019467943839,222.693522012104,1.42882078708612));
#73073=CARTESIAN_POINT('Ctrl Pts',(160.257305254368,222.356642791298,1.37590149867553));
#73074=CARTESIAN_POINT('Ctrl Pts',(159.311649680928,222.434893783368,1.32298221026493));
#73075=CARTESIAN_POINT('Ctrl Pts',(158.615237091009,222.892484986464,1.27006292185433));
#73076=CARTESIAN_POINT('Ctrl Pts',(157.924431697403,223.346391874048,1.21756971540021));
#73077=CARTESIAN_POINT('Ctrl Pts',(157.478871863597,224.173555015805,1.16507650894608));
#73078=CARTESIAN_POINT('Ctrl Pts',(157.478271555719,225.000135319788,1.11258330249196));
#73079=CARTESIAN_POINT('Ctrl Pts',(157.482539767498,224.997698761652,1.38741669750799));
#73080=CARTESIAN_POINT('Ctrl Pts',(157.480712233233,224.797816956687,1.40005438763208));
#73081=CARTESIAN_POINT('Ctrl Pts',(157.502515451918,224.598329079321,1.41269207775617));
#73082=CARTESIAN_POINT('Ctrl Pts',(157.549472852864,224.404949327159,1.42532976788027));
#73083=CARTESIAN_POINT('Ctrl Pts',(157.746103108808,223.595187513332,1.47824905629087));
#73084=CARTESIAN_POINT('Ctrl Pts',(158.383798561664,222.892528423726,1.53116834470147));
#73085=CARTESIAN_POINT('Ctrl Pts',(159.170748307313,222.618507464788,1.58408763311207));
#73086=CARTESIAN_POINT('Ctrl Pts',(159.957698052962,222.34448650585,1.63700692152266));
#73087=CARTESIAN_POINT('Ctrl Pts',(160.893902091404,222.499103677581,1.68992620993326));
#73088=CARTESIAN_POINT('Ctrl Pts',(161.550954185028,223.011606829843,1.74284549834386));
#73089=CARTESIAN_POINT('Ctrl Pts',(162.208006278652,223.524109982105,1.79576478675445));
#73090=CARTESIAN_POINT('Ctrl Pts',(162.585906427457,224.394499114897,1.84868407516505));
#73091=CARTESIAN_POINT('Ctrl Pts',(162.511727187682,225.224483857895,1.90160336357565));
#73092=CARTESIAN_POINT('Ctrl Pts',(162.437547947907,226.054468600893,1.95452265198625));
#73093=CARTESIAN_POINT('Ctrl Pts',(161.911289319553,226.844048954097,2.00744194039685));
#73094=CARTESIAN_POINT('Ctrl Pts',(161.173767405945,227.231913117744,2.06036122880744));
#73095=CARTESIAN_POINT('Ctrl Pts',(160.436245492337,227.619777281391,2.11328051721804));
#73096=CARTESIAN_POINT('Ctrl Pts',(159.487460293475,227.605925255482,2.16619980562864));
#73097=CARTESIAN_POINT('Ctrl Pts',(158.761575818028,227.196695652424,2.21911909403924));
#73098=CARTESIAN_POINT('Ctrl Pts',(158.03569134258,226.787466049366,2.27203838244983));
#73099=CARTESIAN_POINT('Ctrl Pts',(157.532707590547,225.982858869159,2.32495767086043));
#73100=CARTESIAN_POINT('Ctrl Pts',(157.482789955364,225.151062377488,2.37787695927103));
#73101=CARTESIAN_POINT('Ctrl Pts',(157.479790411547,225.101079840967,2.38105687201668));
#73102=CARTESIAN_POINT('Ctrl Pts',(157.478426795029,225.05099912951,2.38423678476234));
#73103=CARTESIAN_POINT('Ctrl Pts',(157.478659078657,225.000905528694,2.38741669750799));
#73104=CARTESIAN_POINT('Origin',(160.,225.,10.));
#73105=CARTESIAN_POINT('',(157.485215863135,225.001726236658,3.38741669750799));
#73106=CARTESIAN_POINT('',(157.485769661895,224.998633683171,3.11258330249196));
#73107=CARTESIAN_POINT('',(157.4825,225.,10.));
#73108=CARTESIAN_POINT('Ctrl Pts',(157.485769661895,224.998633683171,3.11258330249196));
#73109=CARTESIAN_POINT('Ctrl Pts',(157.488277019004,225.507373471095,3.08052201479599));
#73110=CARTESIAN_POINT('Ctrl Pts',(157.638052762054,226.017470645054,3.04846072710002));
#73111=CARTESIAN_POINT('Ctrl Pts',(157.924920111362,226.432902133972,3.01639943940405));
#73112=CARTESIAN_POINT('Ctrl Pts',(158.398413756956,227.118599445487,2.96348015099345));
#73113=CARTESIAN_POINT('Ctrl Pts',(159.245395644497,227.546392416654,2.91056086258285));
#73114=CARTESIAN_POINT('Ctrl Pts',(160.078286881534,227.520523004211,2.85764157417226));
#73115=CARTESIAN_POINT('Ctrl Pts',(160.911178118571,227.494653591767,2.80472228576166));
#73116=CARTESIAN_POINT('Ctrl Pts',(161.729978705104,227.015121795713,2.75180299735106));
#73117=CARTESIAN_POINT('Ctrl Pts',(162.160005503369,226.301361331734,2.69888370894047));
#73118=CARTESIAN_POINT('Ctrl Pts',(162.590032301635,225.587600867755,2.64596442052987));
#73119=CARTESIAN_POINT('Ctrl Pts',(162.631285311633,224.639611735851,2.59304513211927));
#73120=CARTESIAN_POINT('Ctrl Pts',(162.26488716814,223.891193795518,2.54012584370867));
#73121=CARTESIAN_POINT('Ctrl Pts',(161.898489024646,223.142775855184,2.48720655529807));
#73122=CARTESIAN_POINT('Ctrl Pts',(161.124439727659,222.593929106419,2.43428726688747));
#73123=CARTESIAN_POINT('Ctrl Pts',(160.296944196735,222.49580570407,2.38136797847687));
#73124=CARTESIAN_POINT('Ctrl Pts',(159.469448665811,222.39768230172,2.32844869006628));
#73125=CARTESIAN_POINT('Ctrl Pts',(158.588506900948,222.750282245786,2.27552940165568));
#73126=CARTESIAN_POINT('Ctrl Pts',(158.057237885245,223.392256029976,2.22261011324508));
#73127=CARTESIAN_POINT('Ctrl Pts',(157.689042990683,223.837174635795,2.18593450966071));
#73128=CARTESIAN_POINT('Ctrl Pts',(157.488801316835,224.421083965243,2.14925890607633));
#73129=CARTESIAN_POINT('Ctrl Pts',(157.484174776371,225.002114825273,2.11258330249196));
#73130=CARTESIAN_POINT('Ctrl Pts',(157.478659078657,225.000905528694,2.38741669750799));
#73131=CARTESIAN_POINT('Ctrl Pts',(157.482292399308,224.217354334461,2.43715607317293));
#73132=CARTESIAN_POINT('Ctrl Pts',(157.876385195861,223.430649576648,2.48689544883788));
#73133=CARTESIAN_POINT('Ctrl Pts',(158.507754644582,222.967176837434,2.53663482450282));
#73134=CARTESIAN_POINT('Ctrl Pts',(159.179488487313,222.474073592187,2.58955411291342));
#73135=CARTESIAN_POINT('Ctrl Pts',(160.119807691108,222.346852904829,2.64247340132401));
#73136=CARTESIAN_POINT('Ctrl Pts',(160.898422215714,222.643730967717,2.69539268973461));
#73137=CARTESIAN_POINT('Ctrl Pts',(161.677036740321,222.940609030605,2.74831197814521));
#73138=CARTESIAN_POINT('Ctrl Pts',(162.293946585739,223.661585843738,2.80123126655581));
#73139=CARTESIAN_POINT('Ctrl Pts',(162.466853814539,224.476742427593,2.8541505549664));
#73140=CARTESIAN_POINT('Ctrl Pts',(162.639761043338,225.291899011447,2.907069843377));
#73141=CARTESIAN_POINT('Ctrl Pts',(162.368665655519,226.201235366023,2.9599891317876));
#73142=CARTESIAN_POINT('Ctrl Pts',(161.777620897288,226.788639195277,3.0129084201982));
#73143=CARTESIAN_POINT('Ctrl Pts',(161.186576139056,227.376043024532,3.0658277086088));
#73144=CARTESIAN_POINT('Ctrl Pts',(160.275582010412,227.641514328466,3.11874699701939));
#73145=CARTESIAN_POINT('Ctrl Pts',(159.461509405714,227.463573442687,3.17166628542999));
#73146=CARTESIAN_POINT('Ctrl Pts',(158.647436801015,227.285632556909,3.22458557384059));
#73147=CARTESIAN_POINT('Ctrl Pts',(157.930285720262,226.664279481418,3.27750486225119));
#73148=CARTESIAN_POINT('Ctrl Pts',(157.638224484387,225.883845371791,3.33042415066178));
#73149=CARTESIAN_POINT('Ctrl Pts',(157.533377309456,225.603677031858,3.34942166627719));
#73150=CARTESIAN_POINT('Ctrl Pts',(157.483313203619,225.303007267603,3.36841918189259));
#73151=CARTESIAN_POINT('Ctrl Pts',(157.485215863135,225.001726236658,3.38741669750799));
#73152=CARTESIAN_POINT('Origin',(160.,225.,10.));
#73153=CARTESIAN_POINT('',(157.484904367492,224.998127113727,4.38741669750799));
#73154=CARTESIAN_POINT('',(157.479195958542,224.99863044174,4.11258330249196));
#73155=CARTESIAN_POINT('',(157.4825,225.,10.));
#73156=CARTESIAN_POINT('Ctrl Pts',(157.479195958542,224.99863044174,4.11258330249196));
#73157=CARTESIAN_POINT('Ctrl Pts',(157.484147283841,225.753298234935,4.06470441192624));
#73158=CARTESIAN_POINT('Ctrl Pts',(157.845660169901,226.512080307909,4.01682552136052));
#73159=CARTESIAN_POINT('Ctrl Pts',(158.437397204933,226.979251770666,3.9689466307948));
#73160=CARTESIAN_POINT('Ctrl Pts',(159.091428709216,227.495604198275,3.9160273423842));
#73161=CARTESIAN_POINT('Ctrl Pts',(160.026709034588,227.655716237085,3.8631080539736));
#73162=CARTESIAN_POINT('Ctrl Pts',(160.815253922581,227.386320621434,3.81018876556301));
#73163=CARTESIAN_POINT('Ctrl Pts',(161.603798810575,227.116925005784,3.75726947715241));
#73164=CARTESIAN_POINT('Ctrl Pts',(162.245608261189,226.418021735672,3.70435018874181));
#73165=CARTESIAN_POINT('Ctrl Pts',(162.446990282374,225.609428933451,3.65143090033122));
#73166=CARTESIAN_POINT('Ctrl Pts',(162.64837230356,224.80083613123,3.59851161192062));
#73167=CARTESIAN_POINT('Ctrl Pts',(162.409326895316,223.882553796899,3.54559232351002));
#73168=CARTESIAN_POINT('Ctrl Pts',(161.839241231897,223.274787909237,3.49267303509942));
#73169=CARTESIAN_POINT('Ctrl Pts',(161.269155568478,222.667022021574,3.43975374668882));
#73170=CARTESIAN_POINT('Ctrl Pts',(160.368029649885,222.369772580581,3.38683445827823));
#73171=CARTESIAN_POINT('Ctrl Pts',(159.548218678452,222.519060923273,3.33391516986763));
#73172=CARTESIAN_POINT('Ctrl Pts',(158.72840770702,222.668349265967,3.28099588145703));
#73173=CARTESIAN_POINT('Ctrl Pts',(157.989911682748,223.264175392347,3.22807659304644));
#73174=CARTESIAN_POINT('Ctrl Pts',(157.670666372435,224.033889281469,3.17515730463584));
#73175=CARTESIAN_POINT('Ctrl Pts',(157.544836658721,224.337270020922,3.15429930392121));
#73176=CARTESIAN_POINT('Ctrl Pts',(157.484138459279,224.667664604178,3.13344130320659));
#73177=CARTESIAN_POINT('Ctrl Pts',(157.485769661895,224.998633683171,3.11258330249196));
#73178=CARTESIAN_POINT('Ctrl Pts',(157.485215863135,225.001726236658,3.38741669750799));
#73179=CARTESIAN_POINT('Ctrl Pts',(157.488613232829,224.463761858256,3.42133847030319));
#73180=CARTESIAN_POINT('Ctrl Pts',(157.657697874279,223.923848559047,3.45526024309838));
#73181=CARTESIAN_POINT('Ctrl Pts',(157.9764364223,223.495222051598,3.48918201589358));
#73182=CARTESIAN_POINT('Ctrl Pts',(158.473680987085,222.826547984796,3.54210130430417));
#73183=CARTESIAN_POINT('Ctrl Pts',(159.335141507653,222.428714994955,3.59502059271477));
#73184=CARTESIAN_POINT('Ctrl Pts',(160.166613666841,222.483771450508,3.64793988112537));
#73185=CARTESIAN_POINT('Ctrl Pts',(160.998085826029,222.538827906061,3.70085916953596));
#73186=CARTESIAN_POINT('Ctrl Pts',(161.799569623837,223.046773807008,3.75377845794656));
#73187=CARTESIAN_POINT('Ctrl Pts',(162.204306090093,223.775173119013,3.80669774635716));
#73188=CARTESIAN_POINT('Ctrl Pts',(162.60904255635,224.503572431018,3.85961703476776));
#73189=CARTESIAN_POINT('Ctrl Pts',(162.617031691054,225.452425154081,3.91253632317835));
#73190=CARTESIAN_POINT('Ctrl Pts',(162.224617666349,226.187536300809,3.96545561158895));
#73191=CARTESIAN_POINT('Ctrl Pts',(161.832203641644,226.922647447537,4.01837489999955));
#73192=CARTESIAN_POINT('Ctrl Pts',(161.03938645753,227.444017017929,4.07129418841015));
#73193=CARTESIAN_POINT('Ctrl Pts',(160.208959241856,227.513066306815,4.12421347682075));
#73194=CARTESIAN_POINT('Ctrl Pts',(159.378532026181,227.5821155957,4.17713276523135));
#73195=CARTESIAN_POINT('Ctrl Pts',(158.510494778948,227.198844603078,4.23005205364194));
#73196=CARTESIAN_POINT('Ctrl Pts',(158.002061327427,226.538638127642,4.28297134205254));
#73197=CARTESIAN_POINT('Ctrl Pts',(157.667567584443,226.10429429277,4.31778646053769));
#73198=CARTESIAN_POINT('Ctrl Pts',(157.488717715052,225.550087119984,4.35260157902284));
#73199=CARTESIAN_POINT('Ctrl Pts',(157.484904367492,224.998127113727,4.38741669750799));
#73200=CARTESIAN_POINT('Origin',(160.,225.,10.));
#73201=CARTESIAN_POINT('',(157.478473441424,224.999338730904,5.38741669750799));
#73202=CARTESIAN_POINT('',(157.481647251813,225.00223805178,5.11258330249196));
#73203=CARTESIAN_POINT('',(157.4825,225.,10.));
#73204=CARTESIAN_POINT('Ctrl Pts',(157.481647251813,225.00223805178,5.11258330249196));
#73205=CARTESIAN_POINT('Ctrl Pts',(157.480078416762,225.172538839621,5.10180609746709));
#73206=CARTESIAN_POINT('Ctrl Pts',(157.495878683591,225.342550212557,5.09102889244222));
#73207=CARTESIAN_POINT('Ctrl Pts',(157.530116486515,225.508763694247,5.08025168741734));
#73208=CARTESIAN_POINT('Ctrl Pts',(157.698234302151,226.32492142299,5.02733239900675));
#73209=CARTESIAN_POINT('Ctrl Pts',(158.310900040407,227.049508094982,4.97441311059615));
#73210=CARTESIAN_POINT('Ctrl Pts',(159.087757871502,227.350952863366,4.92149382218556));
#73211=CARTESIAN_POINT('Ctrl Pts',(159.864615702598,227.652397631749,4.86857453377496));
#73212=CARTESIAN_POINT('Ctrl Pts',(160.805665626533,227.530700496525,4.81565524536436));
#73213=CARTESIAN_POINT('Ctrl Pts',(161.480283216618,227.04155006438,4.76273595695376));
#73214=CARTESIAN_POINT('Ctrl Pts',(162.154900806703,226.552399632235,4.70981666854317));
#73215=CARTESIAN_POINT('Ctrl Pts',(162.563086062939,225.695795903169,4.65689738013257));
#73216=CARTESIAN_POINT('Ctrl Pts',(162.518053420096,224.863720726757,4.60397809172197));
#73217=CARTESIAN_POINT('Ctrl Pts',(162.473020777253,224.031645550345,4.55105880331137));
#73218=CARTESIAN_POINT('Ctrl Pts',(161.974770235332,223.224098926587,4.49813951490078));
#73219=CARTESIAN_POINT('Ctrl Pts',(161.251301232521,222.810614174644,4.44522022649018));
#73220=CARTESIAN_POINT('Ctrl Pts',(160.52783222971,222.397129422701,4.39230093807958));
#73221=CARTESIAN_POINT('Ctrl Pts',(159.579144766009,222.377706542573,4.33938164966898));
#73222=CARTESIAN_POINT('Ctrl Pts',(158.839358206151,222.761233443809,4.28646236125838));
#73223=CARTESIAN_POINT('Ctrl Pts',(158.099571646293,223.144760345044,4.23354307284779));
#73224=CARTESIAN_POINT('Ctrl Pts',(157.568685990277,223.931237027643,4.18062378443719));
#73225=CARTESIAN_POINT('Ctrl Pts',(157.489634503867,224.760771777146,4.12770449602659));
#73226=CARTESIAN_POINT('Ctrl Pts',(157.482105095333,224.839782385362,4.12266409818172));
#73227=CARTESIAN_POINT('Ctrl Pts',(157.478674713186,224.919183615102,4.11762370033684));
#73228=CARTESIAN_POINT('Ctrl Pts',(157.479195958542,224.99863044174,4.11258330249196));
#73229=CARTESIAN_POINT('Ctrl Pts',(157.484904367492,224.998127113727,4.38741669750799));
#73230=CARTESIAN_POINT('Ctrl Pts',(157.482921392991,224.711103022467,4.40552086743344));
#73231=CARTESIAN_POINT('Ctrl Pts',(157.528269906085,224.424686585732,4.42362503735889));
#73232=CARTESIAN_POINT('Ctrl Pts',(157.623676807573,224.156048394559,4.44172920728433));
#73233=CARTESIAN_POINT('Ctrl Pts',(157.902555395047,223.370807095162,4.49464849569493));
#73234=CARTESIAN_POINT('Ctrl Pts',(158.609142225803,222.737466454618,4.54756778410552));
#73235=CARTESIAN_POINT('Ctrl Pts',(159.42010317998,222.545843137587,4.60048707251612));
#73236=CARTESIAN_POINT('Ctrl Pts',(160.231064134158,222.354219820557,4.65340636092672));
#73237=CARTESIAN_POINT('Ctrl Pts',(161.146399211757,222.604313827041,4.70632564933731));
#73238=CARTESIAN_POINT('Ctrl Pts',(161.747251099266,223.181682144589,4.75924493774791));
#73239=CARTESIAN_POINT('Ctrl Pts',(162.348102986775,223.759050462136,4.81216422615851));
#73240=CARTESIAN_POINT('Ctrl Pts',(162.634471684193,224.663693090748,4.86508351456911));
#73241=CARTESIAN_POINT('Ctrl Pts',(162.475314881213,225.481645581359,4.91800280297971));
#73242=CARTESIAN_POINT('Ctrl Pts',(162.316158078232,226.299598071969,4.9709220913903));
#73243=CARTESIAN_POINT('Ctrl Pts',(161.711475774853,227.030860424578,5.0238413798009));
#73244=CARTESIAN_POINT('Ctrl Pts',(160.937970581213,227.340807001009,5.0767606682115));
#73245=CARTESIAN_POINT('Ctrl Pts',(160.164465387572,227.650753577441,5.1296799566221));
#73246=CARTESIAN_POINT('Ctrl Pts',(159.22213730367,227.539384377695,5.1825992450327));
#73247=CARTESIAN_POINT('Ctrl Pts',(158.542195642172,227.057661945386,5.23551853344329));
#73248=CARTESIAN_POINT('Ctrl Pts',(157.891633291123,226.596754053046,5.28615125479819));
#73249=CARTESIAN_POINT('Ctrl Pts',(157.48127254598,225.796806356742,5.33678397615309));
#73250=CARTESIAN_POINT('Ctrl Pts',(157.478473441424,224.999338730904,5.38741669750799));
#73251=CARTESIAN_POINT('Origin',(160.,225.,10.));
#73252=CARTESIAN_POINT('',(157.482962656938,225.002292268722,6.38741669750799));
#73253=CARTESIAN_POINT('',(157.486517381253,224.999964780133,6.11258330249196));
#73254=CARTESIAN_POINT('',(157.4825,225.,10.));
#73255=CARTESIAN_POINT('Ctrl Pts',(157.486517381253,224.999964780133,6.11258330249196));
#73256=CARTESIAN_POINT('Ctrl Pts',(157.486570082313,225.422277771847,6.08598849459734));
#73257=CARTESIAN_POINT('Ctrl Pts',(157.587291160886,225.844614382724,6.05939368670272));
#73258=CARTESIAN_POINT('Ctrl Pts',(157.788540203288,226.211862465092,6.0327988788081));
#73259=CARTESIAN_POINT('Ctrl Pts',(158.188992658498,226.942625675193,5.97987959039751));
#73260=CARTESIAN_POINT('Ctrl Pts',(158.987480022325,227.455268905782,5.92696030198691));
#73261=CARTESIAN_POINT('Ctrl Pts',(159.818614492781,227.515206624622,5.87404101357631));
#73262=CARTESIAN_POINT('Ctrl Pts',(160.649748963237,227.575144343462,5.82112172516571));
#73263=CARTESIAN_POINT('Ctrl Pts',(161.513530540323,227.182376550552,5.76820243675512));
#73264=CARTESIAN_POINT('Ctrl Pts',(162.014692791348,226.516633780206,5.71528314834452));
#73265=CARTESIAN_POINT('Ctrl Pts',(162.515855042373,225.85089100986,5.66236385993392));
#73266=CARTESIAN_POINT('Ctrl Pts',(162.654397967336,224.912173262077,5.60944457152333));
#73267=CARTESIAN_POINT('Ctrl Pts',(162.366924326499,224.130037759786,5.55652528311273));
#73268=CARTESIAN_POINT('Ctrl Pts',(162.079450685662,223.347902257495,5.50360599470213));
#73269=CARTESIAN_POINT('Ctrl Pts',(161.365960479025,222.722349000695,5.45068670629153));
#73270=CARTESIAN_POINT('Ctrl Pts',(160.552946811115,222.539631147399,5.39776741788093));
#73271=CARTESIAN_POINT('Ctrl Pts',(159.739933143206,222.356913294103,5.34484812947034));
#73272=CARTESIAN_POINT('Ctrl Pts',(158.827396014025,222.617030844311,5.29192884105974));
#73273=CARTESIAN_POINT('Ctrl Pts',(158.232912395943,223.200954012161,5.23900955264914));
#73274=CARTESIAN_POINT('Ctrl Pts',(157.759497522896,223.66595910897,5.19686746926341));
#73275=CARTESIAN_POINT('Ctrl Pts',(157.487781864395,224.336311219614,5.15472538587769));
#73276=CARTESIAN_POINT('Ctrl Pts',(157.481647251813,225.00223805178,5.11258330249196));
#73277=CARTESIAN_POINT('Ctrl Pts',(157.478473441424,224.999338730904,5.38741669750799));
#73278=CARTESIAN_POINT('Ctrl Pts',(157.478347034229,224.963325197512,5.38970326456369));
#73279=CARTESIAN_POINT('Ctrl Pts',(157.47905181385,224.92731672201,5.39198983161939));
#73280=CARTESIAN_POINT('Ctrl Pts',(157.480603194088,224.891344758261,5.39427639867509));
#73281=CARTESIAN_POINT('Ctrl Pts',(157.516507646598,224.058825668318,5.44719568708568));
#73282=CARTESIAN_POINT('Ctrl Pts',(158.00587179071,223.245863153303,5.50011497549628));
#73283=CARTESIAN_POINT('Ctrl Pts',(158.724762603703,222.824468844103,5.55303426390688));
#73284=CARTESIAN_POINT('Ctrl Pts',(159.443653416695,222.403074534903,5.60595355231748));
#73285=CARTESIAN_POINT('Ctrl Pts',(160.392070898566,222.373248431518,5.65887284072807));
#73286=CARTESIAN_POINT('Ctrl Pts',(161.136019228261,222.748638958271,5.71179212913867));
#73287=CARTESIAN_POINT('Ctrl Pts',(161.879967557955,223.124029485023,5.76471141754927));
#73288=CARTESIAN_POINT('Ctrl Pts',(162.419446735472,223.904636641913,5.81763070595987));
#73289=CARTESIAN_POINT('Ctrl Pts',(162.507591099788,224.733254609297,5.87054999437046));
#73290=CARTESIAN_POINT('Ctrl Pts',(162.595735464103,225.56187257668,5.92346928278106));
#73291=CARTESIAN_POINT('Ctrl Pts',(162.232545015216,226.438501354556,5.97638857119166));
#73292=CARTESIAN_POINT('Ctrl Pts',(161.584215695397,226.961995631405,6.02930785960225));
#73293=CARTESIAN_POINT('Ctrl Pts',(160.935886375578,227.485489908254,6.08222714801285));
#73294=CARTESIAN_POINT('Ctrl Pts',(160.002418184827,227.655849684076,6.13514643642345));
#73295=CARTESIAN_POINT('Ctrl Pts',(159.210966148877,227.395118328805,6.18806572483405));
#73296=CARTESIAN_POINT('Ctrl Pts',(158.419514112928,227.134386973534,6.24098501324465));
#73297=CARTESIAN_POINT('Ctrl Pts',(157.770078231779,226.442564487169,6.29390430165524));
#73298=CARTESIAN_POINT('Ctrl Pts',(157.559840351877,225.636228825869,6.34682359006584));
#73299=CARTESIAN_POINT('Ctrl Pts',(157.506084219323,225.430055291815,6.36035462587989));
#73300=CARTESIAN_POINT('Ctrl Pts',(157.48104213666,225.216395072921,6.37388566169394));
#73301=CARTESIAN_POINT('Ctrl Pts',(157.482962656938,225.002292268722,6.38741669750799));
#73302=CARTESIAN_POINT('Origin',(160.,225.,10.));
#73303=CARTESIAN_POINT('',(157.486314893834,224.999260124597,7.38741669750799));
#73304=CARTESIAN_POINT('',(157.481517992965,224.997780425011,7.11258330249197));
#73305=CARTESIAN_POINT('',(157.4825,225.,10.));
#73306=CARTESIAN_POINT('Ctrl Pts',(157.481517992965,224.997780425011,7.11258330249197));
#73307=CARTESIAN_POINT('Ctrl Pts',(157.487674873099,225.667890457605,7.0701708917276));
#73308=CARTESIAN_POINT('Ctrl Pts',(157.763272295833,226.342472777999,7.02775848096323));
#73309=CARTESIAN_POINT('Ctrl Pts',(158.242102427776,226.808026878213,6.98534607019886));
#73310=CARTESIAN_POINT('Ctrl Pts',(158.839553725528,227.388913256892,6.93242678178826));
#73311=CARTESIAN_POINT('Ctrl Pts',(159.753404444403,227.644377570781,6.87950749337766));
#73312=CARTESIAN_POINT('Ctrl Pts',(160.565476513413,227.457519354868,6.82658820496707));
#73313=CARTESIAN_POINT('Ctrl Pts',(161.377548582423,227.270661138954,6.77366891655647));
#73314=CARTESIAN_POINT('Ctrl Pts',(162.087842001567,226.641480393238,6.72074962814587));
#73315=CARTESIAN_POINT('Ctrl Pts',(162.371326516211,225.857890214587,6.66783033973528));
#73316=CARTESIAN_POINT('Ctrl Pts',(162.654811030855,225.074300035937,6.61491105132468));
#73317=CARTESIAN_POINT('Ctrl Pts',(162.511486640999,224.136300424352,6.56199176291408));
#73318=CARTESIAN_POINT('Ctrl Pts',(162.006938584623,223.473119983652,6.50907247450348));
#73319=CARTESIAN_POINT('Ctrl Pts',(161.502390528247,222.809939542952,6.45615318609288));
#73320=CARTESIAN_POINT('Ctrl Pts',(160.636618805351,222.421578273136,6.40323389768229));
#73321=CARTESIAN_POINT('Ctrl Pts',(159.805800539309,222.485750283635,6.35031460927169));
#73322=CARTESIAN_POINT('Ctrl Pts',(158.974982273267,222.549922294135,6.29739532086109));
#73323=CARTESIAN_POINT('Ctrl Pts',(158.17911746408,223.066627584951,6.24447603245049));
#73324=CARTESIAN_POINT('Ctrl Pts',(157.782393832782,223.799421825165,6.19155674403989));
#73325=CARTESIAN_POINT('Ctrl Pts',(157.585045307963,224.163947280403,6.16523226352392));
#73326=CARTESIAN_POINT('Ctrl Pts',(157.486465215882,224.581944459547,6.13890778300794));
#73327=CARTESIAN_POINT('Ctrl Pts',(157.486517381253,224.999964780133,6.11258330249196));
#73328=CARTESIAN_POINT('Ctrl Pts',(157.482962656938,225.002292268722,6.38741669750799));
#73329=CARTESIAN_POINT('Ctrl Pts',(157.488553207347,224.379048383382,6.42680495010454));
#73330=CARTESIAN_POINT('Ctrl Pts',(157.722615849539,223.752054177995,6.46619320270109));
#73331=CARTESIAN_POINT('Ctrl Pts',(158.141948568882,223.295062726516,6.50558145529763));
#73332=CARTESIAN_POINT('Ctrl Pts',(158.705334544446,222.681081124701,6.55850074370823));
#73333=CARTESIAN_POINT('Ctrl Pts',(159.603146374231,222.373966757305,6.61142003211883));
#73334=CARTESIAN_POINT('Ctrl Pts',(160.42454538258,222.514255152811,6.66433932052943));
#73335=CARTESIAN_POINT('Ctrl Pts',(161.245944390929,222.654543548318,6.71725860894002));
#73336=CARTESIAN_POINT('Ctrl Pts',(161.990930577842,223.242234706726,6.77017789735062));
#73337=CARTESIAN_POINT('Ctrl Pts',(162.318598278836,224.008401165504,6.82309718576122));
#73338=CARTESIAN_POINT('Ctrl Pts',(162.64626597983,224.774567624282,6.87601647417181));
#73339=CARTESIAN_POINT('Ctrl Pts',(162.556615194904,225.719209383429,6.92893576258241));
#73340=CARTESIAN_POINT('Ctrl Pts',(162.090670121478,226.410058392533,6.98185505099301));
#73341=CARTESIAN_POINT('Ctrl Pts',(161.624725048052,227.100907401638,7.03477433940361));
#73342=CARTESIAN_POINT('Ctrl Pts',(160.782485686126,227.5379636607,7.0876936278142));
#73343=CARTESIAN_POINT('Ctrl Pts',(159.949360751157,227.521230234166,7.1406129162248));
#73344=CARTESIAN_POINT('Ctrl Pts',(159.116235816188,227.504496807632,7.1935322046354));
#73345=CARTESIAN_POINT('Ctrl Pts',(158.292225308176,227.033973695501,7.246451493046));
#73346=CARTESIAN_POINT('Ctrl Pts',(157.854396419386,226.324972264635,7.29937078145659));
#73347=CARTESIAN_POINT('Ctrl Pts',(157.611579816057,225.931765412355,7.32871942014039));
#73348=CARTESIAN_POINT('Ctrl Pts',(157.487542176156,225.465209114919,7.35806805882419));
#73349=CARTESIAN_POINT('Ctrl Pts',(157.486314893834,224.999260124597,7.38741669750799));
#73350=CARTESIAN_POINT('Origin',(160.,225.,10.));
#73351=CARTESIAN_POINT('',(157.480251844254,224.998100046348,8.387416697508));
#73352=CARTESIAN_POINT('',(157.479288468299,225.001430882652,8.11258330249197));
#73353=CARTESIAN_POINT('',(157.4825,225.,10.));
#73354=CARTESIAN_POINT('Ctrl Pts',(157.479288468299,225.001430882652,8.11258330249197));
#73355=CARTESIAN_POINT('Ctrl Pts',(157.478719681623,225.085146706162,8.10727257726844));
#73356=CARTESIAN_POINT('Ctrl Pts',(157.4825287714,225.168810144924,8.10196185204492));
#73357=CARTESIAN_POINT('Ctrl Pts',(157.490886088512,225.252016757275,8.0966511268214));
#73358=CARTESIAN_POINT('Ctrl Pts',(157.57416346702,226.081137928365,8.0437318384108));
#73359=CARTESIAN_POINT('Ctrl Pts',(158.109049745654,226.864899257462,7.99081255000021));
#73360=CARTESIAN_POINT('Ctrl Pts',(158.85078097383,227.244651575782,7.93789326158961));
#73361=CARTESIAN_POINT('Ctrl Pts',(159.592512202006,227.624403894102,7.88497397317902));
#73362=CARTESIAN_POINT('Ctrl Pts',(160.541088379722,227.600147201645,7.83205468476842));
#73363=CARTESIAN_POINT('Ctrl Pts',(161.262441066707,227.182981360402,7.77913539635782));
#73364=CARTESIAN_POINT('Ctrl Pts',(161.983793753692,226.765815519159,7.72621610794722));
#73365=CARTESIAN_POINT('Ctrl Pts',(162.477922949946,225.955740529131,7.67329681953663));
#73366=CARTESIAN_POINT('Ctrl Pts',(162.518715144978,225.123446689826,7.62037753112603));
#73367=CARTESIAN_POINT('Ctrl Pts',(162.55950734001,224.291152850521,7.56745824271543));
#73368=CARTESIAN_POINT('Ctrl Pts',(162.146962533821,223.43664016194,7.51453895430483));
#73369=CARTESIAN_POINT('Ctrl Pts',(161.469861221611,222.950933613575,7.46161966589423));
#73370=CARTESIAN_POINT('Ctrl Pts',(160.792759909401,222.465227065211,7.40870037748364));
#73371=CARTESIAN_POINT('Ctrl Pts',(159.85110209117,222.348326657064,7.35578108907304));
#73372=CARTESIAN_POINT('Ctrl Pts',(159.075790366026,222.653726013603,7.30286180066244));
#73373=CARTESIAN_POINT('Ctrl Pts',(158.300478640882,222.959125370143,7.24994251225184));
#73374=CARTESIAN_POINT('Ctrl Pts',(157.691513008825,223.686824491369,7.19702322384125));
#73375=CARTESIAN_POINT('Ctrl Pts',(157.527556131111,224.503828273716,7.14410393543065));
#73376=CARTESIAN_POINT('Ctrl Pts',(157.495003258517,224.666040560303,7.13359705778442));
#73377=CARTESIAN_POINT('Ctrl Pts',(157.479992741628,224.831773258829,7.12309018013819));
#73378=CARTESIAN_POINT('Ctrl Pts',(157.481517992965,224.997780425011,7.11258330249197));
#73379=CARTESIAN_POINT('Ctrl Pts',(157.486314893834,224.999260124597,7.38741669750799));
#73380=CARTESIAN_POINT('Ctrl Pts',(157.485329231704,224.625044456207,7.41098734723479));
#73381=CARTESIAN_POINT('Ctrl Pts',(157.563557612755,224.251220507643,7.43455799696159));
#73382=CARTESIAN_POINT('Ctrl Pts',(157.723088400219,223.916099730613,7.45812864668839));
#73383=CARTESIAN_POINT('Ctrl Pts',(158.081256539411,223.163708377062,7.51104793509899));
#73384=CARTESIAN_POINT('Ctrl Pts',(158.849240087364,222.606405419563,7.56396722350959));
#73385=CARTESIAN_POINT('Ctrl Pts',(159.675609787634,222.499212680511,7.61688651192018));
#73386=CARTESIAN_POINT('Ctrl Pts',(160.501979487905,222.392019941459,7.66980580033078));
#73387=CARTESIAN_POINT('Ctrl Pts',(161.386735340493,222.734937420853,7.72272508874138));
#73388=CARTESIAN_POINT('Ctrl Pts',(161.92501308465,223.371046086864,7.77564437715197));
#73389=CARTESIAN_POINT('Ctrl Pts',(162.463290828808,224.007154752876,7.82856366556257));
#73390=CARTESIAN_POINT('Ctrl Pts',(162.655090464535,224.936454605506,7.88148295397317));
#73391=CARTESIAN_POINT('Ctrl Pts',(162.412644482294,225.733698050462,7.93440224238377));
#73392=CARTESIAN_POINT('Ctrl Pts',(162.170198500053,226.530941495419,7.98732153079436));
#73393=CARTESIAN_POINT('Ctrl Pts',(161.493506899843,227.196128532701,8.04024081920496));
#73394=CARTESIAN_POINT('Ctrl Pts',(160.692223744617,227.424869587129,8.09316010761556));
#73395=CARTESIAN_POINT('Ctrl Pts',(159.89094058939,227.653610641557,8.14607939602615));
#73396=CARTESIAN_POINT('Ctrl Pts',(158.965065879146,227.445905713129,8.19899868443675));
#73397=CARTESIAN_POINT('Ctrl Pts',(158.338279863088,226.896800573011,8.25191797284735));
#73398=CARTESIAN_POINT('Ctrl Pts',(157.803322393818,226.428143186607,8.2970842144009));
#73399=CARTESIAN_POINT('Ctrl Pts',(157.486236167406,225.710792720596,8.34225045595445));
#73400=CARTESIAN_POINT('Ctrl Pts',(157.480251844254,224.998100046348,8.387416697508));
#73401=CARTESIAN_POINT('Origin',(160.,225.,10.));
#73402=CARTESIAN_POINT('',(157.480388031054,225.001947791586,9.387416697508));
#73403=CARTESIAN_POINT('',(157.485838515826,225.001308641677,9.11258330249197));
#73404=CARTESIAN_POINT('',(157.4825,225.,10.));
#73405=CARTESIAN_POINT('Ctrl Pts',(157.485838515826,225.001308641677,9.11258330249197));
#73406=CARTESIAN_POINT('Ctrl Pts',(157.484258502333,225.336590190805,9.0914549743987));
#73407=CARTESIAN_POINT('Ctrl Pts',(157.546594678729,225.671308165495,9.07032664630543));
#73408=CARTESIAN_POINT('Ctrl Pts',(157.675619457858,225.977967362484,9.04919831821216));
#73409=CARTESIAN_POINT('Ctrl Pts',(157.998782723248,226.746044534403,8.99627902980156));
#73410=CARTESIAN_POINT('Ctrl Pts',(158.74030520912,227.338099899218,8.94335974139096));
#73411=CARTESIAN_POINT('Ctrl Pts',(159.560866240521,227.483208933629,8.89044045298036));
#73412=CARTESIAN_POINT('Ctrl Pts',(160.381427271921,227.628317968041,8.83752116456977));
#73413=CARTESIAN_POINT('Ctrl Pts',(161.281026848849,227.32648067205,8.78460187615917));
#73414=CARTESIAN_POINT('Ctrl Pts',(161.84800822259,226.715817786367,8.73168258774858));
#73415=CARTESIAN_POINT('Ctrl Pts',(162.414989596331,226.105154900683,8.67876329933798));
#73416=CARTESIAN_POINT('Ctrl Pts',(162.649352766886,225.185666425308,8.62584401092738));
#73417=CARTESIAN_POINT('Ctrl Pts',(162.443853152016,224.378110268494,8.57292472251678));
#73418=CARTESIAN_POINT('Ctrl Pts',(162.238353537146,223.570554111679,8.52000543410618));
#73419=CARTESIAN_POINT('Ctrl Pts',(161.592991136852,222.874930273426,8.46708614569558));
#73420=CARTESIAN_POINT('Ctrl Pts',(160.803083772819,222.60955620844,8.41416685728498));
#73421=CARTESIAN_POINT('Ctrl Pts',(160.013176408786,222.344182143455,8.36124756887439));
#73422=CARTESIAN_POINT('Ctrl Pts',(159.078724081015,222.509057851738,8.30832828046379));
#73423=CARTESIAN_POINT('Ctrl Pts',(158.427332156319,223.02873621242,8.2554089920532));
#73424=CARTESIAN_POINT('Ctrl Pts',(157.841310791749,223.49626215267,8.20780042886612));
#73425=CARTESIAN_POINT('Ctrl Pts',(157.484387417167,224.250951446125,8.16019186567904));
#73426=CARTESIAN_POINT('Ctrl Pts',(157.479288468299,225.001430882652,8.11258330249197));
#73427=CARTESIAN_POINT('Ctrl Pts',(157.480251844254,224.998100046348,8.387416697508));
#73428=CARTESIAN_POINT('Ctrl Pts',(157.479224600539,224.875762222609,8.39516974436504));
#73429=CARTESIAN_POINT('Ctrl Pts',(157.487364195317,224.753561644012,8.40292279122209));
#73430=CARTESIAN_POINT('Ctrl Pts',(157.505142185515,224.632779749063,8.41067583807914));
#73431=CARTESIAN_POINT('Ctrl Pts',(157.626487845874,223.808369417042,8.46359512648974));
#73432=CARTESIAN_POINT('Ctrl Pts',(158.196876488464,223.050054104809,8.51651441490034));
#73433=CARTESIAN_POINT('Ctrl Pts',(158.955298281651,222.704838884332,8.56943370331093));
#73434=CARTESIAN_POINT('Ctrl Pts',(159.713720074839,222.359623663855,8.62235299172153));
#73435=CARTESIAN_POINT('Ctrl Pts',(160.660175018623,222.427508535133,8.67527228013213));
#73436=CARTESIAN_POINT('Ctrl Pts',(161.361565349338,222.877429382405,8.72819156854273));
#73437=CARTESIAN_POINT('Ctrl Pts',(162.062955680054,223.327350229677,8.78111085695333));
#73438=CARTESIAN_POINT('Ctrl Pts',(162.519281397699,224.159307052943,8.83403014536392));
#73439=CARTESIAN_POINT('Ctrl Pts',(162.521727862853,224.992596426233,8.88694943377452));
#73440=CARTESIAN_POINT('Ctrl Pts',(162.524174328007,225.825885799524,8.93986872218511));
#73441=CARTESIAN_POINT('Ctrl Pts',(162.072741540669,226.660507722839,8.99278801059571));
#73442=CARTESIAN_POINT('Ctrl Pts',(161.374005135449,227.114539220481,9.04570729900631));
#73443=CARTESIAN_POINT('Ctrl Pts',(160.67526873023,227.568570718123,9.09862658741691));
#73444=CARTESIAN_POINT('Ctrl Pts',(159.729228707127,227.642011790091,9.15154587582751));
#73445=CARTESIAN_POINT('Ctrl Pts',(158.968792962114,227.301255803297,9.2044651642381));
#73446=CARTESIAN_POINT('Ctrl Pts',(158.2083572171,226.960499816503,9.2573844526487));
#73447=CARTESIAN_POINT('Ctrl Pts',(157.633525750175,226.205546770946,9.3103037410593));
#73448=CARTESIAN_POINT('Ctrl Pts',(157.5073414293,225.38186316543,9.3632230294699));
#73449=CARTESIAN_POINT('Ctrl Pts',(157.488111757962,225.256339131133,9.3712875854826));
#73450=CARTESIAN_POINT('Ctrl Pts',(157.479301369843,225.12921891334,9.3793521414953));
#73451=CARTESIAN_POINT('Ctrl Pts',(157.480388031054,225.001947791586,9.387416697508));
#73452=CARTESIAN_POINT('Origin',(160.,225.,10.));
#73453=CARTESIAN_POINT('',(157.486356032508,225.000662446517,10.387416697508));
#73454=CARTESIAN_POINT('',(157.484060754376,224.997857937859,10.112583302492));
#73455=CARTESIAN_POINT('',(157.4825,225.,10.));
#73456=CARTESIAN_POINT('Ctrl Pts',(157.484060754376,224.997857937859,10.112583302492));
#73457=CARTESIAN_POINT('Ctrl Pts',(157.488797168304,225.583104362717,10.0756373715289));
#73458=CARTESIAN_POINT('Ctrl Pts',(157.692267651195,226.171320282162,10.0386914405659));
#73459=CARTESIAN_POINT('Ctrl Pts',(158.06545542551,226.617622439287,10.0017455096029));
#73460=CARTESIAN_POINT('Ctrl Pts',(158.599988754229,227.256880727156,9.94882622119231));
#73461=CARTESIAN_POINT('Ctrl Pts',(159.482715739494,227.604987350972,9.89590693278172));
#73462=CARTESIAN_POINT('Ctrl Pts',(160.309700530204,227.502648726522,9.84298764437112));
#73463=CARTESIAN_POINT('Ctrl Pts',(161.136685320915,227.400310102072,9.79006835596053));
#73464=CARTESIAN_POINT('Ctrl Pts',(161.90792791707,226.847526229355,9.73714906754993));
#73465=CARTESIAN_POINT('Ctrl Pts',(162.270507721834,226.097250997659,9.68422977913933));
#73466=CARTESIAN_POINT('Ctrl Pts',(162.633087526598,225.346975765962,9.63131049072873));
#73467=CARTESIAN_POINT('Ctrl Pts',(162.587004539971,224.399209175285,9.57839120231813));
#73468=CARTESIAN_POINT('Ctrl Pts',(162.153346335727,223.687649198886,9.52547191390753));
#73469=CARTESIAN_POINT('Ctrl Pts',(161.719688131483,222.976089222488,9.47255262549694));
#73470=CARTESIAN_POINT('Ctrl Pts',(160.898454709622,222.500735860368,9.41963333708634));
#73471=CARTESIAN_POINT('Ctrl Pts',(160.065442467841,222.479110801686,9.36671404867574));
#73472=CARTESIAN_POINT('Ctrl Pts',(159.232430226059,222.457485743005,9.31379476026514));
#73473=CARTESIAN_POINT('Ctrl Pts',(158.387639164358,222.889588987761,9.26087547185455));
#73474=CARTESIAN_POINT('Ctrl Pts',(157.91764565596,223.577690099652,9.20795618344395));
#73475=CARTESIAN_POINT('Ctrl Pts',(157.635299739686,223.991062913221,9.17616522312662));
#73476=CARTESIAN_POINT('Ctrl Pts',(157.488215899689,224.496823744605,9.14437426280929));
#73477=CARTESIAN_POINT('Ctrl Pts',(157.485838515826,225.001308641677,9.11258330249197));
#73478=CARTESIAN_POINT('Ctrl Pts',(157.480388031054,225.001947791586,9.387416697508));
#73479=CARTESIAN_POINT('Ctrl Pts',(157.486431996492,224.29407099102,9.4322714299059));
#73480=CARTESIAN_POINT('Ctrl Pts',(157.798645056327,223.581525917367,9.4771261623038));
#73481=CARTESIAN_POINT('Ctrl Pts',(158.32717092237,223.112989373578,9.5219808947017));
#73482=CARTESIAN_POINT('Ctrl Pts',(158.950721911137,222.560213352718,9.57490018311229));
#73483=CARTESIAN_POINT('Ctrl Pts',(159.875361063495,222.347075476473,9.62781947152289));
#73484=CARTESIAN_POINT('Ctrl Pts',(160.677973521504,222.571107632822,9.68073875993348));
#73485=CARTESIAN_POINT('Ctrl Pts',(161.480585979514,222.795139789172,9.73365804834408));
#73486=CARTESIAN_POINT('Ctrl Pts',(162.161171743175,223.456341978116,9.78657733675468));
#73487=CARTESIAN_POINT('Ctrl Pts',(162.408294780418,224.252148090994,9.83949662516527));
#73488=CARTESIAN_POINT('Ctrl Pts',(162.655417817662,225.047954203872,9.89241591357587));
#73489=CARTESIAN_POINT('Ctrl Pts',(162.469078128488,225.978364240684,9.94533520198646));
#73490=CARTESIAN_POINT('Ctrl Pts',(161.934544750998,226.617622586879,9.99825449039706));
#73491=CARTESIAN_POINT('Ctrl Pts',(161.400011373508,227.256880933074,10.0511737788077));
#73492=CARTESIAN_POINT('Ctrl Pts',(160.517284307703,227.604987588652,10.1040930672183));
#73493=CARTESIAN_POINT('Ctrl Pts',(159.690299441538,227.502648954864,10.1570123556289));
#73494=CARTESIAN_POINT('Ctrl Pts',(158.863314575373,227.400310321077,10.2099316440395));
#73495=CARTESIAN_POINT('Ctrl Pts',(158.09207190885,226.847526397924,10.26285093245));
#73496=CARTESIAN_POINT('Ctrl Pts',(157.729492071004,226.097251097772,10.3157702208606));
#73497=CARTESIAN_POINT('Ctrl Pts',(157.565861955122,225.758656334653,10.3396523797431));
#73498=CARTESIAN_POINT('Ctrl Pts',(157.485462685781,225.379839233365,10.3635345386255));
#73499=CARTESIAN_POINT('Ctrl Pts',(157.486356032508,225.000662446517,10.387416697508));
#73500=CARTESIAN_POINT('Origin',(160.,225.,10.));
#73501=CARTESIAN_POINT('',(157.482816018711,224.997701707894,11.387416697508));
#73502=CARTESIAN_POINT('',(157.478262151323,224.999954178036,11.112583302492));
#73503=CARTESIAN_POINT('',(157.4825,225.,10.));
#73504=CARTESIAN_POINT('Ctrl Pts',(157.478262555774,224.999954182409,11.112583302492));
#73505=CARTESIAN_POINT('Ctrl Pts',(157.478485401468,225.830795425014,11.0598197686592));
#73506=CARTESIAN_POINT('Ctrl Pts',(157.92931520263,226.661843898407,11.0070562348264));
#73507=CARTESIAN_POINT('Ctrl Pts',(158.625994989915,227.11453902755,10.9542927009937));
#73508=CARTESIAN_POINT('Ctrl Pts',(159.324731331382,227.568570483766,10.9013734125831));
#73509=CARTESIAN_POINT('Ctrl Pts',(160.270771268167,227.642011549034,10.8484541241725));
#73510=CARTESIAN_POINT('Ctrl Pts',(161.031206943798,227.30125559333,10.7955348357619));
#73511=CARTESIAN_POINT('Ctrl Pts',(161.79164261943,226.960499637627,10.7426155473513));
#73512=CARTESIAN_POINT('Ctrl Pts',(162.366474033907,226.205546660952,10.6896962589407));
#73513=CARTESIAN_POINT('Ctrl Pts',(162.492658343269,225.381863130589,10.6367769705301));
#73514=CARTESIAN_POINT('Ctrl Pts',(162.61884265263,224.558179600226,10.5838576821195));
#73515=CARTESIAN_POINT('Ctrl Pts',(162.296379856875,223.665765516174,10.5309383937089));
#73516=CARTESIAN_POINT('Ctrl Pts',(161.672828925001,223.112989545749,10.4780191052983));
#73517=CARTESIAN_POINT('Ctrl Pts',(161.049277993127,222.560213575324,10.4250998168877));
#73518=CARTESIAN_POINT('Ctrl Pts',(160.124638925134,222.347075718526,10.3721805284771));
#73519=CARTESIAN_POINT('Ctrl Pts',(159.322026540355,222.571107854435,10.3192612400665));
#73520=CARTESIAN_POINT('Ctrl Pts',(158.519414155576,222.795139990344,10.2663419516559));
#73521=CARTESIAN_POINT('Ctrl Pts',(157.838828454011,223.456342118959,10.2134226632453));
#73522=CARTESIAN_POINT('Ctrl Pts',(157.591705439315,224.252148159228,10.1605033748347));
#73523=CARTESIAN_POINT('Ctrl Pts',(157.517112897242,224.492357253528,10.1445300173871));
#73524=CARTESIAN_POINT('Ctrl Pts',(157.48201299348,224.744830064544,10.1285566599395));
#73525=CARTESIAN_POINT('Ctrl Pts',(157.484060754376,224.997857937859,10.112583302492));
#73526=CARTESIAN_POINT('Ctrl Pts',(157.486356032508,225.000662446517,10.387416697508));
#73527=CARTESIAN_POINT('Ctrl Pts',(157.487442208375,224.53964024463,10.4164538270362));
#73528=CARTESIAN_POINT('Ctrl Pts',(157.60870260008,224.078086322494,10.4454909565643));
#73529=CARTESIAN_POINT('Ctrl Pts',(157.846653467802,223.687649079147,10.4745280860924));
#73530=CARTESIAN_POINT('Ctrl Pts',(158.280311711613,222.976089037826,10.527447374503));
#73531=CARTESIAN_POINT('Ctrl Pts',(159.101545208403,222.500735632334,10.5803666629136));
#73532=CARTESIAN_POINT('Ctrl Pts',(159.934557526189,222.47911057168,10.6332859513242));
#73533=CARTESIAN_POINT('Ctrl Pts',(160.767569843974,222.457485511025,10.6862052397348));
#73534=CARTESIAN_POINT('Ctrl Pts',(161.612360982755,222.889588795207,10.7391245281454));
#73535=CARTESIAN_POINT('Ctrl Pts',(162.082354534035,223.57768996988,10.792043816556));
#73536=CARTESIAN_POINT('Ctrl Pts',(162.552348085314,224.265791144553,10.8449631049666));
#73537=CARTESIAN_POINT('Ctrl Pts',(162.647544049094,225.209890209716,10.8978823933772));
#73538=CARTESIAN_POINT('Ctrl Pts',(162.324380754219,225.977967451715,10.9508016817878));
#73539=CARTESIAN_POINT('Ctrl Pts',(162.001217459344,226.746044693713,11.0037209701984));
#73540=CARTESIAN_POINT('Ctrl Pts',(161.259694905814,227.338100112547,11.056640258609));
#73541=CARTESIAN_POINT('Ctrl Pts',(160.439133799546,227.483209160198,11.1095595470196));
#73542=CARTESIAN_POINT('Ctrl Pts',(159.618572693277,227.628318207849,11.1624788354302));
#73543=CARTESIAN_POINT('Ctrl Pts',(158.71897303427,227.326480884318,11.2153981238408));
#73544=CARTESIAN_POINT('Ctrl Pts',(158.151991608797,226.715817942918,11.2683174122514));
#73545=CARTESIAN_POINT('Ctrl Pts',(157.726645233492,226.257701932431,11.3080171740036));
#73546=CARTESIAN_POINT('Ctrl Pts',(157.488493693424,225.625781377196,11.3477169357558));
#73547=CARTESIAN_POINT('Ctrl Pts',(157.482816018711,224.997701707894,11.387416697508));
#73548=CARTESIAN_POINT('Origin',(160.,225.,10.));
#73549=CARTESIAN_POINT('',(157.478532268341,225.000747722968,12.387416697508));
#73550=CARTESIAN_POINT('',(157.483927228124,225.002171058717,12.112583302492));
#73551=CARTESIAN_POINT('',(157.4825,225.,10.));
#73552=CARTESIAN_POINT('Ctrl Pts',(157.483927228124,225.002171058717,12.112583302492));
#73553=CARTESIAN_POINT('Ctrl Pts',(157.481884324812,225.250231121536,12.0969214542001));
#73554=CARTESIAN_POINT('Ctrl Pts',(157.515602092607,225.497748009088,12.0812596059081));
#73555=CARTESIAN_POINT('Ctrl Pts',(157.587355737836,225.733697983519,12.0655977576162));
#73556=CARTESIAN_POINT('Ctrl Pts',(157.829801697957,226.530941355735,12.0126784692056));
#73557=CARTESIAN_POINT('Ctrl Pts',(158.506493236424,227.196128332326,11.959759180795));
#73558=CARTESIAN_POINT('Ctrl Pts',(159.307776318542,227.424869365883,11.9068398923844));
#73559=CARTESIAN_POINT('Ctrl Pts',(160.109059400659,227.653610399441,11.8539206039738));
#73560=CARTESIAN_POINT('Ctrl Pts',(161.034934026426,227.445905489964,11.8010013155632));
#73561=CARTESIAN_POINT('Ctrl Pts',(161.661719985296,226.896800399947,11.7480820271526));
#73562=CARTESIAN_POINT('Ctrl Pts',(162.288505944167,226.347695309929,11.695162738742));
#73563=CARTESIAN_POINT('Ctrl Pts',(162.616203236141,225.45719003937,11.6422434503314));
#73564=CARTESIAN_POINT('Ctrl Pts',(162.494857586854,224.632779782569,11.5893241619208));
#73565=CARTESIAN_POINT('Ctrl Pts',(162.373511937567,223.808369525767,11.5364048735102));
#73566=CARTESIAN_POINT('Ctrl Pts',(161.803123347019,223.050054282723,11.4834855850996));
#73567=CARTESIAN_POINT('Ctrl Pts',(161.04470162303,222.704839093743,11.430566296689));
#73568=CARTESIAN_POINT('Ctrl Pts',(160.286279899042,222.359623904763,11.3776470082784));
#73569=CARTESIAN_POINT('Ctrl Pts',(159.339825041612,222.427508769848,11.3247277198678));
#73570=CARTESIAN_POINT('Ctrl Pts',(158.638434774892,222.877429576069,11.2718084314573));
#73571=CARTESIAN_POINT('Ctrl Pts',(157.937044508171,223.32735038229,11.2188891430467));
#73572=CARTESIAN_POINT('Ctrl Pts',(157.480718832161,224.159307129647,11.1659698546361));
#73573=CARTESIAN_POINT('Ctrl Pts',(157.47827236723,224.992596426908,11.1130505662255));
#73574=CARTESIAN_POINT('Ctrl Pts',(157.478265166677,224.995049003778,11.1128948116476));
#73575=CARTESIAN_POINT('Ctrl Pts',(157.478261897948,224.997501592191,11.1127390570698));
#73576=CARTESIAN_POINT('Ctrl Pts',(157.478262555774,224.999954182409,11.112583302492));
#73577=CARTESIAN_POINT('Ctrl Pts',(157.482816018711,224.997701707894,11.387416697508));
#73578=CARTESIAN_POINT('Ctrl Pts',(157.480925423682,224.788558993543,11.4006362241664));
#73579=CARTESIAN_POINT('Ctrl Pts',(157.504811696542,224.579842159362,11.4138557508248));
#73580=CARTESIAN_POINT('Ctrl Pts',(157.556146625006,224.378110211752,11.4270752774832));
#73581=CARTESIAN_POINT('Ctrl Pts',(157.761646258626,223.570553981256,11.4799945658938));
#73582=CARTESIAN_POINT('Ctrl Pts',(158.407008717803,222.874930079534,11.5329138543044));
#73583=CARTESIAN_POINT('Ctrl Pts',(159.196916153907,222.609555990336,11.585833142715));
#73584=CARTESIAN_POINT('Ctrl Pts',(159.986823590012,222.344181901138,11.6387524311256));
#73585=CARTESIAN_POINT('Ctrl Pts',(160.921276003043,222.509057624464,11.6916717195362));
#73586=CARTESIAN_POINT('Ctrl Pts',(161.572667987172,223.028736032562,11.7445910079468));
#73587=CARTESIAN_POINT('Ctrl Pts',(162.224059971301,223.54841444066,11.7975102963574));
#73588=CARTESIAN_POINT('Ctrl Pts',(162.592391526527,224.422895533531,11.850429584768));
#73589=CARTESIAN_POINT('Ctrl Pts',(162.50911414042,225.25201678027,11.9033488731786));
#73590=CARTESIAN_POINT('Ctrl Pts',(162.425836754314,226.081138027009,11.9562681615892));
#73591=CARTESIAN_POINT('Ctrl Pts',(161.890950426876,226.864899427616,12.0091874499998));
#73592=CARTESIAN_POINT('Ctrl Pts',(161.149219131025,227.244651780585,12.0621067384104));
#73593=CARTESIAN_POINT('Ctrl Pts',(160.407487835173,227.624404133553,12.115026026821));
#73594=CARTESIAN_POINT('Ctrl Pts',(159.458911570908,227.600147438883,12.1679453152316));
#73595=CARTESIAN_POINT('Ctrl Pts',(158.737558818107,227.182981559578,12.2208646036422));
#73596=CARTESIAN_POINT('Ctrl Pts',(158.016206065306,226.765815680272,12.2737838920528));
#73597=CARTESIAN_POINT('Ctrl Pts',(157.522076823968,225.955740616332,12.3267031804634));
#73598=CARTESIAN_POINT('Ctrl Pts',(157.481284625214,225.123446701089,12.379622468874));
#73599=CARTESIAN_POINT('Ctrl Pts',(157.479281929328,225.082585172391,12.3822205450853));
#73600=CARTESIAN_POINT('Ctrl Pts',(157.478371923492,225.041670089019,12.3848186212967));
#73601=CARTESIAN_POINT('Ctrl Pts',(157.478532268341,225.000747722968,12.387416697508));
#73602=CARTESIAN_POINT('Origin',(160.,225.,10.));
#73603=CARTESIAN_POINT('',(157.485016106425,225.001823857836,13.387416697508));
#73604=CARTESIAN_POINT('',(157.485914018718,224.998759312188,13.112583302492));
#73605=CARTESIAN_POINT('',(157.4825,225.,10.));
#73606=CARTESIAN_POINT('Ctrl Pts',(157.485914018718,224.998759312188,13.112583302492));
#73607=CARTESIAN_POINT('Ctrl Pts',(157.488141905361,225.4983384767,13.0811038513303));
#73608=CARTESIAN_POINT('Ctrl Pts',(157.632159036081,225.999101383862,13.0496244001686));
#73609=CARTESIAN_POINT('Ctrl Pts',(157.909330069275,226.410058263879,13.018144949007));
#73610=CARTESIAN_POINT('Ctrl Pts',(158.375275100188,227.100907209951,12.9652256605964));
#73611=CARTESIAN_POINT('Ctrl Pts',(159.217514385268,227.537963429135,12.9123063721858));
#73612=CARTESIAN_POINT('Ctrl Pts',(160.050639244222,227.521230004128,12.8593870837752));
#73613=CARTESIAN_POINT('Ctrl Pts',(160.883764103177,227.504496579121,12.8064677953646));
#73614=CARTESIAN_POINT('Ctrl Pts',(161.707774536006,227.033973509921,12.753548506954));
#73615=CARTESIAN_POINT('Ctrl Pts',(162.145603384849,226.324972143744,12.7006292185434));
#73616=CARTESIAN_POINT('Ctrl Pts',(162.583432233691,225.615970777567,12.6477099301328));
#73617=CARTESIAN_POINT('Ctrl Pts',(162.635079498548,224.668491114411,12.5947906417222));
#73618=CARTESIAN_POINT('Ctrl Pts',(162.276911392035,223.916099829509,12.5418713533116));
#73619=CARTESIAN_POINT('Ctrl Pts',(161.918743285523,223.163708544606,12.488952064901));
#73620=CARTESIAN_POINT('Ctrl Pts',(161.150759807641,222.606405637956,12.4360327764904));
#73621=CARTESIAN_POINT('Ctrl Pts',(160.324390182769,222.499212908684,12.3831134880798));
#73622=CARTESIAN_POINT('Ctrl Pts',(159.498020557896,222.392020179412,12.3301941996692));
#73623=CARTESIAN_POINT('Ctrl Pts',(158.613264786033,222.734937627517,12.2772749112586));
#73624=CARTESIAN_POINT('Ctrl Pts',(158.074987090988,223.37104623549,12.224355622848));
#73625=CARTESIAN_POINT('Ctrl Pts',(157.696016594735,223.818893874458,12.1870981827293));
#73626=CARTESIAN_POINT('Ctrl Pts',(157.488787021577,224.412069382079,12.1498407426106));
#73627=CARTESIAN_POINT('Ctrl Pts',(157.483927228124,225.002171058717,12.112583302492));
#73628=CARTESIAN_POINT('Ctrl Pts',(157.478532268341,225.000747722968,12.387416697508));
#73629=CARTESIAN_POINT('Ctrl Pts',(157.481637930571,224.208136999396,12.4377379097073));
#73630=CARTESIAN_POINT('Ctrl Pts',(157.886279610186,223.412794219741,12.4880591219065));
#73631=CARTESIAN_POINT('Ctrl Pts',(158.530138644279,222.950933426618,12.5383803341057));
#73632=CARTESIAN_POINT('Ctrl Pts',(159.207240018268,222.465226833938,12.5912996225163));
#73633=CARTESIAN_POINT('Ctrl Pts',(160.148897922415,222.348326415125,12.6442189109269));
#73634=CARTESIAN_POINT('Ctrl Pts',(160.924209718299,222.653725799529,12.6971381993375));
#73635=CARTESIAN_POINT('Ctrl Pts',(161.699521514183,222.959125183933,12.7500574877481));
#73636=CARTESIAN_POINT('Ctrl Pts',(162.308487201802,223.686824371555,12.8029767761587));
#73637=CARTESIAN_POINT('Ctrl Pts',(162.472444094476,224.503828228446,12.8558960645693));
#73638=CARTESIAN_POINT('Ctrl Pts',(162.63640098715,225.320832085337,12.9088153529799));
#73639=CARTESIAN_POINT('Ctrl Pts',(162.355349084878,226.227140611498,12.9617346413905));
#73640=CARTESIAN_POINT('Ctrl Pts',(161.757897732615,226.808027043178,13.0146539298011));
#73641=CARTESIAN_POINT('Ctrl Pts',(161.160446380351,227.388913474857,13.0675732182117));
#73642=CARTESIAN_POINT('Ctrl Pts',(160.246595578096,227.644377812055,13.1204925066223));
#73643=CARTESIAN_POINT('Ctrl Pts',(159.434523434992,227.457519579092,13.1734117950329));
#73644=CARTESIAN_POINT('Ctrl Pts',(158.622451291889,227.27066134613,13.2263310834435));
#73645=CARTESIAN_POINT('Ctrl Pts',(157.912157807938,226.641480543007,13.2792503718541));
#73646=CARTESIAN_POINT('Ctrl Pts',(157.628673267428,225.857890292861,13.3321696602647));
#73647=CARTESIAN_POINT('Ctrl Pts',(157.530021897025,225.585204340136,13.3505853393458));
#73648=CARTESIAN_POINT('Ctrl Pts',(157.483057487382,225.293819259495,13.3690010184269));
#73649=CARTESIAN_POINT('Ctrl Pts',(157.485016106425,225.001823857836,13.387416697508));
#73650=CARTESIAN_POINT('Origin',(160.,225.,10.));
#73651=CARTESIAN_POINT('',(157.485110394447,224.998220537442,14.387416697508));
#73652=CARTESIAN_POINT('',(157.479399062161,224.998500607783,14.112583302492));
#73653=CARTESIAN_POINT('',(157.4825,225.,10.));
#73654=CARTESIAN_POINT('Ctrl Pts',(157.479399062161,224.998500607783,14.112583302492));
#73655=CARTESIAN_POINT('Ctrl Pts',(157.484655142802,225.744155612533,14.0652862484606));
#73656=CARTESIAN_POINT('Ctrl Pts',(157.836334781685,226.494118132385,14.0179891944291));
#73657=CARTESIAN_POINT('Ctrl Pts',(158.415784449147,226.961995452392,13.9706921403977));
#73658=CARTESIAN_POINT('Ctrl Pts',(159.064113709812,227.485489681477,13.9177728519871));
#73659=CARTESIAN_POINT('Ctrl Pts',(159.997581815393,227.655849441756,13.8648535635765));
#73660=CARTESIAN_POINT('Ctrl Pts',(160.789033779131,227.395118110274,13.8119342751659));
#73661=CARTESIAN_POINT('Ctrl Pts',(161.580485742868,227.134386778792,13.7590149867553));
#73662=CARTESIAN_POINT('Ctrl Pts',(162.229921564762,226.442564355549,13.7060956983447));
#73663=CARTESIAN_POINT('Ctrl Pts',(162.440159425482,225.636228767819,13.6531764099341));
#73664=CARTESIAN_POINT('Ctrl Pts',(162.650397286203,224.829893180089,13.6002571215235));
#73665=CARTESIAN_POINT('Ctrl Pts',(162.42143718575,223.909044427871,13.5473378331129));
#73666=CARTESIAN_POINT('Ctrl Pts',(161.85805126159,223.295062882075,13.4944185447023));
#73667=CARTESIAN_POINT('Ctrl Pts',(161.294665337429,222.681081336279,13.4414992562918));
#73668=CARTESIAN_POINT('Ctrl Pts',(160.396853589561,222.373966996905,13.3885799678811));
#73669=CARTESIAN_POINT('Ctrl Pts',(159.575454656156,222.514255379611,13.3356606794705));
#73670=CARTESIAN_POINT('Ctrl Pts',(158.754055722752,222.654543762317,13.28274139106));
#73671=CARTESIAN_POINT('Ctrl Pts',(158.009069603811,223.242234867105,13.2298221026494));
#73672=CARTESIAN_POINT('Ctrl Pts',(157.681401932714,224.008401255977,13.1769028142388));
#73673=CARTESIAN_POINT('Ctrl Pts',(157.548649929596,224.318807596962,13.1554629769898));
#73674=CARTESIAN_POINT('Ctrl Pts',(157.484396662942,224.658508908041,13.1340231397409));
#73675=CARTESIAN_POINT('Ctrl Pts',(157.485914018718,224.998759312188,13.112583302492));
#73676=CARTESIAN_POINT('Ctrl Pts',(157.485016106425,225.001823857836,13.387416697508));
#73677=CARTESIAN_POINT('Ctrl Pts',(157.48868577432,224.454741384228,13.4219203068375));
#73678=CARTESIAN_POINT('Ctrl Pts',(157.664093645276,223.905516454647,13.456423916167));
#73679=CARTESIAN_POINT('Ctrl Pts',(157.993061232263,223.473119844339,13.4909275254965));
#73680=CARTESIAN_POINT('Ctrl Pts',(158.497609334675,222.80993934313,13.5438468139071));
#73681=CARTESIAN_POINT('Ctrl Pts',(159.363381136564,222.42157803788,13.5967661023177));
#73682=CARTESIAN_POINT('Ctrl Pts',(160.19419947841,222.485750054235,13.6496853907283));
#73683=CARTESIAN_POINT('Ctrl Pts',(161.025017820256,222.54992207059,13.7026046791389));
#73684=CARTESIAN_POINT('Ctrl Pts',(161.820882702058,223.06662740855,13.7555239675495));
#73685=CARTESIAN_POINT('Ctrl Pts',(162.217606369553,223.799421715624,13.8084432559601));
#73686=CARTESIAN_POINT('Ctrl Pts',(162.614330037047,224.532216022699,13.8613625443707));
#73687=CARTESIAN_POINT('Ctrl Pts',(162.611912490233,225.481099298887,13.9142818327813));
#73688=CARTESIAN_POINT('Ctrl Pts',(162.211459998486,226.211862575663,13.9672011211919));
#73689=CARTESIAN_POINT('Ctrl Pts',(161.811007506738,226.942625852439,14.0201204096025));
#73690=CARTESIAN_POINT('Ctrl Pts',(161.012520070057,227.455269129802,14.0730396980131));
#73691=CARTESIAN_POINT('Ctrl Pts',(160.181385523768,227.51520685411,14.1259589864237));
#73692=CARTESIAN_POINT('Ctrl Pts',(159.350250977479,227.575144578419,14.1788782748343));
#73693=CARTESIAN_POINT('Ctrl Pts',(158.486469321582,227.182376749673,14.2317975632449));
#73694=CARTESIAN_POINT('Ctrl Pts',(157.985307024831,226.516633918584,14.2847168516555));
#73695=CARTESIAN_POINT('Ctrl Pts',(157.661107083314,226.085967469206,14.3189501336063));
#73696=CARTESIAN_POINT('Ctrl Pts',(157.488654125966,225.541067920259,14.3531834155572));
#73697=CARTESIAN_POINT('Ctrl Pts',(157.485110394447,224.998220537442,14.387416697508));
#73698=CARTESIAN_POINT('Origin',(160.,225.,10.));
#73699=CARTESIAN_POINT('',(157.47858851104,224.999178326175,15.387416697508));
#73700=CARTESIAN_POINT('',(157.481369652601,225.002195372979,15.112583302492));
#73701=CARTESIAN_POINT('',(157.4825,225.,10.));
#73702=CARTESIAN_POINT('Ctrl Pts',(157.481369652601,225.002195372979,15.112583302492));
#73703=CARTESIAN_POINT('Ctrl Pts',(157.479896180238,225.16325630262,15.1023879340014));
#73704=CARTESIAN_POINT('Ctrl Pts',(157.494022383079,225.324059777303,15.0921925655108));
#73705=CARTESIAN_POINT('Ctrl Pts',(157.524685344636,225.481645537413,15.0819971970203));
#73706=CARTESIAN_POINT('Ctrl Pts',(157.683842133094,226.299597953393,15.0290779086097));
#73707=CARTESIAN_POINT('Ctrl Pts',(158.288524381302,227.030860239281,14.9761586201991));
#73708=CARTESIAN_POINT('Ctrl Pts',(159.062029504368,227.340806787434,14.9232393317885));
#73709=CARTESIAN_POINT('Ctrl Pts',(159.835534627433,227.650753335586,14.8703200433779));
#73710=CARTESIAN_POINT('Ctrl Pts',(160.777862625357,227.539384146001,14.8174007549673));
#73711=CARTESIAN_POINT('Ctrl Pts',(161.457804224818,227.057661757645,14.7644814665567));
#73712=CARTESIAN_POINT('Ctrl Pts',(162.137745824278,226.575939369289,14.7115621781461));
#73713=CARTESIAN_POINT('Ctrl Pts',(162.555301025275,225.72386378216,14.6586428897355));
#73714=CARTESIAN_POINT('Ctrl Pts',(162.519396576041,224.891344768175,14.6057236013249));
#73715=CARTESIAN_POINT('Ctrl Pts',(162.483492126808,224.058825754191,14.5528043129143));
#73716=CARTESIAN_POINT('Ctrl Pts',(161.994128027345,223.245863313351,14.4998850245037));
#73717=CARTESIAN_POINT('Ctrl Pts',(161.275237279945,222.824469042599,14.4469657360931));
#73718=CARTESIAN_POINT('Ctrl Pts',(160.556346532544,222.403074771847,14.3940464476825));
#73719=CARTESIAN_POINT('Ctrl Pts',(159.607929137207,222.373248671183,14.3411271592719));
#73720=CARTESIAN_POINT('Ctrl Pts',(158.86398087539,222.748639163685,14.2882078708613));
#73721=CARTESIAN_POINT('Ctrl Pts',(158.120032613574,223.124029656187,14.2352885824507));
#73722=CARTESIAN_POINT('Ctrl Pts',(157.580553485279,223.904636741854,14.1823692940401));
#73723=CARTESIAN_POINT('Ctrl Pts',(157.492409129006,224.733254633634,14.1294500056295));
#73724=CARTESIAN_POINT('Ctrl Pts',(157.483044524056,224.821288394826,14.1238277712503));
#73725=CARTESIAN_POINT('Ctrl Pts',(157.478774268125,224.909864068181,14.1182055368711));
#73726=CARTESIAN_POINT('Ctrl Pts',(157.479399062161,224.998500607783,14.112583302492));
#73727=CARTESIAN_POINT('Ctrl Pts',(157.485110394447,224.998220537442,14.387416697508));
#73728=CARTESIAN_POINT('Ctrl Pts',(157.483176072458,224.70191094853,14.4061027039678));
#73729=CARTESIAN_POINT('Ctrl Pts',(157.531567388157,224.406212791993,14.4247887104275));
#73730=CARTESIAN_POINT('Ctrl Pts',(157.633075457542,224.13003768041,14.4434747168873));
#73731=CARTESIAN_POINT('Ctrl Pts',(157.920549124609,223.347902106756,14.4963940052978));
#73732=CARTESIAN_POINT('Ctrl Pts',(158.634039396345,222.722348792881,14.5493132937084));
#73733=CARTESIAN_POINT('Ctrl Pts',(159.447053138434,222.539630922914,14.602232582119));
#73734=CARTESIAN_POINT('Ctrl Pts',(160.260066880523,222.356913052947,14.6551518705296));
#73735=CARTESIAN_POINT('Ctrl Pts',(161.172604092964,222.617030626888,14.7080711589402));
#73736=CARTESIAN_POINT('Ctrl Pts',(161.767087765287,223.200953848016,14.7609904473508));
#73737=CARTESIAN_POINT('Ctrl Pts',(162.36157143761,223.784877069144,14.8139097357614));
#73738=CARTESIAN_POINT('Ctrl Pts',(162.638001569814,224.692605937458,14.866829024172));
#73739=CARTESIAN_POINT('Ctrl Pts',(162.469883738838,225.508763740667,14.9197483125826));
#73740=CARTESIAN_POINT('Ctrl Pts',(162.301765907862,226.324921543876,14.9726676009932));
#73741=CARTESIAN_POINT('Ctrl Pts',(161.689100113707,227.04950828198,15.0255868894038));
#73742=CARTESIAN_POINT('Ctrl Pts',(160.912242211731,227.350953077867,15.0785061778144));
#73743=CARTESIAN_POINT('Ctrl Pts',(160.135384309754,227.652397873755,15.131425466225));
#73744=CARTESIAN_POINT('Ctrl Pts',(159.194334299958,227.530700727426,15.1843447546356));
#73745=CARTESIAN_POINT('Ctrl Pts',(158.51971664832,227.041550250651,15.2372640430462));
#73746=CARTESIAN_POINT('Ctrl Pts',(157.88166554457,226.578913376491,15.2873149278668));
#73747=CARTESIAN_POINT('Ctrl Pts',(157.481946516999,225.787578007339,15.3373658126874));
#73748=CARTESIAN_POINT('Ctrl Pts',(157.47858851104,224.999178326175,15.387416697508));
#73749=CARTESIAN_POINT('Origin',(160.,225.,10.));
#73750=CARTESIAN_POINT('',(157.482687981659,225.002301033995,16.387416697508));
#73751=CARTESIAN_POINT('',(157.486512950876,225.000116346801,16.112583302492));
#73752=CARTESIAN_POINT('',(157.4825,225.,10.));
#73753=CARTESIAN_POINT('Ctrl Pts',(157.486512950876,225.000116346801,16.112583302492));
#73754=CARTESIAN_POINT('Ctrl Pts',(157.486342648081,225.413188232998,16.0865703311317));
#73755=CARTESIAN_POINT('Ctrl Pts',(157.582487768739,225.826185463148,16.0605573597713));
#73756=CARTESIAN_POINT('Ctrl Pts',(157.775382536625,226.187536192458,16.034544388411));
#73757=CARTESIAN_POINT('Ctrl Pts',(158.167796525526,226.922647272114,15.9816251000004));
#73758=CARTESIAN_POINT('Ctrl Pts',(158.960613637304,227.444016794936,15.9287058115898));
#73759=CARTESIAN_POINT('Ctrl Pts',(159.79104077721,227.513066077522,15.8757865231792));
#73760=CARTESIAN_POINT('Ctrl Pts',(160.621467917115,227.582115360107,15.8228672347686));
#73761=CARTESIAN_POINT('Ctrl Pts',(161.489505085149,227.198844402455,15.769947946358));
#73762=CARTESIAN_POINT('Ctrl Pts',(161.99793849028,226.538637987256,15.7170286579474));
#73763=CARTESIAN_POINT('Ctrl Pts',(162.506371895412,225.878431572058,15.6641093695368));
#73764=CARTESIAN_POINT('Ctrl Pts',(162.65520153764,224.941289699314,15.6111900811262));
#73765=CARTESIAN_POINT('Ctrl Pts',(162.376322975611,224.156048471562,15.5582707927157));
#73766=CARTESIAN_POINT('Ctrl Pts',(162.097444413582,223.370807243811,15.5053515043051));
#73767=CARTESIAN_POINT('Ctrl Pts',(161.390857647295,222.737466661052,15.4524322158944));
#73768=CARTESIAN_POINT('Ctrl Pts',(160.57989676711,222.545843361505,15.3995129274839));
#73769=CARTESIAN_POINT('Ctrl Pts',(159.768935886925,222.354220061959,15.3465936390733));
#73770=CARTESIAN_POINT('Ctrl Pts',(158.853600892841,222.604314045624,15.2936743506627));
#73771=CARTESIAN_POINT('Ctrl Pts',(158.252749060154,223.181682310492,15.2407550622521));
#73772=CARTESIAN_POINT('Ctrl Pts',(157.767656641972,223.647815477689,15.198031142332));
#73773=CARTESIAN_POINT('Ctrl Pts',(157.487544271528,224.327265941386,15.155307222412));
#73774=CARTESIAN_POINT('Ctrl Pts',(157.481369652601,225.002195372979,15.112583302492));
#73775=CARTESIAN_POINT('Ctrl Pts',(157.47858851104,224.999178326175,15.387416697508));
#73776=CARTESIAN_POINT('Ctrl Pts',(157.478396064566,224.953995339222,15.390285101098));
#73777=CARTESIAN_POINT('Ctrl Pts',(157.479505429084,224.908821994265,15.393153504688));
#73778=CARTESIAN_POINT('Ctrl Pts',(157.481946350156,224.863720714323,15.396021908278));
#73779=CARTESIAN_POINT('Ctrl Pts',(157.526978997108,224.031645461992,15.4489411966886));
#73780=CARTESIAN_POINT('Ctrl Pts',(158.025229584489,223.224098764553,15.5018604850992));
#73781=CARTESIAN_POINT('Ctrl Pts',(158.74869865331,222.810613974884,15.5547797735098));
#73782=CARTESIAN_POINT('Ctrl Pts',(159.472167722131,222.397129185214,15.6076990619204));
#73783=CARTESIAN_POINT('Ctrl Pts',(160.42085527239,222.377706303315,15.660618350331));
#73784=CARTESIAN_POINT('Ctrl Pts',(161.160641899746,222.761233239543,15.7135376387416));
#73785=CARTESIAN_POINT('Ctrl Pts',(161.900428527103,223.144760175772,15.7664569271522));
#73786=CARTESIAN_POINT('Ctrl Pts',(162.431314231556,223.931236930129,15.8193762155628));
#73787=CARTESIAN_POINT('Ctrl Pts',(162.51036572518,224.760771755319,15.8722955039734));
#73788=CARTESIAN_POINT('Ctrl Pts',(162.589417218803,225.590306580509,15.925214792384));
#73789=CARTESIAN_POINT('Ctrl Pts',(162.216634501596,226.462899476532,15.9781340807946));
#73790=CARTESIAN_POINT('Ctrl Pts',(161.562602937639,226.979251951253,16.0310533692052));
#73791=CARTESIAN_POINT('Ctrl Pts',(160.908571373682,227.495604425974,16.0839726576158));
#73792=CARTESIAN_POINT('Ctrl Pts',(159.973290962974,227.655716479393,16.1368919460264));
#73793=CARTESIAN_POINT('Ctrl Pts',(159.184746003034,227.386320839163,16.189811234437));
#73794=CARTESIAN_POINT('Ctrl Pts',(158.396201043094,227.116925198932,16.2427305228476));
#73795=CARTESIAN_POINT('Ctrl Pts',(157.754391533921,226.418021865052,16.2956498112582));
#73796=CARTESIAN_POINT('Ctrl Pts',(157.553009494362,225.609428989055,16.3485690996688));
#73797=CARTESIAN_POINT('Ctrl Pts',(157.503731882362,225.41156861334,16.3615182989485));
#73798=CARTESIAN_POINT('Ctrl Pts',(157.480825612644,225.207140390115,16.3744674982282));
#73799=CARTESIAN_POINT('Ctrl Pts',(157.482687981659,225.002301033995,16.387416697508));
#73800=CARTESIAN_POINT('Origin',(160.,225.,10.));
#73801=CARTESIAN_POINT('',(157.486388012783,224.99940538485,17.387416697508));
#73802=CARTESIAN_POINT('',(157.481796636001,224.997743576325,17.112583302492));
#73803=CARTESIAN_POINT('',(157.4825,225.,10.));
#73804=CARTESIAN_POINT('Ctrl Pts',(157.481796636001,224.997743576325,17.112583302492));
#73805=CARTESIAN_POINT('Ctrl Pts',(157.48789794461,225.658848742086,17.0707527282619));
#73806=CARTESIAN_POINT('Ctrl Pts',(157.75518214039,226.324319915578,17.0289221540318));
#73807=CARTESIAN_POINT('Ctrl Pts',(158.222379264903,226.78863903208,16.9870915798018));
#73808=CARTESIAN_POINT('Ctrl Pts',(158.813423969208,227.376042807739,16.9341722913912));
#73809=CARTESIAN_POINT('Ctrl Pts',(159.724418014731,227.641514087453,16.8812530029806));
#73810=CARTESIAN_POINT('Ctrl Pts',(160.538490545154,227.463573217911,16.82833371457));
#73811=CARTESIAN_POINT('Ctrl Pts',(161.352563075576,227.285632348368,16.7754144261594));
#73812=CARTESIAN_POINT('Ctrl Pts',(162.069714090897,226.664279329569,16.7224951377488));
#73813=CARTESIAN_POINT('Ctrl Pts',(162.361775300124,225.883845291148,16.6695758493382));
#73814=CARTESIAN_POINT('Ctrl Pts',(162.653836509352,225.103411252728,16.6166565609276));
#73815=CARTESIAN_POINT('Ctrl Pts',(162.520807912486,224.163896194687,16.563737272517));
#73816=CARTESIAN_POINT('Ctrl Pts',(162.02356339307,223.495222188895,16.5108179841064));
#73817=CARTESIAN_POINT('Ctrl Pts',(161.526318873653,222.826548183103,16.4578986956958));
#73818=CARTESIAN_POINT('Ctrl Pts',(160.664858431685,222.428715229559,16.4049794072852));
#73819=CARTESIAN_POINT('Ctrl Pts',(159.833386348361,222.483771680089,16.3520601188746));
#73820=CARTESIAN_POINT('Ctrl Pts',(159.001914265037,222.538828130619,16.299140830464));
#73821=CARTESIAN_POINT('Ctrl Pts',(158.200430540357,223.046773985221,16.2462215420534));
#73822=CARTESIAN_POINT('Ctrl Pts',(157.795694111028,223.775173230767,16.1933022536428));
#73823=CARTESIAN_POINT('Ctrl Pts',(157.589909660474,224.145521011859,16.1663959365925));
#73824=CARTESIAN_POINT('Ctrl Pts',(157.486689102264,224.57285861524,16.1394896195422));
#73825=CARTESIAN_POINT('Ctrl Pts',(157.486512950876,225.000116346801,16.112583302492));
#73826=CARTESIAN_POINT('Ctrl Pts',(157.482687981659,225.002301033995,16.387416697508));
#73827=CARTESIAN_POINT('Ctrl Pts',(157.488436526714,224.370026624993,16.4273867866388));
#73828=CARTESIAN_POINT('Ctrl Pts',(157.73017123711,223.733835098205,16.4673568757697));
#73829=CARTESIAN_POINT('Ctrl Pts',(158.16075860029,223.274787751828,16.5073269649006));
#73830=CARTESIAN_POINT('Ctrl Pts',(158.730844315724,222.667021808713,16.5602462533112));
#73831=CARTESIAN_POINT('Ctrl Pts',(159.631970316536,222.369772340596,16.6131655417218));
#73832=CARTESIAN_POINT('Ctrl Pts',(160.451781362769,222.519060696911,16.6660848301324));
#73833=CARTESIAN_POINT('Ctrl Pts',(161.271592409001,222.668349053226,16.719004118543));
#73834=CARTESIAN_POINT('Ctrl Pts',(162.010088500653,223.264175233973,16.7719234069535));
#73835=CARTESIAN_POINT('Ctrl Pts',(162.329333840094,224.033889193323,16.8248426953641));
#73836=CARTESIAN_POINT('Ctrl Pts',(162.648579179535,224.803603152672,16.8777619837747));
#73837=CARTESIAN_POINT('Ctrl Pts',(162.548573766764,225.747204890625,16.9306812721853));
#73838=CARTESIAN_POINT('Ctrl Pts',(162.075080077969,226.432902264707,16.9836005605959));
#73839=CARTESIAN_POINT('Ctrl Pts',(161.601586389173,227.118599638789,17.0365198490065));
#73840=CARTESIAN_POINT('Ctrl Pts',(160.754604424353,227.546392649001,17.0894391374171));
#73841=CARTESIAN_POINT('Ctrl Pts',(159.921713111323,227.52052323419,17.1423584258277));
#73842=CARTESIAN_POINT('Ctrl Pts',(159.088821798293,227.49465381938,17.1952777142383));
#73843=CARTESIAN_POINT('Ctrl Pts',(158.270021137053,227.015121979548,17.2481970026489));
#73844=CARTESIAN_POINT('Ctrl Pts',(157.839994299551,226.301361450457,17.3011162910595));
#73845=CARTESIAN_POINT('Ctrl Pts',(157.606232710443,225.913362886245,17.329883093209));
#73846=CARTESIAN_POINT('Ctrl Pts',(157.487353176809,225.456150111532,17.3586498953585));
#73847=CARTESIAN_POINT('Ctrl Pts',(157.486388012783,224.99940538485,17.387416697508));
#73848=CARTESIAN_POINT('Origin',(160.,225.,10.));
#73849=CARTESIAN_POINT('',(157.480508380744,224.998011611683,18.387416697508));
#73850=CARTESIAN_POINT('',(157.479093530148,225.001296842243,18.112583302492));
#73851=CARTESIAN_POINT('',(157.4825,225.,10.));
#73852=CARTESIAN_POINT('Ctrl Pts',(157.479093530148,225.001296842243,18.112583302492));
#73853=CARTESIAN_POINT('Ctrl Pts',(157.478625650357,225.075825676239,18.1078544138028));
#73854=CARTESIAN_POINT('Ctrl Pts',(157.481644355634,225.150316077051,18.1031255251135));
#73855=CARTESIAN_POINT('Ctrl Pts',(157.488273041435,225.224483837494,18.0983966364243));
#73856=CARTESIAN_POINT('Ctrl Pts',(157.562452274396,226.054468504842,18.0454773480137));
#73857=CARTESIAN_POINT('Ctrl Pts',(158.088710854837,226.844048785844,17.9925580596031));
#73858=CARTESIAN_POINT('Ctrl Pts',(158.826232701178,227.231912914062,17.9396387711925));
#73859=CARTESIAN_POINT('Ctrl Pts',(159.563754547518,227.619777042281,17.8867194827819));
#73860=CARTESIAN_POINT('Ctrl Pts',(160.512539659759,227.605925017717,17.8338001943713));
#73861=CARTESIAN_POINT('Ctrl Pts',(161.238424068964,227.196695452017,17.7808809059607));
#73862=CARTESIAN_POINT('Ctrl Pts',(161.964308478168,226.787465886318,17.7279616175501));
#73863=CARTESIAN_POINT('Ctrl Pts',(162.467292184337,225.982858779483,17.6750423291395));
#73864=CARTESIAN_POINT('Ctrl Pts',(162.517209814972,225.151062363695,17.622123040729));
#73865=CARTESIAN_POINT('Ctrl Pts',(162.567127445607,224.319265947907,17.5692037523184));
#73866=CARTESIAN_POINT('Ctrl Pts',(162.163979000708,223.460280223166,17.5162844639078));
#73867=CARTESIAN_POINT('Ctrl Pts',(161.492245219262,222.967177022915,17.4633651754972));
#73868=CARTESIAN_POINT('Ctrl Pts',(160.820511437816,222.474073822664,17.4104458870866));
#73869=CARTESIAN_POINT('Ctrl Pts',(159.880192319824,222.346853146903,17.357526598676));
#73870=CARTESIAN_POINT('Ctrl Pts',(159.10157786626,222.643731182701,17.3046073102654));
#73871=CARTESIAN_POINT('Ctrl Pts',(158.322963412696,222.940609218499,17.2516880218548));
#73872=CARTESIAN_POINT('Ctrl Pts',(157.706053623561,223.661585965856,17.1987687334442));
#73873=CARTESIAN_POINT('Ctrl Pts',(157.533146410537,224.476742475336,17.1458494450336));
#73874=CARTESIAN_POINT('Ctrl Pts',(157.496915411924,224.647550470257,17.134760730853));
#73875=CARTESIAN_POINT('Ctrl Pts',(157.48017926238,224.822493621923,17.1236720166725));
#73876=CARTESIAN_POINT('Ctrl Pts',(157.481796636001,224.997743576325,17.112583302492));
#73877=CARTESIAN_POINT('Ctrl Pts',(157.486388012783,224.99940538485,17.387416697508));
#73878=CARTESIAN_POINT('Ctrl Pts',(157.48557766512,224.615924430704,17.4115691837691));
#73879=CARTESIAN_POINT('Ctrl Pts',(157.567887645435,224.232773413495,17.4357216700302));
#73880=CARTESIAN_POINT('Ctrl Pts',(157.735112625212,223.891193694375,17.4598741562913));
#73881=CARTESIAN_POINT('Ctrl Pts',(158.101510802135,223.142775685731,17.5127934447019));
#73882=CARTESIAN_POINT('Ctrl Pts',(158.875560169744,222.593928886793,17.5657127331125));
#73883=CARTESIAN_POINT('Ctrl Pts',(159.703055776172,222.495805475537,17.6186320215231));
#73884=CARTESIAN_POINT('Ctrl Pts',(160.530551382599,222.397682064281,17.6715513099337));
#73885=CARTESIAN_POINT('Ctrl Pts',(161.411493227846,222.750282040708,17.7244705983443));
#73886=CARTESIAN_POINT('Ctrl Pts',(161.942762292016,223.392255883383,17.7773898867549));
#73887=CARTESIAN_POINT('Ctrl Pts',(162.474031356186,224.034229726058,17.8303091751655));
#73888=CARTESIAN_POINT('Ctrl Pts',(162.65562763928,224.965577434981,17.8832284635761));
#73889=CARTESIAN_POINT('Ctrl Pts',(162.404452787055,225.760113858579,17.9361477519867));
#73890=CARTESIAN_POINT('Ctrl Pts',(162.153277934831,226.554650282177,17.9890670403973));
#73891=CARTESIAN_POINT('Ctrl Pts',(161.46933194729,227.212375420449,18.0419863288079));
#73892=CARTESIAN_POINT('Ctrl Pts',(160.665588284605,227.432315214048,18.0949056172185));
#73893=CARTESIAN_POINT('Ctrl Pts',(159.861844621921,227.652255007647,18.1478249056291));
#73894=CARTESIAN_POINT('Ctrl Pts',(158.938303284093,227.434409456573,18.2007441940397));
#73895=CARTESIAN_POINT('Ctrl Pts',(158.317577205504,226.878462707285,18.2536634824503));
#73896=CARTESIAN_POINT('Ctrl Pts',(157.794616604086,226.410078573941,18.2982478874695));
#73897=CARTESIAN_POINT('Ctrl Pts',(157.48659524579,225.701709124714,18.3428322924888));
#73898=CARTESIAN_POINT('Ctrl Pts',(157.480508380744,224.998011611683,18.387416697508));
#73899=CARTESIAN_POINT('Origin',(160.,225.,10.));
#73900=CARTESIAN_POINT('',(157.480142558574,225.001823580074,19.387416697508));
#73901=CARTESIAN_POINT('',(157.485690591028,225.001427433753,19.112583302492));
#73902=CARTESIAN_POINT('',(157.4825,225.,10.));
#73903=CARTESIAN_POINT('',(161.913465996665,226.635987203375,20.));
#73904=CARTESIAN_POINT('Ctrl Pts',(157.480142558574,225.001823580074,19.387416697508));
#73905=CARTESIAN_POINT('Ctrl Pts',(157.486035875252,224.285086609627,19.4328532664402));
#73906=CARTESIAN_POINT('Ctrl Pts',(157.807332972564,223.563823321433,19.4782898353724));
#73907=CARTESIAN_POINT('Ctrl Pts',(158.347923825584,223.094934991001,19.5237264043046));
#73908=CARTESIAN_POINT('Ctrl Pts',(158.977541860912,222.548827805233,19.5766456927152));
#73909=CARTESIAN_POINT('Ctrl Pts',(159.904629913844,222.345064991681,19.6295649811258));
#73910=CARTESIAN_POINT('Ctrl Pts',(160.704626516463,222.578292344923,19.6824842695364));
#73911=CARTESIAN_POINT('Ctrl Pts',(161.504623119081,222.811519698165,19.735403557947));
#73912=CARTESIAN_POINT('Ctrl Pts',(162.177528271386,223.481737218202,19.7883228463576));
#73913=CARTESIAN_POINT('Ctrl Pts',(162.415731120478,224.278796422505,19.8412421347682));
#73914=CARTESIAN_POINT('Ctrl Pts',(162.653933969571,225.075855626809,19.8941614231788));
#73915=CARTESIAN_POINT('Ctrl Pts',(162.457434515453,225.999756515379,19.9470807115894));
#73916=CARTESIAN_POINT('Ctrl Pts',(161.913465996665,226.635987203375,20.));
#73917=CARTESIAN_POINT('',(158.082847419036,226.638754849416,20.));
#73918=CARTESIAN_POINT('Origin',(160.,225.,20.));
#73919=CARTESIAN_POINT('Ctrl Pts',(158.082843717471,226.638757628308,20.));
#73920=CARTESIAN_POINT('Ctrl Pts',(158.613381501441,227.257451085127,19.948244384658));
#73921=CARTESIAN_POINT('Ctrl Pts',(159.472376079816,227.597124236137,19.896488769316));
#73922=CARTESIAN_POINT('Ctrl Pts',(160.282371283694,227.505771932288,19.844733153974));
#73923=CARTESIAN_POINT('Ctrl Pts',(161.110578416814,227.412365663568,19.7918138655635));
#73924=CARTESIAN_POINT('Ctrl Pts',(161.887558001259,226.868333694107,19.7388945771529));
#73925=CARTESIAN_POINT('Ctrl Pts',(162.258272057625,226.122147391606,19.6859752887423));
#73926=CARTESIAN_POINT('Ctrl Pts',(162.628986113992,225.375961089105,19.6330560003317));
#73927=CARTESIAN_POINT('Ctrl Pts',(162.59343464228,224.427620453564,19.5801367119211));
#73928=CARTESIAN_POINT('Ctrl Pts',(162.167641122797,223.711314725108,19.5272174235105));
#73929=CARTESIAN_POINT('Ctrl Pts',(161.741847603315,222.995008996652,19.4742981350999));
#73930=CARTESIAN_POINT('Ctrl Pts',(160.925812036062,222.510738175281,19.4213788466893));
#73931=CARTESIAN_POINT('Ctrl Pts',(160.093070271787,222.479994334415,19.3684595582787));
#73932=CARTESIAN_POINT('Ctrl Pts',(159.260328507511,222.44925049355,19.3155402698681));
#73933=CARTESIAN_POINT('Ctrl Pts',(158.410880546213,222.87203363319,19.2626209814575));
#73934=CARTESIAN_POINT('Ctrl Pts',(157.93337689175,223.554931319872,19.2097016930469));
#73935=CARTESIAN_POINT('Ctrl Pts',(157.641269245065,223.972686523039,19.1773288961952));
#73936=CARTESIAN_POINT('Ctrl Pts',(157.488352346154,224.48778301533,19.1449560993436));
#73937=CARTESIAN_POINT('Ctrl Pts',(157.485690591028,225.001427433753,19.112583302492));
#73938=CARTESIAN_POINT('Origin',(-160.,225.,10.));
#73939=CARTESIAN_POINT('',(-162.513515873292,225.000575080101,0.387416697508026));
#73940=CARTESIAN_POINT('',(-162.515402535198,224.996259729968,0.112583302491934));
#73941=CARTESIAN_POINT('',(-162.5175,225.,10.));
#73942=CARTESIAN_POINT('',(-161.913465996665,226.635987203375,0.));
#73943=CARTESIAN_POINT('Ctrl Pts',(-162.515402535198,224.996259729968,0.112583302491934));
#73944=CARTESIAN_POINT('Ctrl Pts',(-162.51023742721,225.58895227201,0.0750555349946119));
#73945=CARTESIAN_POINT('Ctrl Pts',(-162.299221828084,226.184803560304,0.0375277674972904));
#73946=CARTESIAN_POINT('Ctrl Pts',(-161.913465996665,226.635987203375,-3.15025783237388E-14));
#73947=CARTESIAN_POINT('',(-158.082847392586,226.638754884714,3.03954323567685E-15));
#73948=CARTESIAN_POINT('Origin',(-160.,225.,0.));
#73949=CARTESIAN_POINT('Ctrl Pts',(-158.082843691308,226.638757663408,2.26599577176544E-15));
#73950=CARTESIAN_POINT('Ctrl Pts',(-158.613381466828,227.257451072063,0.0517556153419928));
#73951=CARTESIAN_POINT('Ctrl Pts',(-159.47237606495,227.597124296558,0.103511230683983));
#73952=CARTESIAN_POINT('Ctrl Pts',(-160.282371286662,227.505772004605,0.155266846025974));
#73953=CARTESIAN_POINT('Ctrl Pts',(-161.110578438016,227.412365748049,0.20818613443657));
#73954=CARTESIAN_POINT('Ctrl Pts',(-161.887558038694,226.868333726363,0.261105422847168));
#73955=CARTESIAN_POINT('Ctrl Pts',(-162.258272100966,226.122147400466,0.314024711257765));
#73956=CARTESIAN_POINT('Ctrl Pts',(-162.429649067526,225.777193804055,0.338488706674519));
#73957=CARTESIAN_POINT('Ctrl Pts',(-162.514202638506,225.38903761854,0.362952702091273));
#73958=CARTESIAN_POINT('Ctrl Pts',(-162.513515873292,225.000575080101,0.387416697508026));
#73959=CARTESIAN_POINT('Origin',(-160.,225.,10.));
#73960=CARTESIAN_POINT('',(-162.517460047887,224.997698761843,1.38741669750802));
#73961=CARTESIAN_POINT('',(-162.521728513626,225.00013531689,1.11258330249193));
#73962=CARTESIAN_POINT('',(-162.5175,225.,10.));
#73963=CARTESIAN_POINT('Ctrl Pts',(-162.521728513626,225.00013531689,1.11258330249193));
#73964=CARTESIAN_POINT('Ctrl Pts',(-162.52173338627,225.006844584385,1.11215722053546));
#73965=CARTESIAN_POINT('Ctrl Pts',(-162.521708943191,225.013553813481,1.11173113857898));
#73966=CARTESIAN_POINT('Ctrl Pts',(-162.521655077588,225.020262804259,1.11130505662251));
#73967=CARTESIAN_POINT('Ctrl Pts',(-162.514964981143,225.853518032503,1.05838576821191));
#73968=CARTESIAN_POINT('Ctrl Pts',(-162.054415170727,226.683097057043,1.00546647980131));
#73969=CARTESIAN_POINT('Ctrl Pts',(-161.35073645221,227.129460505748,0.952547191390717));
#73970=CARTESIAN_POINT('Ctrl Pts',(-160.647057733692,227.575823954453,0.899627902980116));
#73971=CARTESIAN_POINT('Ctrl Pts',(-159.700250107072,227.638971827323,0.846708614569517));
#73972=CARTESIAN_POINT('Ctrl Pts',(-158.943607525641,227.289850001498,0.793789326158917));
#73973=CARTESIAN_POINT('Ctrl Pts',(-158.186964944209,226.940728175673,0.740870037748322));
#73974=CARTESIAN_POINT('Ctrl Pts',(-157.620487407966,226.179336651153,0.687950749337727));
#73975=CARTESIAN_POINT('Ctrl Pts',(-157.503322677412,225.354415202511,0.635031460927131));
#73976=CARTESIAN_POINT('Ctrl Pts',(-157.386157946857,224.529493753869,0.582112172516532));
#73977=CARTESIAN_POINT('Ctrl Pts',(-157.718306021991,223.641042381106,0.529192884105933));
#73978=CARTESIAN_POINT('Ctrl Pts',(-158.347923979622,223.094935196484,0.476273595695335));
#73979=CARTESIAN_POINT('Ctrl Pts',(-158.977541937253,222.548828011861,0.423354307284738));
#73980=CARTESIAN_POINT('Ctrl Pts',(-159.90462977738,222.345065015378,0.370435018874142));
#73981=CARTESIAN_POINT('Ctrl Pts',(-160.704626519453,222.578292509213,0.317515730463546));
#73982=CARTESIAN_POINT('Ctrl Pts',(-161.504623261526,222.811520003047,0.264596442052949));
#73983=CARTESIAN_POINT('Ctrl Pts',(-162.177528905544,223.481737987198,0.211677153642351));
#73984=CARTESIAN_POINT('Ctrl Pts',(-162.415731719026,224.278797115281,0.158757865231754));
#73985=CARTESIAN_POINT('Ctrl Pts',(-162.485012763715,224.510620947525,0.14336634431848));
#73986=CARTESIAN_POINT('Ctrl Pts',(-162.517520936396,224.753174668843,0.127974823405207));
#73987=CARTESIAN_POINT('Ctrl Pts',(-162.515402535198,224.996259729968,0.112583302491934));
#73988=CARTESIAN_POINT('Ctrl Pts',(-162.513515873292,225.000575080101,0.387416697508026));
#73989=CARTESIAN_POINT('Ctrl Pts',(-162.512717062425,224.548734930521,0.415871990501868));
#73990=CARTESIAN_POINT('Ctrl Pts',(-162.396595099549,224.096480310675,0.444327283495711));
#73991=CARTESIAN_POINT('Ctrl Pts',(-162.167641159638,223.711314708389,0.472782576489553));
#73992=CARTESIAN_POINT('Ctrl Pts',(-161.741847632174,222.995008972314,0.525701864900151));
#73993=CARTESIAN_POINT('Ctrl Pts',(-160.925812053378,222.510738130269,0.578621153310749));
#73994=CARTESIAN_POINT('Ctrl Pts',(-160.093070274692,222.479994286021,0.631540441721348));
#73995=CARTESIAN_POINT('Ctrl Pts',(-159.260328496006,222.449250441774,0.684459730131945));
#73996=CARTESIAN_POINT('Ctrl Pts',(-158.410880517429,222.872033595323,0.737379018542543));
#73997=CARTESIAN_POINT('Ctrl Pts',(-157.933376854027,223.554931295734,0.790298306953139));
#73998=CARTESIAN_POINT('Ctrl Pts',(-157.455873190625,224.237828996146,0.843217595363738));
#73999=CARTESIAN_POINT('Ctrl Pts',(-157.350313842398,225.18084124342,0.896136883774334));
#74000=CARTESIAN_POINT('Ctrl Pts',(-157.665030169378,225.952420054605,0.949056172184933));
#74001=CARTESIAN_POINT('Ctrl Pts',(-157.979746496357,226.72399886579,1.00197546059553));
#74002=CARTESIAN_POINT('Ctrl Pts',(-158.714738498543,227.324144240887,1.05489474900613));
#74003=CARTESIAN_POINT('Ctrl Pts',(-159.533660643004,227.478242004204,1.10781403741672));
#74004=CARTESIAN_POINT('Ctrl Pts',(-160.352582787465,227.63233976752,1.16073332582732));
#74005=CARTESIAN_POINT('Ctrl Pts',(-161.255435074201,227.340389919056,1.21365261423792));
#74006=CARTESIAN_POINT('Ctrl Pts',(-161.829078679583,226.735982758477,1.26657190264851));
#74007=CARTESIAN_POINT('Ctrl Pts',(-162.265730077695,226.275914470048,1.30685350093502));
#74008=CARTESIAN_POINT('Ctrl Pts',(-162.511634932737,225.634805536221,1.34713509922152));
#74009=CARTESIAN_POINT('Ctrl Pts',(-162.517460047887,224.997698761843,1.38741669750802));
#74010=CARTESIAN_POINT('Origin',(-160.,225.,10.));
#74011=CARTESIAN_POINT('',(-162.521340736424,225.000905528618,2.38741669750802));
#74012=CARTESIAN_POINT('',(-162.515825293396,225.002114825265,2.11258330249193));
#74013=CARTESIAN_POINT('',(-162.5175,225.,10.));
#74014=CARTESIAN_POINT('Ctrl Pts',(-162.515825293396,225.002114825265,2.11258330249193));
#74015=CARTESIAN_POINT('Ctrl Pts',(-162.517874395793,225.259454350827,2.09633961766571));
#74016=CARTESIAN_POINT('Ctrl Pts',(-162.481551268892,225.516229230468,2.08009593283949));
#74017=CARTESIAN_POINT('Ctrl Pts',(-162.40445263436,225.760113810438,2.06385224801326));
#74018=CARTESIAN_POINT('Ctrl Pts',(-162.153277798076,226.554650183456,2.01093295960267));
#74019=CARTESIAN_POINT('Ctrl Pts',(-161.469331853934,227.21237527946,1.95801367119207));
#74020=CARTESIAN_POINT('Ctrl Pts',(-160.665588242321,227.432315059322,1.90509438278147));
#74021=CARTESIAN_POINT('Ctrl Pts',(-159.861844630708,227.652254839184,1.85217509437087));
#74022=CARTESIAN_POINT('Ctrl Pts',(-158.938303351623,227.434409302904,1.79925580596027));
#74023=CARTESIAN_POINT('Ctrl Pts',(-158.317577312389,226.878462588484,1.74633651754968));
#74024=CARTESIAN_POINT('Ctrl Pts',(-157.696851273154,226.322515874064,1.69341722913908));
#74025=CARTESIAN_POINT('Ctrl Pts',(-157.37894047377,225.428467981504,1.64049794072848));
#74026=CARTESIAN_POINT('Ctrl Pts',(-157.509319984736,224.605439307191,1.58757865231788));
#74027=CARTESIAN_POINT('Ctrl Pts',(-157.639699495703,223.782410632878,1.53465936390729));
#74028=CARTESIAN_POINT('Ctrl Pts',(-158.21836931702,223.030401176814,1.48174007549669));
#74029=CARTESIAN_POINT('Ctrl Pts',(-158.980532027786,222.693521947342,1.42882078708609));
#74030=CARTESIAN_POINT('Ctrl Pts',(-159.742694738552,222.356642717871,1.37590149867549));
#74031=CARTESIAN_POINT('Ctrl Pts',(-160.688350338767,222.434893714993,1.3229822102649));
#74032=CARTESIAN_POINT('Ctrl Pts',(-161.384762947637,222.892484929529,1.2700629218543));
#74033=CARTESIAN_POINT('Ctrl Pts',(-162.075568360043,223.346391828462,1.21756971540018));
#74034=CARTESIAN_POINT('Ctrl Pts',(-162.52112820495,224.173554987853,1.16507650894606));
#74035=CARTESIAN_POINT('Ctrl Pts',(-162.521728513626,225.00013531689,1.11258330249193));
#74036=CARTESIAN_POINT('Ctrl Pts',(-162.517460047887,224.997698761843,1.38741669750802));
#74037=CARTESIAN_POINT('Ctrl Pts',(-162.51928758213,224.797816971322,1.40005438763212));
#74038=CARTESIAN_POINT('Ctrl Pts',(-162.497484365141,224.598329108395,1.41269207775621));
#74039=CARTESIAN_POINT('Ctrl Pts',(-162.450526967693,224.404949370306,1.42532976788031));
#74040=CARTESIAN_POINT('Ctrl Pts',(-162.253896726394,223.595187615409,1.47824905629091));
#74041=CARTESIAN_POINT('Ctrl Pts',(-161.616201319768,222.892528578311,1.5311683447015));
#74042=CARTESIAN_POINT('Ctrl Pts',(-160.829251631713,222.618507639709,1.5840876331121));
#74043=CARTESIAN_POINT('Ctrl Pts',(-160.042301943657,222.344486701107,1.6370069215227));
#74044=CARTESIAN_POINT('Ctrl Pts',(-159.106097974171,222.499103861,1.68992620993329));
#74045=CARTESIAN_POINT('Ctrl Pts',(-158.449045928806,223.011606975551,1.74284549834389));
#74046=CARTESIAN_POINT('Ctrl Pts',(-157.791993883441,223.524110090102,1.79576478675449));
#74047=CARTESIAN_POINT('Ctrl Pts',(-157.414093762197,224.39449915931,1.84868407516509));
#74048=CARTESIAN_POINT('Ctrl Pts',(-157.488272996495,225.224483841496,1.90160336357569));
#74049=CARTESIAN_POINT('Ctrl Pts',(-157.562452230793,226.054468523682,1.95452265198628));
#74050=CARTESIAN_POINT('Ctrl Pts',(-158.088710820631,226.844048818846,2.00744194039688));
#74051=CARTESIAN_POINT('Ctrl Pts',(-158.826232680166,227.231912954014,2.06036122880748));
#74052=CARTESIAN_POINT('Ctrl Pts',(-159.563754539701,227.619777089181,2.11328051721807));
#74053=CARTESIAN_POINT('Ctrl Pts',(-160.512539668932,227.605925064353,2.16619980562867));
#74054=CARTESIAN_POINT('Ctrl Pts',(-161.23842409113,227.196695491326,2.21911909403927));
#74055=CARTESIAN_POINT('Ctrl Pts',(-161.964308513328,226.787465918299,2.27203838244987));
#74056=CARTESIAN_POINT('Ctrl Pts',(-162.467292228493,225.982858797072,2.32495767086046));
#74057=CARTESIAN_POINT('Ctrl Pts',(-162.517209860019,225.1510623664,2.37787695927106));
#74058=CARTESIAN_POINT('Ctrl Pts',(-162.520209403617,225.101079833544,2.38105687201672));
#74059=CARTESIAN_POINT('Ctrl Pts',(-162.521573020035,225.05099912576,2.38423678476237));
#74060=CARTESIAN_POINT('Ctrl Pts',(-162.521340736424,225.000905528618,2.38741669750802));
#74061=CARTESIAN_POINT('Origin',(-160.,225.,10.));
#74062=CARTESIAN_POINT('',(-162.514783952421,225.001726236531,3.38741669750803));
#74063=CARTESIAN_POINT('',(-162.514230407831,224.998633683133,3.11258330249194));
#74064=CARTESIAN_POINT('',(-162.5175,225.,10.));
#74065=CARTESIAN_POINT('Ctrl Pts',(-162.514230407831,224.998633683133,3.11258330249194));
#74066=CARTESIAN_POINT('Ctrl Pts',(-162.511723050653,225.507373485165,3.08052201479596));
#74067=CARTESIAN_POINT('Ctrl Pts',(-162.361947303449,226.01747067327,3.04846072709999));
#74068=CARTESIAN_POINT('Ctrl Pts',(-162.075079946186,226.432902173709,3.01639943940401));
#74069=CARTESIAN_POINT('Ctrl Pts',(-161.601586287461,227.118599504242,2.96348015099342));
#74070=CARTESIAN_POINT('Ctrl Pts',(-160.75460437643,227.546392487277,2.91056086258282));
#74071=CARTESIAN_POINT('Ctrl Pts',(-159.921713116295,227.520523074114,2.85764157417222));
#74072=CARTESIAN_POINT('Ctrl Pts',(-159.08882185616,227.494653660951,2.80472228576163));
#74073=CARTESIAN_POINT('Ctrl Pts',(-158.270021246919,227.01512185159,2.75180299735103));
#74074=CARTESIAN_POINT('Ctrl Pts',(-157.839994436728,226.30136136782,2.69888370894043));
#74075=CARTESIAN_POINT('Ctrl Pts',(-157.409967626536,225.58760088405,2.64596442052983));
#74076=CARTESIAN_POINT('Ctrl Pts',(-157.368714615394,224.639611725872,2.59304513211924));
#74077=CARTESIAN_POINT('Ctrl Pts',(-157.735112769049,223.891193764775,2.54012584370864));
#74078=CARTESIAN_POINT('Ctrl Pts',(-158.101510922704,223.142775803678,2.48720655529804));
#74079=CARTESIAN_POINT('Ctrl Pts',(-158.875560241156,222.593929039663,2.43428726688744));
#74080=CARTESIAN_POINT('Ctrl Pts',(-159.70305579503,222.495805634607,2.38136797847684));
#74081=CARTESIAN_POINT('Ctrl Pts',(-160.530551348904,222.39768222955,2.32844869006625));
#74082=CARTESIAN_POINT('Ctrl Pts',(-161.411493138199,222.750282183452,2.27552940165565));
#74083=CARTESIAN_POINT('Ctrl Pts',(-161.942762168634,223.392255985419,2.22261011324505));
#74084=CARTESIAN_POINT('Ctrl Pts',(-162.310957073405,223.837174603557,2.18593450966068));
#74085=CARTESIAN_POINT('Ctrl Pts',(-162.511198752803,224.421083949139,2.14925890607631));
#74086=CARTESIAN_POINT('Ctrl Pts',(-162.515825293396,225.002114825265,2.11258330249193));
#74087=CARTESIAN_POINT('Ctrl Pts',(-162.521340736424,225.000905528618,2.38741669750802));
#74088=CARTESIAN_POINT('Ctrl Pts',(-162.517707416043,224.217354391848,2.43715607317297));
#74089=CARTESIAN_POINT('Ctrl Pts',(-162.123614648384,223.430649691751,2.48689544883791));
#74090=CARTESIAN_POINT('Ctrl Pts',(-161.492245245968,222.967176986533,2.53663482450285));
#74091=CARTESIAN_POINT('Ctrl Pts',(-160.820511452501,222.474073777457,2.58955411291345));
#74092=CARTESIAN_POINT('Ctrl Pts',(-159.880192317679,222.346853099421,2.64247340132405));
#74093=CARTESIAN_POINT('Ctrl Pts',(-159.101577850181,222.643731140533,2.69539268973465));
#74094=CARTESIAN_POINT('Ctrl Pts',(-158.322963382683,222.940609181644,2.74831197814524));
#74095=CARTESIAN_POINT('Ctrl Pts',(-157.706053582508,223.661585941903,2.80123126655584));
#74096=CARTESIAN_POINT('Ctrl Pts',(-157.533146366389,224.476742465972,2.85415055496644));
#74097=CARTESIAN_POINT('Ctrl Pts',(-157.36023915027,225.291898990041,2.90706984337704));
#74098=CARTESIAN_POINT('Ctrl Pts',(-157.631334518208,226.201235277919,2.95998913178763));
#74099=CARTESIAN_POINT('Ctrl Pts',(-158.22237923309,226.788639064091,3.01290842019823));
#74100=CARTESIAN_POINT('Ctrl Pts',(-158.813423947973,227.376042850262,3.06582770860883));
#74101=CARTESIAN_POINT('Ctrl Pts',(-159.7244180098,227.641514134727,3.11874699701942));
#74102=CARTESIAN_POINT('Ctrl Pts',(-160.538490554791,227.463573261999,3.17166628543002));
#74103=CARTESIAN_POINT('Ctrl Pts',(-161.352563099782,227.285632389272,3.22458557384062));
#74104=CARTESIAN_POINT('Ctrl Pts',(-162.069714127937,226.664279359353,3.27750486225122));
#74105=CARTESIAN_POINT('Ctrl Pts',(-162.361775342391,225.883845306966,3.33042415066182));
#74106=CARTESIAN_POINT('Ctrl Pts',(-162.466622509632,225.603676987581,3.34942166627722));
#74107=CARTESIAN_POINT('Ctrl Pts',(-162.516686611797,225.303007245379,3.36841918189262));
#74108=CARTESIAN_POINT('Ctrl Pts',(-162.514783952421,225.001726236531,3.38741669750803));
#74109=CARTESIAN_POINT('Origin',(-160.,225.,10.));
#74110=CARTESIAN_POINT('',(-162.515095448041,224.998127113865,4.38741669750803));
#74111=CARTESIAN_POINT('',(-162.520804111367,224.998630441702,4.11258330249194));
#74112=CARTESIAN_POINT('',(-162.5175,225.,10.));
#74113=CARTESIAN_POINT('Ctrl Pts',(-162.520804111367,224.998630441702,4.11258330249194));
#74114=CARTESIAN_POINT('Ctrl Pts',(-162.515852785931,225.753298255826,4.06470441192622));
#74115=CARTESIAN_POINT('Ctrl Pts',(-162.154339889845,226.512080349843,4.01682552136049));
#74116=CARTESIAN_POINT('Ctrl Pts',(-161.562602838402,226.979251825556,3.96894663079477));
#74117=CARTESIAN_POINT('Ctrl Pts',(-160.908571315981,227.495604267485,3.91602734238417));
#74118=CARTESIAN_POINT('Ctrl Pts',(-159.973290964671,227.655716310735,3.86310805397357));
#74119=CARTESIAN_POINT('Ctrl Pts',(-159.184746054809,227.386320687613,3.81018876556298));
#74120=CARTESIAN_POINT('Ctrl Pts',(-158.396201144947,227.116925064492,3.75726947715238));
#74121=CARTESIAN_POINT('Ctrl Pts',(-157.754391676534,226.418021774998,3.70435018874178));
#74122=CARTESIAN_POINT('Ctrl Pts',(-157.553009649764,225.609428950352,3.65143090033119));
#74123=CARTESIAN_POINT('Ctrl Pts',(-157.351627622994,224.800836125707,3.59851161192059));
#74124=CARTESIAN_POINT('Ctrl Pts',(-157.590673037867,223.88255376591,3.54559232350999));
#74125=CARTESIAN_POINT('Ctrl Pts',(-158.160758717096,223.274787861392,3.49267303509939));
#74126=CARTESIAN_POINT('Ctrl Pts',(-158.730844396324,222.667021956874,3.43975374668879));
#74127=CARTESIAN_POINT('Ctrl Pts',(-159.631970339908,222.369772507636,3.3868344582782));
#74128=CARTESIAN_POINT('Ctrl Pts',(-160.451781334077,222.51906085447,3.3339151698676));
#74129=CARTESIAN_POINT('Ctrl Pts',(-161.271592328245,222.668349201303,3.28099588145701));
#74130=CARTESIAN_POINT('Ctrl Pts',(-162.010088372997,223.264175344208,3.22807659304641));
#74131=CARTESIAN_POINT('Ctrl Pts',(-162.329333692164,224.033889254676,3.17515730463581));
#74132=CARTESIAN_POINT('Ctrl Pts',(-162.455163409367,224.337270002544,3.15429930392119));
#74133=CARTESIAN_POINT('Ctrl Pts',(-162.515861610493,224.667664594961,3.13344130320656));
#74134=CARTESIAN_POINT('Ctrl Pts',(-162.514230407831,224.998633683133,3.11258330249194));
#74135=CARTESIAN_POINT('Ctrl Pts',(-162.514783952421,225.001726236531,3.38741669750803));
#74136=CARTESIAN_POINT('Ctrl Pts',(-162.511386582976,224.463761897586,3.42133847030322));
#74137=CARTESIAN_POINT('Ctrl Pts',(-162.342301953927,223.923848637976,3.45526024309842));
#74138=CARTESIAN_POINT('Ctrl Pts',(-162.023563429284,223.495222161964,3.48918201589361));
#74139=CARTESIAN_POINT('Ctrl Pts',(-161.526318900968,222.826548144206,3.54210130430421));
#74140=CARTESIAN_POINT('Ctrl Pts',(-160.664858443584,222.428715183543,3.5950205927148));
#74141=CARTESIAN_POINT('Ctrl Pts',(-159.833386345379,222.483771635058,3.6479398811254));
#74142=CARTESIAN_POINT('Ctrl Pts',(-159.001914247175,222.538828086573,3.700859169536));
#74143=CARTESIAN_POINT('Ctrl Pts',(-158.200430508151,223.046773950265,3.7537784579466));
#74144=CARTESIAN_POINT('Ctrl Pts',(-157.795694071579,223.775173208847,3.80669774635719));
#74145=CARTESIAN_POINT('Ctrl Pts',(-157.390957635008,224.503572467428,3.85961703476779));
#74146=CARTESIAN_POINT('Ctrl Pts',(-157.382968500889,225.452425120899,3.91253632317839));
#74147=CARTESIAN_POINT('Ctrl Pts',(-157.775382496813,226.18753621371,3.96545561158898));
#74148=CARTESIAN_POINT('Ctrl Pts',(-158.167796492737,226.922647306522,4.01837489999958));
#74149=CARTESIAN_POINT('Ctrl Pts',(-158.960613618703,227.444016838676,4.07129418841018));
#74150=CARTESIAN_POINT('Ctrl Pts',(-159.79104077347,227.513066122497,4.12421347682078));
#74151=CARTESIAN_POINT('Ctrl Pts',(-160.621467928238,227.582115406317,4.17713276523138));
#74152=CARTESIAN_POINT('Ctrl Pts',(-161.489505111806,227.198844441806,4.23005205364197));
#74153=CARTESIAN_POINT('Ctrl Pts',(-161.997938526036,226.538638014792,4.28297134205257));
#74154=CARTESIAN_POINT('Ctrl Pts',(-162.332432244487,226.104294211776,4.31778646053772));
#74155=CARTESIAN_POINT('Ctrl Pts',(-162.511282100761,225.550087079639,4.35260157902287));
#74156=CARTESIAN_POINT('Ctrl Pts',(-162.515095448041,224.998127113865,4.38741669750803));
#74157=CARTESIAN_POINT('Origin',(-160.,225.,10.));
#74158=CARTESIAN_POINT('',(-162.521526373637,224.999338730952,5.38741669750803));
#74159=CARTESIAN_POINT('',(-162.518352818028,225.002238051842,5.11258330249194));
#74160=CARTESIAN_POINT('',(-162.5175,225.,10.));
#74161=CARTESIAN_POINT('Ctrl Pts',(-162.518352818028,225.002238051842,5.11258330249194));
#74162=CARTESIAN_POINT('Ctrl Pts',(-162.519921653123,225.172538844406,5.10180609746706));
#74163=CARTESIAN_POINT('Ctrl Pts',(-162.504121385855,225.342550222057,5.09102889244219));
#74164=CARTESIAN_POINT('Ctrl Pts',(-162.469883581982,225.508763708357,5.08025168741732));
#74165=CARTESIAN_POINT('Ctrl Pts',(-162.301765761683,226.324921459734,5.02733239900672));
#74166=CARTESIAN_POINT('Ctrl Pts',(-161.689100006436,227.049508151821,4.97441311059612));
#74167=CARTESIAN_POINT('Ctrl Pts',(-160.912242153797,227.350952928564,4.92149382218553));
#74168=CARTESIAN_POINT('Ctrl Pts',(-160.135384301157,227.652397705307,4.86857453377493));
#74169=CARTESIAN_POINT('Ctrl Pts',(-159.194334351124,227.530700566708,4.81565524536433));
#74170=CARTESIAN_POINT('Ctrl Pts',(-158.51971674233,227.041550120997,4.76273595695374));
#74171=CARTESIAN_POINT('Ctrl Pts',(-157.845099133535,226.552399675287,4.70981666854314));
#74172=CARTESIAN_POINT('Ctrl Pts',(-157.43691386598,225.695795922466,4.65689738013254));
#74173=CARTESIAN_POINT('Ctrl Pts',(-157.481946510071,224.863720722978,4.60397809172194));
#74174=CARTESIAN_POINT('Ctrl Pts',(-157.526979154163,224.03164552349,4.55105880331134));
#74175=CARTESIAN_POINT('Ctrl Pts',(-158.025229709902,223.224098877336,4.49813951490075));
#74176=CARTESIAN_POINT('Ctrl Pts',(-158.748698732777,222.810614113926,4.44522022649015));
#74177=CARTESIAN_POINT('Ctrl Pts',(-159.472167755651,222.397129350516,4.39230093807955));
#74178=CARTESIAN_POINT('Ctrl Pts',(-160.420855245662,222.37770646985,4.33938164966895));
#74179=CARTESIAN_POINT('Ctrl Pts',(-161.160641826037,222.761233381722,4.28646236125835));
#74180=CARTESIAN_POINT('Ctrl Pts',(-161.900428406411,223.144760293593,4.23354307284776));
#74181=CARTESIAN_POINT('Ctrl Pts',(-162.43131407715,223.931236998003,4.18062378443716));
#74182=CARTESIAN_POINT('Ctrl Pts',(-162.510365565753,224.760771770512,4.12770449602657));
#74183=CARTESIAN_POINT('Ctrl Pts',(-162.517894974495,224.839782380918,4.12266409818169));
#74184=CARTESIAN_POINT('Ctrl Pts',(-162.521325356737,224.919183612861,4.11762370033681));
#74185=CARTESIAN_POINT('Ctrl Pts',(-162.520804111367,224.998630441702,4.11258330249194));
#74186=CARTESIAN_POINT('Ctrl Pts',(-162.515095448041,224.998127113865,4.38741669750803));
#74187=CARTESIAN_POINT('Ctrl Pts',(-162.517078422397,224.711103043656,4.40552086743347));
#74188=CARTESIAN_POINT('Ctrl Pts',(-162.471729912629,224.424686627928,4.42362503735892));
#74189=CARTESIAN_POINT('Ctrl Pts',(-162.376323018138,224.156048456458,4.44172920728436));
#74190=CARTESIAN_POINT('Ctrl Pts',(-162.097444451118,223.370807214654,4.49464849569496));
#74191=CARTESIAN_POINT('Ctrl Pts',(-161.390857672187,222.737466620561,4.54756778410556));
#74192=CARTESIAN_POINT('Ctrl Pts',(-160.579896777488,222.545843317585,4.60048707251616));
#74193=CARTESIAN_POINT('Ctrl Pts',(-159.768935882789,222.354220014609,4.65340636092675));
#74194=CARTESIAN_POINT('Ctrl Pts',(-158.853600872324,222.60431400275,4.70632564933735));
#74195=CARTESIAN_POINT('Ctrl Pts',(-158.252749028884,223.181682277951,4.75924493774795));
#74196=CARTESIAN_POINT('Ctrl Pts',(-157.651897185444,223.759050553152,4.81216422615854));
#74197=CARTESIAN_POINT('Ctrl Pts',(-157.365528509029,224.663693115414,4.86508351456914));
#74198=CARTESIAN_POINT('Ctrl Pts',(-157.524685300337,225.481645546033,4.91800280297974));
#74199=CARTESIAN_POINT('Ctrl Pts',(-157.683842091644,226.299597976651,4.97092209139034));
#74200=CARTESIAN_POINT('Ctrl Pts',(-158.288524350673,227.030860275626,5.02384137980094));
#74201=CARTESIAN_POINT('Ctrl Pts',(-159.062029487582,227.340806829325,5.07676066821153));
#74202=CARTESIAN_POINT('Ctrl Pts',(-159.83553462449,227.650753383024,5.12967995662213));
#74203=CARTESIAN_POINT('Ctrl Pts',(-160.777862639279,227.539384191447,5.18259924503273));
#74204=CARTESIAN_POINT('Ctrl Pts',(-161.457804250907,227.05766179447,5.23551853344333));
#74205=CARTESIAN_POINT('Ctrl Pts',(-162.108366554241,226.596753935934,5.28615125479823));
#74206=CARTESIAN_POINT('Ctrl Pts',(-162.518727269286,225.796806298301,5.33678397615313));
#74207=CARTESIAN_POINT('Ctrl Pts',(-162.521526373637,224.999338730952,5.38741669750803));
#74208=CARTESIAN_POINT('Origin',(-160.,225.,10.));
#74209=CARTESIAN_POINT('',(-162.517037158453,225.002292268554,6.38741669750803));
#74210=CARTESIAN_POINT('',(-162.513482688453,224.999964780132,6.11258330249194));
#74211=CARTESIAN_POINT('',(-162.5175,225.,10.));
#74212=CARTESIAN_POINT('Ctrl Pts',(-162.513482688453,224.999964780132,6.11258330249194));
#74213=CARTESIAN_POINT('Ctrl Pts',(-162.513429987392,225.422277783558,6.08598849459732));
#74214=CARTESIAN_POINT('Ctrl Pts',(-162.412708906025,225.844614406147,6.05939368670269));
#74215=CARTESIAN_POINT('Ctrl Pts',(-162.211459858042,226.2118624987,6.03279887880807));
#74216=CARTESIAN_POINT('Ctrl Pts',(-161.811007391726,226.942625729067,5.97987959039748));
#74217=CARTESIAN_POINT('Ctrl Pts',(-161.012520005755,227.455268973874,5.92696030198688));
#74218=CARTESIAN_POINT('Ctrl Pts',(-160.181385512249,227.515206694376,5.87404101357628));
#74219=CARTESIAN_POINT('Ctrl Pts',(-159.350251018743,227.575144414878,5.82112172516568));
#74220=CARTESIAN_POINT('Ctrl Pts',(-158.486469417702,227.182376611076,5.76820243675509));
#74221=CARTESIAN_POINT('Ctrl Pts',(-157.985307152779,226.516633822266,5.71528314834449));
#74222=CARTESIAN_POINT('Ctrl Pts',(-157.484144887856,225.850891033457,5.66236385993389));
#74223=CARTESIAN_POINT('Ctrl Pts',(-157.34560195905,224.912173259641,5.60944457152329));
#74224=CARTESIAN_POINT('Ctrl Pts',(-157.63307560786,224.130037735659,5.5565252831127));
#74225=CARTESIAN_POINT('Ctrl Pts',(-157.920549256669,223.347902211677,5.5036059947021));
#74226=CARTESIAN_POINT('Ctrl Pts',(-158.634039483094,222.722348937529,5.4506867062915));
#74227=CARTESIAN_POINT('Ctrl Pts',(-159.44705317355,222.539631079166,5.3977674178809));
#74228=CARTESIAN_POINT('Ctrl Pts',(-160.260066864006,222.356913220803,5.3448481294703));
#74229=CARTESIAN_POINT('Ctrl Pts',(-161.172604018495,222.617030778224,5.29192884105971));
#74230=CARTESIAN_POINT('Ctrl Pts',(-161.767087653063,223.200953962269,5.23900955264911));
#74231=CARTESIAN_POINT('Ctrl Pts',(-162.24050253924,223.665959071973,5.19686746926338));
#74232=CARTESIAN_POINT('Ctrl Pts',(-162.512218205276,224.336311201209,5.15472538587766));
#74233=CARTESIAN_POINT('Ctrl Pts',(-162.518352818028,225.002238051842,5.11258330249194));
#74234=CARTESIAN_POINT('Ctrl Pts',(-162.521526373637,224.999338730952,5.38741669750803));
#74235=CARTESIAN_POINT('Ctrl Pts',(-162.521652780823,224.963325200202,5.38970326456372));
#74236=CARTESIAN_POINT('Ctrl Pts',(-162.520948001254,224.927316727341,5.39198983161942));
#74237=CARTESIAN_POINT('Ctrl Pts',(-162.519396621129,224.891344766231,5.39427639867511));
#74238=CARTESIAN_POINT('Ctrl Pts',(-162.483492171253,224.058825737347,5.44719568708571));
#74239=CARTESIAN_POINT('Ctrl Pts',(-161.994128063033,223.245863281958,5.50011497549631));
#74240=CARTESIAN_POINT('Ctrl Pts',(-161.275237302767,222.824469003665,5.55303426390691));
#74241=CARTESIAN_POINT('Ctrl Pts',(-160.556346542501,222.403074725371,5.60595355231751));
#74242=CARTESIAN_POINT('Ctrl Pts',(-159.60792913019,222.373248624174,5.65887284072811));
#74243=CARTESIAN_POINT('Ctrl Pts',(-158.863980855059,222.748639123394,5.7117921291387));
#74244=CARTESIAN_POINT('Ctrl Pts',(-158.120032579929,223.124029622614,5.7647114175493));
#74245=CARTESIAN_POINT('Ctrl Pts',(-157.580553441979,223.904636722252,5.81763070595989));
#74246=CARTESIAN_POINT('Ctrl Pts',(-157.492409084129,224.733254628861,5.87054999437049));
#74247=CARTESIAN_POINT('Ctrl Pts',(-157.404264726278,225.56187253547,5.92346928278109));
#74248=CARTESIAN_POINT('Ctrl Pts',(-157.767455148527,226.43850124905,5.97638857119169));
#74249=CARTESIAN_POINT('Ctrl Pts',(-158.415784420795,226.961995487504,6.02930785960229));
#74250=CARTESIAN_POINT('Ctrl Pts',(-159.064113693063,227.485489725958,6.08222714801289));
#74251=CARTESIAN_POINT('Ctrl Pts',(-159.99758181535,227.655849489286,6.13514643642348));
#74252=CARTESIAN_POINT('Ctrl Pts',(-160.789033793252,227.395118153138,6.18806572483408));
#74253=CARTESIAN_POINT('Ctrl Pts',(-161.580485771153,227.13438681699,6.24098501324468));
#74254=CARTESIAN_POINT('Ctrl Pts',(-162.22992160467,226.442564381366,6.29390430165527));
#74255=CARTESIAN_POINT('Ctrl Pts',(-162.440159469152,225.636228779205,6.34682359006587));
#74256=CARTESIAN_POINT('Ctrl Pts',(-162.493915597763,225.430055260273,6.36035462587993));
#74257=CARTESIAN_POINT('Ctrl Pts',(-162.51895767859,225.21639505705,6.37388566169398));
#74258=CARTESIAN_POINT('Ctrl Pts',(-162.517037158453,225.002292268554,6.38741669750803));
#74259=CARTESIAN_POINT('Origin',(-160.,225.,10.));
#74260=CARTESIAN_POINT('',(-162.513684921802,224.999260124652,7.38741669750803));
#74261=CARTESIAN_POINT('',(-162.518482076879,224.99778042495,7.11258330249194));
#74262=CARTESIAN_POINT('',(-162.5175,225.,10.));
#74263=CARTESIAN_POINT('Ctrl Pts',(-162.518482076879,224.99778042495,7.11258330249194));
#74264=CARTESIAN_POINT('Ctrl Pts',(-162.512325196575,225.667890476128,7.07017089172757));
#74265=CARTESIAN_POINT('Ctrl Pts',(-162.236727766197,226.342472815229,7.0277584809632));
#74266=CARTESIAN_POINT('Ctrl Pts',(-161.757897620975,226.808026928355,6.98534607019882));
#74267=CARTESIAN_POINT('Ctrl Pts',(-161.160446306655,227.388913323143,6.93242678178823));
#74268=CARTESIAN_POINT('Ctrl Pts',(-160.246595562436,227.644377644117,6.87950749337763));
#74269=CARTESIAN_POINT('Ctrl Pts',(-159.434523470905,227.457519423022,6.82658820496703));
#74270=CARTESIAN_POINT('Ctrl Pts',(-158.622451379374,227.270661201926,6.77366891655644));
#74271=CARTESIAN_POINT('Ctrl Pts',(-157.912157940531,226.641480438761,6.72074962814584));
#74272=CARTESIAN_POINT('Ctrl Pts',(-157.628673418025,225.857890238379,6.66783033973525));
#74273=CARTESIAN_POINT('Ctrl Pts',(-157.345188895519,225.074300037998,6.61491105132465));
#74274=CARTESIAN_POINT('Ctrl Pts',(-157.48851328935,224.1363004004,6.56199176291404));
#74275=CARTESIAN_POINT('Ctrl Pts',(-157.993061359719,223.473119941308,6.50907247450345));
#74276=CARTESIAN_POINT('Ctrl Pts',(-158.497609430088,222.809939482215,6.45615318609285));
#74277=CARTESIAN_POINT('Ctrl Pts',(-159.363381176994,222.421578201629,6.40323389768225));
#74278=CARTESIAN_POINT('Ctrl Pts',(-160.194199466077,222.485750213908,6.35031460927166));
#74279=CARTESIAN_POINT('Ctrl Pts',(-161.02501775516,222.549922226188,6.29739532086106));
#74280=CARTESIAN_POINT('Ctrl Pts',(-161.820882586419,223.066627531333,6.24447603245046));
#74281=CARTESIAN_POINT('Ctrl Pts',(-162.217606228718,223.79942179187,6.19155674403986));
#74282=CARTESIAN_POINT('Ctrl Pts',(-162.41495475901,224.163947257217,6.16523226352389));
#74283=CARTESIAN_POINT('Ctrl Pts',(-162.513534853826,224.581944447954,6.13890778300791));
#74284=CARTESIAN_POINT('Ctrl Pts',(-162.513482688453,224.999964780132,6.11258330249194));
#74285=CARTESIAN_POINT('Ctrl Pts',(-162.517037158453,225.002292268554,6.38741669750803));
#74286=CARTESIAN_POINT('Ctrl Pts',(-162.511446608453,224.379048428925,6.42680495010458));
#74287=CARTESIAN_POINT('Ctrl Pts',(-162.277383983428,223.752054269524,6.46619320270112));
#74288=CARTESIAN_POINT('Ctrl Pts',(-161.858051294842,223.295062851563,6.50558145529767));
#74289=CARTESIAN_POINT('Ctrl Pts',(-161.294665360598,222.681081294779,6.55850074370826));
#74290=CARTESIAN_POINT('Ctrl Pts',(-160.396853596663,222.373966949908,6.61142003211886));
#74291=CARTESIAN_POINT('Ctrl Pts',(-159.575454648558,222.514255335125,6.66433932052946));
#74292=CARTESIAN_POINT('Ctrl Pts',(-158.754055700454,222.654543720342,6.71725860894005));
#74293=CARTESIAN_POINT('Ctrl Pts',(-158.009069568181,223.242234835647,6.77017789735065));
#74294=CARTESIAN_POINT('Ctrl Pts',(-157.681401891219,224.008401238231,6.82309718576125));
#74295=CARTESIAN_POINT('Ctrl Pts',(-157.353734214258,224.774567640816,6.87601647417185));
#74296=CARTESIAN_POINT('Ctrl Pts',(-157.443384992608,225.719209330679,6.92893576258244));
#74297=CARTESIAN_POINT('Ctrl Pts',(-157.90933003186,226.410058289114,6.98185505099304));
#74298=CARTESIAN_POINT('Ctrl Pts',(-158.375275071111,227.100907247549,7.03477433940364));
#74299=CARTESIAN_POINT('Ctrl Pts',(-159.217514371264,227.537963474556,7.08769362781424));
#74300=CARTESIAN_POINT('Ctrl Pts',(-160.050639245129,227.521230049249,7.14061291622484));
#74301=CARTESIAN_POINT('Ctrl Pts',(-160.883764118993,227.504496623942,7.19353220463543));
#74302=CARTESIAN_POINT('Ctrl Pts',(-161.707774566569,227.033973546322,7.24645149304603));
#74303=CARTESIAN_POINT('Ctrl Pts',(-162.145603423247,226.324972167456,7.29937078145663));
#74304=CARTESIAN_POINT('Ctrl Pts',(-162.388420008767,225.931765344016,7.32871942014043));
#74305=CARTESIAN_POINT('Ctrl Pts',(-162.51245763957,225.465209080798,7.35806805882423));
#74306=CARTESIAN_POINT('Ctrl Pts',(-162.513684921802,224.999260124652,7.38741669750803));
#74307=CARTESIAN_POINT('Origin',(-160.,225.,10.));
#74308=CARTESIAN_POINT('',(-162.519747970937,224.998100046487,8.38741669750803));
#74309=CARTESIAN_POINT('',(-162.520711601608,225.001430882692,8.11258330249194));
#74310=CARTESIAN_POINT('',(-162.5175,225.,10.));
#74311=CARTESIAN_POINT('Ctrl Pts',(-162.520711601608,225.001430882692,8.11258330249194));
#74312=CARTESIAN_POINT('Ctrl Pts',(-162.521280388299,225.085146708523,8.10727257726842));
#74313=CARTESIAN_POINT('Ctrl Pts',(-162.517471298417,225.168810149606,8.10196185204489));
#74314=CARTESIAN_POINT('Ctrl Pts',(-162.509113981073,225.252016764264,8.09665112682137));
#74315=CARTESIAN_POINT('Ctrl Pts',(-162.425836600256,226.081137958348,8.04373183841077));
#74316=CARTESIAN_POINT('Ctrl Pts',(-161.890950306787,226.864899309181,7.99081255000018));
#74317=CARTESIAN_POINT('Ctrl Pts',(-161.149219058041,227.244651638032,7.93789326158958));
#74318=CARTESIAN_POINT('Ctrl Pts',(-160.407487809295,227.624403966884,7.88497397317899));
#74319=CARTESIAN_POINT('Ctrl Pts',(-159.458911605272,227.600147273754,7.83205468476839));
#74320=CARTESIAN_POINT('Ctrl Pts',(-158.737558898282,227.182981420942,7.77913539635779));
#74321=CARTESIAN_POINT('Ctrl Pts',(-158.016206191292,226.76581556813,7.72621610794719));
#74322=CARTESIAN_POINT('Ctrl Pts',(-157.522076981334,225.955740555636,7.67329681953659));
#74323=CARTESIAN_POINT('Ctrl Pts',(-157.481284785171,225.123446693249,7.620377531126));
#74324=CARTESIAN_POINT('Ctrl Pts',(-157.440492589007,224.291152830862,7.5674582427154));
#74325=CARTESIAN_POINT('Ctrl Pts',(-157.853037406638,223.436640118583,7.5145389543048));
#74326=CARTESIAN_POINT('Ctrl Pts',(-158.530138737626,222.950933556749,7.46161966589421));
#74327=CARTESIAN_POINT('Ctrl Pts',(-159.207240068613,222.465226994915,7.40870037748361));
#74328=CARTESIAN_POINT('Ctrl Pts',(-160.148897912959,222.348326583526,7.35578108907301));
#74329=CARTESIAN_POINT('Ctrl Pts',(-160.924209659605,222.653725948535,7.30286180066241));
#74330=CARTESIAN_POINT('Ctrl Pts',(-161.69952140625,222.959125313544,7.24994251225181));
#74331=CARTESIAN_POINT('Ctrl Pts',(-162.308487055195,223.686824454951,7.19702322384122));
#74332=CARTESIAN_POINT('Ctrl Pts',(-162.472443937457,224.503828259956,7.14410393543062));
#74333=CARTESIAN_POINT('Ctrl Pts',(-162.504996810954,224.666040551042,7.13359705778439));
#74334=CARTESIAN_POINT('Ctrl Pts',(-162.520007328259,224.831773254163,7.12309018013817));
#74335=CARTESIAN_POINT('Ctrl Pts',(-162.518482076879,224.99778042495,7.11258330249194));
#74336=CARTESIAN_POINT('Ctrl Pts',(-162.513684921802,224.999260124652,7.38741669750803));
#74337=CARTESIAN_POINT('Ctrl Pts',(-162.51467058386,224.625044483707,7.41098734723483));
#74338=CARTESIAN_POINT('Ctrl Pts',(-162.436442208547,224.251220562561,7.43455799696162));
#74339=CARTESIAN_POINT('Ctrl Pts',(-162.276911432784,223.91609981011,7.45812864668842));
#74340=CARTESIAN_POINT('Ctrl Pts',(-161.918743319861,223.163708511743,7.51104793509902));
#74341=CARTESIAN_POINT('Ctrl Pts',(-161.150759828235,222.606405595119,7.56396722350962));
#74342=CARTESIAN_POINT('Ctrl Pts',(-160.324390188574,222.499212863929,7.61688651192021));
#74343=CARTESIAN_POINT('Ctrl Pts',(-159.498020548912,222.392020132738,7.66980580033081));
#74344=CARTESIAN_POINT('Ctrl Pts',(-158.613264761216,222.734937586981,7.72272508874141));
#74345=CARTESIAN_POINT('Ctrl Pts',(-158.074987056538,223.371046206338,7.775644377152));
#74346=CARTESIAN_POINT('Ctrl Pts',(-157.536709351859,224.007154825695,7.8285636655626));
#74347=CARTESIAN_POINT('Ctrl Pts',(-157.3449097302,224.936454610167,7.88148295397319));
#74348=CARTESIAN_POINT('Ctrl Pts',(-157.587355694659,225.73369799665,7.93440224238379));
#74349=CARTESIAN_POINT('Ctrl Pts',(-157.829801659118,226.530941383133,7.98732153079439));
#74350=CARTESIAN_POINT('Ctrl Pts',(-158.506493209696,227.196128371629,8.04024081920499));
#74351=CARTESIAN_POINT('Ctrl Pts',(-159.307776306153,227.42486940928,8.09316010761559));
#74352=CARTESIAN_POINT('Ctrl Pts',(-160.109059402611,227.653610446931,8.14607939602619));
#74353=CARTESIAN_POINT('Ctrl Pts',(-161.034934044948,227.445905533737,8.19899868443678));
#74354=CARTESIAN_POINT('Ctrl Pts',(-161.661720015035,226.896800433892,8.25191797284738));
#74355=CARTESIAN_POINT('Ctrl Pts',(-162.196677445069,226.428143081861,8.29708421440093));
#74356=CARTESIAN_POINT('Ctrl Pts',(-162.513763648225,225.710792668463,8.34225045595448));
#74357=CARTESIAN_POINT('Ctrl Pts',(-162.519747970937,224.998100046487,8.38741669750803));
#74358=CARTESIAN_POINT('Origin',(-160.,225.,10.));
#74359=CARTESIAN_POINT('',(-162.519611784148,225.001947791443,9.38741669750804));
#74360=CARTESIAN_POINT('',(-162.514161553899,225.001308641714,9.11258330249194));
#74361=CARTESIAN_POINT('',(-162.5175,225.,10.));
#74362=CARTESIAN_POINT('Ctrl Pts',(-162.514161553899,225.001308641714,9.11258330249194));
#74363=CARTESIAN_POINT('Ctrl Pts',(-162.515741567435,225.33659020014,9.09145497439867));
#74364=CARTESIAN_POINT('Ctrl Pts',(-162.45340538931,225.671308184112,9.0703266463054));
#74365=CARTESIAN_POINT('Ctrl Pts',(-162.324380606603,225.977967389606,9.04919831821213));
#74366=CARTESIAN_POINT('Ctrl Pts',(-162.001217332251,226.746044582826,8.99627902980153));
#74367=CARTESIAN_POINT('Ctrl Pts',(-161.259694825814,227.33809996406,8.94335974139093));
#74368=CARTESIAN_POINT('Ctrl Pts',(-160.439133771658,227.483209002496,8.89044045298033));
#74369=CARTESIAN_POINT('Ctrl Pts',(-159.618572717501,227.628318040932,8.83752116456974));
#74370=CARTESIAN_POINT('Ctrl Pts',(-158.718973115625,227.326480736569,8.78460187615914));
#74371=CARTESIAN_POINT('Ctrl Pts',(-158.15199172616,226.715817833951,8.73168258774854));
#74372=CARTESIAN_POINT('Ctrl Pts',(-157.585010336694,226.105154931332,8.67876329933794));
#74373=CARTESIAN_POINT('Ctrl Pts',(-157.35064715964,225.185666430457,8.62584401092735));
#74374=CARTESIAN_POINT('Ctrl Pts',(-157.556146780209,224.378110251247,8.57292472251675));
#74375=CARTESIAN_POINT('Ctrl Pts',(-157.761646400778,223.570554072037,8.52000543410616));
#74376=CARTESIAN_POINT('Ctrl Pts',(-158.40700881897,222.874930214492,8.46708614569555));
#74377=CARTESIAN_POINT('Ctrl Pts',(-159.196916204909,222.609556142147,8.41416685728496));
#74378=CARTESIAN_POINT('Ctrl Pts',(-159.986823590848,222.344182069802,8.36124756887436));
#74379=CARTESIAN_POINT('Ctrl Pts',(-160.921275944535,222.509057782657,8.30832828046377));
#74380=CARTESIAN_POINT('Ctrl Pts',(-161.572667887295,223.028736157752,8.25540899205317));
#74381=CARTESIAN_POINT('Ctrl Pts',(-162.158689268117,223.496262110967,8.20780042886609));
#74382=CARTESIAN_POINT('Ctrl Pts',(-162.515612652598,224.250951425351,8.16019186567902));
#74383=CARTESIAN_POINT('Ctrl Pts',(-162.520711601608,225.001430882692,8.11258330249194));
#74384=CARTESIAN_POINT('Ctrl Pts',(-162.519747970937,224.998100046487,8.38741669750803));
#74385=CARTESIAN_POINT('Ctrl Pts',(-162.520775214578,224.875762231721,8.39516974436508));
#74386=CARTESIAN_POINT('Ctrl Pts',(-162.512635620397,224.753561662087,8.40292279122213));
#74387=CARTESIAN_POINT('Ctrl Pts',(-162.494857631502,224.632779775997,8.41067583807918));
#74388=CARTESIAN_POINT('Ctrl Pts',(-162.373511980044,223.808369504441,8.46359512648977));
#74389=CARTESIAN_POINT('Ctrl Pts',(-161.803123379288,223.050054247826,8.51651441490037));
#74390=CARTESIAN_POINT('Ctrl Pts',(-161.044701641726,222.704839052668,8.56943370331096));
#74391=CARTESIAN_POINT('Ctrl Pts',(-160.286279904165,222.35962385751,8.62235299172156));
#74392=CARTESIAN_POINT('Ctrl Pts',(-159.339825029797,222.42750872381,8.67527228013216));
#74393=CARTESIAN_POINT('Ctrl Pts',(-158.638434750524,222.877429538083,8.72819156854276));
#74394=CARTESIAN_POINT('Ctrl Pts',(-157.937044471252,223.327350352356,8.78111085695335));
#74395=CARTESIAN_POINT('Ctrl Pts',(-157.480718787075,224.159307114602,8.83403014536395));
#74396=CARTESIAN_POINT('Ctrl Pts',(-157.4782723221,224.992596426776,8.88694943377455));
#74397=CARTESIAN_POINT('Ctrl Pts',(-157.475825857125,225.82588573895,8.93986872218515));
#74398=CARTESIAN_POINT('Ctrl Pts',(-157.927258611353,226.660507601051,8.99278801059575));
#74399=CARTESIAN_POINT('Ctrl Pts',(-158.625994965325,227.114539065393,9.04570729900634));
#74400=CARTESIAN_POINT('Ctrl Pts',(-159.324731319297,227.568570529734,9.09862658741694));
#74401=CARTESIAN_POINT('Ctrl Pts',(-160.270771273013,227.642011596316,9.15154587582754));
#74402=CARTESIAN_POINT('Ctrl Pts',(-161.031206962253,227.301255634514,9.20446516423813));
#74403=CARTESIAN_POINT('Ctrl Pts',(-161.791642651494,226.960499672712,9.25738445264873));
#74404=CARTESIAN_POINT('Ctrl Pts',(-162.366474076259,226.205546682527,9.31030374105933));
#74405=CARTESIAN_POINT('Ctrl Pts',(-162.492658387878,225.381863137423,9.36322302946993));
#74406=CARTESIAN_POINT('Ctrl Pts',(-162.511888057807,225.256339112332,9.37128758548263));
#74407=CARTESIAN_POINT('Ctrl Pts',(-162.520698445279,225.129218903863,9.37935214149533));
#74408=CARTESIAN_POINT('Ctrl Pts',(-162.519611784148,225.001947791443,9.38741669750804));
#74409=CARTESIAN_POINT('Origin',(-160.,225.,10.));
#74410=CARTESIAN_POINT('',(-162.513643783132,225.000662446468,10.387416697508));
#74411=CARTESIAN_POINT('',(-162.515939315398,224.997857937799,10.1125833024919));
#74412=CARTESIAN_POINT('',(-162.5175,225.,10.));
#74413=CARTESIAN_POINT('Ctrl Pts',(-162.515939315398,224.997857937799,10.1125833024919));
#74414=CARTESIAN_POINT('Ctrl Pts',(-162.511202901338,225.583104378889,10.0756373715289));
#74415=CARTESIAN_POINT('Ctrl Pts',(-162.307732412804,226.171320314646,10.0386914405659));
#74416=CARTESIAN_POINT('Ctrl Pts',(-161.93454462814,226.617622484148,10.0017455096029));
#74417=CARTESIAN_POINT('Ctrl Pts',(-161.400011284597,227.256880789745,9.94882622119229));
#74418=CARTESIAN_POINT('Ctrl Pts',(-160.517284274851,227.604987423216,9.89590693278168));
#74419=CARTESIAN_POINT('Ctrl Pts',(-159.690299461207,227.502648795927,9.84298764437109));
#74420=CARTESIAN_POINT('Ctrl Pts',(-158.863314647562,227.400310168639,9.79006835596049));
#74421=CARTESIAN_POINT('Ctrl Pts',(-158.092072030018,226.847526280592,9.7371490675499));
#74422=CARTESIAN_POINT('Ctrl Pts',(-157.729492215198,226.097251028089,9.6842297791393));
#74423=CARTESIAN_POINT('Ctrl Pts',(-157.366912400379,225.346975775584,9.6313104907287));
#74424=CARTESIAN_POINT('Ctrl Pts',(-157.412995388284,224.399209158623,9.5783912023181));
#74425=CARTESIAN_POINT('Ctrl Pts',(-157.846653604555,223.687649162491,9.5254719139075));
#74426=CARTESIAN_POINT('Ctrl Pts',(-158.280311820826,222.976089166359,9.4725526254969));
#74427=CARTESIAN_POINT('Ctrl Pts',(-159.101545265462,222.500735791056,9.41963333708631));
#74428=CARTESIAN_POINT('Ctrl Pts',(-159.934557530345,222.479110731775,9.36671404867571));
#74429=CARTESIAN_POINT('Ctrl Pts',(-160.767569795228,222.457485672494,9.31379476026512));
#74430=CARTESIAN_POINT('Ctrl Pts',(-161.612360880358,222.889588929234,9.26087547185452));
#74431=CARTESIAN_POINT('Ctrl Pts',(-162.082354401789,223.577690060207,9.20795618344392));
#74432=CARTESIAN_POINT('Ctrl Pts',(-162.364700325894,223.991062885241,9.17616522312659));
#74433=CARTESIAN_POINT('Ctrl Pts',(-162.51178416997,224.49682373065,9.14437426280927));
#74434=CARTESIAN_POINT('Ctrl Pts',(-162.514161553899,225.001308641714,9.11258330249194));
#74435=CARTESIAN_POINT('Ctrl Pts',(-162.519611784148,225.001947791443,9.38741669750804));
#74436=CARTESIAN_POINT('Ctrl Pts',(-162.513567819153,224.294071042795,9.43227142990593));
#74437=CARTESIAN_POINT('Ctrl Pts',(-162.201354782218,223.581526021403,9.47712616230383));
#74438=CARTESIAN_POINT('Ctrl Pts',(-161.672828954939,223.112989511979,9.52198089470172));
#74439=CARTESIAN_POINT('Ctrl Pts',(-161.049278011905,222.560213531661,9.57490018311232));
#74440=CARTESIAN_POINT('Ctrl Pts',(-160.124638927364,222.347075671048,9.62781947152292));
#74441=CARTESIAN_POINT('Ctrl Pts',(-159.322026528221,222.571107810967,9.68073875993352));
#74442=CARTESIAN_POINT('Ctrl Pts',(-158.519414129078,222.795139950885,9.73365804834411));
#74443=CARTESIAN_POINT('Ctrl Pts',(-157.838828415334,223.456342091334,9.78657733675471));
#74444=CARTESIAN_POINT('Ctrl Pts',(-157.591705396215,224.252148145844,9.8394966251653));
#74445=CARTESIAN_POINT('Ctrl Pts',(-157.344582377097,225.047954200355,9.8924159135759));
#74446=CARTESIAN_POINT('Ctrl Pts',(-157.530922052604,225.978364168927,9.9453352019865));
#74447=CARTESIAN_POINT('Ctrl Pts',(-158.065455390889,226.617622468237,9.9982544903971));
#74448=CARTESIAN_POINT('Ctrl Pts',(-158.599988729174,227.256880767546,10.0511737788077));
#74449=CARTESIAN_POINT('Ctrl Pts',(-159.482715730237,227.604987397592,10.1040930672183));
#74450=CARTESIAN_POINT('Ctrl Pts',(-160.309700535747,227.50264877131,10.1570123556289));
#74451=CARTESIAN_POINT('Ctrl Pts',(-161.136685341257,227.400310145029,10.2099316440395));
#74452=CARTESIAN_POINT('Ctrl Pts',(-161.907927951215,226.847526262419,10.2628509324501));
#74453=CARTESIAN_POINT('Ctrl Pts',(-162.270507762468,226.097251017295,10.3157702208607));
#74454=CARTESIAN_POINT('Ctrl Pts',(-162.434137866349,225.75865627901,10.3396523797431));
#74455=CARTESIAN_POINT('Ctrl Pts',(-162.514537129793,225.379839205506,10.3635345386256));
#74456=CARTESIAN_POINT('Ctrl Pts',(-162.513643783132,225.000662446468,10.387416697508));
#74457=CARTESIAN_POINT('Origin',(-160.,225.,10.));
#74458=CARTESIAN_POINT('',(-162.517183796669,224.997701708063,11.387416697508));
#74459=CARTESIAN_POINT('',(-162.521737918614,224.999954178035,11.1125833024919));
#74460=CARTESIAN_POINT('',(-162.5175,225.,10.));
#74461=CARTESIAN_POINT('Ctrl Pts',(-162.521737514161,224.999954182408,11.1125833024919));
#74462=CARTESIAN_POINT('Ctrl Pts',(-162.52151466846,225.830795448054,11.0598197686592));
#74463=CARTESIAN_POINT('Ctrl Pts',(-162.070684854796,226.661843944495,11.0070562348264));
#74464=CARTESIAN_POINT('Ctrl Pts',(-161.37400504819,227.114539086192,10.9542927009936));
#74465=CARTESIAN_POINT('Ctrl Pts',(-160.675268687345,227.568570555,10.901373412583));
#74466=CARTESIAN_POINT('Ctrl Pts',(-159.729228724324,227.642011622304,10.8484541241724));
#74467=CARTESIAN_POINT('Ctrl Pts',(-158.968793027603,227.30125565715,10.7955348357618));
#74468=CARTESIAN_POINT('Ctrl Pts',(-158.208357330883,226.960499691997,10.7426155473512));
#74469=CARTESIAN_POINT('Ctrl Pts',(-157.633525900464,226.205546694385,10.6896962589407));
#74470=CARTESIAN_POINT('Ctrl Pts',(-157.507341587603,225.381863141179,10.6367769705301));
#74471=CARTESIAN_POINT('Ctrl Pts',(-157.381157274742,224.558179587973,10.5838576821195));
#74472=CARTESIAN_POINT('Ctrl Pts',(-157.70362007944,223.665765479172,10.5309383937089));
#74473=CARTESIAN_POINT('Ctrl Pts',(-158.327171028607,223.112989493417,10.4780191052983));
#74474=CARTESIAN_POINT('Ctrl Pts',(-158.950721977774,222.560213507662,10.4250998168877));
#74475=CARTESIAN_POINT('Ctrl Pts',(-159.87536107141,222.347075644953,10.3721805284771));
#74476=CARTESIAN_POINT('Ctrl Pts',(-160.677973478447,222.571107787075,10.3192612400665));
#74477=CARTESIAN_POINT('Ctrl Pts',(-161.480585885485,222.795139929197,10.2663419516559));
#74478=CARTESIAN_POINT('Ctrl Pts',(-162.161171605924,223.456342076149,10.2134226632453));
#74479=CARTESIAN_POINT('Ctrl Pts',(-162.408294627474,224.252148138488,10.1605033748347));
#74480=CARTESIAN_POINT('Ctrl Pts',(-162.482887171616,224.49235723945,10.1445300173871));
#74481=CARTESIAN_POINT('Ctrl Pts',(-162.51798707635,224.744830057468,10.1285566599395));
#74482=CARTESIAN_POINT('Ctrl Pts',(-162.515939315398,224.997857937799,10.1125833024919));
#74483=CARTESIAN_POINT('Ctrl Pts',(-162.513643783132,225.000662446468,10.387416697508));
#74484=CARTESIAN_POINT('Ctrl Pts',(-162.512557607345,224.539640278395,10.4164538270362));
#74485=CARTESIAN_POINT('Ctrl Pts',(-162.391297224533,224.07808639011,10.4454909565643));
#74486=CARTESIAN_POINT('Ctrl Pts',(-162.153346374264,223.6876491754,10.4745280860925));
#74487=CARTESIAN_POINT('Ctrl Pts',(-161.719688162259,222.976089186267,10.5274473745031));
#74488=CARTESIAN_POINT('Ctrl Pts',(-160.898454725701,222.50073581564,10.5803666629137));
#74489=CARTESIAN_POINT('Ctrl Pts',(-160.065442469011,222.479110756572,10.6332859513243));
#74490=CARTESIAN_POINT('Ctrl Pts',(-159.232430212322,222.457485697503,10.6862052397349));
#74491=CARTESIAN_POINT('Ctrl Pts',(-158.387639135502,222.889588949993,10.7391245281455));
#74492=CARTESIAN_POINT('Ctrl Pts',(-157.917645618693,223.577690074197,10.7920438165561));
#74493=CARTESIAN_POINT('Ctrl Pts',(-157.447652101885,224.265791198402,10.8449631049667));
#74494=CARTESIAN_POINT('Ctrl Pts',(-157.352456145088,225.209890194322,10.8978823933773));
#74495=CARTESIAN_POINT('Ctrl Pts',(-157.675619416261,225.977967379987,10.9508016817879));
#74496=CARTESIAN_POINT('Ctrl Pts',(-157.998782687434,226.746044565652,11.0037209701985));
#74497=CARTESIAN_POINT('Ctrl Pts',(-158.740305186577,227.338099941062,11.0566402586091));
#74498=CARTESIAN_POINT('Ctrl Pts',(-159.560866232662,227.48320897807,11.1095595470196));
#74499=CARTESIAN_POINT('Ctrl Pts',(-160.381427278747,227.628318015078,11.1624788354302));
#74500=CARTESIAN_POINT('Ctrl Pts',(-161.281026871775,227.326480713685,11.2153981238408));
#74501=CARTESIAN_POINT('Ctrl Pts',(-161.848008255663,226.715817817073,11.2683174122514));
#74502=CARTESIAN_POINT('Ctrl Pts',(-162.273354599771,226.257701840186,11.3080171740036));
#74503=CARTESIAN_POINT('Ctrl Pts',(-162.511506122372,225.625781331299,11.3477169357558));
#74504=CARTESIAN_POINT('Ctrl Pts',(-162.517183796669,224.997701708063,11.387416697508));
#74505=CARTESIAN_POINT('Origin',(-160.,225.,10.));
#74506=CARTESIAN_POINT('',(-162.521467546725,225.000747722913,12.387416697508));
#74507=CARTESIAN_POINT('',(-162.516072841654,225.002171058777,12.1125833024919));
#74508=CARTESIAN_POINT('',(-162.5175,225.,10.));
#74509=CARTESIAN_POINT('Ctrl Pts',(-162.516072841654,225.002171058777,12.1125833024919));
#74510=CARTESIAN_POINT('Ctrl Pts',(-162.518115745022,225.250231128475,12.0969214542));
#74511=CARTESIAN_POINT('Ctrl Pts',(-162.484397976292,225.497748022892,12.0812596059081));
#74512=CARTESIAN_POINT('Ctrl Pts',(-162.412644329073,225.733698003867,12.0655977576162));
#74513=CARTESIAN_POINT('Ctrl Pts',(-162.170198362229,226.530941398192,12.0126784692056));
#74514=CARTESIAN_POINT('Ctrl Pts',(-161.493506804995,227.196128393231,11.959759180795));
#74515=CARTESIAN_POINT('Ctrl Pts',(-160.692223700656,227.424869433132,11.9068398923844));
#74516=CARTESIAN_POINT('Ctrl Pts',(-159.890940596317,227.653610473033,11.8539206039738));
#74517=CARTESIAN_POINT('Ctrl Pts',(-158.965065944872,227.445905557796,11.8010013155632));
#74518=CARTESIAN_POINT('Ctrl Pts',(-158.338279968619,226.89680045255,11.7480820271526));
#74519=CARTESIAN_POINT('Ctrl Pts',(-157.711493992366,226.347695347304,11.695162738742));
#74520=CARTESIAN_POINT('Ctrl Pts',(-157.383796691305,225.457190052049,11.6422434503314));
#74521=CARTESIAN_POINT('Ctrl Pts',(-157.505142343957,224.632779772385,11.5893241619208));
#74522=CARTESIAN_POINT('Ctrl Pts',(-157.626487996609,223.80836949272,11.5364048735102));
#74523=CARTESIAN_POINT('Ctrl Pts',(-158.196876602975,223.050054228646,11.4834855850996));
#74524=CARTESIAN_POINT('Ctrl Pts',(-158.955298347997,222.704839030092,11.430566296689));
#74525=CARTESIAN_POINT('Ctrl Pts',(-159.713720093019,222.359623831538,11.3776470082784));
#74526=CARTESIAN_POINT('Ctrl Pts',(-160.660174976697,222.427508698506,11.3247277198678));
#74527=CARTESIAN_POINT('Ctrl Pts',(-161.361565262868,222.877429517204,11.2718084314572));
#74528=CARTESIAN_POINT('Ctrl Pts',(-162.06295554904,223.327350335903,11.2188891430466));
#74529=CARTESIAN_POINT('Ctrl Pts',(-162.519281237706,224.159307106333,11.165969854636));
#74530=CARTESIAN_POINT('Ctrl Pts',(-162.521727702705,224.992596426703,11.1130505662254));
#74531=CARTESIAN_POINT('Ctrl Pts',(-162.521734903257,224.995049003641,11.1128948116476));
#74532=CARTESIAN_POINT('Ctrl Pts',(-162.521738171987,224.997501592121,11.1127390570698));
#74533=CARTESIAN_POINT('Ctrl Pts',(-162.521737514161,224.999954182408,11.1125833024919));
#74534=CARTESIAN_POINT('Ctrl Pts',(-162.517183796669,224.997701708063,11.387416697508));
#74535=CARTESIAN_POINT('Ctrl Pts',(-162.51907439156,224.788559009051,11.4006362241664));
#74536=CARTESIAN_POINT('Ctrl Pts',(-162.495188120451,224.579842190178,11.4138557508248));
#74537=CARTESIAN_POINT('Ctrl Pts',(-162.443853195752,224.378110257364,11.4270752774832));
#74538=CARTESIAN_POINT('Ctrl Pts',(-162.238353577205,223.570554086097,11.4799945658938));
#74539=CARTESIAN_POINT('Ctrl Pts',(-161.592991165361,222.874930235395,11.5329138543044));
#74540=CARTESIAN_POINT('Ctrl Pts',(-160.803083787191,222.60955616566,11.585833142715));
#74541=CARTESIAN_POINT('Ctrl Pts',(-160.013176409022,222.344182095926,11.6387524311256));
#74542=CARTESIAN_POINT('Ctrl Pts',(-159.078724064527,222.509057807159,11.6916717195362));
#74543=CARTESIAN_POINT('Ctrl Pts',(-158.427332128174,223.028736177142,11.7445910079468));
#74544=CARTESIAN_POINT('Ctrl Pts',(-157.775940191821,223.548414547125,11.7975102963574));
#74545=CARTESIAN_POINT('Ctrl Pts',(-157.407608663609,224.422895575858,11.850429584768));
#74546=CARTESIAN_POINT('Ctrl Pts',(-157.490886043608,225.252016761786,11.9033488731786));
#74547=CARTESIAN_POINT('Ctrl Pts',(-157.574163423606,226.081137947714,11.9562681615892));
#74548=CARTESIAN_POINT('Ctrl Pts',(-158.109049711814,226.864899290837,12.0091874499998));
#74549=CARTESIAN_POINT('Ctrl Pts',(-158.850780953264,227.244651615953,12.0621067384104));
#74550=CARTESIAN_POINT('Ctrl Pts',(-159.592512194714,227.624403941069,12.115026026821));
#74551=CARTESIAN_POINT('Ctrl Pts',(-160.541088389406,227.600147248178,12.1679453152316));
#74552=CARTESIAN_POINT('Ctrl Pts',(-161.262441089301,227.182981399469,12.2208646036422));
#74553=CARTESIAN_POINT('Ctrl Pts',(-161.983793789195,226.765815550761,12.2737838920528));
#74554=CARTESIAN_POINT('Ctrl Pts',(-162.477922994292,225.955740546234,12.3267031804634));
#74555=CARTESIAN_POINT('Ctrl Pts',(-162.518715190054,225.123446692035,12.379622468874));
#74556=CARTESIAN_POINT('Ctrl Pts',(-162.520717885793,225.082585166334,12.3822205450853));
#74557=CARTESIAN_POINT('Ctrl Pts',(-162.521627891562,225.041670085963,12.3848186212967));
#74558=CARTESIAN_POINT('Ctrl Pts',(-162.521467546725,225.000747722913,12.387416697508));
#74559=CARTESIAN_POINT('Origin',(-160.,225.,10.));
#74560=CARTESIAN_POINT('',(-162.514983709116,225.001823857702,13.387416697508));
#74561=CARTESIAN_POINT('',(-162.514086051005,224.998759312154,13.1125833024919));
#74562=CARTESIAN_POINT('',(-162.5175,225.,10.));
#74563=CARTESIAN_POINT('Ctrl Pts',(-162.514086051005,224.998759312154,13.1125833024919));
#74564=CARTESIAN_POINT('Ctrl Pts',(-162.511858164299,225.49833849052,13.0811038513303));
#74565=CARTESIAN_POINT('Ctrl Pts',(-162.367841029585,225.99910141157,13.0496244001686));
#74566=CARTESIAN_POINT('Ctrl Pts',(-162.090669988705,226.410058302984,13.0181449490069));
#74567=CARTESIAN_POINT('Ctrl Pts',(-161.62472494487,227.100907268215,12.9652256605963));
#74568=CARTESIAN_POINT('Ctrl Pts',(-160.782485636433,227.53796349952,12.9123063721857));
#74569=CARTESIAN_POINT('Ctrl Pts',(-159.949360754373,227.521230074049,12.8593870837751));
#74570=CARTESIAN_POINT('Ctrl Pts',(-159.116235872314,227.504496648577,12.8064677953645));
#74571=CARTESIAN_POINT('Ctrl Pts',(-158.292225416633,227.033973566329,12.753548506954));
#74572=CARTESIAN_POINT('Ctrl Pts',(-157.854396555648,226.324972180489,12.7006292185434));
#74573=CARTESIAN_POINT('Ctrl Pts',(-157.416567694663,225.615970794649,12.6477099301328));
#74574=CARTESIAN_POINT('Ctrl Pts',(-157.364920428374,224.668491105218,12.5947906417222));
#74575=CARTESIAN_POINT('Ctrl Pts',(-157.72308854482,223.916099799449,12.5418713533116));
#74576=CARTESIAN_POINT('Ctrl Pts',(-158.081256661265,223.16370849368,12.488952064901));
#74577=CARTESIAN_POINT('Ctrl Pts',(-158.849240160445,222.606405571575,12.4360327764904));
#74578=CARTESIAN_POINT('Ctrl Pts',(-159.675609808235,222.49921283933,12.3831134880798));
#74579=CARTESIAN_POINT('Ctrl Pts',(-160.501979456025,222.392020107085,12.3301941996692));
#74580=CARTESIAN_POINT('Ctrl Pts',(-161.386735252425,222.734937564701,12.2772749112586));
#74581=CARTESIAN_POINT('Ctrl Pts',(-161.925012962398,223.371046190315,12.224355622848));
#74582=CARTESIAN_POINT('Ctrl Pts',(-162.303983469161,223.818893841703,12.1870981827293));
#74583=CARTESIAN_POINT('Ctrl Pts',(-162.511213048066,224.412069365775,12.1498407426106));
#74584=CARTESIAN_POINT('Ctrl Pts',(-162.516072841654,225.002171058777,12.1125833024919));
#74585=CARTESIAN_POINT('Ctrl Pts',(-162.521467546725,225.000747722913,12.387416697508));
#74586=CARTESIAN_POINT('Ctrl Pts',(-162.518361884723,224.208137057474,12.4377379097073));
#74587=CARTESIAN_POINT('Ctrl Pts',(-162.113720234785,223.412794336153,12.4880591219065));
#74588=CARTESIAN_POINT('Ctrl Pts',(-161.469861247916,222.950933576905,12.5383803341058));
#74589=CARTESIAN_POINT('Ctrl Pts',(-160.792759923588,222.465227019848,12.5912996225164));
#74590=CARTESIAN_POINT('Ctrl Pts',(-159.851102088505,222.348326609609,12.644218910927));
#74591=CARTESIAN_POINT('Ctrl Pts',(-159.075790349486,222.653725971614,12.6971381993376));
#74592=CARTESIAN_POINT('Ctrl Pts',(-158.300478610467,222.959125333619,12.7500574877482));
#74593=CARTESIAN_POINT('Ctrl Pts',(-157.691512967512,223.686824467868,12.8029767761588));
#74594=CARTESIAN_POINT('Ctrl Pts',(-157.527556086863,224.503828264837,12.8558960645694));
#74595=CARTESIAN_POINT('Ctrl Pts',(-157.363599206214,225.320832061806,12.90881535298));
#74596=CARTESIAN_POINT('Ctrl Pts',(-157.644651087872,226.227140521495,12.9617346413906));
#74597=CARTESIAN_POINT('Ctrl Pts',(-158.242102396316,226.80802691057,13.0146539298012));
#74598=CARTESIAN_POINT('Ctrl Pts',(-158.83955370476,227.388913299645,13.0675732182118));
#74599=CARTESIAN_POINT('Ctrl Pts',(-159.75340443999,227.644377618106,13.1204925066223));
#74600=CARTESIAN_POINT('Ctrl Pts',(-160.565476523533,227.457519398848,13.1734117950329));
#74601=CARTESIAN_POINT('Ctrl Pts',(-161.377548607076,227.270661179591,13.2263310834435));
#74602=CARTESIAN_POINT('Ctrl Pts',(-162.087842038932,226.641480422614,13.2792503718541));
#74603=CARTESIAN_POINT('Ctrl Pts',(-162.371326558649,225.85789022994,13.3321696602647));
#74604=CARTESIAN_POINT('Ctrl Pts',(-162.469977921817,225.585204297215,13.3505853393458));
#74605=CARTESIAN_POINT('Ctrl Pts',(-162.516942328016,225.293819237946,13.3690010184269));
#74606=CARTESIAN_POINT('Ctrl Pts',(-162.514983709116,225.001823857702,13.387416697508));
#74607=CARTESIAN_POINT('Origin',(-160.,225.,10.));
#74608=CARTESIAN_POINT('',(-162.514889421101,224.998220537573,14.387416697508));
#74609=CARTESIAN_POINT('',(-162.520601007743,224.998500607742,14.1125833024919));
#74610=CARTESIAN_POINT('',(-162.5175,225.,10.));
#74611=CARTESIAN_POINT('Ctrl Pts',(-162.520601007743,224.998500607742,14.1125833024919));
#74612=CARTESIAN_POINT('Ctrl Pts',(-162.515344926956,225.74415563317,14.0652862484605));
#74613=CARTESIAN_POINT('Ctrl Pts',(-162.163665278319,226.494118173821,14.0179891944291));
#74614=CARTESIAN_POINT('Ctrl Pts',(-161.584215594788,226.961995506803,13.9706921403977));
#74615=CARTESIAN_POINT('Ctrl Pts',(-160.935886316143,227.485489750407,13.9177728519871));
#74616=CARTESIAN_POINT('Ctrl Pts',(-160.002418184674,227.65584951541,13.8648535635765));
#74617=CARTESIAN_POINT('Ctrl Pts',(-159.210966198987,227.395118176697,13.8119342751659));
#74618=CARTESIAN_POINT('Ctrl Pts',(-158.4195142133,227.134386837984,13.7590149867553));
#74619=CARTESIAN_POINT('Ctrl Pts',(-157.770078373396,226.442564395556,13.7060956983447));
#74620=CARTESIAN_POINT('Ctrl Pts',(-157.559840506845,225.636228785463,13.6531764099341));
#74621=CARTESIAN_POINT('Ctrl Pts',(-157.349602640294,224.829893175371,13.6002571215235));
#74622=CARTESIAN_POINT('Ctrl Pts',(-157.578562747097,223.909044397616,13.5473378331129));
#74623=CARTESIAN_POINT('Ctrl Pts',(-158.141948686882,223.295062834793,13.4944185447023));
#74624=CARTESIAN_POINT('Ctrl Pts',(-158.705334626666,222.681081271969,13.4414992562917));
#74625=CARTESIAN_POINT('Ctrl Pts',(-159.603146399434,222.373966924078,13.3885799678811));
#74626=CARTESIAN_POINT('Ctrl Pts',(-160.424545355618,222.514255310675,13.3356606794705));
#74627=CARTESIAN_POINT('Ctrl Pts',(-161.245944311802,222.654543697272,13.2827413910599));
#74628=CARTESIAN_POINT('Ctrl Pts',(-161.990930451403,223.242234818357,13.2298221026493));
#74629=CARTESIAN_POINT('Ctrl Pts',(-162.318598131587,224.008401228477,13.1769028142387));
#74630=CARTESIAN_POINT('Ctrl Pts',(-162.451350138387,224.31880757807,13.1554629769898));
#74631=CARTESIAN_POINT('Ctrl Pts',(-162.515603406823,224.658508898571,13.1340231397409));
#74632=CARTESIAN_POINT('Ctrl Pts',(-162.514086051005,224.998759312154,13.1125833024919));
#74633=CARTESIAN_POINT('Ctrl Pts',(-162.514983709116,225.001823857702,13.387416697508));
#74634=CARTESIAN_POINT('Ctrl Pts',(-162.511314041491,224.454741424219,13.4219203068375));
#74635=CARTESIAN_POINT('Ctrl Pts',(-162.3359061834,223.905516534921,13.456423916167));
#74636=CARTESIAN_POINT('Ctrl Pts',(-162.00693862054,223.473119956326,13.4909275254965));
#74637=CARTESIAN_POINT('Ctrl Pts',(-161.502390555134,222.809939503758,13.5438468139071));
#74638=CARTESIAN_POINT('Ctrl Pts',(-160.636618816744,222.421578226991,13.5967661023177));
#74639=CARTESIAN_POINT('Ctrl Pts',(-159.805800535833,222.48575023864,13.6496853907283));
#74640=CARTESIAN_POINT('Ctrl Pts',(-158.974982254923,222.549922250288,13.7026046791389));
#74641=CARTESIAN_POINT('Ctrl Pts',(-158.179117431492,223.066627550351,13.7555239675495));
#74642=CARTESIAN_POINT('Ctrl Pts',(-157.782393793095,223.799421803679,13.8084432559601));
#74643=CARTESIAN_POINT('Ctrl Pts',(-157.385670154698,224.532216057008,13.8613625443707));
#74644=CARTESIAN_POINT('Ctrl Pts',(-157.388087701335,225.481099263601,13.9142818327813));
#74645=CARTESIAN_POINT('Ctrl Pts',(-157.788540163711,226.21186248678,13.9672011211919));
#74646=CARTESIAN_POINT('Ctrl Pts',(-158.188992626088,226.942625709959,14.0201204096025));
#74647=CARTESIAN_POINT('Ctrl Pts',(-158.987480004205,227.455268949723,14.0730396980131));
#74648=CARTESIAN_POINT('Ctrl Pts',(-159.818614489535,227.515206669635,14.1259589864237));
#74649=CARTESIAN_POINT('Ctrl Pts',(-160.649748974866,227.575144389548,14.1788782748343));
#74650=CARTESIAN_POINT('Ctrl Pts',(-161.51353056741,227.182376589609,14.2317975632449));
#74651=CARTESIAN_POINT('Ctrl Pts',(-162.014692827404,226.516633807348,14.2847168516555));
#74652=CARTESIAN_POINT('Ctrl Pts',(-162.338892745142,226.085967389556,14.3189501336063));
#74653=CARTESIAN_POINT('Ctrl Pts',(-162.511345689842,225.541067880575,14.3531834155572));
#74654=CARTESIAN_POINT('Ctrl Pts',(-162.514889421101,224.998220537573,14.387416697508));
#74655=CARTESIAN_POINT('Origin',(-160.,225.,10.));
#74656=CARTESIAN_POINT('',(-162.521411304029,224.999178326235,15.387416697508));
#74657=CARTESIAN_POINT('',(-162.518630417247,225.00219537304,15.112583302492));
#74658=CARTESIAN_POINT('',(-162.5175,225.,10.));
#74659=CARTESIAN_POINT('Ctrl Pts',(-162.518630417247,225.00219537304,15.112583302492));
#74660=CARTESIAN_POINT('Ctrl Pts',(-162.520103889651,225.163256307148,15.1023879340014));
#74661=CARTESIAN_POINT('Ctrl Pts',(-162.505977686418,225.32405978629,15.0921925655108));
#74662=CARTESIAN_POINT('Ctrl Pts',(-162.475314724012,225.48164555077,15.0819971970202));
#74663=CARTESIAN_POINT('Ctrl Pts',(-162.316157931139,226.299597989434,15.0290779086096));
#74664=CARTESIAN_POINT('Ctrl Pts',(-161.711475666162,227.030860295603,14.9761586201991));
#74665=CARTESIAN_POINT('Ctrl Pts',(-160.937970521645,227.340806852351,14.9232393317885));
#74666=CARTESIAN_POINT('Ctrl Pts',(-160.164465377128,227.650753409099,14.8703200433779));
#74667=CARTESIAN_POINT('Ctrl Pts',(-159.22213735307,227.539384216426,14.8174007549673));
#74668=CARTESIAN_POINT('Ctrl Pts',(-158.542195734753,227.05766181471,14.7644814665567));
#74669=CARTESIAN_POINT('Ctrl Pts',(-157.862254116436,226.575939412994,14.7115621781461));
#74670=CARTESIAN_POINT('Ctrl Pts',(-157.44469890386,225.723863802235,14.6586428897355));
#74671=CARTESIAN_POINT('Ctrl Pts',(-157.480603354089,224.891344765162,14.6057236013249));
#74672=CARTESIAN_POINT('Ctrl Pts',(-157.516507804318,224.05882572809,14.5528043129143));
#74673=CARTESIAN_POINT('Ctrl Pts',(-158.005871917352,223.245863264704,14.4998850245037));
#74674=CARTESIAN_POINT('Ctrl Pts',(-158.724762684689,222.824468982265,14.4469657360931));
#74675=CARTESIAN_POINT('Ctrl Pts',(-159.443653452027,222.403074699827,14.3940464476825));
#74676=CARTESIAN_POINT('Ctrl Pts',(-160.392070873667,222.373248598336,14.3411271592719));
#74677=CARTESIAN_POINT('Ctrl Pts',(-161.136019156115,222.748639101249,14.2882078708613));
#74678=CARTESIAN_POINT('Ctrl Pts',(-161.879967438563,223.124029604161,14.2352885824507));
#74679=CARTESIAN_POINT('Ctrl Pts',(-162.419446581819,223.904636711477,14.1823692940401));
#74680=CARTESIAN_POINT('Ctrl Pts',(-162.507590940537,224.733254626237,14.1294500056295));
#74681=CARTESIAN_POINT('Ctrl Pts',(-162.516955545746,224.82128838987,14.1238277712503));
#74682=CARTESIAN_POINT('Ctrl Pts',(-162.521225801796,224.909864065682,14.1182055368711));
#74683=CARTESIAN_POINT('Ctrl Pts',(-162.520601007743,224.998500607742,14.1125833024919));
#74684=CARTESIAN_POINT('Ctrl Pts',(-162.514889421101,224.998220537573,14.387416697508));
#74685=CARTESIAN_POINT('Ctrl Pts',(-162.516823742949,224.701910970393,14.4061027039678));
#74686=CARTESIAN_POINT('Ctrl Pts',(-162.468432430799,224.406212835544,14.4247887104275));
#74687=CARTESIAN_POINT('Ctrl Pts',(-162.366924368858,224.130037744216,14.4434747168873));
#74688=CARTESIAN_POINT('Ctrl Pts',(-162.079450722877,223.347902227928,14.4963940052979));
#74689=CARTESIAN_POINT('Ctrl Pts',(-161.36596050347,222.722348959933,14.5493132937085));
#74690=CARTESIAN_POINT('Ctrl Pts',(-160.552946821011,222.539631103367,14.6022325821191));
#74691=CARTESIAN_POINT('Ctrl Pts',(-159.739933138551,222.356913246801,14.6551518705297));
#74692=CARTESIAN_POINT('Ctrl Pts',(-158.827395993039,222.617030801664,14.7080711589403));
#74693=CARTESIAN_POINT('Ctrl Pts',(-158.232912364318,223.200953979965,14.7609904473509));
#74694=CARTESIAN_POINT('Ctrl Pts',(-157.638428735597,223.784877158266,14.8139097357615));
#74695=CARTESIAN_POINT('Ctrl Pts',(-157.361998623667,224.692605960004,14.8668290241721));
#74696=CARTESIAN_POINT('Ctrl Pts',(-157.530116442313,225.508763703353,14.9197483125827));
#74697=CARTESIAN_POINT('Ctrl Pts',(-157.698234260958,226.324921446702,14.9726676009933));
#74698=CARTESIAN_POINT('Ctrl Pts',(-158.310900010178,227.049508131661,15.0255868894039));
#74699=CARTESIAN_POINT('Ctrl Pts',(-159.087757855177,227.350952905439,15.0785061778145));
#74700=CARTESIAN_POINT('Ctrl Pts',(-159.864615700175,227.652397679217,15.131425466225));
#74701=CARTESIAN_POINT('Ctrl Pts',(-160.805665640952,227.530700541815,15.1843447546356));
#74702=CARTESIAN_POINT('Ctrl Pts',(-161.48028324311,227.041550100916,15.2372640430462));
#74703=CARTESIAN_POINT('Ctrl Pts',(-162.118334300063,226.578913260688,15.2873149278668));
#74704=CARTESIAN_POINT('Ctrl Pts',(-162.518053298317,225.787577949575,15.3373658126874));
#74705=CARTESIAN_POINT('Ctrl Pts',(-162.521411304029,224.999178326235,15.387416697508));
#74706=CARTESIAN_POINT('Origin',(-160.,225.,10.));
#74707=CARTESIAN_POINT('',(-162.517311833712,225.002301033826,16.387416697508));
#74708=CARTESIAN_POINT('',(-162.51348711883,225.000116346804,16.1125833024919));
#74709=CARTESIAN_POINT('',(-162.5175,225.,10.));
#74710=CARTESIAN_POINT('Ctrl Pts',(-162.51348711883,225.000116346804,16.1125833024919));
#74711=CARTESIAN_POINT('Ctrl Pts',(-162.513657421629,225.413188244457,16.0865703311316));
#74712=CARTESIAN_POINT('Ctrl Pts',(-162.417512298305,225.82618548606,16.0605573597713));
#74713=CARTESIAN_POINT('Ctrl Pts',(-162.22461752507,226.187536225391,16.034544388411));
#74714=CARTESIAN_POINT('Ctrl Pts',(-161.832203525286,226.922647325434,15.9816251000004));
#74715=CARTESIAN_POINT('Ctrl Pts',(-161.039386391521,227.444016862716,15.9287058115898));
#74716=CARTESIAN_POINT('Ctrl Pts',(-160.208959228585,227.513066147216,15.8757865231792));
#74717=CARTESIAN_POINT('Ctrl Pts',(-159.37853206565,227.582115431716,15.8228672347686));
#74718=CARTESIAN_POINT('Ctrl Pts',(-158.510494873542,227.198844463435,15.769947946358));
#74719=CARTESIAN_POINT('Ctrl Pts',(-158.002061454311,226.538638029927,15.7170286579474));
#74720=CARTESIAN_POINT('Ctrl Pts',(-157.49362803508,225.878431596419,15.6641093695368));
#74721=CARTESIAN_POINT('Ctrl Pts',(-157.344798388724,224.941289697685,15.6111900811262));
#74722=CARTESIAN_POINT('Ctrl Pts',(-157.623676958487,224.156048448157,15.5582707927156));
#74723=CARTESIAN_POINT('Ctrl Pts',(-157.90255552825,223.370807198628,15.505351504305));
#74724=CARTESIAN_POINT('Ctrl Pts',(-158.609142314132,222.737466598306,15.4524322158944));
#74725=CARTESIAN_POINT('Ctrl Pts',(-159.420103216808,222.545843293445,15.3995129274838));
#74726=CARTESIAN_POINT('Ctrl Pts',(-160.231064119483,222.354219988584,15.3465936390732));
#74727=CARTESIAN_POINT('Ctrl Pts',(-161.146399138952,222.604313979185,15.2936743506626));
#74728=CARTESIAN_POINT('Ctrl Pts',(-161.747250988303,223.181682260065,15.240755062252));
#74729=CARTESIAN_POINT('Ctrl Pts',(-162.232343419937,223.647815440189,15.198031142332));
#74730=CARTESIAN_POINT('Ctrl Pts',(-162.512455798149,224.327265922729,15.155307222412));
#74731=CARTESIAN_POINT('Ctrl Pts',(-162.518630417247,225.00219537304,15.112583302492));
#74732=CARTESIAN_POINT('Ctrl Pts',(-162.521411304029,224.999178326235,15.387416697508));
#74733=CARTESIAN_POINT('Ctrl Pts',(-162.52160375049,224.953995342597,15.390285101098));
#74734=CARTESIAN_POINT('Ctrl Pts',(-162.520494386053,224.908822000952,15.393153504688));
#74735=CARTESIAN_POINT('Ctrl Pts',(-162.51805346516,224.863720724318,15.396021908278));
#74736=CARTESIAN_POINT('Ctrl Pts',(-162.473020821511,224.031645533015,15.4489411966886));
#74737=CARTESIAN_POINT('Ctrl Pts',(-161.974770270673,223.224098894804,15.5018604850992));
#74738=CARTESIAN_POINT('Ctrl Pts',(-161.251301254915,222.810614135462,15.5547797735098));
#74739=CARTESIAN_POINT('Ctrl Pts',(-160.527832239156,222.397129376119,15.6076990619204));
#74740=CARTESIAN_POINT('Ctrl Pts',(-159.579144758477,222.377706495644,15.660618350331));
#74741=CARTESIAN_POINT('Ctrl Pts',(-158.83935818538,222.761233403743,15.7135376387416));
#74742=CARTESIAN_POINT('Ctrl Pts',(-158.099571612282,223.144760311842,15.7664569271522));
#74743=CARTESIAN_POINT('Ctrl Pts',(-157.568685946766,223.931237008516,15.8193762155628));
#74744=CARTESIAN_POINT('Ctrl Pts',(-157.48963445894,224.760771772865,15.8722955039734));
#74745=CARTESIAN_POINT('Ctrl Pts',(-157.410582971115,225.590306537214,15.925214792384));
#74746=CARTESIAN_POINT('Ctrl Pts',(-157.783365660981,226.462899369238,15.9781340807946));
#74747=CARTESIAN_POINT('Ctrl Pts',(-158.437397176969,226.979251806087,16.0310533692052));
#74748=CARTESIAN_POINT('Ctrl Pts',(-159.091428692956,227.495604242937,16.0839726576158));
#74749=CARTESIAN_POINT('Ctrl Pts',(-160.026709035066,227.655716284612,16.1368919460264));
#74750=CARTESIAN_POINT('Ctrl Pts',(-160.815253937172,227.38632066414,16.189811234437));
#74751=CARTESIAN_POINT('Ctrl Pts',(-161.603798839277,227.116925043669,16.2427305228476));
#74752=CARTESIAN_POINT('Ctrl Pts',(-162.245608301378,226.418021761049,16.2956498112582));
#74753=CARTESIAN_POINT('Ctrl Pts',(-162.446990326167,225.609428944358,16.3485690996688));
#74754=CARTESIAN_POINT('Ctrl Pts',(-162.496267934553,225.411568583155,16.3615182989485));
#74755=CARTESIAN_POINT('Ctrl Pts',(-162.51917420259,225.207140374923,16.3744674982283));
#74756=CARTESIAN_POINT('Ctrl Pts',(-162.517311833712,225.002301033826,16.387416697508));
#74757=CARTESIAN_POINT('Origin',(-160.,225.,10.));
#74758=CARTESIAN_POINT('',(-162.51361180286,224.999405384875,17.387416697508));
#74759=CARTESIAN_POINT('',(-162.518203433835,224.997743576262,17.1125833024919));
#74760=CARTESIAN_POINT('',(-162.5175,225.,10.));
#74761=CARTESIAN_POINT('Ctrl Pts',(-162.518203433835,224.997743576262,17.1125833024919));
#74762=CARTESIAN_POINT('Ctrl Pts',(-162.512102125057,225.658848760357,17.0707527282619));
#74763=CARTESIAN_POINT('Ctrl Pts',(-162.244817921865,226.324319952305,17.0289221540318));
#74764=CARTESIAN_POINT('Ctrl Pts',(-161.777620784395,226.788639081685,16.9870915798017));
#74765=CARTESIAN_POINT('Ctrl Pts',(-161.186576063699,227.376042873634,16.9341722913911));
#74766=CARTESIAN_POINT('Ctrl Pts',(-160.275581992911,227.64151416071,16.8812530029806));
#74767=CARTESIAN_POINT('Ctrl Pts',(-159.461509439912,227.463573286232,16.82833371457));
#74768=CARTESIAN_POINT('Ctrl Pts',(-158.647436886914,227.285632411754,16.7754144261594));
#74769=CARTESIAN_POINT('Ctrl Pts',(-157.930285851704,226.664279375724,16.7224951377488));
#74770=CARTESIAN_POINT('Ctrl Pts',(-157.638224634377,225.88384531566,16.6695758493382));
#74771=CARTESIAN_POINT('Ctrl Pts',(-157.34616341705,225.103411255596,16.6166565609276));
#74772=CARTESIAN_POINT('Ctrl Pts',(-157.479192017605,224.163896171499,16.563737272517));
#74773=CARTESIAN_POINT('Ctrl Pts',(-157.976436550811,223.495222147163,16.5108179841064));
#74774=CARTESIAN_POINT('Ctrl Pts',(-158.473681084018,222.826548122827,16.4578986956958));
#74775=CARTESIAN_POINT('Ctrl Pts',(-159.335141549876,222.428715158251,16.4049794072852));
#74776=CARTESIAN_POINT('Ctrl Pts',(-160.166613656259,222.483771610307,16.3520601188746));
#74777=CARTESIAN_POINT('Ctrl Pts',(-160.998085762643,222.538828062363,16.299140830464));
#74778=CARTESIAN_POINT('Ctrl Pts',(-161.799569509551,223.046773931052,16.2462215420534));
#74779=CARTESIAN_POINT('Ctrl Pts',(-162.204305950103,223.775173196799,16.1933022536428));
#74780=CARTESIAN_POINT('Ctrl Pts',(-162.410090406365,224.145520988162,16.1663959365925));
#74781=CARTESIAN_POINT('Ctrl Pts',(-162.513310967437,224.572858603394,16.1394896195422));
#74782=CARTESIAN_POINT('Ctrl Pts',(-162.51348711883,225.000116346804,16.1125833024919));
#74783=CARTESIAN_POINT('Ctrl Pts',(-162.517311833712,225.002301033826,16.387416697508));
#74784=CARTESIAN_POINT('Ctrl Pts',(-162.511563289078,224.370026671198,16.4273867866389));
#74785=CARTESIAN_POINT('Ctrl Pts',(-162.269828596412,223.73383519107,16.4673568757697));
#74786=CARTESIAN_POINT('Ctrl Pts',(-161.839241264813,223.274787878362,16.5073269649006));
#74787=CARTESIAN_POINT('Ctrl Pts',(-161.269155591191,222.667021979822,16.5602462533112));
#74788=CARTESIAN_POINT('Ctrl Pts',(-160.368029656471,222.369772533509,16.6131655417218));
#74789=CARTESIAN_POINT('Ctrl Pts',(-159.548218670367,222.519060878874,16.6660848301324));
#74790=CARTESIAN_POINT('Ctrl Pts',(-158.728407684263,222.668349224239,16.719004118543));
#74791=CARTESIAN_POINT('Ctrl Pts',(-157.989911646774,223.264175361282,16.7719234069536));
#74792=CARTESIAN_POINT('Ctrl Pts',(-157.670666330748,224.03388926418,16.8248426953642));
#74793=CARTESIAN_POINT('Ctrl Pts',(-157.351421014722,224.803603167077,16.8777619837748));
#74794=CARTESIAN_POINT('Ctrl Pts',(-157.451426420158,225.747204835827,16.9306812721854));
#74795=CARTESIAN_POINT('Ctrl Pts',(-157.924920074226,226.432902159615,16.983600560596));
#74796=CARTESIAN_POINT('Ctrl Pts',(-158.398413728293,227.118599483403,17.0365198490066));
#74797=CARTESIAN_POINT('Ctrl Pts',(-159.245395630993,227.546392462228,17.0894391374172));
#74798=CARTESIAN_POINT('Ctrl Pts',(-160.078286882935,227.52052304932,17.1423584258278));
#74799=CARTESIAN_POINT('Ctrl Pts',(-160.911178134878,227.494653636412,17.1952777142384));
#74800=CARTESIAN_POINT('Ctrl Pts',(-161.729978736064,227.015121831771,17.248197002649));
#74801=CARTESIAN_POINT('Ctrl Pts',(-162.160005542026,226.301361355021,17.3011162910596));
#74802=CARTESIAN_POINT('Ctrl Pts',(-162.393767113989,225.91336281926,17.329883093209));
#74803=CARTESIAN_POINT('Ctrl Pts',(-162.512646638904,225.456150078067,17.3586498953585));
#74804=CARTESIAN_POINT('Ctrl Pts',(-162.51361180286,224.999405384875,17.387416697508));
#74805=CARTESIAN_POINT('Origin',(-160.,225.,10.));
#74806=CARTESIAN_POINT('',(-162.519491434632,224.998011610487,18.387416697508));
#74807=CARTESIAN_POINT('',(-162.520906539752,225.001296842262,18.1125833024919));
#74808=CARTESIAN_POINT('',(-162.5175,225.,10.));
#74809=CARTESIAN_POINT('Ctrl Pts',(-162.520906539752,225.001296842262,18.1125833024919));
#74810=CARTESIAN_POINT('Ctrl Pts',(-162.521374419554,225.075825678322,18.1078544138027));
#74811=CARTESIAN_POINT('Ctrl Pts',(-162.518355714192,225.150316081198,18.1031255251135));
#74812=CARTESIAN_POINT('Ctrl Pts',(-162.511727028206,225.224483843695,18.0983966364243));
#74813=CARTESIAN_POINT('Ctrl Pts',(-162.437547793174,226.054468534037,18.0454773480137));
#74814=CARTESIAN_POINT('Ctrl Pts',(-161.911289198169,226.844048836985,17.9925580596031));
#74815=CARTESIAN_POINT('Ctrl Pts',(-161.173767331383,227.231912975972,17.9396387711925));
#74816=CARTESIAN_POINT('Ctrl Pts',(-160.436245464596,227.619777114959,17.8867194827819));
#74817=CARTESIAN_POINT('Ctrl Pts',(-159.487460326027,227.605925089986,17.8338001943713));
#74818=CARTESIAN_POINT('Ctrl Pts',(-158.761575896687,227.196695512932,17.7808809059607));
#74819=CARTESIAN_POINT('Ctrl Pts',(-158.035691467348,226.787465935877,17.7279616175501));
#74820=CARTESIAN_POINT('Ctrl Pts',(-157.532707747238,225.98285880674,17.6750423291395));
#74821=CARTESIAN_POINT('Ctrl Pts',(-157.482790115221,225.151062367887,17.6221230407289));
#74822=CARTESIAN_POINT('Ctrl Pts',(-157.432872483204,224.319265929034,17.5692037523183));
#74823=CARTESIAN_POINT('Ctrl Pts',(-157.836020939279,223.460280180465,17.5162844639077));
#74824=CARTESIAN_POINT('Ctrl Pts',(-158.507754739353,222.967176966537,17.4633651754971));
#74825=CARTESIAN_POINT('Ctrl Pts',(-159.179488539427,222.47407375261,17.4104458870865));
#74826=CARTESIAN_POINT('Ctrl Pts',(-160.119807683499,222.346853073324,17.3575265986759));
#74827=CARTESIAN_POINT('Ctrl Pts',(-160.898422158656,222.643731117356,17.3046073102653));
#74828=CARTESIAN_POINT('Ctrl Pts',(-161.677036633814,222.940609161388,17.2516880218547));
#74829=CARTESIAN_POINT('Ctrl Pts',(-162.293946440056,223.661585928738,17.1987687334441));
#74830=CARTESIAN_POINT('Ctrl Pts',(-162.466853657876,224.476742460824,17.1458494450335));
#74831=CARTESIAN_POINT('Ctrl Pts',(-162.503084657493,224.647550460482,17.134760730853));
#74832=CARTESIAN_POINT('Ctrl Pts',(-162.519820807501,224.822493617,17.1236720166725));
#74833=CARTESIAN_POINT('Ctrl Pts',(-162.518203433835,224.997743576262,17.1125833024919));
#74834=CARTESIAN_POINT('Ctrl Pts',(-162.51361180286,224.999405384875,17.387416697508));
#74835=CARTESIAN_POINT('Ctrl Pts',(-162.514422150463,224.615924458848,17.4115691837691));
#74836=CARTESIAN_POINT('Ctrl Pts',(-162.432112176184,224.232773469737,17.4357216700302));
#74837=CARTESIAN_POINT('Ctrl Pts',(-162.264887208673,223.891193775679,17.4598741562913));
#74838=CARTESIAN_POINT('Ctrl Pts',(-161.898489058622,223.142775821946,17.5127934447019));
#74839=CARTESIAN_POINT('Ctrl Pts',(-161.124439747783,222.593929063341,17.5657127331125));
#74840=CARTESIAN_POINT('Ctrl Pts',(-160.296944202049,222.495805659244,17.6186320215231));
#74841=CARTESIAN_POINT('Ctrl Pts',(-159.469448656315,222.397682255148,17.6715513099337));
#74842=CARTESIAN_POINT('Ctrl Pts',(-158.588506875685,222.750282205561,17.7244705983443));
#74843=CARTESIAN_POINT('Ctrl Pts',(-158.057237850476,223.392256001223,17.7773898867549));
#74844=CARTESIAN_POINT('Ctrl Pts',(-157.525968825266,224.034229796885,17.8303091751655));
#74845=CARTESIAN_POINT('Ctrl Pts',(-157.344372555475,224.965577437797,17.8832284635761));
#74846=CARTESIAN_POINT('Ctrl Pts',(-157.59554738929,225.760113802981,17.9361477519867));
#74847=CARTESIAN_POINT('Ctrl Pts',(-157.846722223105,226.554650168166,17.9890670403973));
#74848=CARTESIAN_POINT('Ctrl Pts',(-158.530668160525,227.212375257623,18.0419863288079));
#74849=CARTESIAN_POINT('Ctrl Pts',(-159.334411764228,227.432315035357,18.0949056172185));
#74850=CARTESIAN_POINT('Ctrl Pts',(-160.138155367931,227.652254813092,18.1478249056291));
#74851=CARTESIAN_POINT('Ctrl Pts',(-161.061696637917,227.434409279103,18.2007441940397));
#74852=CARTESIAN_POINT('Ctrl Pts',(-161.682422671056,226.878462570083,18.2536634824503));
#74853=CARTESIAN_POINT('Ctrl Pts',(-162.205383234183,226.410078470665,18.2982478874695));
#74854=CARTESIAN_POINT('Ctrl Pts',(-162.513404570081,225.701709071819,18.3428322924888));
#74855=CARTESIAN_POINT('Ctrl Pts',(-162.519491434632,224.998011610487,18.387416697508));
#74856=CARTESIAN_POINT('Origin',(-160.,225.,10.));
#74857=CARTESIAN_POINT('',(-162.519857258493,225.0018235551,19.387416697508));
#74858=CARTESIAN_POINT('',(-162.514309478995,225.001427434952,19.112583302492));
#74859=CARTESIAN_POINT('',(-162.5175,225.,10.));
#74860=CARTESIAN_POINT('',(-158.086534003335,226.635987203375,20.));
#74861=CARTESIAN_POINT('Ctrl Pts',(-162.519857258493,225.0018235551,19.387416697508));
#74862=CARTESIAN_POINT('Ctrl Pts',(-162.513963907793,224.285086687949,19.4328532664402));
#74863=CARTESIAN_POINT('Ctrl Pts',(-162.192666772489,223.563823557618,19.4782898353725));
#74864=CARTESIAN_POINT('Ctrl Pts',(-161.652075996519,223.094935228314,19.5237264043047));
#74865=CARTESIAN_POINT('Ctrl Pts',(-161.022458050931,222.548828043862,19.5766456927152));
#74866=CARTESIAN_POINT('Ctrl Pts',(-160.095370243792,222.345065019015,19.6295649811258));
#74867=CARTESIAN_POINT('Ctrl Pts',(-159.295373480112,222.578292534632,19.6824842695364));
#74868=CARTESIAN_POINT('Ctrl Pts',(-158.495376716432,222.811520050248,19.735403557947));
#74869=CARTESIAN_POINT('Ctrl Pts',(-157.82247099621,223.481738106327,19.7883228463576));
#74870=CARTESIAN_POINT('Ctrl Pts',(-157.584268188238,224.278797222609,19.8412421347682));
#74871=CARTESIAN_POINT('Ctrl Pts',(-157.346065380267,225.075856338892,19.8941614231788));
#74872=CARTESIAN_POINT('Ctrl Pts',(-157.542565484547,225.999756515379,19.9470807115894));
#74873=CARTESIAN_POINT('Ctrl Pts',(-158.086534003335,226.635987203375,20.));
#74874=CARTESIAN_POINT('',(-161.917152621948,226.63875490413,20.));
#74875=CARTESIAN_POINT('Origin',(-160.,225.,20.));
#74876=CARTESIAN_POINT('Ctrl Pts',(-161.917156323069,226.638757682714,20.));
#74877=CARTESIAN_POINT('Ctrl Pts',(-161.386618552193,227.2574510649,19.948244384658));
#74878=CARTESIAN_POINT('Ctrl Pts',(-160.527623943219,227.59712432977,19.896488769316));
#74879=CARTESIAN_POINT('Ctrl Pts',(-159.717628711707,227.505772044351,19.844733153974));
#74880=CARTESIAN_POINT('Ctrl Pts',(-158.889421550332,227.412365794477,19.7918138655634));
#74881=CARTESIAN_POINT('Ctrl Pts',(-158.112441940732,226.868333744093,19.7388945771528));
#74882=CARTESIAN_POINT('Ctrl Pts',(-157.741727875214,226.12214740534,19.6859752887422));
#74883=CARTESIAN_POINT('Ctrl Pts',(-157.371013809696,225.375961066586,19.6330560003316));
#74884=CARTESIAN_POINT('Ctrl Pts',(-157.40656528826,224.427620439464,19.580136711921));
#74885=CARTESIAN_POINT('Ctrl Pts',(-157.832358820112,223.7113146992,19.5272174235104));
#74886=CARTESIAN_POINT('Ctrl Pts',(-158.258152351964,222.995008958935,19.4742981350998));
#74887=CARTESIAN_POINT('Ctrl Pts',(-159.074187937105,222.51073810553,19.4213788466892));
#74888=CARTESIAN_POINT('Ctrl Pts',(-159.906929723711,222.479994259423,19.3684595582786));
#74889=CARTESIAN_POINT('Ctrl Pts',(-160.739671510318,222.449250413317,19.315540269868));
#74890=CARTESIAN_POINT('Ctrl Pts',(-161.589119498392,222.872033574509,19.2626209814574));
#74891=CARTESIAN_POINT('Ctrl Pts',(-162.066623166706,223.554931282467,19.2097016930469));
#74892=CARTESIAN_POINT('Ctrl Pts',(-162.358730821865,223.972686498648,19.1773288961952));
#74893=CARTESIAN_POINT('Ctrl Pts',(-162.511647724414,224.487783003849,19.1449560993436));
#74894=CARTESIAN_POINT('Ctrl Pts',(-162.514309478995,225.001427434952,19.112583302492));
#74895=CARTESIAN_POINT('Origin',(0.,-225.,10.));
#74896=CARTESIAN_POINT('',(-2.5134738280043,-224.999414148646,0.387416697508012));
#74897=CARTESIAN_POINT('',(-2.51553384111454,-225.003594604017,0.112583302491983));
#74898=CARTESIAN_POINT('',(-2.5175,-225.,10.));
#74899=CARTESIAN_POINT('',(-1.91346599666507,-223.364012796625,0.));
#74900=CARTESIAN_POINT('Ctrl Pts',(-2.51553384111454,-225.003594604017,
0.112583302491983));
#74901=CARTESIAN_POINT('Ctrl Pts',(-2.510318857578,-224.410959591099,0.0750555349946555));
#74902=CARTESIAN_POINT('Ctrl Pts',(-2.29922182808404,-223.815196439696,
0.037527767497328));
#74903=CARTESIAN_POINT('Ctrl Pts',(-1.91346599666507,-223.364012796625,
0.));
#74904=CARTESIAN_POINT('',(1.91712505749227,-223.361260570198,1.64203312618124E-15));
#74905=CARTESIAN_POINT('Origin',(0.,-225.,0.));
#74906=CARTESIAN_POINT('Ctrl Pts',(1.91712862604369,-223.36125788605,1.4081598368354E-15));
#74907=CARTESIAN_POINT('Ctrl Pts',(1.38658196318478,-222.742517051696,0.0517556153419835));
#74908=CARTESIAN_POINT('Ctrl Pts',(0.527608265094371,-222.402929728057,
0.103511230683964));
#74909=CARTESIAN_POINT('Ctrl Pts',(-0.282369175077661,-222.49429768012,
0.155266846025946));
#74910=CARTESIAN_POINT('Ctrl Pts',(-1.11055814509214,-222.587719948888,
0.208186134436544));
#74911=CARTESIAN_POINT('Ctrl Pts',(-1.88752282473288,-223.131694547948,
0.261105422847144));
#74912=CARTESIAN_POINT('Ctrl Pts',(-2.25823169761475,-223.877857467097,
0.314024711257743));
#74913=CARTESIAN_POINT('Ctrl Pts',(-2.42960626517823,-224.222800242831,
0.3384887066745));
#74914=CARTESIAN_POINT('Ctrl Pts',(-2.51415951692064,-224.610952877235,
0.362952702091256));
#74915=CARTESIAN_POINT('Ctrl Pts',(-2.5134738280043,-224.999414148646,0.387416697508012));
#74916=CARTESIAN_POINT('Origin',(0.,-225.,10.));
#74917=CARTESIAN_POINT('',(-2.5174184095497,-225.002301197522,1.38741669750801));
#74918=CARTESIAN_POINT('',(-2.52168724981252,-224.999862409999,1.11258330249199));
#74919=CARTESIAN_POINT('',(-2.5175,-225.,10.));
#74920=CARTESIAN_POINT('Ctrl Pts',(-2.52168724981252,-224.999862409999,
1.11258330249199));
#74921=CARTESIAN_POINT('Ctrl Pts',(-2.52169211725575,-224.99315326678,1.11215722053551));
#74922=CARTESIAN_POINT('Ctrl Pts',(-2.52166766934934,-224.986444162339,
1.11173113857903));
#74923=CARTESIAN_POINT('Ctrl Pts',(-2.52161379929192,-224.979735296596,
1.11130505662256));
#74924=CARTESIAN_POINT('Ctrl Pts',(-2.514923149613,-224.146495597611,1.05838576821196));
#74925=CARTESIAN_POINT('Ctrl Pts',(-2.05437854416698,-223.316937960849,
1.00546647980136));
#74926=CARTESIAN_POINT('Ctrl Pts',(-1.35071294162604,-222.870578888206,
0.952547191390766));
#74927=CARTESIAN_POINT('Ctrl Pts',(-0.647047339085058,-222.424219815563,
0.899627902980166));
#74928=CARTESIAN_POINT('Ctrl Pts',(0.299739260550884,-222.361059307038,
0.846708614569566));
#74929=CARTESIAN_POINT('Ctrl Pts',(1.05637246458552,-222.710180484341,0.793789326158967));
#74930=CARTESIAN_POINT('Ctrl Pts',(1.81300566862008,-223.059301661644,0.740870037748372));
#74931=CARTESIAN_POINT('Ctrl Pts',(2.37948547705339,-223.820704524774,0.687950749337777));
#74932=CARTESIAN_POINT('Ctrl Pts',(2.49664120954915,-224.645603706033,0.635031460927181));
#74933=CARTESIAN_POINT('Ctrl Pts',(2.61379694204491,-225.470502887292,0.582112172516582));
#74934=CARTESIAN_POINT('Ctrl Pts',(2.28162859860309,-226.358898386679,0.529192884105983));
#74935=CARTESIAN_POINT('Ctrl Pts',(1.65203473703061,-226.905008475225,0.476273595695384));
#74936=CARTESIAN_POINT('Ctrl Pts',(1.02244087545817,-227.45111856377,0.423354307284788));
#74937=CARTESIAN_POINT('Ctrl Pts',(0.0954214957550896,-227.654943241475,
0.370435018874193));
#74938=CARTESIAN_POINT('Ctrl Pts',(-0.704614946080803,-227.421676512248,
0.317515730463596));
#74939=CARTESIAN_POINT('Ctrl Pts',(-1.50465138791669,-227.188409783022,
0.264596442052999));
#74940=CARTESIAN_POINT('Ctrl Pts',(-2.17770489188541,-226.518051646864,
0.2116771536424));
#74941=CARTESIAN_POINT('Ctrl Pts',(-2.41590067376944,-225.721010072264,
0.158757865231803));
#74942=CARTESIAN_POINT('Ctrl Pts',(-2.48517967332582,-225.489191345432,
0.14336634431853));
#74943=CARTESIAN_POINT('Ctrl Pts',(-2.51767269811346,-225.246656070328,
0.127974823405257));
#74944=CARTESIAN_POINT('Ctrl Pts',(-2.51553384111454,-225.003594604017,
0.112583302491983));
#74945=CARTESIAN_POINT('Ctrl Pts',(-2.5134738280043,-224.999414148646,0.387416697508012));
#74946=CARTESIAN_POINT('Ctrl Pts',(-2.51267626903306,-225.451252824483,
0.415871990501852));
#74947=CARTESIAN_POINT('Ctrl Pts',(-2.39655744609628,-225.903509060763,
0.444327283495693));
#74948=CARTESIAN_POINT('Ctrl Pts',(-2.16760745744079,-226.288671524275,
0.472782576489533));
#74949=CARTESIAN_POINT('Ctrl Pts',(-1.74182127826191,-227.004971423064,
0.525701864900131));
#74950=CARTESIAN_POINT('Ctrl Pts',(-0.925795853781111,-227.489219981405,
0.578621153310729));
#74951=CARTESIAN_POINT('Ctrl Pts',(-0.0930673405406173,-227.519960009479,
0.631540441721328));
#74952=CARTESIAN_POINT('Ctrl Pts',(0.739661172699829,-227.550700037554,
0.684459730131924));
#74953=CARTESIAN_POINT('Ctrl Pts',(1.58909277469996,-227.127931535363,0.73737901854252));
#74954=CARTESIAN_POINT('Ctrl Pts',(2.0665881116238,-226.445046923735,0.790298306953116));
#74955=CARTESIAN_POINT('Ctrl Pts',(2.54408344854767,-225.762162312107,0.843217595363715));
#74956=CARTESIAN_POINT('Ctrl Pts',(2.64964252039518,-224.819161591042,0.896136883774315));
#74957=CARTESIAN_POINT('Ctrl Pts',(2.33493169451256,-224.047594583661,0.949056172184913));
#74958=CARTESIAN_POINT('Ctrl Pts',(2.02022086862996,-223.27602757628,1.00197546059551));
#74959=CARTESIAN_POINT('Ctrl Pts',(1.28524014501729,-222.675894282583,1.05489474900611));
#74960=CARTESIAN_POINT('Ctrl Pts',(0.466331362713798,-222.521799579672,
1.1078140374167));
#74961=CARTESIAN_POINT('Ctrl Pts',(-0.352577419589698,-222.367704876761,
1.1607333258273));
#74962=CARTESIAN_POINT('Ctrl Pts',(-1.25541426058401,-222.659648764636,
1.2136526142379));
#74963=CARTESIAN_POINT('Ctrl Pts',(-1.82904826482005,-223.264045656224,
1.2665719026485));
#74964=CARTESIAN_POINT('Ctrl Pts',(-2.26569235464287,-223.724106128007,
1.306853500935));
#74965=CARTESIAN_POINT('Ctrl Pts',(-2.51159328780835,-224.365204748859,
1.34713509922151));
#74966=CARTESIAN_POINT('Ctrl Pts',(-2.5174184095497,-225.002301197522,1.38741669750801));
#74967=CARTESIAN_POINT('Origin',(0.,-225.,10.));
#74968=CARTESIAN_POINT('',(-2.52129902664413,-224.999094489651,2.38741669750801));
#74969=CARTESIAN_POINT('',(-2.51578360809179,-224.997885154191,2.11258330249199));
#74970=CARTESIAN_POINT('',(-2.5175,-225.,10.));
#74971=CARTESIAN_POINT('Ctrl Pts',(-2.51578360809179,-224.997885154191,
2.11258330249199));
#74972=CARTESIAN_POINT('Ctrl Pts',(-2.5178326768567,-224.740549886453,2.09633961766576));
#74973=CARTESIAN_POINT('Ctrl Pts',(-2.48151015149358,-224.483779262187,
2.08009593283954));
#74974=CARTESIAN_POINT('Ctrl Pts',(-2.40441279294324,-224.239898736946,
2.06385224801331));
#74975=CARTESIAN_POINT('Ctrl Pts',(-2.15324211360122,-223.445375573575,
2.01093295960272));
#74976=CARTESIAN_POINT('Ctrl Pts',(-1.46930748461902,-222.787661557655,
1.95801367119212));
#74977=CARTESIAN_POINT('Ctrl Pts',(-0.665577204289779,-222.567725340847,
1.90509438278152));
#74978=CARTESIAN_POINT('Ctrl Pts',(0.138153076039436,-222.347789124039,
1.85217509437092));
#74979=CARTESIAN_POINT('Ctrl Pts',(1.06167900771567,-222.565630706345,1.79925580596032));
#74980=CARTESIAN_POINT('Ctrl Pts',(1.6823947882024,-223.121568361418,1.74633651754973));
#74981=CARTESIAN_POINT('Ctrl Pts',(2.30311056868915,-223.677506016492,1.69341722913913));
#74982=CARTESIAN_POINT('Ctrl Pts',(2.62101619798637,-224.571539744334,1.64049794072853));
#74983=CARTESIAN_POINT('Ctrl Pts',(2.49063878605849,-225.394554494071,1.58757865231793));
#74984=CARTESIAN_POINT('Ctrl Pts',(2.36026137413062,-226.217569243809,1.53465936390734));
#74985=CARTESIAN_POINT('Ctrl Pts',(1.78160092097767,-226.969565015442,1.48174007549674));
#74986=CARTESIAN_POINT('Ctrl Pts',(1.01945097696467,-227.306439189746,1.42882078708614));
#74987=CARTESIAN_POINT('Ctrl Pts',(0.257301032951665,-227.643313364049,
1.37590149867554));
#74988=CARTESIAN_POINT('Ctrl Pts',(-0.688338401921387,-227.565065941023,
1.32298221026495));
#74989=CARTESIAN_POINT('Ctrl Pts',(-1.38473977240201,-227.107481348906,
1.27006292185435));
#74990=CARTESIAN_POINT('Ctrl Pts',(-2.07553403690411,-226.65358101907,1.21756971540023));
#74991=CARTESIAN_POINT('Ctrl Pts',(-2.52108758184044,-225.82642742821,1.16507650894611));
#74992=CARTESIAN_POINT('Ctrl Pts',(-2.52168724981252,-224.999862409999,
1.11258330249199));
#74993=CARTESIAN_POINT('Ctrl Pts',(-2.5174184095497,-225.002301197522,1.38741669750801));
#74994=CARTESIAN_POINT('Ctrl Pts',(-2.51924594585992,-225.20217974852,1.4000543876321));
#74995=CARTESIAN_POINT('Ctrl Pts',(-2.49744311761311,-225.401664370669,
1.4126920777562));
#74996=CARTESIAN_POINT('Ctrl Pts',(-2.4504865123205,-225.595040943422,1.42532976788029));
#74997=CARTESIAN_POINT('Ctrl Pts',(-2.25385958810712,-226.404789443731,
1.47824905629089));
#74998=CARTESIAN_POINT('Ctrl Pts',(-1.6161745722026,-227.107436549047,1.53116834470148));
#74999=CARTESIAN_POINT('Ctrl Pts',(-0.829237866958627,-227.381452880329,
1.58408763311208));
#75000=CARTESIAN_POINT('Ctrl Pts',(-0.0423011617146431,-227.65546921161,
1.63700692152268));
#75001=CARTESIAN_POINT('Ctrl Pts',(0.893887232868802,-227.500854768856,
1.68992620993328));
#75002=CARTESIAN_POINT('Ctrl Pts',(1.5509283882814,-226.988360171431,1.74284549834387));
#75003=CARTESIAN_POINT('Ctrl Pts',(2.207969543694,-226.475865574005,1.79576478675447));
#75004=CARTESIAN_POINT('Ctrl Pts',(2.58586345993575,-225.605490821907,1.84868407516507));
#75005=CARTESIAN_POINT('Ctrl Pts',(2.51168546372192,-224.775519850663,1.90160336357567));
#75006=CARTESIAN_POINT('Ctrl Pts',(2.43750746750809,-223.945548879419,1.95452265198626));
#75007=CARTESIAN_POINT('Ctrl Pts',(1.91125755883869,-223.155981689029,2.00744194039686));
#75008=CARTESIAN_POINT('Ctrl Pts',(1.17374789465563,-222.768123980806,2.06036122880746));
#75009=CARTESIAN_POINT('Ctrl Pts',(0.436238230472565,-222.380266272584,
2.11328051721805));
#75010=CARTESIAN_POINT('Ctrl Pts',(-0.512531189224167,-222.394118046529,
2.16619980562865));
#75011=CARTESIAN_POINT('Ctrl Pts',(-1.23840359958205,-222.803340844149,
2.21911909403925));
#75012=CARTESIAN_POINT('Ctrl Pts',(-1.96427600993995,-223.212563641768,
2.27203838244984));
#75013=CARTESIAN_POINT('Ctrl Pts',(-2.46725141095899,-224.017157463062,
2.32495767086044));
#75014=CARTESIAN_POINT('Ctrl Pts',(-2.5171682183347,-224.848940135592,2.37787695927104));
#75015=CARTESIAN_POINT('Ctrl Pts',(-2.52016771240887,-224.898921841723,
2.3810568720167));
#75016=CARTESIAN_POINT('Ctrl Pts',(-2.52153130634907,-224.949001721128,
2.38423678476236));
#75017=CARTESIAN_POINT('Ctrl Pts',(-2.52129902664413,-224.999094489651,
2.38741669750801));
#75018=CARTESIAN_POINT('Origin',(0.,-225.,10.));
#75019=CARTESIAN_POINT('',(-2.51474234901689,-224.998273792081,3.38741669750801));
#75020=CARTESIAN_POINT('',(-2.51418874373752,-225.001366293789,3.11258330249199));
#75021=CARTESIAN_POINT('',(-2.5175,-225.,10.));
#75022=CARTESIAN_POINT('Ctrl Pts',(-2.51418874373752,-225.001366293789,
3.11258330249199));
#75023=CARTESIAN_POINT('Ctrl Pts',(-2.5116814281143,-224.492634921714,3.08052201479602));
#75024=CARTESIAN_POINT('Ctrl Pts',(-2.36190816289223,-223.982546186139,
3.04846072710004));
#75025=CARTESIAN_POINT('Ctrl Pts',(-2.07504555938352,-223.567121570461,
3.01639943940406));
#75026=CARTESIAN_POINT('Ctrl Pts',(-1.60155974704675,-222.881435603683,
2.96348015099347));
#75027=CARTESIAN_POINT('Ctrl Pts',(-0.754591871553214,-222.453649713216,
2.91056086258287));
#75028=CARTESIAN_POINT('Ctrl Pts',(0.0782855864108173,-222.479518696041,
2.85764157417228));
#75029=CARTESIAN_POINT('Ctrl Pts',(0.911163044374884,-222.505387678867,
2.80472228576168));
#75030=CARTESIAN_POINT('Ctrl Pts',(1.72995008480944,-222.984911534986,2.75180299735108));
#75031=CARTESIAN_POINT('Ctrl Pts',(2.15996976906083,-223.698660193995,2.69888370894048));
#75032=CARTESIAN_POINT('Ctrl Pts',(2.5899894533122,-224.412408853004,2.64596442052988));
#75033=CARTESIAN_POINT('Ctrl Pts',(2.63124178138043,-225.360382314904,2.59304513211929));
#75034=CARTESIAN_POINT('Ctrl Pts',(2.26484969900841,-226.108787867573,2.54012584370869));
#75035=CARTESIAN_POINT('Ctrl Pts',(1.89845761663637,-226.857193420243,2.48720655529809));
#75036=CARTESIAN_POINT('Ctrl Pts',(1.12442112382405,-227.406031063681,2.43428726688749));
#75037=CARTESIAN_POINT('Ctrl Pts',(0.296939283634431,-227.50415285454,2.38136797847689));
#75038=CARTESIAN_POINT('Ctrl Pts',(-0.530542556555167,-227.6022746454,2.3284486900663));
#75039=CARTESIAN_POINT('Ctrl Pts',(-1.41146974412205,-227.24968058368,2.2755294016557));
#75040=CARTESIAN_POINT('Ctrl Pts',(-1.94272997305458,-226.60771739741,2.2226101132451));
#75041=CARTESIAN_POINT('Ctrl Pts',(-2.31091877796244,-226.162806136458,
2.18593450966073));
#75042=CARTESIAN_POINT('Ctrl Pts',(-2.51115714343535,-225.57890641684,2.14925890607636));
#75043=CARTESIAN_POINT('Ctrl Pts',(-2.51578360809179,-224.997885154191,
2.11258330249199));
#75044=CARTESIAN_POINT('Ctrl Pts',(-2.52129902664413,-224.999094489651,
2.38741669750801));
#75045=CARTESIAN_POINT('Ctrl Pts',(-2.51766576736073,-225.782632665356,
2.43715607317295));
#75046=CARTESIAN_POINT('Ctrl Pts',(-2.12357951610955,-226.569324345471,
2.4868954488379));
#75047=CARTESIAN_POINT('Ctrl Pts',(-1.49222055795853,-227.032789381898,
2.53663482450284));
#75048=CARTESIAN_POINT('Ctrl Pts',(-0.82049787647425,-227.525884431906,
2.58955411291343));
#75049=CARTESIAN_POINT('Ctrl Pts',(0.119805700226725,-227.653103008158,
2.64247340132403));
#75050=CARTESIAN_POINT('Ctrl Pts',(0.898407286222473,-227.356229879173,
2.69539268973463));
#75051=CARTESIAN_POINT('Ctrl Pts',(1.67700887221823,-227.059356750188,2.74831197814523));
#75052=CARTESIAN_POINT('Ctrl Pts',(2.29390846750877,-226.338391915967,2.80123126655583));
#75053=CARTESIAN_POINT('Ctrl Pts',(2.46681282336827,-225.523248877115,2.85415055496643));
#75054=CARTESIAN_POINT('Ctrl Pts',(2.63971717922775,-224.708105838262,2.90706984337702));
#75055=CARTESIAN_POINT('Ctrl Pts',(2.36862629565625,-223.798784594779,2.95998913178761));
#75056=CARTESIAN_POINT('Ctrl Pts',(1.7775913586249,-223.211390526533,3.01290842019821));
#75057=CARTESIAN_POINT('Ctrl Pts',(1.18655642159351,-222.623996458287,3.06582770860881));
#75058=CARTESIAN_POINT('Ctrl Pts',(0.275577431102228,-222.358529565279,
3.11874699701941));
#75059=CARTESIAN_POINT('Ctrl Pts',(-0.538481646178591,-222.53646749414,
3.17166628543));
#75060=CARTESIAN_POINT('Ctrl Pts',(-1.35254072345939,-222.714405423,3.2245855738406));
#75061=CARTESIAN_POINT('Ctrl Pts',(-2.06967988752974,-223.33574817373,3.2775048622512));
#75062=CARTESIAN_POINT('Ctrl Pts',(-2.36173627028926,-224.116169315018,
3.33042415066179));
#75063=CARTESIAN_POINT('Ctrl Pts',(-2.4665817029981,-224.396332999442,3.3494216662772));
#75064=CARTESIAN_POINT('Ctrl Pts',(-2.51664497692405,-224.696997767499,
3.36841918189261));
#75065=CARTESIAN_POINT('Ctrl Pts',(-2.51474234901689,-224.998273792081,
3.38741669750801));
#75066=CARTESIAN_POINT('Origin',(0.,-225.,10.));
#75067=CARTESIAN_POINT('',(-2.51505383944565,-225.001872855151,4.38741669750802));
#75068=CARTESIAN_POINT('',(-2.52076233832513,-225.001369535607,4.11258330249199));
#75069=CARTESIAN_POINT('',(-2.5175,-225.,10.));
#75070=CARTESIAN_POINT('Ctrl Pts',(-2.52076233832513,-225.001369535607,
4.11258330249199));
#75071=CARTESIAN_POINT('Ctrl Pts',(-2.51581109493886,-224.246714227313,
4.06470441192627));
#75072=CARTESIAN_POINT('Ctrl Pts',(-2.15430418959668,-223.487944707289,
4.01682552136055));
#75073=CARTESIAN_POINT('Ctrl Pts',(-1.56257694401589,-223.020780973236,
3.96894663079482));
#75074=CARTESIAN_POINT('Ctrl Pts',(-0.90855625975808,-222.504437087962,
3.91602734238422));
#75075=CARTESIAN_POINT('Ctrl Pts',(0.0267085927239957,-222.34432769804,
3.86310805397363));
#75076=CARTESIAN_POINT('Ctrl Pts',(0.81524043535916,-222.613718856892,3.81018876556303));
#75077=CARTESIAN_POINT('Ctrl Pts',(1.6037722779943,-222.883110015744,3.75726947715243));
#75078=CARTESIAN_POINT('Ctrl Pts',(2.24557111078254,-223.582001723371,3.70435018874184));
#75079=CARTESIAN_POINT('Ctrl Pts',(2.44694980038708,-224.390581148627,3.65143090033124));
#75080=CARTESIAN_POINT('Ctrl Pts',(2.64832848999163,-225.199160573883,3.59851161192064));
#75081=CARTESIAN_POINT('Ctrl Pts',(2.40928703641246,-226.117427716769,3.54559232351004));
#75082=CARTESIAN_POINT('Ctrl Pts',(1.83921080425351,-226.725183549692,3.49267303509944));
#75083=CARTESIAN_POINT('Ctrl Pts',(1.26913457209457,-227.332939382615,3.43975374668885));
#75084=CARTESIAN_POINT('Ctrl Pts',(0.368023561355883,-227.630183905574,
3.38683445827825));
#75085=CARTESIAN_POINT('Ctrl Pts',(-0.451773847463035,-227.480898032868,
3.33391516986765));
#75086=CARTESIAN_POINT('Ctrl Pts',(-1.27157125628195,-227.331612160162,
3.28099588145706));
#75087=CARTESIAN_POINT('Ctrl Pts',(-2.0100550631811,-226.73579589179,3.22807659304646));
#75088=CARTESIAN_POINT('Ctrl Pts',(-2.32929509204069,-225.966094736059,
3.17515730463586));
#75089=CARTESIAN_POINT('Ctrl Pts',(-2.45512272408338,-225.662719015438,
3.15429930392124));
#75090=CARTESIAN_POINT('Ctrl Pts',(-2.51581991936454,-225.332329897713,
3.13344130320662));
#75091=CARTESIAN_POINT('Ctrl Pts',(-2.51418874373752,-225.001366293789,
3.11258330249199));
#75092=CARTESIAN_POINT('Ctrl Pts',(-2.51474234901689,-224.998273792081,
3.38741669750801));
#75093=CARTESIAN_POINT('Ctrl Pts',(-2.51134503576355,-225.536229231171,
3.4213384703032));
#75094=CARTESIAN_POINT('Ctrl Pts',(-2.3422632039414,-226.076133558656,3.4552602430984));
#75095=CARTESIAN_POINT('Ctrl Pts',(-2.02352995235238,-226.50475294365,3.48918201589359));
#75096=CARTESIAN_POINT('Ctrl Pts',(-1.52629365020732,-227.173415899146,
3.54210130430419));
#75097=CARTESIAN_POINT('Ctrl Pts',(-0.66484744446852,-227.57124227829,3.59502059271479));
#75098=CARTESIAN_POINT('Ctrl Pts',(0.166610898230793,-227.516186737616,
3.64793988112538));
#75099=CARTESIAN_POINT('Ctrl Pts',(0.998069240930105,-227.461131196943,
3.70085916953598));
#75100=CARTESIAN_POINT('Ctrl Pts',(1.79953972058993,-226.953193736451,3.75377845794658));
#75101=CARTESIAN_POINT('Ctrl Pts',(2.20426946139026,-226.224806528169,3.80669774635718));
#75102=CARTESIAN_POINT('Ctrl Pts',(2.60899920219058,-225.496419319888,3.85961703476777));
#75103=CARTESIAN_POINT('Ctrl Pts',(2.61698820413141,-224.547582363817,3.91253632317837));
#75104=CARTESIAN_POINT('Ctrl Pts',(2.22458070012416,-223.812483432352,3.96545561158897));
#75105=CARTESIAN_POINT('Ctrl Pts',(1.83217319611691,-223.077384500887,4.01837489999956));
#75106=CARTESIAN_POINT('Ctrl Pts',(1.03936918616155,-222.556023594028,4.07129418841016));
#75107=CARTESIAN_POINT('Ctrl Pts',(0.208955769604636,-222.486975452526,
4.12421347682076));
#75108=CARTESIAN_POINT('Ctrl Pts',(-0.621457646952277,-222.417927311023,
4.17713276523135));
#75109=CARTESIAN_POINT('Ctrl Pts',(-1.48948047011075,-222.801191934877,
4.23005205364195));
#75110=CARTESIAN_POINT('Ctrl Pts',(-1.99790547305025,-223.461387439737,
4.28297134205255));
#75111=CARTESIAN_POINT('Ctrl Pts',(-2.33239365778951,-223.895724057166,
4.31778646053771));
#75112=CARTESIAN_POINT('Ctrl Pts',(-2.51124055525204,-224.449922020752,
4.35260157902286));
#75113=CARTESIAN_POINT('Ctrl Pts',(-2.51505383944565,-225.001872855151,
4.38741669750802));
#75114=CARTESIAN_POINT('Origin',(0.,-225.,10.));
#75115=CARTESIAN_POINT('',(-2.52148465865137,-225.000661258108,5.38741669750802));
#75116=CARTESIAN_POINT('',(-2.51831108560746,-224.997761985245,5.11258330249199));
#75117=CARTESIAN_POINT('',(-2.5175,-225.,10.));
#75118=CARTESIAN_POINT('Ctrl Pts',(-2.51831108560746,-224.997761985245,
5.11258330249199));
#75119=CARTESIAN_POINT('Ctrl Pts',(-2.51987989470443,-224.82746401479,5.10180609746711));
#75120=CARTESIAN_POINT('Ctrl Pts',(-2.50407988926802,-224.657455454451,
5.09102889244224));
#75121=CARTESIAN_POINT('Ctrl Pts',(-2.46984265276056,-224.491244722527,
5.08025168741736));
#75122=CARTESIAN_POINT('Ctrl Pts',(-2.30172761839515,-223.675100495958,
5.02733239900677));
#75123=CARTESIAN_POINT('Ctrl Pts',(-1.68907201582617,-222.950525811226,
4.97441311059617));
#75124=CARTESIAN_POINT('Ctrl Pts',(-0.912227036743379,-222.64908602982,
4.92149382218558));
#75125=CARTESIAN_POINT('Ctrl Pts',(-0.135382057660579,-222.347646248413,
4.86857453377498));
#75126=CARTESIAN_POINT('Ctrl Pts',(0.805652297936047,-222.469341370332,
4.81565524536438));
#75127=CARTESIAN_POINT('Ctrl Pts',(1.48025872742862,-222.958483710176,4.76273595695379));
#75128=CARTESIAN_POINT('Ctrl Pts',(2.15486515692122,-223.447626050019,4.70981666854319));
#75129=CARTESIAN_POINT('Ctrl Pts',(2.56304366030976,-224.304215607787,4.65689738013259));
#75130=CARTESIAN_POINT('Ctrl Pts',(2.51801176246824,-225.136277018694,4.60397809172199));
#75131=CARTESIAN_POINT('Ctrl Pts',(2.47297986462671,-225.968338429602,4.55105880331139));
#75132=CARTESIAN_POINT('Ctrl Pts',(1.97473756555515,-226.775871693649,4.4981395149008));
#75133=CARTESIAN_POINT('Ctrl Pts',(1.25128053151431,-227.18934960507,4.4452202264902));
#75134=CARTESIAN_POINT('Ctrl Pts',(0.527823497473455,-227.602827516492,
4.3923009380796));
#75135=CARTESIAN_POINT('Ctrl Pts',(-0.420848271536683,-227.622250075287,
4.339381649669));
#75136=CARTESIAN_POINT('Ctrl Pts',(-1.16062259267408,-227.238729518965,
4.2864623612584));
#75137=CARTESIAN_POINT('Ctrl Pts',(-1.90039691381146,-226.855208962643,
4.23354307284781));
#75138=CARTESIAN_POINT('Ctrl Pts',(-2.43127378707612,-226.068745291203,
4.18062378443721));
#75139=CARTESIAN_POINT('Ctrl Pts',(-2.51032396569167,-225.239224265169,
4.12770449602661));
#75140=CARTESIAN_POINT('Ctrl Pts',(-2.51785324966162,-225.160214964072,
4.12266409818174));
#75141=CARTESIAN_POINT('Ctrl Pts',(-2.52128357505804,-225.080815047912,
4.11762370033687));
#75142=CARTESIAN_POINT('Ctrl Pts',(-2.52076233832513,-225.001369535607,
4.11258330249199));
#75143=CARTESIAN_POINT('Ctrl Pts',(-2.51505383944565,-225.001872855151,
4.38741669750802));
#75144=CARTESIAN_POINT('Ctrl Pts',(-2.51703678099574,-225.288892176964,
4.40552086743346));
#75145=CARTESIAN_POINT('Ctrl Pts',(-2.4716890214524,-225.575303854349,4.4236250373589));
#75146=CARTESIAN_POINT('Ctrl Pts',(-2.37628370533025,-225.843937581591,
4.44172920728434));
#75147=CARTESIAN_POINT('Ctrl Pts',(-2.09740975195022,-226.629165832721,
4.49464849569494));
#75148=CARTESIAN_POINT('Ctrl Pts',(-1.39083466246961,-227.262495949115,
4.54756778410554));
#75149=CARTESIAN_POINT('Ctrl Pts',(-0.579887183939557,-227.454116081963,
4.60048707251614));
#75150=CARTESIAN_POINT('Ctrl Pts',(0.231060294590482,-227.64573621481,4.65340636092673));
#75151=CARTESIAN_POINT('Ctrl Pts',(1.14638016216995,-227.39564636411,4.70632564933733));
#75152=CARTESIAN_POINT('Ctrl Pts',(1.74722206539031,-226.818287640627,4.75924493774793));
#75153=CARTESIAN_POINT('Ctrl Pts',(2.34806396861067,-226.240928917144,4.81216422615853));
#75154=CARTESIAN_POINT('Ctrl Pts',(2.63442790747192,-225.336301320878,4.86508351456912));
#75155=CARTESIAN_POINT('Ctrl Pts',(2.47527374918222,-224.518362422092,4.91800280297972));
#75156=CARTESIAN_POINT('Ctrl Pts',(2.31611959089252,-223.700423523307,4.97092209139032));
#75157=CARTESIAN_POINT('Ctrl Pts',(1.71144733545193,-222.969173322003,5.02384137980092));
#75158=CARTESIAN_POINT('Ctrl Pts',(0.937954995060642,-222.659231895919,
5.07676066821151));
#75159=CARTESIAN_POINT('Ctrl Pts',(0.164462654669351,-222.349290469834,
5.12967995662211));
#75160=CARTESIAN_POINT('Ctrl Pts',(-0.777849770672657,-222.460657818971,
5.18259924503271));
#75161=CARTESIAN_POINT('Ctrl Pts',(-1.45778013365644,-222.942372246552,
5.23551853344331));
#75162=CARTESIAN_POINT('Ctrl Pts',(-2.10833167438353,-223.403272480038,
5.28615125479821));
#75163=CARTESIAN_POINT('Ctrl Pts',(-2.51868560060727,-224.2032068837,5.33678397615311));
#75164=CARTESIAN_POINT('Ctrl Pts',(-2.52148465865137,-225.000661258108,
5.38741669750802));
#75165=CARTESIAN_POINT('Origin',(0.,-225.,10.));
#75166=CARTESIAN_POINT('',(-2.51699551773447,-224.997707769369,6.38741669750802));
#75167=CARTESIAN_POINT('',(-2.51344103673693,-225.000035219284,6.11258330249199));
#75168=CARTESIAN_POINT('',(-2.5175,-225.,10.));
#75169=CARTESIAN_POINT('Ctrl Pts',(-2.51344103673693,-225.000035219284,
6.11258330249199));
#75170=CARTESIAN_POINT('Ctrl Pts',(-2.51338833654886,-224.577729214141,
6.08598849459737));
#75171=CARTESIAN_POINT('Ctrl Pts',(-2.41266892426312,-224.155399590225,
6.05939368670275));
#75172=CARTESIAN_POINT('Ctrl Pts',(-2.2114232112413,-223.788157583456,6.03279887880812));
#75173=CARTESIAN_POINT('Ctrl Pts',(-1.8109773809501,-223.057406462798,5.97987959039753));
#75174=CARTESIAN_POINT('Ctrl Pts',(-1.01250322696598,-222.544771713165,
5.92696030198693));
#75175=CARTESIAN_POINT('Ctrl Pts',(-0.181382506452433,-222.48483498591,
5.87404101357633));
#75176=CARTESIAN_POINT('Ctrl Pts',(0.649738214061123,-222.424898258654,
5.82112172516574));
#75177=CARTESIAN_POINT('Ctrl Pts',(1.51350550110408,-222.817659553777,5.76820243675514));
#75178=CARTESIAN_POINT('Ctrl Pts',(2.01465946110902,-223.483391310352,5.71528314834454));
#75179=CARTESIAN_POINT('Ctrl Pts',(2.51581342111396,-224.149123066927,5.66236385993394));
#75180=CARTESIAN_POINT('Ctrl Pts',(2.65435405408086,-225.087825284954,5.60944457152334));
#75181=CARTESIAN_POINT('Ctrl Pts',(2.36688516908806,-225.869947847921,5.55652528311275));
#75182=CARTESIAN_POINT('Ctrl Pts',(2.07941628409525,-226.652070410888,5.50360599470214));
#75183=CARTESIAN_POINT('Ctrl Pts',(1.36593788114273,-227.277613318795,5.45068670629155));
#75184=CARTESIAN_POINT('Ctrl Pts',(0.552937663393149,-227.460328149283,
5.39776741788095));
#75185=CARTESIAN_POINT('Ctrl Pts',(-0.260062554356385,-227.643042979771,
5.34484812947036));
#75186=CARTESIAN_POINT('Ctrl Pts',(-1.17258458690298,-227.382929732839,
5.29192884105976));
#75187=CARTESIAN_POINT('Ctrl Pts',(-1.76705837009536,-226.799016225171,
5.23900955264916));
#75188=CARTESIAN_POINT('Ctrl Pts',(-2.24046541116404,-226.334018821213,
5.19686746926344));
#75189=CARTESIAN_POINT('Ctrl Pts',(-2.51217657451406,-225.663677800595,
5.15472538587771));
#75190=CARTESIAN_POINT('Ctrl Pts',(-2.51831108560746,-224.997761985245,
5.11258330249199));
#75191=CARTESIAN_POINT('Ctrl Pts',(-2.52148465865137,-225.000661258108,
5.38741669750802));
#75192=CARTESIAN_POINT('Ctrl Pts',(-2.52161106374553,-225.036674193067,
5.38970326456371));
#75193=CARTESIAN_POINT('Ctrl Pts',(-2.52090629583595,-225.07268207022,5.39198983161941));
#75194=CARTESIAN_POINT('Ctrl Pts',(-2.51935494137685,-225.108653436226,
5.3942763986751));
#75195=CARTESIAN_POINT('Ctrl Pts',(-2.4834510854879,-225.941158692294,5.4471956870857));
#75196=CARTESIAN_POINT('Ctrl Pts',(-1.99409507308441,-226.754107698402,
5.5001149754963));
#75197=CARTESIAN_POINT('Ctrl Pts',(-1.27521620582045,-227.17549500534,5.55303426390689));
#75198=CARTESIAN_POINT('Ctrl Pts',(-0.556337338556501,-227.596882312277,
5.60595355231749));
#75199=CARTESIAN_POINT('Ctrl Pts',(0.392064383567916,-227.626707920045,
5.65887284072808));
#75200=CARTESIAN_POINT('Ctrl Pts',(1.13600035115615,-227.251323631115,5.71179212913868));
#75201=CARTESIAN_POINT('Ctrl Pts',(1.8799363187444,-226.875939342185,5.76471141754928));
#75202=CARTESIAN_POINT('Ctrl Pts',(2.41940653179646,-226.095345156556,5.81763070595987));
#75203=CARTESIAN_POINT('Ctrl Pts',(2.50754943142679,-225.266740958225,5.87054999437047));
#75204=CARTESIAN_POINT('Ctrl Pts',(2.59569233105713,-224.438136759894,5.92346928278107));
#75205=CARTESIAN_POINT('Ctrl Pts',(2.23250791726574,-223.56152254886,5.97638857119167));
#75206=CARTESIAN_POINT('Ctrl Pts',(1.58418937066262,-223.038036970857,6.02930785960227));
#75207=CARTESIAN_POINT('Ctrl Pts',(0.935870824059497,-222.514551392854,
6.08222714801287));
#75208=CARTESIAN_POINT('Ctrl Pts',(0.00241814464464793,-222.344194447881,
6.13514643642346));
#75209=CARTESIAN_POINT('Ctrl Pts',(-0.789020739835259,-222.604921470608,
6.18806572483406));
#75210=CARTESIAN_POINT('Ctrl Pts',(-1.58045962431517,-222.865648493336,
6.24098501324466));
#75211=CARTESIAN_POINT('Ctrl Pts',(-2.22988471386013,-223.557459483763,
6.29390430165526));
#75212=CARTESIAN_POINT('Ctrl Pts',(-2.44011910026339,-224.363781746274,
6.34682359006585));
#75213=CARTESIAN_POINT('Ctrl Pts',(-2.49387433955717,-224.569951854365,
6.36035462587991));
#75214=CARTESIAN_POINT('Ctrl Pts',(-2.5189160060991,-224.783608522892,6.37388566169396));
#75215=CARTESIAN_POINT('Ctrl Pts',(-2.51699551773447,-224.997707769369,
6.38741669750802));
#75216=CARTESIAN_POINT('Origin',(0.,-225.,10.));
#75217=CARTESIAN_POINT('',(-2.51364333654142,-225.000739863108,7.38741669750802));
#75218=CARTESIAN_POINT('',(-2.5184403423166,-225.002219538269,7.11258330249199));
#75219=CARTESIAN_POINT('',(-2.5175,-225.,10.));
#75220=CARTESIAN_POINT('Ctrl Pts',(-2.5184403423166,-225.002219538269,7.11258330249199));
#75221=CARTESIAN_POINT('Ctrl Pts',(-2.51228356404023,-224.332120591697,
7.07017089172762));
#75222=CARTESIAN_POINT('Ctrl Pts',(-2.23669070067441,-223.657549431312,
7.02775848096325));
#75223=CARTESIAN_POINT('Ctrl Pts',(-1.75786849029817,-223.192003033031,
6.98534607019888));
#75224=CARTESIAN_POINT('Ctrl Pts',(-1.16042707653199,-222.611126264295,
6.93242678178828));
#75225=CARTESIAN_POINT('Ctrl Pts',(-0.246591476022486,-222.355666176701,
6.87950749337768));
#75226=CARTESIAN_POINT('Ctrl Pts',(0.565467158405056,-222.54252130131,6.82658820496709));
#75227=CARTESIAN_POINT('Ctrl Pts',(1.3775257928326,-222.729376425919,6.77366891655649));
#75228=CARTESIAN_POINT('Ctrl Pts',(2.08780746117818,-223.358546762731,6.72074962814589));
#75229=CARTESIAN_POINT('Ctrl Pts',(2.37128728597244,-224.142123977991,6.6678303397353));
#75230=CARTESIAN_POINT('Ctrl Pts',(2.65476711076672,-224.925701193252,6.6149110513247));
#75231=CARTESIAN_POINT('Ctrl Pts',(2.51144509200964,-225.863685286961,6.5619917629141));
#75232=CARTESIAN_POINT('Ctrl Pts',(2.00690538266646,-226.526854756281,6.5090724745035));
#75233=CARTESIAN_POINT('Ctrl Pts',(1.5023656733233,-227.1900242256,6.4561531860929));
#75234=CARTESIAN_POINT('Ctrl Pts',(0.636608273394049,-227.578379070528,
6.4032338976823));
#75235=CARTESIAN_POINT('Ctrl Pts',(-0.194196247936209,-227.514208121664,
6.35031460927171));
#75236=CARTESIAN_POINT('Ctrl Pts',(-1.02500076926649,-227.450037172799,
6.29739532086111));
#75237=CARTESIAN_POINT('Ctrl Pts',(-1.82085241199778,-226.93334043014,6.24447603245051));
#75238=CARTESIAN_POINT('Ctrl Pts',(-2.21756948006428,-226.200558312969,
6.19155674403991));
#75239=CARTESIAN_POINT('Ctrl Pts',(-2.41491474003151,-225.836038888289,
6.16523226352394));
#75240=CARTESIAN_POINT('Ctrl Pts',(-2.51349320124512,-225.418048624316,
6.13890778300797));
#75241=CARTESIAN_POINT('Ctrl Pts',(-2.51344103673693,-225.000035219284,
6.11258330249199));
#75242=CARTESIAN_POINT('Ctrl Pts',(-2.51699551773447,-224.997707769369,
6.38741669750802));
#75243=CARTESIAN_POINT('Ctrl Pts',(-2.51140506022227,-225.620941298335,
6.42680495010456));
#75244=CARTESIAN_POINT('Ctrl Pts',(-2.27734630742311,-226.247925085029,
6.4661932027011));
#75245=CARTESIAN_POINT('Ctrl Pts',(-1.85802055608581,-226.704908942732,
6.50558145529765));
#75246=CARTESIAN_POINT('Ctrl Pts',(-1.29464394224344,-227.318880342084,
6.55850074370824));
#75247=CARTESIAN_POINT('Ctrl Pts',(-0.396847031297126,-227.625989606195,
6.61142003211884));
#75248=CARTESIAN_POINT('Ctrl Pts',(0.424538327956587,-227.485703541845,
6.66433932052944));
#75249=CARTESIAN_POINT('Ctrl Pts',(1.24592368721032,-227.345417477495,6.71725860894004));
#75250=CARTESIAN_POINT('Ctrl Pts',(1.99089749477147,-226.757736084685,6.77017789735063));
#75251=CARTESIAN_POINT('Ctrl Pts',(2.31855975094772,-225.991582357209,6.82309718576123));
#75252=CARTESIAN_POINT('Ctrl Pts',(2.64622200712396,-225.225428629734,6.87601647417183));
#75253=CARTESIAN_POINT('Ctrl Pts',(2.55657271191534,-224.280802567593,6.92893576258243));
#75254=CARTESIAN_POINT('Ctrl Pts',(2.09063538104663,-223.589965038249,6.98185505099302));
#75255=CARTESIAN_POINT('Ctrl Pts',(1.6246980501779,-222.899127508905,7.03477433940362));
#75256=CARTESIAN_POINT('Ctrl Pts',(0.782472683649099,-222.462078512358,
7.08769362781421));
#75257=CARTESIAN_POINT('Ctrl Pts',(-0.0506384073760926,-222.478811660835,
7.14061291622481));
#75258=CARTESIAN_POINT('Ctrl Pts',(-0.883749498401272,-222.495544809311,
7.19353220463541));
#75259=CARTESIAN_POINT('Ctrl Pts',(-1.70774631392282,-222.966060102812,
7.24645149304601));
#75260=CARTESIAN_POINT('Ctrl Pts',(-2.14556792735952,-223.675049752281,
7.29937078145661));
#75261=CARTESIAN_POINT('Ctrl Pts',(-2.388380495832,-224.068250070687,7.32871942014041));
#75262=CARTESIAN_POINT('Ctrl Pts',(-2.51241607461331,-224.534798615409,
7.35806805882421));
#75263=CARTESIAN_POINT('Ctrl Pts',(-2.51364333654142,-225.000739863108,
7.38741669750802));
#75264=CARTESIAN_POINT('Origin',(0.,-225.,10.));
#75265=CARTESIAN_POINT('',(-2.51970628537248,-225.001899922081,8.38741669750802));
#75266=CARTESIAN_POINT('',(-2.52066983009894,-224.998569141019,8.112583302492));
#75267=CARTESIAN_POINT('',(-2.5175,-225.,10.));
#75268=CARTESIAN_POINT('Ctrl Pts',(-2.52066983009894,-224.998569141019,
8.112583302492));
#75269=CARTESIAN_POINT('Ctrl Pts',(-2.52123860736442,-224.91485470247,8.10727257726847));
#75270=CARTESIAN_POINT('Ctrl Pts',(-2.5174295806041,-224.8311926478,8.10196185204495));
#75271=CARTESIAN_POINT('Ctrl Pts',(-2.50907240175204,-224.747987411985,
8.09665112682143));
#75272=CARTESIAN_POINT('Ctrl Pts',(-2.42579640095047,-223.918879957531,
8.04373183841083));
#75273=CARTESIAN_POINT('Ctrl Pts',(-1.89091897125145,-223.135131594655,
7.99081255000023));
#75274=CARTESIAN_POINT('Ctrl Pts',(-1.14920001396848,-222.755385558799,
7.93789326158963));
#75275=CARTESIAN_POINT('Ctrl Pts',(-0.407481056685504,-222.375639522944,
7.88497397317903));
#75276=CARTESIAN_POINT('Ctrl Pts',(0.541079428181421,-222.399895814108,
7.83205468476844));
#75277=CARTESIAN_POINT('Ctrl Pts',(1.26242018140782,-222.817054753933,7.77913539635784));
#75278=CARTESIAN_POINT('Ctrl Pts',(1.98376093463424,-223.234213693758,7.72621610794725));
#75279=CARTESIAN_POINT('Ctrl Pts',(2.47788195622012,-224.044275282243,7.67329681953665));
#75280=CARTESIAN_POINT('Ctrl Pts',(2.51867347640318,-224.876555352425,7.62037753112605));
#75281=CARTESIAN_POINT('Ctrl Pts',(2.55946499658623,-225.708835422607,7.56745824271545));
#75282=CARTESIAN_POINT('Ctrl Pts',(2.14692701536649,-226.563333974486,7.51453895430485));
#75283=CARTESIAN_POINT('Ctrl Pts',(1.46983690483877,-227.049032487523,7.46161966589425));
#75284=CARTESIAN_POINT('Ctrl Pts',(0.792746794311025,-227.534731000561,
7.40870037748366));
#75285=CARTESIAN_POINT('Ctrl Pts',(-0.148895445524709,-227.651629474756,
7.35578108907306));
#75286=CARTESIAN_POINT('Ctrl Pts',(-0.924194344234185,-227.346235170617,
7.30286180066246));
#75287=CARTESIAN_POINT('Ctrl Pts',(-1.69949324294364,-227.040840866477,
7.24994251225187));
#75288=CARTESIAN_POINT('Ctrl Pts',(-2.30844880052685,-226.313153784002,
7.19702322384126));
#75289=CARTESIAN_POINT('Ctrl Pts',(-2.47240296580703,-225.496163517825,
7.14410393543067));
#75290=CARTESIAN_POINT('Ctrl Pts',(-2.50495529986001,-225.333953914811,
7.13359705778444));
#75291=CARTESIAN_POINT('Ctrl Pts',(-2.51996556842092,-225.168223958098,
7.12309018013822));
#75292=CARTESIAN_POINT('Ctrl Pts',(-2.5184403423166,-225.002219538269,7.11258330249199));
#75293=CARTESIAN_POINT('Ctrl Pts',(-2.51364333654142,-225.000739863108,
7.38741669750802));
#75294=CARTESIAN_POINT('Ctrl Pts',(-2.51462898229289,-225.374949313199,
7.41098734723481));
#75295=CARTESIAN_POINT('Ctrl Pts',(-2.43640190115498,-225.748767049972,
7.43455799696161));
#75296=CARTESIAN_POINT('Ctrl Pts',(-2.27687376459592,-226.083882258337,
7.4581286466884));
#75297=CARTESIAN_POINT('Ctrl Pts',(-1.91871157704378,-226.836261109486,
7.511047935099));
#75298=CARTESIAN_POINT('Ctrl Pts',(-1.15074079058765,-227.393554806343,
7.5639672235096));
#75299=CARTESIAN_POINT('Ctrl Pts',(-0.32438482201001,-227.500745764186,
7.61688651192019));
#75300=CARTESIAN_POINT('Ctrl Pts',(0.501971146567617,-227.607936722028,
7.66980580033079));
#75301=CARTESIAN_POINT('Ctrl Pts',(1.38671229726677,-227.265024940856,7.72272508874138));
#75302=CARTESIAN_POINT('Ctrl Pts',(1.92498109692331,-226.628926844991,7.77564437715198));
#75303=CARTESIAN_POINT('Ctrl Pts',(2.46324989657986,-225.992828749126,7.82856366556258));
#75304=CARTESIAN_POINT('Ctrl Pts',(2.6550463451938,-225.063544338567,7.88148295397318));
#75305=CARTESIAN_POINT('Ctrl Pts',(2.4126043916505,-224.266314141316,7.93440224238378));
#75306=CARTESIAN_POINT('Ctrl Pts',(2.1701624381072,-223.469083944065,7.98732153079437));
#75307=CARTESIAN_POINT('Ctrl Pts',(1.49348208240664,-222.803907960121,8.04024081920497));
#75308=CARTESIAN_POINT('Ctrl Pts',(0.692212242012499,-222.575170706658,
8.09316010761557));
#75309=CARTESIAN_POINT('Ctrl Pts',(-0.109057598381629,-222.346433453194,
8.14607939602617));
#75310=CARTESIAN_POINT('Ctrl Pts',(-1.03491692346934,-222.554134930212,
8.19899868443676));
#75311=CARTESIAN_POINT('Ctrl Pts',(-1.66169252429475,-223.103230945912,
8.25191797284736));
#75312=CARTESIAN_POINT('Ctrl Pts',(-2.19664110423604,-223.571880544688,
8.29708421440091));
#75313=CARTESIAN_POINT('Ctrl Pts',(-2.51372206166214,-224.289219090568,
8.34225045595447));
#75314=CARTESIAN_POINT('Ctrl Pts',(-2.51970628537248,-225.001899922081,
8.38741669750802));
#75315=CARTESIAN_POINT('Origin',(0.,-225.,10.));
#75316=CARTESIAN_POINT('',(-2.51957010083597,-224.99805224078,9.38741669750802));
#75317=CARTESIAN_POINT('',(-2.51411989093267,-224.998691379972,9.112583302492));
#75318=CARTESIAN_POINT('',(-2.5175,-225.,10.));
#75319=CARTESIAN_POINT('Ctrl Pts',(-2.51411989093267,-224.998691379972,
9.112583302492));
#75320=CARTESIAN_POINT('Ctrl Pts',(-2.51569987828659,-224.663415377603,
9.09145497439872));
#75321=CARTESIAN_POINT('Ctrl Pts',(-2.45336473315411,-224.328702940348,
9.07032664630545));
#75322=CARTESIAN_POINT('Ctrl Pts',(-2.32434208855732,-224.0220488166,9.04919831821218));
#75323=CARTESIAN_POINT('Ctrl Pts',(-2.00118416944635,-223.25398435143,8.99627902980158));
#75324=CARTESIAN_POINT('Ctrl Pts',(-1.2596739510131,-222.661938781334,8.94335974139098));
#75325=CARTESIAN_POINT('Ctrl Pts',(-0.439126494633056,-222.516832147546,
8.89044045298038));
#75326=CARTESIAN_POINT('Ctrl Pts',(0.381420961746965,-222.371725513758,
8.83752116456979));
#75327=CARTESIAN_POINT('Ctrl Pts',(1.28100565607379,-222.673557816278,8.78460187615919));
#75328=CARTESIAN_POINT('Ctrl Pts',(1.84797764991111,-223.284210599409,8.73168258774859));
#75329=CARTESIAN_POINT('Ctrl Pts',(2.41494964374844,-223.89486338254,8.678763299338));
#75330=CARTESIAN_POINT('Ctrl Pts',(2.64930893709627,-224.81433664628,8.6258440109274));
#75331=CARTESIAN_POINT('Ctrl Pts',(2.44381272192663,-225.621879443221,8.5729247225168));
#75332=CARTESIAN_POINT('Ctrl Pts',(2.23831650675697,-226.429422240163,8.52000543410621));
#75333=CARTESIAN_POINT('Ctrl Pts',(1.59296478306982,-227.125034570305,8.46708614569561));
#75334=CARTESIAN_POINT('Ctrl Pts',(0.803070486935476,-227.390404245053,
8.41416685728501));
#75335=CARTESIAN_POINT('Ctrl Pts',(0.0131761908011642,-227.6557739198,8.36124756887441));
#75336=CARTESIAN_POINT('Ctrl Pts',(-0.921260677780323,-227.490900939152,
8.30832828046381));
#75337=CARTESIAN_POINT('Ctrl Pts',(-1.57264182611901,-226.971231175812,
8.25540899205322));
#75338=CARTESIAN_POINT('Ctrl Pts',(-2.15865349579485,-226.503712970117,
8.20780042886614));
#75339=CARTESIAN_POINT('Ctrl Pts',(-2.51557096558552,-225.749036161928,
8.16019186567907));
#75340=CARTESIAN_POINT('Ctrl Pts',(-2.52066983009894,-224.998569141019,
8.112583302492));
#75341=CARTESIAN_POINT('Ctrl Pts',(-2.51970628537248,-225.001899922081,
8.38741669750802));
#75342=CARTESIAN_POINT('Ctrl Pts',(-2.52073351201861,-225.124235712946,
8.39516974436506));
#75343=CARTESIAN_POINT('Ctrl Pts',(-2.51259405249524,-225.246434260949,
8.40292279122211));
#75344=CARTESIAN_POINT('Ctrl Pts',(-2.4948163577119,-225.367214148879,8.41067583807916));
#75345=CARTESIAN_POINT('Ctrl Pts',(-2.37347271374052,-226.191610781766,
8.46359512648976));
#75346=CARTESIAN_POINT('Ctrl Pts',(-1.80309354923468,-226.949913493158,
8.51651441490035));
#75347=CARTESIAN_POINT('Ctrl Pts',(-1.04468435865743,-227.295122977232,
8.56943370331095));
#75348=CARTESIAN_POINT('Ctrl Pts',(-0.286275168080149,-227.640332461307,
8.62235299172155));
#75349=CARTESIAN_POINT('Ctrl Pts',(0.660164048568542,-227.572448718064,
8.67527228013214));
#75350=CARTESIAN_POINT('Ctrl Pts',(1.36154272435913,-227.122535347076,8.72819156854274));
#75351=CARTESIAN_POINT('Ctrl Pts',(2.0629214001497,-226.672621976089,8.78111085695333));
#75352=CARTESIAN_POINT('Ctrl Pts',(2.51923953508218,-225.840678977357,8.83403014536393));
#75353=CARTESIAN_POINT('Ctrl Pts',(2.52168595958357,-225.007403450743,8.88694943377453));
#75354=CARTESIAN_POINT('Ctrl Pts',(2.52413238408496,-224.174127924128,8.93986872218513));
#75355=CARTESIAN_POINT('Ctrl Pts',(2.07270709815529,-223.339519869632,8.99278801059572));
#75356=CARTESIAN_POINT('Ctrl Pts',(1.37398230376001,-222.88549591658,9.04570729900632));
#75357=CARTESIAN_POINT('Ctrl Pts',(0.675257509364757,-222.431471963529,
9.09862658741692));
#75358=CARTESIAN_POINT('Ctrl Pts',(-0.270766793496115,-222.358032111923,
9.15154587582752));
#75359=CARTESIAN_POINT('Ctrl Pts',(-1.03118990243417,-222.698782436413,
9.20446516423812));
#75360=CARTESIAN_POINT('Ctrl Pts',(-1.79161301137223,-223.039532760903,
9.25738445264872));
#75361=CARTESIAN_POINT('Ctrl Pts',(-2.3664349263875,-223.794473261489,9.31030374105932));
#75362=CARTESIAN_POINT('Ctrl Pts',(-2.49261715047116,-224.618143179947,
9.36322302946991));
#75363=CARTESIAN_POINT('Ctrl Pts',(-2.51184650227261,-224.743665128426,
9.37128758548262));
#75364=CARTESIAN_POINT('Ctrl Pts',(-2.52065674398981,-224.870783233876,
9.37935214149532));
#75365=CARTESIAN_POINT('Ctrl Pts',(-2.51957010083597,-224.99805224078,9.38741669750802));
#75366=CARTESIAN_POINT('Origin',(0.,-225.,10.));
#75367=CARTESIAN_POINT('',(-2.51360219855143,-224.999337564491,10.387416697508));
#75368=CARTESIAN_POINT('',(-2.51589762297194,-225.002142026704,10.112583302492));
#75369=CARTESIAN_POINT('',(-2.5175,-225.,10.));
#75370=CARTESIAN_POINT('Ctrl Pts',(-2.51589762297194,-225.002142026704,
10.112583302492));
#75371=CARTESIAN_POINT('Ctrl Pts',(-2.51116128740118,-224.416905283918,
10.075637371529));
#75372=CARTESIAN_POINT('Ctrl Pts',(-2.30769417064104,-223.828699095673,
10.038691440566));
#75373=CARTESIAN_POINT('Ctrl Pts',(-1.93451257018931,-223.382404321986,
10.0017455096029));
#75374=CARTESIAN_POINT('Ctrl Pts',(-1.39998808456736,-222.74315660974,9.94882622119234));
#75375=CARTESIAN_POINT('Ctrl Pts',(-0.517275702770113,-222.395055744854,
9.89590693278174));
#75376=CARTESIAN_POINT('Ctrl Pts',(0.309695406647945,-222.497392676257,
9.84298764437114));
#75377=CARTESIAN_POINT('Ctrl Pts',(1.136666516066,-222.599729607659,9.79006835596054));
#75378=CARTESIAN_POINT('Ctrl Pts',(1.90789635310486,-223.15250433535,9.73714906754995));
#75379=CARTESIAN_POINT('Ctrl Pts',(2.27047015949948,-223.902767154805,9.68422977913935));
#75380=CARTESIAN_POINT('Ctrl Pts',(2.63304396589411,-224.653029974261,9.63131049072875));
#75381=CARTESIAN_POINT('Ctrl Pts',(2.58696174164449,-225.600780885482,9.57839120231815));
#75382=CARTESIAN_POINT('Ctrl Pts',(2.15331071166118,-226.312329090128,9.52547191390755));
#75383=CARTESIAN_POINT('Ctrl Pts',(1.71965968167787,-227.023877294775,9.47255262549696));
#75384=CARTESIAN_POINT('Ctrl Pts',(0.898439845960882,-227.499222792846,
9.41963333708636));
#75385=CARTESIAN_POINT('Ctrl Pts',(0.0654413851874604,-227.520847493772,
9.36671404867577));
#75386=CARTESIAN_POINT('Ctrl Pts',(-0.767557075585986,-227.542472194698,
9.31379476026517));
#75387=CARTESIAN_POINT('Ctrl Pts',(-1.61233416141586,-227.110376098477,
9.26087547185457));
#75388=CARTESIAN_POINT('Ctrl Pts',(-2.08231989443644,-226.422286370245,
9.20795618344397));
#75389=CARTESIAN_POINT('Ctrl Pts',(-2.36466113969728,-226.008920395343,
9.17616522312665));
#75390=CARTESIAN_POINT('Ctrl Pts',(-2.51174254640032,-225.503167931057,
9.14437426280932));
#75391=CARTESIAN_POINT('Ctrl Pts',(-2.51411989093267,-224.998691379972,
9.112583302492));
#75392=CARTESIAN_POINT('Ctrl Pts',(-2.51957010083597,-224.99805224078,9.38741669750802));
#75393=CARTESIAN_POINT('Ctrl Pts',(-2.51352623582953,-225.705917278637,
9.43227142990591));
#75394=CARTESIAN_POINT('Ctrl Pts',(-2.2013183640046,-226.418450512008,9.4771261623038));
#75395=CARTESIAN_POINT('Ctrl Pts',(-1.67280128041678,-226.886979270178,
9.5219808947017));
#75396=CARTESIAN_POINT('Ctrl Pts',(-1.04926065312667,-227.439746105621,
9.57490018311229));
#75397=CARTESIAN_POINT('Ctrl Pts',(-0.124636865394406,-227.652880440177,
9.62781947152289));
#75398=CARTESIAN_POINT('Ctrl Pts',(0.677962255693717,-227.428852006545,
9.68073875993349));
#75399=CARTESIAN_POINT('Ctrl Pts',(1.48056137678185,-227.204823572913,9.73365804834409));
#75400=CARTESIAN_POINT('Ctrl Pts',(2.16113583122583,-226.543632371092,9.78657733675469));
#75401=CARTESIAN_POINT('Ctrl Pts',(2.40825476205355,-225.747839482035,9.83949662516528));
#75402=CARTESIAN_POINT('Ctrl Pts',(2.65537369288127,-224.952046592978,9.89241591357588));
#75403=CARTESIAN_POINT('Ctrl Pts',(2.46903710009274,-224.021652016685,9.94533520198648));
#75404=CARTESIAN_POINT('Ctrl Pts',(1.93451260488425,-223.382404292974,9.99825449039708));
#75405=CARTESIAN_POINT('Ctrl Pts',(1.39998810967575,-222.743156569264,10.0511737788077));
#75406=CARTESIAN_POINT('Ctrl Pts',(0.517275712047266,-222.395055698135,
10.1040930672183));
#75407=CARTESIAN_POINT('Ctrl Pts',(-0.309695412202296,-222.497392631373,
10.1570123556289));
#75408=CARTESIAN_POINT('Ctrl Pts',(-1.13666653645184,-222.599729564611,
10.2099316440395));
#75409=CARTESIAN_POINT('Ctrl Pts',(-1.90789638732247,-223.152504302215,
10.2628509324501));
#75410=CARTESIAN_POINT('Ctrl Pts',(-2.27047020021974,-223.902767135127,
10.3157702208607));
#75411=CARTESIAN_POINT('Ctrl Pts',(-2.43409759707822,-224.241356271855,
10.3396523797431));
#75412=CARTESIAN_POINT('Ctrl Pts',(-2.51449553043366,-224.620167078381,
10.3635345386256));
#75413=CARTESIAN_POINT('Ctrl Pts',(-2.51360219855143,-224.999337564491,
10.387416697508));
#75414=CARTESIAN_POINT('Origin',(0.,-225.,10.));
#75415=CARTESIAN_POINT('',(-2.51714215352465,-225.002298253916,11.387416697508));
#75416=CARTESIAN_POINT('',(-2.52169612886588,-225.000045821236,11.112583302492));
#75417=CARTESIAN_POINT('',(-2.5175,-225.,10.));
#75418=CARTESIAN_POINT('Ctrl Pts',(-2.5216957256514,-225.000045816832,11.112583302492));
#75419=CARTESIAN_POINT('Ctrl Pts',(-2.52147288364372,-224.169218319319,
11.0598197686592));
#75420=CARTESIAN_POINT('Ctrl Pts',(-2.07065054082289,-223.338183594447,
11.0070562348265));
#75421=CARTESIAN_POINT('Ctrl Pts',(-1.37398227911805,-222.885495954503,
10.9542927009937));
#75422=CARTESIAN_POINT('Ctrl Pts',(-0.675257497254214,-222.431472009595,
10.9013734125831));
#75423=CARTESIAN_POINT('Ctrl Pts',(0.270766788639961,-222.358032159306,
10.8484541241725));
#75424=CARTESIAN_POINT('Ctrl Pts',(1.03118988394006,-222.698782477684,10.7955348357619));
#75425=CARTESIAN_POINT('Ctrl Pts',(1.79161297924015,-223.039532796063,10.7426155473513));
#75426=CARTESIAN_POINT('Ctrl Pts',(2.36643488394616,-223.79447328311,10.6896962589407));
#75427=CARTESIAN_POINT('Ctrl Pts',(2.49261710576678,-224.618143186796,10.6367769705301));
#75428=CARTESIAN_POINT('Ctrl Pts',(2.6187993275874,-225.441813090481,10.5838576821195));
#75429=CARTESIAN_POINT('Ctrl Pts',(2.29634186652262,-226.334212410806,10.5309383937089));
#75430=CARTESIAN_POINT('Ctrl Pts',(1.67280125041553,-226.886979236335,10.4780191052983));
#75431=CARTESIAN_POINT('Ctrl Pts',(1.04926063430843,-227.439746061865,10.4250998168877));
#75432=CARTESIAN_POINT('Ctrl Pts',(0.124636863159021,-227.652880392599,
10.3721805284771));
#75433=CARTESIAN_POINT('Ctrl Pts',(-0.677962243534711,-227.428851962984,
10.3192612400665));
#75434=CARTESIAN_POINT('Ctrl Pts',(-1.48056135022843,-227.20482353337,10.2663419516559));
#75435=CARTESIAN_POINT('Ctrl Pts',(-2.16113579246647,-226.543632343407,
10.2134226632453));
#75436=CARTESIAN_POINT('Ctrl Pts',(-2.40825471886219,-225.747839468623,
10.1605033748347));
#75437=CARTESIAN_POINT('Ctrl Pts',(-2.48284602690762,-225.507634348241,
10.1445300173872));
#75438=CARTESIAN_POINT('Ctrl Pts',(-2.51794534999063,-225.25516571403,10.1285566599396));
#75439=CARTESIAN_POINT('Ctrl Pts',(-2.51589762297194,-225.002142026704,
10.112583302492));
#75440=CARTESIAN_POINT('Ctrl Pts',(-2.51360219855143,-224.999337564491,
10.387416697508));
#75441=CARTESIAN_POINT('Ctrl Pts',(-2.51251604073364,-225.460352105623,
10.4164538270362));
#75442=CARTESIAN_POINT('Ctrl Pts',(-2.39125766399852,-225.92189835817,10.4454909565643));
#75443=CARTESIAN_POINT('Ctrl Pts',(-2.15331075028016,-226.312329113665,
10.4745280860925));
#75444=CARTESIAN_POINT('Ctrl Pts',(-1.71965971251943,-227.023877331072,
10.5274473745031));
#75445=CARTESIAN_POINT('Ctrl Pts',(-0.898439862074109,-227.499222837669,
10.5803666629136));
#75446=CARTESIAN_POINT('Ctrl Pts',(-0.0654413863611154,-227.520847538983,
10.6332859513242));
#75447=CARTESIAN_POINT('Ctrl Pts',(0.767557089351907,-227.542472240296,
10.6862052397348));
#75448=CARTESIAN_POINT('Ctrl Pts',(1.6123341903326,-227.110376136326,10.7391245281454));
#75449=CARTESIAN_POINT('Ctrl Pts',(2.08231993178224,-226.422286395754,10.792043816556));
#75450=CARTESIAN_POINT('Ctrl Pts',(2.55230567323187,-225.734196655181,10.8449631049666));
#75451=CARTESIAN_POINT('Ctrl Pts',(2.64750005515044,-224.790113278006,10.8978823933772));
#75452=CARTESIAN_POINT('Ctrl Pts',(2.32434213024372,-224.022048799061,10.9508016817878));
#75453=CARTESIAN_POINT('Ctrl Pts',(2.001184205337,-223.253984320116,11.0037209701984));
#75454=CARTESIAN_POINT('Ctrl Pts',(1.259673973605,-222.661938739401,11.056640258609));
#75455=CARTESIAN_POINT('Ctrl Pts',(0.439126502508681,-222.516832103011,
11.1095595470196));
#75456=CARTESIAN_POINT('Ctrl Pts',(-0.381420968587641,-222.37172546662,
11.1624788354302));
#75457=CARTESIAN_POINT('Ctrl Pts',(-1.28100567904826,-222.673557774554,
11.2153981238408));
#75458=CARTESIAN_POINT('Ctrl Pts',(-1.84797768305408,-223.284210568637,
11.2683174122514));
#75459=CARTESIAN_POINT('Ctrl Pts',(-2.27331699042637,-223.742318966661,
11.3080171740036));
#75460=CARTESIAN_POINT('Ctrl Pts',(-2.51146457315667,-224.374229021343,
11.3477169357558));
#75461=CARTESIAN_POINT('Ctrl Pts',(-2.51714215352465,-225.002298253916,
11.387416697508));
#75462=CARTESIAN_POINT('Origin',(0.,-225.,10.));
#75463=CARTESIAN_POINT('',(-2.52142583271238,-224.999252289457,12.387416697508));
#75464=CARTESIAN_POINT('',(-2.51603114701545,-224.9978289772,12.112583302492));
#75465=CARTESIAN_POINT('',(-2.5175,-225.,10.));
#75466=CARTESIAN_POINT('Ctrl Pts',(-2.51603114701545,-224.9978289772,12.112583302492));
#75467=CARTESIAN_POINT('Ctrl Pts',(-2.51807401653,-224.749773018184,12.0969214542001));
#75468=CARTESIAN_POINT('Ctrl Pts',(-2.48435680654783,-224.502260225447,
12.0812596059082));
#75469=CARTESIAN_POINT('Ctrl Pts',(-2.41260434838113,-224.266314154475,
12.0655977576162));
#75470=CARTESIAN_POINT('Ctrl Pts',(-2.17016239918595,-223.469083971522,
12.0126784692056));
#75471=CARTESIAN_POINT('Ctrl Pts',(-1.49348205562143,-222.803907999507,
11.959759180795));
#75472=CARTESIAN_POINT('Ctrl Pts',(-0.69221222959782,-222.575170750146,
11.9068398923844));
#75473=CARTESIAN_POINT('Ctrl Pts',(0.109057596425746,-222.346433500785,
11.8539206039738));
#75474=CARTESIAN_POINT('Ctrl Pts',(1.0349169049084,-222.554134974078,11.8010013155632));
#75475=CARTESIAN_POINT('Ctrl Pts',(1.66169249449276,-223.10323097993,11.7480820271526));
#75476=CARTESIAN_POINT('Ctrl Pts',(2.28846808407714,-223.652326985781,11.6951627387421));
#75477=CARTESIAN_POINT('Ctrl Pts',(2.61615995476321,-224.542817524192,11.6422434503315));
#75478=CARTESIAN_POINT('Ctrl Pts',(2.49481631296809,-225.367214142293,11.5893241619209));
#75479=CARTESIAN_POINT('Ctrl Pts',(2.37347267117298,-226.191610760395,11.5364048735103));
#75480=CARTESIAN_POINT('Ctrl Pts',(1.80309351689672,-226.949913458187,11.4834855850997));
#75481=CARTESIAN_POINT('Ctrl Pts',(1.0446843399213,-227.29512293607,11.4305662966891));
#75482=CARTESIAN_POINT('Ctrl Pts',(0.286275162945881,-227.640332413953,
11.3776470082785));
#75483=CARTESIAN_POINT('Ctrl Pts',(-0.660164036728685,-227.572448671928,
11.3247277198679));
#75484=CARTESIAN_POINT('Ctrl Pts',(-1.36154269994023,-227.122535309009,
11.2718084314573));
#75485=CARTESIAN_POINT('Ctrl Pts',(-2.0629213631518,-226.672621946091,11.2188891430467));
#75486=CARTESIAN_POINT('Ctrl Pts',(-2.51923948990035,-225.84067896228,11.1659698546361));
#75487=CARTESIAN_POINT('Ctrl Pts',(-2.52168591435786,-225.00740345061,11.1130505662255));
#75488=CARTESIAN_POINT('Ctrl Pts',(-2.5216931147912,-225.004950914315,11.1128948116477));
#75489=CARTESIAN_POINT('Ctrl Pts',(-2.52169638346675,-225.002498366477,
11.1127390570698));
#75490=CARTESIAN_POINT('Ctrl Pts',(-2.5216957256514,-225.000045816832,11.112583302492));
#75491=CARTESIAN_POINT('Ctrl Pts',(-2.51714215352465,-225.002298253916,
11.387416697508));
#75492=CARTESIAN_POINT('Ctrl Pts',(-2.51903271713805,-225.211437492965,
11.4006362241664));
#75493=CARTESIAN_POINT('Ctrl Pts',(-2.49514684119296,-225.420150858922,
11.4138557508248));
#75494=CARTESIAN_POINT('Ctrl Pts',(-2.44381276575569,-225.621879454375,
11.4270752774832));
#75495=CARTESIAN_POINT('Ctrl Pts',(-2.23831654690051,-226.429422265799,
11.4799945658938));
#75496=CARTESIAN_POINT('Ctrl Pts',(-1.59296481163917,-227.125034608417,
11.5329138543044));
#75497=CARTESIAN_POINT('Ctrl Pts',(-0.803070501338331,-227.390404287924,
11.585833142715));
#75498=CARTESIAN_POINT('Ctrl Pts',(-0.013176191037481,-227.65577396743,
11.6387524311256));
#75499=CARTESIAN_POINT('Ctrl Pts',(0.921260694302875,-227.490900983826,
11.6916717195362));
#75500=CARTESIAN_POINT('Ctrl Pts',(1.5726418543239,-226.971231211165,11.7445910079468));
#75501=CARTESIAN_POINT('Ctrl Pts',(2.22402301434493,-226.451561438505,11.7975102963574));
#75502=CARTESIAN_POINT('Ctrl Pts',(2.59234844904663,-225.577094876789,11.850429584768));
#75503=CARTESIAN_POINT('Ctrl Pts',(2.50907244675153,-224.747987407465,11.9033488731786));
#75504=CARTESIAN_POINT('Ctrl Pts',(2.42579644445644,-223.918879938141,11.9562681615892));
#75505=CARTESIAN_POINT('Ctrl Pts',(1.89091900516453,-223.135131561209,12.0091874499998));
#75506=CARTESIAN_POINT('Ctrl Pts',(1.14920003457903,-222.755385518543,12.0621067384104));
#75507=CARTESIAN_POINT('Ctrl Pts',(0.407481063993527,-222.375639475876,
12.115026026821));
#75508=CARTESIAN_POINT('Ctrl Pts',(-0.541079437885564,-222.399895767476,
12.1679453152316));
#75509=CARTESIAN_POINT('Ctrl Pts',(-1.26242020404901,-222.817054714783,
12.2208646036422));
#75510=CARTESIAN_POINT('Ctrl Pts',(-1.98376097021244,-223.234213662089,
12.2737838920528));
#75511=CARTESIAN_POINT('Ctrl Pts',(-2.47788200066022,-224.044275265102,
12.3267031804634));
#75512=CARTESIAN_POINT('Ctrl Pts',(-2.51867352157486,-224.876555350211,
12.379622468874));
#75513=CARTESIAN_POINT('Ctrl Pts',(-2.52067618418232,-224.917416199917,
12.3822205450853));
#75514=CARTESIAN_POINT('Ctrl Pts',(-2.52158617489675,-224.958330603408,
12.3848186212967));
#75515=CARTESIAN_POINT('Ctrl Pts',(-2.52142583271238,-224.999252289457,
12.387416697508));
#75516=CARTESIAN_POINT('Origin',(0.,-225.,10.));
#75517=CARTESIAN_POINT('',(-2.51494210236921,-224.998176172471,13.387416697508));
#75518=CARTESIAN_POINT('',(-2.51404438929022,-225.001240667286,13.112583302492));
#75519=CARTESIAN_POINT('',(-2.5175,-225.,10.));
#75520=CARTESIAN_POINT('Ctrl Pts',(-2.51404438929022,-225.001240667286,
13.112583302492));
#75521=CARTESIAN_POINT('Ctrl Pts',(-2.51181653950388,-224.501669767605,
13.0811038513303));
#75522=CARTESIAN_POINT('Ctrl Pts',(-2.36780179134328,-224.000915144855,
13.0496244001687));
#75523=CARTESIAN_POINT('Ctrl Pts',(-2.09063534355168,-223.589965063538,
13.018144949007));
#75524=CARTESIAN_POINT('Ctrl Pts',(-1.62469802103941,-222.899127546584,
12.9652256605964));
#75525=CARTESIAN_POINT('Ctrl Pts',(-0.782472669615672,-222.462078557875,
12.9123063721858));
#75526=CARTESIAN_POINT('Ctrl Pts',(0.0506384064679075,-222.478811706052,
12.8593870837752));
#75527=CARTESIAN_POINT('Ctrl Pts',(0.883749482551476,-222.495544854228,
12.8064677953646));
#75528=CARTESIAN_POINT('Ctrl Pts',(1.70774628329489,-222.96606013929,12.753548506954));
#75529=CARTESIAN_POINT('Ctrl Pts',(2.14556788887937,-223.675049776044,12.7006292185434));
#75530=CARTESIAN_POINT('Ctrl Pts',(2.58338949446386,-224.384039412798,12.6477099301328));
#75531=CARTESIAN_POINT('Ctrl Pts',(2.63503590488944,-225.331503401244,12.5947906417222));
#75532=CARTESIAN_POINT('Ctrl Pts',(2.27687372376085,-226.083882238898,12.5418713533116));
#75533=CARTESIAN_POINT('Ctrl Pts',(1.91871154263225,-226.836261076553,12.488952064901));
#75534=CARTESIAN_POINT('Ctrl Pts',(1.15074076994946,-227.393554763416,12.4360327764904));
#75535=CARTESIAN_POINT('Ctrl Pts',(0.32438481619228,-227.500745719336,12.3831134880798));
#75536=CARTESIAN_POINT('Ctrl Pts',(-0.501971137564902,-227.607936675256,
12.3301941996692));
#75537=CARTESIAN_POINT('Ctrl Pts',(-1.38671227239649,-227.265024900234,
12.2772749112586));
#75538=CARTESIAN_POINT('Ctrl Pts',(-1.92498106239934,-226.628926815777,
12.224355622848));
#75539=CARTESIAN_POINT('Ctrl Pts',(-2.30394528912289,-226.181086585814,
12.1870981827293));
#75540=CARTESIAN_POINT('Ctrl Pts',(-2.51117143396052,-225.587920891441,
12.1498407426107));
#75541=CARTESIAN_POINT('Ctrl Pts',(-2.51603114701545,-224.9978289772,12.112583302492));
#75542=CARTESIAN_POINT('Ctrl Pts',(-2.52142583271238,-224.999252289457,
12.387416697508));
#75543=CARTESIAN_POINT('Ctrl Pts',(-2.51832022208835,-225.791849842305,
12.4377379097073));
#75544=CARTESIAN_POINT('Ctrl Pts',(-2.11368526635859,-226.587179405838,
12.4880591219065));
#75545=CARTESIAN_POINT('Ctrl Pts',(-1.46983693119985,-227.049032524272,
12.5383803341058));
#75546=CARTESIAN_POINT('Ctrl Pts',(-0.792746808528703,-227.53473104602,
12.5912996225164));
#75547=CARTESIAN_POINT('Ctrl Pts',(0.148895448195099,-227.651629522312,
12.644218910927));
#75548=CARTESIAN_POINT('Ctrl Pts',(0.92419436080933,-227.346235212695,12.6971381993376));
#75549=CARTESIAN_POINT('Ctrl Pts',(1.69949327342356,-227.040840903079,12.7500574877481));
#75550=CARTESIAN_POINT('Ctrl Pts',(2.30844884192822,-226.313153807553,12.8029767761587));
#75551=CARTESIAN_POINT('Ctrl Pts',(2.47240301014887,-225.496163526723,12.8558960645693));
#75552=CARTESIAN_POINT('Ctrl Pts',(2.63635717836953,-224.679173245894,12.9088153529799));
#75553=CARTESIAN_POINT('Ctrl Pts',(2.35530994630617,-223.77287977976,12.9617346413905));
#75554=CARTESIAN_POINT('Ctrl Pts',(1.75786852182505,-223.192003000605,13.0146539298011));
#75555=CARTESIAN_POINT('Ctrl Pts',(1.16042709734392,-222.611126221451,13.0675732182117));
#75556=CARTESIAN_POINT('Ctrl Pts',(0.246591480445025,-222.355666129275,
13.1204925066223));
#75557=CARTESIAN_POINT('Ctrl Pts',(-0.565467168546566,-222.542521257235,
13.1734117950329));
#75558=CARTESIAN_POINT('Ctrl Pts',(-1.37752581753814,-222.729376385196,
13.2263310834435));
#75559=CARTESIAN_POINT('Ctrl Pts',(-2.08780749862242,-223.358546733292,
13.2792503718541));
#75560=CARTESIAN_POINT('Ctrl Pts',(-2.3712873285008,-224.142123962606,13.3321696602647));
#75561=CARTESIAN_POINT('Ctrl Pts',(-2.46993705962531,-224.414805384138,
13.3505853393458));
#75562=CARTESIAN_POINT('Ctrl Pts',(-2.51690068886609,-224.706185622866,
13.3690010184269));
#75563=CARTESIAN_POINT('Ctrl Pts',(-2.51494210236921,-224.998176172471,
13.387416697508));
#75564=CARTESIAN_POINT('Origin',(0.,-225.,10.));
#75565=CARTESIAN_POINT('',(-2.51484781591379,-225.001779432988,14.387416697508));
#75566=CARTESIAN_POINT('',(-2.52055923806654,-225.001499367411,14.112583302492));
#75567=CARTESIAN_POINT('',(-2.5175,-225.,10.));
#75568=CARTESIAN_POINT('Ctrl Pts',(-2.52055923806654,-225.001499367411,
14.112583302492));
#75569=CARTESIAN_POINT('Ctrl Pts',(-2.51530324437999,-224.255856698468,
14.0652862484606));
#75570=CARTESIAN_POINT('Ctrl Pts',(-2.1636294235382,-223.505906585683,14.0179891944292));
#75571=CARTESIAN_POINT('Ctrl Pts',(-1.58418934225064,-223.038037006044,
13.9706921403977));
#75572=CARTESIAN_POINT('Ctrl Pts',(-0.935870807274923,-222.51455143743,
13.9177728519872));
#75573=CARTESIAN_POINT('Ctrl Pts',(-0.00241814460127818,-222.344194495512,
13.8648535635766));
#75574=CARTESIAN_POINT('Ctrl Pts',(0.789020725684399,-222.604921513563,
13.811934275166));
#75575=CARTESIAN_POINT('Ctrl Pts',(1.58045959597008,-222.865648531615,13.7590149867554));
#75576=CARTESIAN_POINT('Ctrl Pts',(2.22988467386778,-223.557459509635,13.7060956983448));
#75577=CARTESIAN_POINT('Ctrl Pts',(2.44011905650055,-224.363781757685,13.6531764099342));
#75578=CARTESIAN_POINT('Ctrl Pts',(2.65035343913332,-225.170104005735,13.6002571215236));
#75579=CARTESIAN_POINT('Ctrl Pts',(2.42139712650114,-226.090937523814,13.547337833113));
#75580=CARTESIAN_POINT('Ctrl Pts',(1.85802052276276,-226.704908912155,13.4944185447024));
#75581=CARTESIAN_POINT('Ctrl Pts',(1.29464391902438,-227.318880300496,13.4414992562918));
#75582=CARTESIAN_POINT('Ctrl Pts',(0.396847024179783,-227.625989559098,
13.3885799678812));
#75583=CARTESIAN_POINT('Ctrl Pts',(-0.424538320342631,-227.485703497264,
13.3356606794706));
#75584=CARTESIAN_POINT('Ctrl Pts',(-1.24592366486505,-227.345417435431,
13.28274139106));
#75585=CARTESIAN_POINT('Ctrl Pts',(-1.99089745906529,-226.757736053161,
13.2298221026494));
#75586=CARTESIAN_POINT('Ctrl Pts',(-2.31855970936501,-225.991582339426,
13.1769028142388));
#75587=CARTESIAN_POINT('Ctrl Pts',(-2.45130951628865,-225.681181133675,
13.1554629769899));
#75588=CARTESIAN_POINT('Ctrl Pts',(-2.51556171996378,-225.341485442472,
13.1340231397409));
#75589=CARTESIAN_POINT('Ctrl Pts',(-2.51404438929022,-225.001240667286,
13.112583302492));
#75590=CARTESIAN_POINT('Ctrl Pts',(-2.51494210236921,-224.998176172471,
13.387416697508));
#75591=CARTESIAN_POINT('Ctrl Pts',(-2.51127249545279,-225.545249555271,
13.4219203068375));
#75592=CARTESIAN_POINT('Ctrl Pts',(-2.33586753922983,-226.094465358442,
13.456423916167));
#75593=CARTESIAN_POINT('Ctrl Pts',(-2.00690541865975,-226.526854783664,
13.4909275254965));
#75594=CARTESIAN_POINT('Ctrl Pts',(-1.5023657002678,-227.190024264877,13.5438468139071));
#75595=CARTESIAN_POINT('Ctrl Pts',(-0.636608284811431,-227.578379116771,
13.5967661023177));
#75596=CARTESIAN_POINT('Ctrl Pts',(0.19419625141908,-227.514208166755,13.6496853907283));
#75597=CARTESIAN_POINT('Ctrl Pts',(1.02500078764959,-227.450037216739,13.7026046791389));
#75598=CARTESIAN_POINT('Ctrl Pts',(1.82085244465424,-226.933340464814,13.7555239675495));
#75599=CARTESIAN_POINT('Ctrl Pts',(2.21756951983575,-226.200558334501,13.8084432559601));
#75600=CARTESIAN_POINT('Ctrl Pts',(2.61428659501725,-225.467776204187,13.8613625443707));
#75601=CARTESIAN_POINT('Ctrl Pts',(2.61186908837563,-224.518908695486,13.9142818327813));
#75602=CARTESIAN_POINT('Ctrl Pts',(2.21142325090253,-223.788157561722,13.9672011211919));
#75603=CARTESIAN_POINT('Ctrl Pts',(1.81097741342944,-223.057406427958,14.0201204096025));
#75604=CARTESIAN_POINT('Ctrl Pts',(1.01250324512489,-222.544771669131,14.0730396980131));
#75605=CARTESIAN_POINT('Ctrl Pts',(0.181382509705423,-222.484834940801,
14.1259589864237));
#75606=CARTESIAN_POINT('Ctrl Pts',(-0.649738225714033,-222.424898212471,
14.1788782748343));
#75607=CARTESIAN_POINT('Ctrl Pts',(-1.5135055282484,-222.817659514637,14.2317975632449));
#75608=CARTESIAN_POINT('Ctrl Pts',(-2.01465949724137,-223.483391283152,
14.2847168516555));
#75609=CARTESIAN_POINT('Ctrl Pts',(-2.33885405156362,-223.914050576194,
14.3189501336063));
#75610=CARTESIAN_POINT('Ctrl Pts',(-2.51130414328076,-224.458941070606,
14.3531834155572));
#75611=CARTESIAN_POINT('Ctrl Pts',(-2.51484781591379,-225.001779432988,
14.387416697508));
#75612=CARTESIAN_POINT('Origin',(0.,-225.,10.));
#75613=CARTESIAN_POINT('',(-2.52136959094702,-225.00082166017,15.387416697508));
#75614=CARTESIAN_POINT('',(-2.51858868022655,-224.99780466334,15.112583302492));
#75615=CARTESIAN_POINT('',(-2.5175,-225.,10.));
#75616=CARTESIAN_POINT('Ctrl Pts',(-2.51858868022655,-224.99780466334,15.112583302492));
#75617=CARTESIAN_POINT('Ctrl Pts',(-2.52006212821327,-224.836746398224,
15.1023879340014));
#75618=CARTESIAN_POINT('Ctrl Pts',(-2.50593615906982,-224.675945583807,
15.0921925655109));
#75619=CARTESIAN_POINT('Ctrl Pts',(-2.4752737047889,-224.51836243073,15.0819971970203));
#75620=CARTESIAN_POINT('Ctrl Pts',(-2.3161195493536,-223.700423546615,15.0290779086097));
#75621=CARTESIAN_POINT('Ctrl Pts',(-1.71144730475761,-222.969173358425,
14.9761586201991));
#75622=CARTESIAN_POINT('Ctrl Pts',(-0.937954978238689,-222.6592319379,14.9232393317885));
#75623=CARTESIAN_POINT('Ctrl Pts',(-0.164462651719764,-222.349290517374,
14.8703200433779));
#75624=CARTESIAN_POINT('Ctrl Pts',(0.777849756722116,-222.460657864513,
14.8174007549673));
#75625=CARTESIAN_POINT('Ctrl Pts',(1.45778010751154,-222.942372283455,14.7644814665567));
#75626=CARTESIAN_POINT('Ctrl Pts',(2.13771045830097,-223.424086702396,14.7115621781461));
#75627=CARTESIAN_POINT('Ctrl Pts',(2.55525875143796,-224.276148193141,14.6586428897355));
#75628=CARTESIAN_POINT('Ctrl Pts',(2.51935489619294,-225.108653434278,14.6057236013249));
#75629=CARTESIAN_POINT('Ctrl Pts',(2.48345104094792,-225.941158675414,14.5528043129143));
#75630=CARTESIAN_POINT('Ctrl Pts',(1.9940950373209,-226.754107666942,14.4998850245037));
#75631=CARTESIAN_POINT('Ctrl Pts',(1.27521618294983,-227.175494966323,14.4469657360931));
#75632=CARTESIAN_POINT('Ctrl Pts',(0.556337328578752,-227.596882265703,
14.3940464476825));
#75633=CARTESIAN_POINT('Ctrl Pts',(-0.392064376536375,-227.626707872936,
14.3411271592719));
#75634=CARTESIAN_POINT('Ctrl Pts',(-1.13600033078234,-227.251323590738,
14.2882078708613));
#75635=CARTESIAN_POINT('Ctrl Pts',(-1.8799362850283,-226.87593930854,14.2352885824507));
#75636=CARTESIAN_POINT('Ctrl Pts',(-2.41940648840511,-226.095345136912,
14.1823692940401));
#75637=CARTESIAN_POINT('Ctrl Pts',(-2.50754938645462,-225.266740953441,
14.1294500056295));
#75638=CARTESIAN_POINT('Ctrl Pts',(-2.5169138364799,-225.178708648644,14.1238277712504));
#75639=CARTESIAN_POINT('Ctrl Pts',(-2.52118402176622,-225.090134440647,
14.1182055368712));
#75640=CARTESIAN_POINT('Ctrl Pts',(-2.52055923806654,-225.001499367411,
14.112583302492));
#75641=CARTESIAN_POINT('Ctrl Pts',(-2.51484781591379,-225.001779432988,
14.387416697508));
#75642=CARTESIAN_POINT('Ctrl Pts',(-2.51678210576093,-225.298084098157,
14.4061027039678));
#75643=CARTESIAN_POINT('Ctrl Pts',(-2.4683915941746,-225.593777341111,14.4247887104275));
#75644=CARTESIAN_POINT('Ctrl Pts',(-2.36688521153746,-225.869947863523,
14.4434747168873));
#75645=CARTESIAN_POINT('Ctrl Pts',(-2.07941632138898,-226.652070440518,
14.4963940052979));
#75646=CARTESIAN_POINT('Ctrl Pts',(-1.36593790564043,-227.277613359643,
14.5493132937085));
#75647=CARTESIAN_POINT('Ctrl Pts',(-0.552937673309945,-227.460328193408,
14.6022325821191));
#75648=CARTESIAN_POINT('Ctrl Pts',(0.260062559020537,-227.643043027173,
14.6551518705297));
#75649=CARTESIAN_POINT('Ctrl Pts',(1.17258460793295,-227.382929775576,14.7080711589402));
#75650=CARTESIAN_POINT('Ctrl Pts',(1.76705840178706,-226.799016257435,14.7609904473508));
#75651=CARTESIAN_POINT('Ctrl Pts',(2.36153219564117,-226.215102739294,14.8139097357615));
#75652=CARTESIAN_POINT('Ctrl Pts',(2.63795773443698,-225.307388954609,14.8668290241721));
#75653=CARTESIAN_POINT('Ctrl Pts',(2.46984269705649,-224.491244713403,14.9197483125826));
#75654=CARTESIAN_POINT('Ctrl Pts',(2.30172765967599,-223.675100472197,14.9726676009932));
#75655=CARTESIAN_POINT('Ctrl Pts',(1.68907204611922,-222.95052577447,15.0255868894038));
#75656=CARTESIAN_POINT('Ctrl Pts',(0.912227053103926,-222.649085987657,
15.0785061778144));
#75657=CARTESIAN_POINT('Ctrl Pts',(0.135382060088619,-222.347646200844,
15.131425466225));
#75658=CARTESIAN_POINT('Ctrl Pts',(-0.805652312385208,-222.469341324945,
15.1843447546356));
#75659=CARTESIAN_POINT('Ctrl Pts',(-1.48025875397667,-222.958483673561,
15.2372640430462));
#75660=CARTESIAN_POINT('Ctrl Pts',(-2.11829925530295,-223.421112860135,
15.2873149278668));
#75661=CARTESIAN_POINT('Ctrl Pts',(-2.51801164078776,-224.212435079755,
15.3373658126874));
#75662=CARTESIAN_POINT('Ctrl Pts',(-2.52136959094702,-225.00082166017,15.387416697508));
#75663=CARTESIAN_POINT('Origin',(0.,-225.,10.));
#75664=CARTESIAN_POINT('',(-2.51727018845018,-224.997699004247,16.387416697508));
#75665=CARTESIAN_POINT('',(-2.51344546704351,-224.999883655119,16.112583302492));
#75666=CARTESIAN_POINT('',(-2.5175,-225.,10.));
#75667=CARTESIAN_POINT('Ctrl Pts',(-2.51344546704351,-224.999883655119,
16.112583302492));
#75668=CARTESIAN_POINT('Ctrl Pts',(-2.5136157670192,-224.586818602614,16.0865703311317));
#75669=CARTESIAN_POINT('Ctrl Pts',(-2.41747223694359,-224.173828204922,
16.0605573597714));
#75670=CARTESIAN_POINT('Ctrl Pts',(-2.22458066022694,-223.81248345365,16.034544388411));
#75671=CARTESIAN_POINT('Ctrl Pts',(-1.83217316325739,-223.077384535369,
15.9816251000004));
#75672=CARTESIAN_POINT('Ctrl Pts',(-1.03936916752074,-222.55602363786,15.9287058115898));
#75673=CARTESIAN_POINT('Ctrl Pts',(-0.208955765857058,-222.486975497596,
15.8757865231793));
#75674=CARTESIAN_POINT('Ctrl Pts',(0.621457635806621,-222.417927357332,
15.8228672347687));
#75675=CARTESIAN_POINT('Ctrl Pts',(1.48948044339735,-222.801191974312,15.7699479463581));
#75676=CARTESIAN_POINT('Ctrl Pts',(1.99790543721839,-223.461387467331,15.7170286579475));
#75677=CARTESIAN_POINT('Ctrl Pts',(2.50633043103944,-224.12158296035,15.6641093695369));
#75678=CARTESIAN_POINT('Ctrl Pts',(2.6551576110908,-225.058709329408,15.6111900811263));
#75679=CARTESIAN_POINT('Ctrl Pts',(2.37628366271229,-225.843937566455,15.5582707927157));
#75680=CARTESIAN_POINT('Ctrl Pts',(2.09740971433378,-226.629165803502,15.5053515043051));
#75681=CARTESIAN_POINT('Ctrl Pts',(1.3908346375254,-227.262495908538,15.4524322158945));
#75682=CARTESIAN_POINT('Ctrl Pts',(0.579887173539465,-227.454116037949,
15.3995129274839));
#75683=CARTESIAN_POINT('Ctrl Pts',(-0.23106029044647,-227.64573616736,15.3465936390733));
#75684=CARTESIAN_POINT('Ctrl Pts',(-1.14638014160996,-227.395646321145,
15.2936743506627));
#75685=CARTESIAN_POINT('Ctrl Pts',(-1.74722203405439,-226.818287608017,
15.2407550622521));
#75686=CARTESIAN_POINT('Ctrl Pts',(-2.2323064270685,-226.352162152333,15.1980311423321));
#75687=CARTESIAN_POINT('Ctrl Pts',(-2.51241416344975,-225.672722929182,
15.155307222412));
#75688=CARTESIAN_POINT('Ctrl Pts',(-2.51858868022655,-224.99780466334,15.112583302492));
#75689=CARTESIAN_POINT('Ctrl Pts',(-2.52136959094702,-225.00082166017,15.387416697508));
#75690=CARTESIAN_POINT('Ctrl Pts',(-2.52156203422402,-225.046003896322,
15.390285101098));
#75691=CARTESIAN_POINT('Ctrl Pts',(-2.52045268813929,-225.091176490639,
15.393153504688));
#75692=CARTESIAN_POINT('Ctrl Pts',(-2.51801180762806,-225.136277021139,
15.396021908278));
#75693=CARTESIAN_POINT('Ctrl Pts',(-2.4729799089789,-225.968338446969,15.4489411966886));
#75694=CARTESIAN_POINT('Ctrl Pts',(-1.97473760097149,-226.775871725499,
15.5018604850992));
#75695=CARTESIAN_POINT('Ctrl Pts',(-1.25128055395565,-227.189349644336,
15.5547797735098));
#75696=CARTESIAN_POINT('Ctrl Pts',(-0.527823506939808,-227.602827563173,
15.6076990619204));
#75697=CARTESIAN_POINT('Ctrl Pts',(0.420848279084464,-227.622250122317,
15.660618350331));
#75698=CARTESIAN_POINT('Ctrl Pts',(1.1606226134895,-227.238729559116,15.7135376387416));
#75699=CARTESIAN_POINT('Ctrl Pts',(1.90039694789453,-226.855208995915,15.7664569271522));
#75700=CARTESIAN_POINT('Ctrl Pts',(2.43127383068032,-226.06874531037,15.8193762155628));
#75701=CARTESIAN_POINT('Ctrl Pts',(2.51032401071362,-225.23922426946,15.8722955039734));
#75702=CARTESIAN_POINT('Ctrl Pts',(2.58937419074691,-224.409703228549,15.925214792384));
#75703=CARTESIAN_POINT('Ctrl Pts',(2.21659766802771,-223.537124832274,15.9781340807946));
#75704=CARTESIAN_POINT('Ctrl Pts',(1.56257697204023,-223.020780937739,16.0310533692052));
#75705=CARTESIAN_POINT('Ctrl Pts',(0.908556276052754,-222.504437043205,
16.0839726576158));
#75706=CARTESIAN_POINT('Ctrl Pts',(-0.0267085932030033,-222.344327650411,
16.1368919460264));
#75707=CARTESIAN_POINT('Ctrl Pts',(-0.815240449980246,-222.613718814094,
16.189811234437));
#75708=CARTESIAN_POINT('Ctrl Pts',(-1.60377230675749,-222.883109977778,
16.2427305228476));
#75709=CARTESIAN_POINT('Ctrl Pts',(-2.24557115105622,-223.582001697939,
16.2956498112582));
#75710=CARTESIAN_POINT('Ctrl Pts',(-2.44694984427243,-224.390581137697,
16.3485690996688));
#75711=CARTESIAN_POINT('Ctrl Pts',(-2.49622663743184,-224.588438225602,
16.3615182989485));
#75712=CARTESIAN_POINT('Ctrl Pts',(-2.5191325265179,-224.792863051892,16.3744674982283));
#75713=CARTESIAN_POINT('Ctrl Pts',(-2.51727018845018,-224.997699004247,
16.387416697508));
#75714=CARTESIAN_POINT('Origin',(0.,-225.,10.));
#75715=CARTESIAN_POINT('',(-2.51357021912498,-225.000594611151,17.387416697508));
#75716=CARTESIAN_POINT('',(-2.51816170421521,-225.00225638587,17.112583302492));
#75717=CARTESIAN_POINT('',(-2.5175,-225.,10.));
#75718=CARTESIAN_POINT('Ctrl Pts',(-2.51816170421521,-225.00225638587,17.112583302492));
#75719=CARTESIAN_POINT('Ctrl Pts',(-2.51206049652332,-224.34116215718,17.0707527282619));
#75720=CARTESIAN_POINT('Ctrl Pts',(-2.24478072224065,-223.675701993465,
17.0289221540319));
#75721=CARTESIAN_POINT('Ctrl Pts',(-1.77759132674405,-223.211390558611,
16.9870915798018));
#75722=CARTESIAN_POINT('Ctrl Pts',(-1.18655640031251,-222.623996500901,
16.9341722913912));
#75723=CARTESIAN_POINT('Ctrl Pts',(-0.275577426159809,-222.358529612653,
16.8812530029806));
#75724=CARTESIAN_POINT('Ctrl Pts',(0.538481636520985,-222.536467538322,
16.82833371457));
#75725=CARTESIAN_POINT('Ctrl Pts',(1.35254069920178,-222.714405463992,16.7754144261594));
#75726=CARTESIAN_POINT('Ctrl Pts',(2.06967985041067,-223.335748203578,16.7224951377488));
#75727=CARTESIAN_POINT('Ctrl Pts',(2.36173622793228,-224.11616933087,16.6695758493382));
#75728=CARTESIAN_POINT('Ctrl Pts',(2.65379260545388,-224.896590458161,16.6166565609276));
#75729=CARTESIAN_POINT('Ctrl Pts',(2.52076620928823,-225.836089973159,16.563737272517));
#75730=CARTESIAN_POINT('Ctrl Pts',(2.02352991606093,-226.504752916663,16.5108179841064));
#75731=CARTESIAN_POINT('Ctrl Pts',(1.52629362283363,-227.173415860166,16.4578986956958));
#75732=CARTESIAN_POINT('Ctrl Pts',(0.664847432544685,-227.571242232176,
16.4049794072852));
#75733=CARTESIAN_POINT('Ctrl Pts',(-0.16661089524264,-227.516186692489,
16.3520601188746));
#75734=CARTESIAN_POINT('Ctrl Pts',(-0.998069223029971,-227.461131152803,
16.299140830464));
#75735=CARTESIAN_POINT('Ctrl Pts',(-1.79953968831569,-226.953193701421,
16.2462215420534));
#75736=CARTESIAN_POINT('Ctrl Pts',(-2.20426942185732,-226.224806506203,
16.1933022536428));
#75737=CARTESIAN_POINT('Ctrl Pts',(-2.41005046800164,-225.854464851987,
16.1663959365926));
#75738=CARTESIAN_POINT('Ctrl Pts',(-2.5132693185722,-225.427134318303,16.1394896195423));
#75739=CARTESIAN_POINT('Ctrl Pts',(-2.51344546704351,-224.999883655119,
16.112583302492));
#75740=CARTESIAN_POINT('Ctrl Pts',(-2.51727018845018,-224.997699004247,
16.387416697508));
#75741=CARTESIAN_POINT('Ctrl Pts',(-2.51152173891671,-225.629962906901,
16.4273867866389));
#75742=CARTESIAN_POINT('Ctrl Pts',(-2.26979104539765,-226.26614386228,16.4673568757697));
#75743=CARTESIAN_POINT('Ctrl Pts',(-1.83921083723923,-226.725183580632,
16.5073269649006));
#75744=CARTESIAN_POINT('Ctrl Pts',(-1.26913459485615,-227.332939424455,
16.5602462533112));
#75745=CARTESIAN_POINT('Ctrl Pts',(-0.368023567956294,-227.630183952747,
16.6131655417217));
#75746=CARTESIAN_POINT('Ctrl Pts',(0.451773855565479,-227.480898077363,
16.6660848301324));
#75747=CARTESIAN_POINT('Ctrl Pts',(1.27157127908725,-227.331612201979,16.7190041185429));
#75748=CARTESIAN_POINT('Ctrl Pts',(2.01005509923094,-226.735795922919,16.7719234069536));
#75749=CARTESIAN_POINT('Ctrl Pts',(2.32929513381597,-225.966094753385,16.8248426953642));
#75750=CARTESIAN_POINT('Ctrl Pts',(2.64853516840099,-225.19639358385,16.8777619837748));
#75751=CARTESIAN_POINT('Ctrl Pts',(2.54853141742736,-224.252807523841,16.9306812721853));
#75752=CARTESIAN_POINT('Ctrl Pts',(2.07504559659883,-223.567121544764,16.9836005605959));
#75753=CARTESIAN_POINT('Ctrl Pts',(1.60155977577031,-222.881435565687,17.0365198490065));
#75754=CARTESIAN_POINT('Ctrl Pts',(0.754591885086894,-222.453649667542,
17.0894391374171));
#75755=CARTESIAN_POINT('Ctrl Pts',(-0.078285587814752,-222.479518650835,
17.1423584258277));
#75756=CARTESIAN_POINT('Ctrl Pts',(-0.911163060716401,-222.505387634127,
17.1952777142383));
#75757=CARTESIAN_POINT('Ctrl Pts',(-1.72995011583628,-222.984911498856,
17.2481970026489));
#75758=CARTESIAN_POINT('Ctrl Pts',(-2.15996980779954,-223.698660170661,
17.3011162910595));
#75759=CARTESIAN_POINT('Ctrl Pts',(-2.3937275126106,-224.086652289281,17.329883093209));
#75760=CARTESIAN_POINT('Ctrl Pts',(-2.51260507103825,-224.543857471223,
17.3586498953585));
#75761=CARTESIAN_POINT('Ctrl Pts',(-2.51357021912498,-225.000594611151,
17.387416697508));
#75762=CARTESIAN_POINT('Origin',(0.,-225.,10.));
#75763=CARTESIAN_POINT('',(-2.51944981591128,-225.001988766476,18.387416697508));
#75764=CARTESIAN_POINT('',(-2.52086477440939,-224.998703164308,18.112583302492));
#75765=CARTESIAN_POINT('',(-2.5175,-225.,10.));
#75766=CARTESIAN_POINT('Ctrl Pts',(-2.52086477440939,-224.998703164308,
18.112583302492));
#75767=CARTESIAN_POINT('Ctrl Pts',(-2.52133264793523,-224.924175560637,
18.1078544138028));
#75768=CARTESIAN_POINT('Ctrl Pts',(-2.51831399385996,-224.849686389881,
18.1031255251136));
#75769=CARTESIAN_POINT('Ctrl Pts',(-2.51168541869473,-224.775519854655,
18.0983966364243));
#75770=CARTESIAN_POINT('Ctrl Pts',(-2.43750742382676,-223.945548898266,
18.0454773480137));
#75771=CARTESIAN_POINT('Ctrl Pts',(-1.91125752455906,-223.155981722102,
17.9925580596032));
#75772=CARTESIAN_POINT('Ctrl Pts',(-1.17374787359455,-222.768124020852,
17.9396387711926));
#75773=CARTESIAN_POINT('Ctrl Pts',(-0.436238222630047,-222.380266319601,
17.886719482782));
#75774=CARTESIAN_POINT('Ctrl Pts',(0.512531180031255,-222.394118093264,
17.8338001943714));
#75775=CARTESIAN_POINT('Ctrl Pts',(1.23840357736626,-222.803340883536,17.7808809059608));
#75776=CARTESIAN_POINT('Ctrl Pts',(1.96427597470126,-223.212563673808,17.7279616175502));
#75777=CARTESIAN_POINT('Ctrl Pts',(2.46725136670996,-224.01715748069,17.6750423291396));
#75778=CARTESIAN_POINT('Ctrl Pts',(2.51716817319288,-224.848940138306,17.622123040729));
#75779=CARTESIAN_POINT('Ctrl Pts',(2.5670849796758,-225.680722795923,17.5692037523184));
#75780=CARTESIAN_POINT('Ctrl Pts',(2.16394320063292,-226.539694304275,17.5162844639078));
#75781=CARTESIAN_POINT('Ctrl Pts',(1.49222053119448,-227.032789345438,17.4633651754972));
#75782=CARTESIAN_POINT('Ctrl Pts',(0.820497861756054,-227.525884386601,
17.4104458870866));
#75783=CARTESIAN_POINT('Ctrl Pts',(-0.119805698077932,-227.653102960575,
17.357526598676));
#75784=CARTESIAN_POINT('Ctrl Pts',(-0.898407270108993,-227.356229836916,
17.3046073102654));
#75785=CARTESIAN_POINT('Ctrl Pts',(-1.67700884214006,-227.059356713256,
17.2516880218548));
#75786=CARTESIAN_POINT('Ctrl Pts',(-2.2939084263682,-226.338391891963,17.1987687334442));
#75787=CARTESIAN_POINT('Ctrl Pts',(-2.46681277912709,-225.52324886773,17.1458494450336));
#75788=CARTESIAN_POINT('Ctrl Pts',(-2.50304317839922,-225.35244369851,17.1347607308531));
#75789=CARTESIAN_POINT('Ctrl Pts',(-2.51977905108402,-225.177503441002,
17.1236720166725));
#75790=CARTESIAN_POINT('Ctrl Pts',(-2.51816170421521,-225.00225638587,17.112583302492));
#75791=CARTESIAN_POINT('Ctrl Pts',(-2.51357021912498,-225.000594611151,
17.387416697508));
#75792=CARTESIAN_POINT('Ctrl Pts',(-2.51438055340487,-225.38406919549,17.4115691837691));
#75793=CARTESIAN_POINT('Ctrl Pts',(-2.43207194083465,-225.767213847134,
17.4357216700302));
#75794=CARTESIAN_POINT('Ctrl Pts',(-2.26484973962718,-226.108787887449,
17.4598741562913));
#75795=CARTESIAN_POINT('Ctrl Pts',(-1.89845765068491,-226.85719345355,17.5127934447019));
#75796=CARTESIAN_POINT('Ctrl Pts',(-1.12442114399372,-227.40603110687,17.5657127331125));
#75797=CARTESIAN_POINT('Ctrl Pts',(-0.296939288961462,-227.504152899472,
17.6186320215231));
#75798=CARTESIAN_POINT('Ctrl Pts',(0.53054256607079,-227.602274692073,17.6715513099337));
#75799=CARTESIAN_POINT('Ctrl Pts',(1.41146976944411,-227.249680623955,17.7244705983443));
#75800=CARTESIAN_POINT('Ctrl Pts',(1.94273000790024,-226.607717426205,17.7773898867549));
#75801=CARTESIAN_POINT('Ctrl Pts',(2.47399024635636,-225.965754228455,17.8303091751655));
#75802=CARTESIAN_POINT('Ctrl Pts',(2.65558351989528,-225.034421901072,17.8832284635761));
#75803=CARTESIAN_POINT('Ctrl Pts',(2.40441283605821,-224.239898723388,17.9361477519867));
#75804=CARTESIAN_POINT('Ctrl Pts',(2.15324215222114,-223.445375545704,17.9890670403973));
#75805=CARTESIAN_POINT('Ctrl Pts',(1.46930751100809,-222.787661517718,18.0419863288079));
#75806=CARTESIAN_POINT('Ctrl Pts',(0.665577216243244,-222.567725297085,
18.0949056172185));
#75807=CARTESIAN_POINT('Ctrl Pts',(-0.138153078521605,-222.347789076451,
18.1478249056291));
#75808=CARTESIAN_POINT('Ctrl Pts',(-1.06167902683825,-222.565630663171,
18.2007441940397));
#75809=CARTESIAN_POINT('Ctrl Pts',(-1.68239481841196,-223.121568327994,
18.2536634824503));
#75810=CARTESIAN_POINT('Ctrl Pts',(-2.20534675303818,-223.589944807693,
18.2982478874695));
#75811=CARTESIAN_POINT('Ctrl Pts',(-2.51336306631068,-224.298302969004,
18.3428322924888));
#75812=CARTESIAN_POINT('Ctrl Pts',(-2.51944981591128,-225.001988766476,
18.387416697508));
#75813=CARTESIAN_POINT('Origin',(0.,-225.,10.));
#75814=CARTESIAN_POINT('',(-2.51981687702631,-224.998184138844,19.387416697508));
#75815=CARTESIAN_POINT('',(-2.51426761094033,-224.998573473955,19.112583302492));
#75816=CARTESIAN_POINT('',(-2.5175,-225.,10.));
#75817=CARTESIAN_POINT('',(1.91346599666508,-223.364012796625,20.));
#75818=CARTESIAN_POINT('Ctrl Pts',(-2.51981687702631,-224.998184138844,
19.387416697508));
#75819=CARTESIAN_POINT('Ctrl Pts',(-2.51391403651899,-225.714895358089,
19.4328532664402));
#75820=CARTESIAN_POINT('Ctrl Pts',(-2.19260490784885,-226.43611772376,19.4782898353724));
#75821=CARTESIAN_POINT('Ctrl Pts',(-1.6520347840379,-226.905008540457,19.5237264043046));
#75822=CARTESIAN_POINT('Ctrl Pts',(-1.02244089170878,-227.45111862194,19.5766456927152));
#75823=CARTESIAN_POINT('Ctrl Pts',(-0.0954214211907685,-227.65494321484,
19.6295649811258));
#75824=CARTESIAN_POINT('Ctrl Pts',(0.704614973850839,-227.421676530985,
19.6824842695364));
#75825=CARTESIAN_POINT('Ctrl Pts',(1.50465136889245,-227.18840984713,19.735403557947));
#75826=CARTESIAN_POINT('Ctrl Pts',(2.17770468845765,-226.51805188652,19.7883228463576));
#75827=CARTESIAN_POINT('Ctrl Pts',(2.41590047509774,-225.721010295893,19.8412421347682));
#75828=CARTESIAN_POINT('Ctrl Pts',(2.65409626173783,-224.923968705266,19.8941614231788));
#75829=CARTESIAN_POINT('Ctrl Pts',(2.45743451545281,-224.000243484622,19.9470807115894));
#75830=CARTESIAN_POINT('Ctrl Pts',(1.91346599666508,-223.364012796625,20.));
#75831=CARTESIAN_POINT('',(-1.9171250238334,-223.361260565514,20.));
#75832=CARTESIAN_POINT('Origin',(0.,-225.,20.));
#75833=CARTESIAN_POINT('Ctrl Pts',(-1.91712859175364,-223.361257881811,
20.));
#75834=CARTESIAN_POINT('Ctrl Pts',(-1.38658191799954,-222.742516992798,
19.948244384658));
#75835=CARTESIAN_POINT('Ctrl Pts',(-0.527608246006481,-222.40292978571,
19.896488769316));
#75836=CARTESIAN_POINT('Ctrl Pts',(0.28236917328897,-222.494297760505,19.8447331539741));
#75837=CARTESIAN_POINT('Ctrl Pts',(1.1105581219575,-222.587720052515,19.7918138655635));
#75838=CARTESIAN_POINT('Ctrl Pts',(1.88752278571044,-223.131694576731,19.7388945771529));
#75839=CARTESIAN_POINT('Ctrl Pts',(2.25823165337626,-223.877857468017,19.6859752887423));
#75840=CARTESIAN_POINT('Ctrl Pts',(2.62894052104207,-224.624020359302,19.6330560003317));
#75841=CARTESIAN_POINT('Ctrl Pts',(2.59339359262077,-225.572371617659,19.5801367119211));
#75842=CARTESIAN_POINT('Ctrl Pts',(2.16760742134957,-226.288671511728,19.5272174235105));
#75843=CARTESIAN_POINT('Ctrl Pts',(1.74182125007838,-227.004971405797,19.4742981350999));
#75844=CARTESIAN_POINT('Ctrl Pts',(0.925795835957292,-227.489219935578,
19.4213788466893));
#75845=CARTESIAN_POINT('Ctrl Pts',(0.0930673370354757,-227.519959958572,
19.3684595582787));
#75846=CARTESIAN_POINT('Ctrl Pts',(-0.739661161886337,-227.550699981566,
19.3155402698681));
#75847=CARTESIAN_POINT('Ctrl Pts',(-1.58909274560888,-227.127931497772,
19.2626209814575));
#75848=CARTESIAN_POINT('Ctrl Pts',(-2.06658807342754,-226.445046900883,
19.2097016930469));
#75849=CARTESIAN_POINT('Ctrl Pts',(-2.35869062637836,-226.027299705254,
19.1773288961953));
#75850=CARTESIAN_POINT('Ctrl Pts',(-2.51160544441321,-225.512210634445,
19.1449560993436));
#75851=CARTESIAN_POINT('Ctrl Pts',(-2.51426761094033,-224.998573473955,
19.112583302492));
#75852=CARTESIAN_POINT('Origin',(-160.,-225.,10.));
#75853=CARTESIAN_POINT('',(-162.51351594159,-224.999424933735,0.387416697508052));
#75854=CARTESIAN_POINT('',(-162.515402351214,-225.003740476838,0.112583302491938));
#75855=CARTESIAN_POINT('',(-162.5175,-225.,10.));
#75856=CARTESIAN_POINT('',(-161.913465996665,-223.364012796625,0.));
#75857=CARTESIAN_POINT('Ctrl Pts',(-162.515402351214,-225.003740476838,
0.112583302491938));
#75858=CARTESIAN_POINT('Ctrl Pts',(-162.510237314095,-224.411047851875,
0.075055534994612));
#75859=CARTESIAN_POINT('Ctrl Pts',(-162.299221828084,-223.815196439696,
0.0375277674972861));
#75860=CARTESIAN_POINT('Ctrl Pts',(-161.913465996665,-223.364012796625,
-4.02455846426619E-14));
#75861=CARTESIAN_POINT('',(-158.082847352964,-223.361245062325,1.97453514552116E-15));
#75862=CARTESIAN_POINT('Origin',(-160.,-225.,0.));
#75863=CARTESIAN_POINT('Ctrl Pts',(-158.082843652116,-223.361242283932,
1.5839321182582E-15));
#75864=CARTESIAN_POINT('Ctrl Pts',(-158.613381414978,-222.742548947437,
0.0517556153419938));
#75865=CARTESIAN_POINT('Ctrl Pts',(-159.472376042683,-222.40287561289,0.103511230683985));
#75866=CARTESIAN_POINT('Ctrl Pts',(-160.282371291112,-222.494227887034,
0.155266846025977));
#75867=CARTESIAN_POINT('Ctrl Pts',(-161.110578469784,-222.587634125381,
0.208186134436575));
#75868=CARTESIAN_POINT('Ctrl Pts',(-161.887558094787,-223.131666225295,
0.261105422847174));
#75869=CARTESIAN_POINT('Ctrl Pts',(-162.25827216591,-223.877852586243,0.314024711257772));
#75870=CARTESIAN_POINT('Ctrl Pts',(-162.429649136561,-224.222806198858,
0.338488706674532));
#75871=CARTESIAN_POINT('Ctrl Pts',(-162.514202708326,-224.61096239135,0.362952702091292));
#75872=CARTESIAN_POINT('Ctrl Pts',(-162.51351594159,-224.999424933735,0.387416697508052));
#75873=CARTESIAN_POINT('Origin',(-160.,-225.,10.));
#75874=CARTESIAN_POINT('',(-162.517460115391,-225.002301238227,1.38741669750805));
#75875=CARTESIAN_POINT('',(-162.521728577063,-224.999864685758,1.11258330249194));
#75876=CARTESIAN_POINT('',(-162.5175,-225.,10.));
#75877=CARTESIAN_POINT('Ctrl Pts',(-162.521728577063,-224.999864685758,
1.11258330249194));
#75878=CARTESIAN_POINT('Ctrl Pts',(-162.521733449713,-224.993155418077,
1.11215722053546));
#75879=CARTESIAN_POINT('Ctrl Pts',(-162.521709006639,-224.986446188795,
1.11173113857898));
#75880=CARTESIAN_POINT('Ctrl Pts',(-162.521655141041,-224.97973719783,1.11130505662251));
#75881=CARTESIAN_POINT('Ctrl Pts',(-162.514965045176,-224.146481946371,
1.05838576821191));
#75882=CARTESIAN_POINT('Ctrl Pts',(-162.054415225741,-223.316902891715,
1.00546647980131));
#75883=CARTESIAN_POINT('Ctrl Pts',(-161.350736487674,-222.870539435387,
0.952547191390716));
#75884=CARTESIAN_POINT('Ctrl Pts',(-160.647057749606,-222.424175979059,
0.899627902980117));
#75885=CARTESIAN_POINT('Ctrl Pts',(-159.700250092906,-222.361028121059,
0.846708614569519));
#75886=CARTESIAN_POINT('Ctrl Pts',(-158.943607496028,-222.71014994938,0.793789326158921));
#75887=CARTESIAN_POINT('Ctrl Pts',(-158.186964899149,-223.059271777701,
0.740870037748324));
#75888=CARTESIAN_POINT('Ctrl Pts',(-157.620487362092,-223.820663292344,
0.687950749337728));
#75889=CARTESIAN_POINT('Ctrl Pts',(-157.503322619656,-224.645584773054,
0.635031460927131));
#75890=CARTESIAN_POINT('Ctrl Pts',(-157.386157877221,-225.470506253763,
0.582112172516533));
#75891=CARTESIAN_POINT('Ctrl Pts',(-157.718305929406,-226.358957700538,
0.529192884105933));
#75892=CARTESIAN_POINT('Ctrl Pts',(-158.347923918086,-226.905064885608,
0.476273595695335));
#75893=CARTESIAN_POINT('Ctrl Pts',(-158.977541906767,-227.451172070678,
0.423354307284737));
#75894=CARTESIAN_POINT('Ctrl Pts',(-159.904629831943,-227.654934994044,
0.370435018874143));
#75895=CARTESIAN_POINT('Ctrl Pts',(-160.704626518296,-227.421707556381,
0.317515730463546));
#75896=CARTESIAN_POINT('Ctrl Pts',(-161.504623204649,-227.188480118719,
0.264596442052949));
#75897=CARTESIAN_POINT('Ctrl Pts',(-162.177528652179,-226.518262320029,
0.21167715364235));
#75898=CARTESIAN_POINT('Ctrl Pts',(-162.41573147988,-225.721203161505,0.158757865231754));
#75899=CARTESIAN_POINT('Ctrl Pts',(-162.485012528705,-225.489379320406,
0.143366344318482));
#75900=CARTESIAN_POINT('Ctrl Pts',(-162.517520723346,-225.246825571972,
0.12797482340521));
#75901=CARTESIAN_POINT('Ctrl Pts',(-162.515402351214,-225.003740476838,
0.112583302491938));
#75902=CARTESIAN_POINT('Ctrl Pts',(-162.51351594159,-224.999424933735,0.387416697508052));
#75903=CARTESIAN_POINT('Ctrl Pts',(-162.512717128954,-225.451265087905,
0.415871990501891));
#75904=CARTESIAN_POINT('Ctrl Pts',(-162.39659516119,-225.903519708241,0.44432728349573));
#75905=CARTESIAN_POINT('Ctrl Pts',(-162.167641214847,-226.288685316668,
0.472782576489569));
#75906=CARTESIAN_POINT('Ctrl Pts',(-161.74184767542,-227.004991064166,0.525701864900165));
#75907=CARTESIAN_POINT('Ctrl Pts',(-160.925812079326,-227.48926193718,0.578621153310761));
#75908=CARTESIAN_POINT('Ctrl Pts',(-160.093070279045,-227.520005786494,
0.631540441721358));
#75909=CARTESIAN_POINT('Ctrl Pts',(-159.260328478764,-227.550749635808,
0.684459730131956));
#75910=CARTESIAN_POINT('Ctrl Pts',(-158.410880474296,-227.127966461422,
0.737379018542555));
#75911=CARTESIAN_POINT('Ctrl Pts',(-157.9333767975,-226.445068740439,0.790298306953154));
#75912=CARTESIAN_POINT('Ctrl Pts',(-157.455873120704,-225.762171019456,
0.843217595363751));
#75913=CARTESIAN_POINT('Ctrl Pts',(-157.350313771578,-224.819158751875,
0.896136883774348));
#75914=CARTESIAN_POINT('Ctrl Pts',(-157.665030107393,-224.047579921191,
0.949056172184944));
#75915=CARTESIAN_POINT('Ctrl Pts',(-157.979746443209,-223.276001090507,
1.00197546059554));
#75916=CARTESIAN_POINT('Ctrl Pts',(-158.714738463965,-222.67585569672,1.05489474900614));
#75917=CARTESIAN_POINT('Ctrl Pts',(-159.533660630143,-222.521757928645,
1.10781403741674));
#75918=CARTESIAN_POINT('Ctrl Pts',(-160.352582796321,-222.36766016057,1.16073332582734));
#75919=CARTESIAN_POINT('Ctrl Pts',(-161.255435107919,-222.659610018209,
1.21365261423794));
#75920=CARTESIAN_POINT('Ctrl Pts',(-161.829078728829,-223.264017195323,
1.26657190264853));
#75921=CARTESIAN_POINT('Ctrl Pts',(-162.265730138761,-223.724085496338,
1.30685350093504));
#75922=CARTESIAN_POINT('Ctrl Pts',(-162.511635000215,-224.365194447016,
1.34713509922154));
#75923=CARTESIAN_POINT('Ctrl Pts',(-162.517460115391,-225.002301238227,
1.38741669750805));
#75924=CARTESIAN_POINT('Origin',(-160.,-225.,10.));
#75925=CARTESIAN_POINT('',(-162.521340804038,-224.999094471355,2.38741669750805));
#75926=CARTESIAN_POINT('',(-162.515825357218,-224.997885174742,2.11258330249194));
#75927=CARTESIAN_POINT('',(-162.5175,-225.,10.));
#75928=CARTESIAN_POINT('Ctrl Pts',(-162.515825357218,-224.997885174742,
2.11258330249194));
#75929=CARTESIAN_POINT('Ctrl Pts',(-162.517874459667,-224.740545642659,
2.09633961766571));
#75930=CARTESIAN_POINT('Ctrl Pts',(-162.481551331845,-224.483770756502,
2.08009593283949));
#75931=CARTESIAN_POINT('Ctrl Pts',(-162.404452695359,-224.239886170331,
2.06385224801326));
#75932=CARTESIAN_POINT('Ctrl Pts',(-162.153277852707,-223.445349777107,
2.01093295960267));
#75933=CARTESIAN_POINT('Ctrl Pts',(-161.469331891228,-222.787624664217,
1.95801367119207));
#75934=CARTESIAN_POINT('Ctrl Pts',(-160.665588259213,-222.567684878868,
1.90509438278147));
#75935=CARTESIAN_POINT('Ctrl Pts',(-159.861844627198,-222.347745093518,
1.85217509437087));
#75936=CARTESIAN_POINT('Ctrl Pts',(-158.938303324646,-222.565590635709,
1.79925580596027));
#75937=CARTESIAN_POINT('Ctrl Pts',(-158.317577269691,-223.121537364058,
1.74633651754968));
#75938=CARTESIAN_POINT('Ctrl Pts',(-157.696851214735,-223.677484092407,
1.69341722913908));
#75939=CARTESIAN_POINT('Ctrl Pts',(-157.378940407375,-224.571532006914,
1.64049794072848));
#75940=CARTESIAN_POINT('Ctrl Pts',(-157.509319921586,-225.394560702438,
1.58757865231788));
#75941=CARTESIAN_POINT('Ctrl Pts',(-157.639699435798,-226.217589397962,
1.53465936390729));
#75942=CARTESIAN_POINT('Ctrl Pts',(-158.218369271582,-226.969598874502,
1.48174007549669));
#75943=CARTESIAN_POINT('Ctrl Pts',(-158.980532001829,-227.306478111901,
1.42882078708609));
#75944=CARTESIAN_POINT('Ctrl Pts',(-159.742694732075,-227.6433573493,1.37590149867549));
#75945=CARTESIAN_POINT('Ctrl Pts',(-160.688350356784,-227.565106347558,
1.3229822102649));
#75946=CARTESIAN_POINT('Ctrl Pts',(-161.384762982991,-227.107515122556,
1.2700629218543));
#75947=CARTESIAN_POINT('Ctrl Pts',(-162.075568412594,-226.65360821324,1.21756971540018));
#75948=CARTESIAN_POINT('Ctrl Pts',(-162.521128267657,-225.826445037713,
1.16507650894606));
#75949=CARTESIAN_POINT('Ctrl Pts',(-162.521728577063,-224.999864685758,
1.11258330249194));
#75950=CARTESIAN_POINT('Ctrl Pts',(-162.517460115391,-225.002301238227,
1.38741669750805));
#75951=CARTESIAN_POINT('Ctrl Pts',(-162.519287649641,-225.202183034029,
1.40005438763214));
#75952=CARTESIAN_POINT('Ctrl Pts',(-162.497484432032,-225.401670902235,
1.41269207775623));
#75953=CARTESIAN_POINT('Ctrl Pts',(-162.450527033305,-225.595050645471,
1.42532976788032));
#75954=CARTESIAN_POINT('Ctrl Pts',(-162.253896786651,-226.404812421914,
1.47824905629092));
#75955=CARTESIAN_POINT('Ctrl Pts',(-161.616201363122,-227.107471478212,
1.53116834470152));
#75956=CARTESIAN_POINT('Ctrl Pts',(-160.829251654008,-227.38149242425,1.58408763311212));
#75957=CARTESIAN_POINT('Ctrl Pts',(-160.042301944894,-227.655513370288,
1.63700692152271));
#75958=CARTESIAN_POINT('Ctrl Pts',(-159.106097950194,-227.500896206066,
1.68992620993331));
#75959=CARTESIAN_POINT('Ctrl Pts',(-158.449045887184,-226.988393077726,
1.74284549834391));
#75960=CARTESIAN_POINT('Ctrl Pts',(-157.791993824173,-226.475889949387,
1.79576478675451));
#75961=CARTESIAN_POINT('Ctrl Pts',(-157.414093692852,-225.605500856929,
1.84868407516511));
#75962=CARTESIAN_POINT('Ctrl Pts',(-157.488272929152,-224.775516152508,
1.9016033635757));
#75963=CARTESIAN_POINT('Ctrl Pts',(-157.562452165452,-223.945531448086,
1.9545226519863));
#75964=CARTESIAN_POINT('Ctrl Pts',(-158.088710769374,-223.155951131701,
2.0074419403969));
#75965=CARTESIAN_POINT('Ctrl Pts',(-158.82623264868,-222.76808698612,2.0603612288075));
#75966=CARTESIAN_POINT('Ctrl Pts',(-159.563754527987,-222.380222840538,
2.11328051721809));
#75967=CARTESIAN_POINT('Ctrl Pts',(-160.512539682677,-222.394074865762,
2.16619980562869));
#75968=CARTESIAN_POINT('Ctrl Pts',(-161.238424124346,-222.80330444977,2.21911909403929));
#75969=CARTESIAN_POINT('Ctrl Pts',(-161.964308566014,-223.212534033777,
2.27203838244988));
#75970=CARTESIAN_POINT('Ctrl Pts',(-162.46729229466,-224.01714117657,2.32495767086048));
#75971=CARTESIAN_POINT('Ctrl Pts',(-162.517209927523,-224.848937629546,
2.37787695927108));
#75972=CARTESIAN_POINT('Ctrl Pts',(-162.520209471201,-224.898920163742,
2.38105687201674));
#75973=CARTESIAN_POINT('Ctrl Pts',(-162.521573087656,-224.949000872869,
2.3842367847624));
#75974=CARTESIAN_POINT('Ctrl Pts',(-162.521340804038,-224.999094471355,
2.38741669750805));
#75975=CARTESIAN_POINT('Origin',(-160.,-225.,10.));
#75976=CARTESIAN_POINT('',(-162.514784019862,-224.998273763422,3.38741669750805));
#75977=CARTESIAN_POINT('',(-162.514230471617,-225.001366316902,3.11258330249194));
#75978=CARTESIAN_POINT('',(-162.5175,-225.,10.));
#75979=CARTESIAN_POINT('Ctrl Pts',(-162.514230471617,-225.001366316902,
3.11258330249194));
#75980=CARTESIAN_POINT('Ctrl Pts',(-162.511723114375,-224.492626501964,
3.08052201479597));
#75981=CARTESIAN_POINT('Ctrl Pts',(-162.361947363371,-223.982529300918,
3.04846072709999));
#75982=CARTESIAN_POINT('Ctrl Pts',(-162.07507999883,-223.567097789939,3.01639943940401));
#75983=CARTESIAN_POINT('Ctrl Pts',(-161.601586328093,-222.881400442009,
2.96348015099342));
#75984=CARTESIAN_POINT('Ctrl Pts',(-160.754604395574,-222.453607448118,
2.91056086258282));
#75985=CARTESIAN_POINT('Ctrl Pts',(-159.921713114309,-222.479476861939,
2.85764157417222));
#75986=CARTESIAN_POINT('Ctrl Pts',(-159.088821833043,-222.50534627576,2.80472228576163));
#75987=CARTESIAN_POINT('Ctrl Pts',(-158.27002120303,-222.984878097294,2.75180299735103));
#75988=CARTESIAN_POINT('Ctrl Pts',(-157.839994381929,-223.698638599168,
2.69888370894043));
#75989=CARTESIAN_POINT('Ctrl Pts',(-157.409967560828,-224.412399101043,
2.64596442052983));
#75990=CARTESIAN_POINT('Ctrl Pts',(-157.368714548639,-225.360388283258,
2.59304513211923));
#75991=CARTESIAN_POINT('Ctrl Pts',(-157.735112711589,-226.108806263348,
2.54012584370864));
#75992=CARTESIAN_POINT('Ctrl Pts',(-158.101510874539,-226.857224243439,
2.48720655529804));
#75993=CARTESIAN_POINT('Ctrl Pts',(-158.875560212628,-227.406071021405,
2.43428726688744));
#75994=CARTESIAN_POINT('Ctrl Pts',(-159.703055787496,-227.504194428938,
2.38136797847685));
#75995=CARTESIAN_POINT('Ctrl Pts',(-160.530551362364,-227.602317836471,
2.32844869006625));
#75996=CARTESIAN_POINT('Ctrl Pts',(-161.411493174011,-227.249717873572,
2.27552940165565));
#75997=CARTESIAN_POINT('Ctrl Pts',(-161.942762217923,-226.607744055342,
2.22261011324505));
#75998=CARTESIAN_POINT('Ctrl Pts',(-162.310957132034,-226.162825425934,
2.18593450966068));
#75999=CARTESIAN_POINT('Ctrl Pts',(-162.511198816508,-225.578916065593,
2.14925890607631));
#76000=CARTESIAN_POINT('Ctrl Pts',(-162.515825357218,-224.997885174742,
2.11258330249194));
#76001=CARTESIAN_POINT('Ctrl Pts',(-162.521340804038,-224.999094471355,
2.38741669750805));
#76002=CARTESIAN_POINT('Ctrl Pts',(-162.517707483559,-225.782645629135,
2.43715607317299));
#76003=CARTESIAN_POINT('Ctrl Pts',(-162.123614705335,-226.569350350335,
2.48689544883793));
#76004=CARTESIAN_POINT('Ctrl Pts',(-161.492245285988,-227.032823067984,
2.53663482450287));
#76005=CARTESIAN_POINT('Ctrl Pts',(-160.820511474508,-227.525926290286,
2.58955411291347));
#76006=CARTESIAN_POINT('Ctrl Pts',(-159.880192314467,-227.65314697173,2.64247340132407));
#76007=CARTESIAN_POINT('Ctrl Pts',(-159.101577826087,-227.356268922656,
2.69539268973466));
#76008=CARTESIAN_POINT('Ctrl Pts',(-158.322963337707,-227.059390873582,
2.74831197814526));
#76009=CARTESIAN_POINT('Ctrl Pts',(-157.706053520989,-226.33841409399,2.80123126655585));
#76010=CARTESIAN_POINT('Ctrl Pts',(-157.533146300234,-225.523257548061,
2.85415055496645));
#76011=CARTESIAN_POINT('Ctrl Pts',(-157.360239079479,-224.708101002132,
2.90706984337705));
#76012=CARTESIAN_POINT('Ctrl Pts',(-157.631334454686,-223.798764689866,
2.95998913178765));
#76013=CARTESIAN_POINT('Ctrl Pts',(-158.222379185418,-223.211360887942,
3.01290842019825));
#76014=CARTESIAN_POINT('Ctrl Pts',(-158.813423916151,-222.623957086017,
3.06582770860885));
#76015=CARTESIAN_POINT('Ctrl Pts',(-159.724418002409,-222.358485794434,
3.11874699701945));
#76016=CARTESIAN_POINT('Ctrl Pts',(-160.538490569232,-222.536426671933,
3.17166628543004));
#76017=CARTESIAN_POINT('Ctrl Pts',(-161.352563136055,-222.714367549433,
3.22458557384064));
#76018=CARTESIAN_POINT('Ctrl Pts',(-162.069714183442,-223.335720596015,
3.27750486225124));
#76019=CARTESIAN_POINT('Ctrl Pts',(-162.361775405729,-224.116154669331,
3.33042415066184));
#76020=CARTESIAN_POINT('Ctrl Pts',(-162.466622575781,-224.396322996229,
3.34942166627724));
#76021=CARTESIAN_POINT('Ctrl Pts',(-162.516686679289,-224.696992746495,
3.36841918189265));
#76022=CARTESIAN_POINT('Ctrl Pts',(-162.514784019862,-224.998273763422,
3.38741669750805));
#76023=CARTESIAN_POINT('Origin',(-160.,-225.,10.));
#76024=CARTESIAN_POINT('',(-162.51509551549,-225.001872886185,4.38741669750805));
#76025=CARTESIAN_POINT('',(-162.520804175319,-225.001369558332,4.11258330249194));
#76026=CARTESIAN_POINT('',(-162.5175,-225.,10.));
#76027=CARTESIAN_POINT('Ctrl Pts',(-162.520804175319,-225.001369558332,
4.11258330249194));
#76028=CARTESIAN_POINT('Ctrl Pts',(-162.515852849758,-224.246701725063,
4.06470441192622));
#76029=CARTESIAN_POINT('Ctrl Pts',(-162.1543399445,-223.487919611795,4.01682552136049));
#76030=CARTESIAN_POINT('Ctrl Pts',(-161.562602878045,-223.020748124231,
3.96894663079477));
#76031=CARTESIAN_POINT('Ctrl Pts',(-160.908571339031,-222.504395669202,
3.91602734238417));
#76032=CARTESIAN_POINT('Ctrl Pts',(-159.973290963993,-222.34428362189,3.86310805397358));
#76033=CARTESIAN_POINT('Ctrl Pts',(-159.184746034126,-222.613679251846,
3.81018876556298));
#76034=CARTESIAN_POINT('Ctrl Pts',(-158.396201104259,-222.883074881802,
3.75726947715238));
#76035=CARTESIAN_POINT('Ctrl Pts',(-157.754391619563,-223.581978189027,
3.70435018874178));
#76036=CARTESIAN_POINT('Ctrl Pts',(-157.553009587684,-224.390571034187,
3.65143090033118));
#76037=CARTESIAN_POINT('Ctrl Pts',(-157.351627555805,-225.199163879346,
3.59851161192058));
#76038=CARTESIAN_POINT('Ctrl Pts',(-157.590672976743,-226.11744626244,3.54559232350999));
#76039=CARTESIAN_POINT('Ctrl Pts',(-158.160758670434,-226.725212182376,
3.49267303509939));
#76040=CARTESIAN_POINT('Ctrl Pts',(-158.730844364126,-227.332978102313,
3.4397537466888));
#76041=CARTESIAN_POINT('Ctrl Pts',(-159.631970330572,-227.630227559093,
3.3868344582782));
#76042=CARTESIAN_POINT('Ctrl Pts',(-160.451781345539,-227.480939208471,
3.3339151698676));
#76043=CARTESIAN_POINT('Ctrl Pts',(-161.271592360505,-227.33165085785,3.280995881457));
#76044=CARTESIAN_POINT('Ctrl Pts',(-162.010088423993,-226.735824699828,
3.2280765930464));
#76045=CARTESIAN_POINT('Ctrl Pts',(-162.329333751259,-225.966110769833,
3.17515730463581));
#76046=CARTESIAN_POINT('Ctrl Pts',(-162.455163471654,-225.662730014269,
3.15429930392119));
#76047=CARTESIAN_POINT('Ctrl Pts',(-162.51586167432,-225.33233541347,3.13344130320656));
#76048=CARTESIAN_POINT('Ctrl Pts',(-162.514230471617,-225.001366316902,
3.11258330249194));
#76049=CARTESIAN_POINT('Ctrl Pts',(-162.514784019862,-224.998273763422,
3.38741669750805));
#76050=CARTESIAN_POINT('Ctrl Pts',(-162.511386650326,-225.536238116795,
3.42133847030324));
#76051=CARTESIAN_POINT('Ctrl Pts',(-162.342302016743,-226.076151390884,
3.45526024309843));
#76052=CARTESIAN_POINT('Ctrl Pts',(-162.023563483551,-226.50477787839,3.48918201589362));
#76053=CARTESIAN_POINT('Ctrl Pts',(-161.526318941901,-227.173451914081,
3.54210130430422));
#76054=CARTESIAN_POINT('Ctrl Pts',(-160.664858461414,-227.571284885413,
3.59502059271482));
#76055=CARTESIAN_POINT('Ctrl Pts',(-159.833386340911,-227.516228432422,
3.64793988112542));
#76056=CARTESIAN_POINT('Ctrl Pts',(-159.001914220409,-227.46117197943,3.70085916953602));
#76057=CARTESIAN_POINT('Ctrl Pts',(-158.20043045989,-226.953226102116,3.75377845794661));
#76058=CARTESIAN_POINT('Ctrl Pts',(-157.795694012465,-226.224826824,3.80669774635721));
#76059=CARTESIAN_POINT('Ctrl Pts',(-157.390957565039,-225.496427545885,
3.85961703476781));
#76060=CARTESIAN_POINT('Ctrl Pts',(-157.382968430706,-224.547574866968,
3.91253632317841));
#76061=CARTESIAN_POINT('Ctrl Pts',(-157.775382437154,-223.812463754443,
3.965455611589));
#76062=CARTESIAN_POINT('Ctrl Pts',(-158.167796443601,-223.077352641917,
4.0183748999996));
#76063=CARTESIAN_POINT('Ctrl Pts',(-158.960613590829,-222.555983095782,
4.0712941884102));
#76064=CARTESIAN_POINT('Ctrl Pts',(-159.791040767866,-222.486933810109,
4.1242134768208));
#76065=CARTESIAN_POINT('Ctrl Pts',(-160.621467944904,-222.417884524436,
4.17713276523139));
#76066=CARTESIAN_POINT('Ctrl Pts',(-161.489505151751,-222.801155499226,
4.23005205364199));
#76067=CARTESIAN_POINT('Ctrl Pts',(-161.997938579617,-223.461361943945,
4.28297134205259));
#76068=CARTESIAN_POINT('Ctrl Pts',(-162.332432307038,-223.895705758609,
4.31778646053774));
#76069=CARTESIAN_POINT('Ctrl Pts',(-162.511282168108,-224.449912905609,
4.3526015790229));
#76070=CARTESIAN_POINT('Ctrl Pts',(-162.51509551549,-225.001872886185,4.38741669750805));
#76071=CARTESIAN_POINT('Origin',(-160.,-225.,10.));
#76072=CARTESIAN_POINT('',(-162.521526441259,-225.000661269066,5.38741669750805));
#76073=CARTESIAN_POINT('',(-162.518352881918,-224.997761948101,5.11258330249194));
#76074=CARTESIAN_POINT('',(-162.5175,-225.,10.));
#76075=CARTESIAN_POINT('Ctrl Pts',(-162.518352881918,-224.997761948101,
5.11258330249194));
#76076=CARTESIAN_POINT('Ctrl Pts',(-162.519921717053,-224.827461151217,
5.10180609746706));
#76077=CARTESIAN_POINT('Ctrl Pts',(-162.504121449384,-224.657449769252,
5.09102889244219));
#76078=CARTESIAN_POINT('Ctrl Pts',(-162.469883644643,-224.491236278736,
5.08025168741731));
#76079=CARTESIAN_POINT('Ctrl Pts',(-162.301765820079,-223.675078506653,
5.02733239900672));
#76080=CARTESIAN_POINT('Ctrl Pts',(-161.689100049289,-222.950491796184,
4.97441311059612));
#76081=CARTESIAN_POINT('Ctrl Pts',(-160.91224217694,-222.649047011793,4.92149382218553));
#76082=CARTESIAN_POINT('Ctrl Pts',(-160.135384304591,-222.347602227401,
4.86857453377493));
#76083=CARTESIAN_POINT('Ctrl Pts',(-159.194334330684,-222.469299369089,
4.81565524536433));
#76084=CARTESIAN_POINT('Ctrl Pts',(-158.519716704775,-222.958449827209,
4.76273595695373));
#76085=CARTESIAN_POINT('Ctrl Pts',(-157.845099078866,-223.447600285329,
4.70981666854313));
#76086=CARTESIAN_POINT('Ctrl Pts',(-157.436913800955,-224.304204059882,
4.65689738013254));
#76087=CARTESIAN_POINT('Ctrl Pts',(-157.481946446189,-225.13627928048,4.60397809172194));
#76088=CARTESIAN_POINT('Ctrl Pts',(-157.526979091423,-225.968354501077,
4.55105880331134));
#76089=CARTESIAN_POINT('Ctrl Pts',(-158.025229659802,-226.775901167718,
4.49813951490074));
#76090=CARTESIAN_POINT('Ctrl Pts',(-158.748698701031,-227.189385941618,
4.44522022649015));
#76091=CARTESIAN_POINT('Ctrl Pts',(-159.472167742261,-227.602870715519,
4.39230093807955));
#76092=CARTESIAN_POINT('Ctrl Pts',(-160.420855256339,-227.622293596678,
4.33938164966895));
#76093=CARTESIAN_POINT('Ctrl Pts',(-161.160641855482,-227.238766675076,
4.28646236125836));
#76094=CARTESIAN_POINT('Ctrl Pts',(-161.900428454625,-226.855239753474,
4.23354307284776));
#76095=CARTESIAN_POINT('Ctrl Pts',(-162.431314138832,-226.068763029111,
4.18062378443716));
#76096=CARTESIAN_POINT('Ctrl Pts',(-162.51036562944,-225.239228235557,4.12770449602656));
#76097=CARTESIAN_POINT('Ctrl Pts',(-162.517895038374,-225.160217623146,
4.12266409818169));
#76098=CARTESIAN_POINT('Ctrl Pts',(-162.521325420703,-225.08081638919,4.11762370033682));
#76099=CARTESIAN_POINT('Ctrl Pts',(-162.520804175319,-225.001369558332,
4.11258330249194));
#76100=CARTESIAN_POINT('Ctrl Pts',(-162.51509551549,-225.001872886185,4.38741669750805));
#76101=CARTESIAN_POINT('Ctrl Pts',(-162.517078489899,-225.288896964092,
4.4055208674335));
#76102=CARTESIAN_POINT('Ctrl Pts',(-162.471729978915,-225.575313387501,
4.42362503735894));
#76103=CARTESIAN_POINT('Ctrl Pts',(-162.376323081866,-225.843951566175,
4.44172920728438));
#76104=CARTESIAN_POINT('Ctrl Pts',(-162.097444507367,-226.629192829037,
4.49464849569498));
#76105=CARTESIAN_POINT('Ctrl Pts',(-161.390857709486,-227.262533440115,
4.54756778410558));
#76106=CARTESIAN_POINT('Ctrl Pts',(-160.57989679304,-227.45415674823,4.60048707251617));
#76107=CARTESIAN_POINT('Ctrl Pts',(-159.768935876593,-227.645780056345,
4.65340636092677));
#76108=CARTESIAN_POINT('Ctrl Pts',(-158.85360084158,-227.395686061497,4.70632564933737));
#76109=CARTESIAN_POINT('Ctrl Pts',(-158.252748982027,-226.818317770812,
4.75924493774797));
#76110=CARTESIAN_POINT('Ctrl Pts',(-157.651897122473,-226.240949480127,
4.81216422615857));
#76111=CARTESIAN_POINT('Ctrl Pts',(-157.365528438379,-225.336306893605,
4.86508351456916));
#76112=CARTESIAN_POINT('Ctrl Pts',(-157.524685233954,-224.518354441051,
4.91800280297976));
#76113=CARTESIAN_POINT('Ctrl Pts',(-157.68384202953,-223.700401988497,4.97092209139036));
#76114=CARTESIAN_POINT('Ctrl Pts',(-158.288524304775,-222.96913966991,5.02384137980096));
#76115=CARTESIAN_POINT('Ctrl Pts',(-159.062029462427,-222.659193107899,
5.07676066821155));
#76116=CARTESIAN_POINT('Ctrl Pts',(-159.83553462008,-222.349246545888,5.12967995662215));
#76117=CARTESIAN_POINT('Ctrl Pts',(-160.777862660139,-222.460615740452,
5.18259924503275));
#76118=CARTESIAN_POINT('Ctrl Pts',(-161.457804290002,-222.942338150349,
5.23551853344334));
#76119=CARTESIAN_POINT('Ctrl Pts',(-162.108366610783,-223.403246021245,
5.28615125479825));
#76120=CARTESIAN_POINT('Ctrl Pts',(-162.518727336833,-224.20319368033,5.33678397615315));
#76121=CARTESIAN_POINT('Ctrl Pts',(-162.521526441259,-225.000661269066,
5.38741669750805));
#76122=CARTESIAN_POINT('Origin',(-160.,-225.,10.));
#76123=CARTESIAN_POINT('',(-162.517037225954,-224.997707731385,6.38741669750805));
#76124=CARTESIAN_POINT('',(-162.51348275222,-225.000035219869,6.11258330249194));
#76125=CARTESIAN_POINT('',(-162.5175,-225.,10.));
#76126=CARTESIAN_POINT('Ctrl Pts',(-162.51348275222,-225.000035219869,6.11258330249194));
#76127=CARTESIAN_POINT('Ctrl Pts',(-162.513430051157,-224.577722205729,
6.08598849459732));
#76128=CARTESIAN_POINT('Ctrl Pts',(-162.412708967235,-224.155385572425,
6.0593936867027));
#76129=CARTESIAN_POINT('Ctrl Pts',(-162.211459914146,-223.788137470555,
6.03279887880807));
#76130=CARTESIAN_POINT('Ctrl Pts',(-161.811007437671,-223.057374221649,
5.97987959039747));
#76131=CARTESIAN_POINT('Ctrl Pts',(-161.012520031443,-222.544730963836,
5.92696030198687));
#76132=CARTESIAN_POINT('Ctrl Pts',(-160.181385516851,-222.484793241814,
5.87404101357628));
#76133=CARTESIAN_POINT('Ctrl Pts',(-159.350251002259,-222.424855519791,
5.82112172516568));
#76134=CARTESIAN_POINT('Ctrl Pts',(-158.486469379304,-222.817623333558,
5.76820243675509));
#76135=CARTESIAN_POINT('Ctrl Pts',(-157.985307101667,-223.483366139257,
5.71528314834449));
#76136=CARTESIAN_POINT('Ctrl Pts',(-157.484144824029,-224.149108944956,
5.66236385993389));
#76137=CARTESIAN_POINT('Ctrl Pts',(-157.345601891708,-225.087826742587,
5.60944457152329));
#76138=CARTESIAN_POINT('Ctrl Pts',(-157.633075547811,-225.869962286412,
5.55652528311269));
#76139=CARTESIAN_POINT('Ctrl Pts',(-157.920549203914,-226.652097830236,
5.50360599470209));
#76140=CARTESIAN_POINT('Ctrl Pts',(-158.634039448439,-227.277651120254,
5.4506867062915));
#76141=CARTESIAN_POINT('Ctrl Pts',(-159.447053159522,-227.460368983253,
5.3977674178809));
#76142=CARTESIAN_POINT('Ctrl Pts',(-160.260066870604,-227.643086846252,
5.34484812947031));
#76143=CARTESIAN_POINT('Ctrl Pts',(-161.172604048244,-227.382969282231,
5.29192884105971));
#76144=CARTESIAN_POINT('Ctrl Pts',(-161.767087697894,-226.799046083373,
5.23900955264911));
#76145=CARTESIAN_POINT('Ctrl Pts',(-162.240502596081,-226.334040961871,
5.19686746926339));
#76146=CARTESIAN_POINT('Ctrl Pts',(-162.512218269011,-225.663688815629,
5.15472538587766));
#76147=CARTESIAN_POINT('Ctrl Pts',(-162.518352881918,-224.997761948101,
5.11258330249194));
#76148=CARTESIAN_POINT('Ctrl Pts',(-162.521526441259,-225.000661269066,
5.38741669750805));
#76149=CARTESIAN_POINT('Ctrl Pts',(-162.521652848448,-225.036674800782,
5.38970326456375));
#76150=CARTESIAN_POINT('Ctrl Pts',(-162.52094806886,-225.072683274608,5.39198983161944));
#76151=CARTESIAN_POINT('Ctrl Pts',(-162.519396688694,-225.108655236683,
5.39427639867514));
#76152=CARTESIAN_POINT('Ctrl Pts',(-162.483492237855,-225.941174287893,
5.44719568708573));
#76153=CARTESIAN_POINT('Ctrl Pts',(-161.994128116511,-226.754136765084,
5.50011497549633));
#76154=CARTESIAN_POINT('Ctrl Pts',(-161.275237336966,-227.175531054678,
5.55303426390693));
#76155=CARTESIAN_POINT('Ctrl Pts',(-160.556346557421,-227.596925344272,
5.60595355231753));
#76156=CARTESIAN_POINT('Ctrl Pts',(-159.607929119675,-227.626751446269,
5.65887284072812));
#76157=CARTESIAN_POINT('Ctrl Pts',(-158.863980824594,-227.251360936982,
5.71179212913872));
#76158=CARTESIAN_POINT('Ctrl Pts',(-158.120032529513,-226.875970427695,
5.76471141754932));
#76159=CARTESIAN_POINT('Ctrl Pts',(-157.580553377096,-226.095363307124,
5.81763070595992));
#76160=CARTESIAN_POINT('Ctrl Pts',(-157.492409016881,-225.266745378293,
5.87054999437051));
#76161=CARTESIAN_POINT('Ctrl Pts',(-157.404264656667,-224.438127449462,
5.92346928278111));
#76162=CARTESIAN_POINT('Ctrl Pts',(-157.767455088655,-223.561498712372,
5.97638857119171));
#76163=CARTESIAN_POINT('Ctrl Pts',(-158.41578437831,-223.038004459879,6.02930785960231));
#76164=CARTESIAN_POINT('Ctrl Pts',(-159.064113667964,-222.514510207386,
6.0822271480129));
#76165=CARTESIAN_POINT('Ctrl Pts',(-159.997581815285,-222.34415043949,6.1351464364235));
#76166=CARTESIAN_POINT('Ctrl Pts',(-160.789033814412,-222.604881782631,
6.1880657248341));
#76167=CARTESIAN_POINT('Ctrl Pts',(-161.580485813538,-222.865613125771,
6.24098501324469));
#76168=CARTESIAN_POINT('Ctrl Pts',(-162.229921664471,-223.557435579948,
6.29390430165529));
#76169=CARTESIAN_POINT('Ctrl Pts',(-162.440159534592,-224.363771203733,
6.34682359006589));
#76170=CARTESIAN_POINT('Ctrl Pts',(-162.493915664644,-224.569944728194,
6.36035462587995));
#76171=CARTESIAN_POINT('Ctrl Pts',(-162.518957746143,-224.783604937147,
6.373885661694));
#76172=CARTESIAN_POINT('Ctrl Pts',(-162.517037225954,-224.997707731385,
6.38741669750805));
#76173=CARTESIAN_POINT('Origin',(-160.,-225.,10.));
#76174=CARTESIAN_POINT('',(-162.513684989213,-225.000739875368,7.38741669750805));
#76175=CARTESIAN_POINT('',(-162.518482140773,-225.002219575106,7.11258330249195));
#76176=CARTESIAN_POINT('',(-162.5175,-225.,10.));
#76177=CARTESIAN_POINT('Ctrl Pts',(-162.518482140773,-225.002219575106,
7.11258330249195));
#76178=CARTESIAN_POINT('Ctrl Pts',(-162.512325260313,-224.332109506928,
7.07017089172757));
#76179=CARTESIAN_POINT('Ctrl Pts',(-162.236727822943,-223.657527150712,
7.0277584809632));
#76180=CARTESIAN_POINT('Ctrl Pts',(-161.757897665573,-223.191973025776,
6.98534607019882));
#76181=CARTESIAN_POINT('Ctrl Pts',(-161.160446336095,-222.61108661625,6.93242678178823));
#76182=CARTESIAN_POINT('Ctrl Pts',(-160.246595568692,-222.355622288795,
6.87950749337763));
#76183=CARTESIAN_POINT('Ctrl Pts',(-159.434523456559,-222.542480514631,
6.82658820496703));
#76184=CARTESIAN_POINT('Ctrl Pts',(-158.622451344426,-222.729338740468,
6.77366891655644));
#76185=CARTESIAN_POINT('Ctrl Pts',(-157.912157887563,-223.358519519595,
6.72074962814584));
#76186=CARTESIAN_POINT('Ctrl Pts',(-157.628673357865,-224.142109739857,
6.66783033973524));
#76187=CARTESIAN_POINT('Ctrl Pts',(-157.345188828167,-224.925699960118,
6.61491105132465));
#76188=CARTESIAN_POINT('Ctrl Pts',(-157.488513225634,-225.863699621512,
6.56199176291405));
#76189=CARTESIAN_POINT('Ctrl Pts',(-157.993061308803,-226.526880097429,
6.50907247450345));
#76190=CARTESIAN_POINT('Ctrl Pts',(-158.497609391972,-227.190060573346,
6.45615318609285));
#76191=CARTESIAN_POINT('Ctrl Pts',(-159.363381160843,-227.578421863785,
6.40323389768225));
#76192=CARTESIAN_POINT('Ctrl Pts',(-160.194199471004,-227.514249849878,
6.35031460927165));
#76193=CARTESIAN_POINT('Ctrl Pts',(-161.025017781164,-227.45007783597,6.29739532086106));
#76194=CARTESIAN_POINT('Ctrl Pts',(-161.820882632614,-226.933372517716,
6.24447603245046));
#76195=CARTESIAN_POINT('Ctrl Pts',(-162.217606284979,-226.200578238589,
6.19155674403986));
#76196=CARTESIAN_POINT('Ctrl Pts',(-162.414954820277,-225.836052763994,
6.16523226352389));
#76197=CARTESIAN_POINT('Ctrl Pts',(-162.513534917594,-225.418055562652,
6.13890778300792));
#76198=CARTESIAN_POINT('Ctrl Pts',(-162.51348275222,-225.000035219869,6.11258330249194));
#76199=CARTESIAN_POINT('Ctrl Pts',(-162.517037225954,-224.997707731385,
6.38741669750805));
#76200=CARTESIAN_POINT('Ctrl Pts',(-162.511446675805,-225.620951587728,
6.4268049501046));
#76201=CARTESIAN_POINT('Ctrl Pts',(-162.277384044503,-226.247945763943,
6.46619320270114));
#76202=CARTESIAN_POINT('Ctrl Pts',(-161.85805134467,-226.704937194159,6.50558145529768));
#76203=CARTESIAN_POINT('Ctrl Pts',(-161.294665395319,-227.318918767409,
6.55850074370828));
#76204=CARTESIAN_POINT('Ctrl Pts',(-160.396853607305,-227.626033120516,
6.61142003211888));
#76205=CARTESIAN_POINT('Ctrl Pts',(-159.575454637173,-227.485744731537,
6.66433932052947));
#76206=CARTESIAN_POINT('Ctrl Pts',(-158.75405566704,-227.345456342557,6.71725860894007));
#76207=CARTESIAN_POINT('Ctrl Pts',(-158.009069514788,-226.757765211492,
6.77017789735067));
#76208=CARTESIAN_POINT('Ctrl Pts',(-157.68140182904,-225.991598788361,6.82309718576127));
#76209=CARTESIAN_POINT('Ctrl Pts',(-157.353734143291,-225.22543236523,6.87601647417187));
#76210=CARTESIAN_POINT('Ctrl Pts',(-157.443384924046,-224.280790650033,
6.92893576258246));
#76211=CARTESIAN_POINT('Ctrl Pts',(-157.909329975793,-223.589941673071,
6.98185505099306));
#76212=CARTESIAN_POINT('Ctrl Pts',(-158.37527502754,-222.899092696109,7.03477433940366));
#76213=CARTESIAN_POINT('Ctrl Pts',(-159.21751435028,-222.462036457382,7.08769362781425));
#76214=CARTESIAN_POINT('Ctrl Pts',(-160.050639246487,-222.478769883137,
7.14061291622485));
#76215=CARTESIAN_POINT('Ctrl Pts',(-160.883764142694,-222.495503308893,
7.19353220463545));
#76216=CARTESIAN_POINT('Ctrl Pts',(-161.707774612368,-222.966026399131,
7.24645149304605));
#76217=CARTESIAN_POINT('Ctrl Pts',(-162.145603480787,-223.675027797011,
7.29937078145664));
#76218=CARTESIAN_POINT('Ctrl Pts',(-162.388420072819,-224.068234630997,
7.32871942014045));
#76219=CARTESIAN_POINT('Ctrl Pts',(-162.512457706949,-224.534790906726,
7.35806805882425));
#76220=CARTESIAN_POINT('Ctrl Pts',(-162.513684989213,-225.000739875368,
7.38741669750805));
#76221=CARTESIAN_POINT('Origin',(-160.,-225.,10.));
#76222=CARTESIAN_POINT('',(-162.519748038511,-225.001899953564,8.38741669750805));
#76223=CARTESIAN_POINT('',(-162.520711665558,-224.998569117271,8.11258330249194));
#76224=CARTESIAN_POINT('',(-162.5175,-225.,10.));
#76225=CARTESIAN_POINT('Ctrl Pts',(-162.520711665558,-224.998569117271,
8.11258330249194));
#76226=CARTESIAN_POINT('Ctrl Pts',(-162.521280452263,-224.914853289316,
8.10727257726842));
#76227=CARTESIAN_POINT('Ctrl Pts',(-162.517471362285,-224.831189846111,
8.1019618520449));
#76228=CARTESIAN_POINT('Ctrl Pts',(-162.509114044729,-224.747983229342,
8.09665112682137));
#76229=CARTESIAN_POINT('Ctrl Pts',(-162.425836661799,-223.918862014224,
8.04373183841077));
#76230=CARTESIAN_POINT('Ctrl Pts',(-161.89095035476,-223.135100643507,7.99081255000018));
#76231=CARTESIAN_POINT('Ctrl Pts',(-161.149219087196,-222.755348305021,
7.93789326158958));
#76232=CARTESIAN_POINT('Ctrl Pts',(-160.407487819633,-222.375595966535,
7.88497397317898));
#76233=CARTESIAN_POINT('Ctrl Pts',(-159.458911591544,-222.39985266028,7.83205468476838));
#76234=CARTESIAN_POINT('Ctrl Pts',(-158.737558866254,-222.817018523676,
7.77913539635778));
#76235=CARTESIAN_POINT('Ctrl Pts',(-158.016206140963,-223.234184387072,
7.72621610794719));
#76236=CARTESIAN_POINT('Ctrl Pts',(-157.52207691847,-224.044259420117,7.67329681953659));
#76237=CARTESIAN_POINT('Ctrl Pts',(-157.481284721271,-224.876553303619,
7.620377531126));
#76238=CARTESIAN_POINT('Ctrl Pts',(-157.440492524073,-225.708847187121,
7.5674582427154));
#76239=CARTESIAN_POINT('Ctrl Pts',(-157.85303735217,-226.563359921079,7.5145389543048));
#76240=CARTESIAN_POINT('Ctrl Pts',(-158.530138700335,-227.049066495236,
7.4616196658942));
#76241=CARTESIAN_POINT('Ctrl Pts',(-159.207240048501,-227.534773069392,
7.40870037748361));
#76242=CARTESIAN_POINT('Ctrl Pts',(-160.148897916737,-227.651673483747,
7.35578108907301));
#76243=CARTESIAN_POINT('Ctrl Pts',(-160.924209683052,-227.34627411099,7.30286180066241));
#76244=CARTESIAN_POINT('Ctrl Pts',(-161.699521449367,-227.040874738233,
7.24994251225181));
#76245=CARTESIAN_POINT('Ctrl Pts',(-162.308487113762,-226.313175578364,
7.19702322384122));
#76246=CARTESIAN_POINT('Ctrl Pts',(-162.472444000183,-225.496171752631,
7.14410393543062));
#76247=CARTESIAN_POINT('Ctrl Pts',(-162.504996874505,-225.333959457431,
7.13359705778439));
#76248=CARTESIAN_POINT('Ctrl Pts',(-162.520007392191,-225.168226750104,
7.12309018013817));
#76249=CARTESIAN_POINT('Ctrl Pts',(-162.518482140773,-225.002219575106,
7.11258330249195));
#76250=CARTESIAN_POINT('Ctrl Pts',(-162.513684989213,-225.000739875368,
7.38741669750805));
#76251=CARTESIAN_POINT('Ctrl Pts',(-162.514670651298,-225.374955526348,
7.41098734723485));
#76252=CARTESIAN_POINT('Ctrl Pts',(-162.436442273887,-225.748779457519,
7.43455799696164));
#76253=CARTESIAN_POINT('Ctrl Pts',(-162.276911493845,-226.083900218957,
7.45812864668843));
#76254=CARTESIAN_POINT('Ctrl Pts',(-161.918743371317,-226.836291537502,
7.51104793509903));
#76255=CARTESIAN_POINT('Ctrl Pts',(-161.150759859096,-227.393594469072,
7.56396722350963));
#76256=CARTESIAN_POINT('Ctrl Pts',(-160.324390197273,-227.500787203137,
7.61688651192023));
#76257=CARTESIAN_POINT('Ctrl Pts',(-159.498020535451,-227.607979937202,
7.66980580033083));
#76258=CARTESIAN_POINT('Ctrl Pts',(-158.613264724027,-227.265062473763,
7.72272508874142));
#76259=CARTESIAN_POINT('Ctrl Pts',(-158.074987004913,-226.628953837347,
7.77564437715202));
#76260=CARTESIAN_POINT('Ctrl Pts',(-157.5367092858,-225.992845200931,7.82856366556262));
#76261=CARTESIAN_POINT('Ctrl Pts',(-157.344909658996,-225.063545391538,
7.88148295397322));
#76262=CARTESIAN_POINT('Ctrl Pts',(-157.587355629957,-224.266301983674,
7.93440224238382));
#76263=CARTESIAN_POINT('Ctrl Pts',(-157.829801600918,-223.46905857581,7.98732153079441));
#76264=CARTESIAN_POINT('Ctrl Pts',(-158.506493169644,-222.803871569476,
8.040240819205));
#76265=CARTESIAN_POINT('Ctrl Pts',(-159.30777628759,-222.575130525691,8.0931601076156));
#76266=CARTESIAN_POINT('Ctrl Pts',(-160.109059405536,-222.346389481906,
8.1460793960262));
#76267=CARTESIAN_POINT('Ctrl Pts',(-161.034934072702,-222.554094400669,
8.1989986844368));
#76268=CARTESIAN_POINT('Ctrl Pts',(-161.661720059599,-223.10319951524,8.2519179728474));
#76269=CARTESIAN_POINT('Ctrl Pts',(-162.196677503979,-223.571856879839,
8.29708421440095));
#76270=CARTESIAN_POINT('Ctrl Pts',(-162.513763715639,-224.289207312475,
8.3422504559545));
#76271=CARTESIAN_POINT('Ctrl Pts',(-162.519748038511,-225.001899953564,
8.38741669750805));
#76272=CARTESIAN_POINT('Origin',(-160.,-225.,10.));
#76273=CARTESIAN_POINT('',(-162.519611851718,-224.998052208505,9.38741669750806));
#76274=CARTESIAN_POINT('',(-162.514161617683,-224.998691358253,9.11258330249195));
#76275=CARTESIAN_POINT('',(-162.5175,-225.,10.));
#76276=CARTESIAN_POINT('Ctrl Pts',(-162.514161617683,-224.998691358253,
9.11258330249195));
#76277=CARTESIAN_POINT('Ctrl Pts',(-162.515741631259,-224.663409791321,
9.09145497439867));
#76278=CARTESIAN_POINT('Ctrl Pts',(-162.453405451553,-224.328691798857,
9.0703266463054));
#76279=CARTESIAN_POINT('Ctrl Pts',(-162.324380665572,-224.022032585583,
9.04919831821212));
#76280=CARTESIAN_POINT('Ctrl Pts',(-162.001217383022,-223.253955372877,
8.99627902980152));
#76281=CARTESIAN_POINT('Ctrl Pts',(-161.259694857773,-222.661899976623,
8.94335974139093));
#76282=CARTESIAN_POINT('Ctrl Pts',(-160.439133782798,-222.516790934506,
8.89044045298034));
#76283=CARTESIAN_POINT('Ctrl Pts',(-159.618572707824,-222.371681892388,
8.83752116456974));
#76284=CARTESIAN_POINT('Ctrl Pts',(-158.718973083125,-222.673519204408,
8.78460187615914));
#76285=CARTESIAN_POINT('Ctrl Pts',(-158.151991679276,-223.284182122519,
8.73168258774854));
#76286=CARTESIAN_POINT('Ctrl Pts',(-157.585010275426,-223.89484504063,8.67876329933795));
#76287=CARTESIAN_POINT('Ctrl Pts',(-157.350647092427,-224.814333564833,
8.62584401092735));
#76288=CARTESIAN_POINT('Ctrl Pts',(-157.556146718209,-225.62188976453,8.57292472251675));
#76289=CARTESIAN_POINT('Ctrl Pts',(-157.761646343991,-226.429445964228,
8.52000543410615));
#76290=CARTESIAN_POINT('Ctrl Pts',(-158.407008778556,-227.125069839421,
8.46708614569556));
#76291=CARTESIAN_POINT('Ctrl Pts',(-159.196916184535,-227.390443918499,
8.41416685728496));
#76292=CARTESIAN_POINT('Ctrl Pts',(-159.986823590514,-227.655817997576,
8.36124756887436));
#76293=CARTESIAN_POINT('Ctrl Pts',(-160.921275967908,-227.490942280538,
8.30832828046376));
#76294=CARTESIAN_POINT('Ctrl Pts',(-161.572667927194,-226.971263892259,
8.25540899205316));
#76295=CARTESIAN_POINT('Ctrl Pts',(-162.158689322883,-226.503737927182,
8.20780042886609));
#76296=CARTESIAN_POINT('Ctrl Pts',(-162.515612716419,-225.749048593652,
8.16019186567902));
#76297=CARTESIAN_POINT('Ctrl Pts',(-162.520711665558,-224.998569117271,
8.11258330249194));
#76298=CARTESIAN_POINT('Ctrl Pts',(-162.519748038511,-225.001899953564,
8.38741669750805));
#76299=CARTESIAN_POINT('Ctrl Pts',(-162.520775282179,-225.12423777161,8.3951697443651));
#76300=CARTESIAN_POINT('Ctrl Pts',(-162.51263568778,-225.246438344522,8.40292279122215));
#76301=CARTESIAN_POINT('Ctrl Pts',(-162.494857698409,-225.367220233851,
8.41067583807919));
#76302=CARTESIAN_POINT('Ctrl Pts',(-162.373512043696,-226.191630527516,
8.46359512648979));
#76303=CARTESIAN_POINT('Ctrl Pts',(-161.803123427644,-226.949945804467,
8.51651441490039));
#76304=CARTESIAN_POINT('Ctrl Pts',(-161.044701669743,-227.295161008883,
8.56943370331098));
#76305=CARTESIAN_POINT('Ctrl Pts',(-160.286279911842,-227.640376213298,
8.62235299172158));
#76306=CARTESIAN_POINT('Ctrl Pts',(-159.339825012092,-227.572491345178,
8.67527228013218));
#76307=CARTESIAN_POINT('Ctrl Pts',(-158.63843471401,-227.12257051884,8.72819156854278));
#76308=CARTESIAN_POINT('Ctrl Pts',(-157.937044415928,-226.672649692501,
8.78111085695338));
#76309=CARTESIAN_POINT('Ctrl Pts',(-157.480718719513,-225.840692907943,
8.83403014536398));
#76310=CARTESIAN_POINT('Ctrl Pts',(-157.478272254473,-225.007403573423,
8.88694943377457));
#76311=CARTESIAN_POINT('Ctrl Pts',(-157.475825789433,-224.174114238902,
8.93986872218517));
#76312=CARTESIAN_POINT('Ctrl Pts',(-157.927258555767,-223.339492354418,
8.99278801059577));
#76313=CARTESIAN_POINT('Ctrl Pts',(-158.625994928478,-222.8854608779,9.04570729900636));
#76314=CARTESIAN_POINT('Ctrl Pts',(-159.324731301188,-222.431429401383,
9.09862658741696));
#76315=CARTESIAN_POINT('Ctrl Pts',(-160.270771280274,-222.357988332831,
9.15154587582756));
#76316=CARTESIAN_POINT('Ctrl Pts',(-161.031206989908,-222.698744303771,
9.20446516423815));
#76317=CARTESIAN_POINT('Ctrl Pts',(-161.791642699542,-223.039500274711,
9.25738445264875));
#76318=CARTESIAN_POINT('Ctrl Pts',(-162.366474139722,-223.794453285143,
9.31030374105935));
#76319=CARTESIAN_POINT('Ctrl Pts',(-162.492658454726,-224.618136852336,
9.36322302946995));
#76320=CARTESIAN_POINT('Ctrl Pts',(-162.51188812517,-224.743660880793,9.37128758548265));
#76321=CARTESIAN_POINT('Ctrl Pts',(-162.520698512878,-224.870781092672,
9.37935214149535));
#76322=CARTESIAN_POINT('Ctrl Pts',(-162.519611851718,-224.998052208505,
9.38741669750806));
#76323=CARTESIAN_POINT('Origin',(-160.,-225.,10.));
#76324=CARTESIAN_POINT('',(-162.513643850542,-224.999337553514,10.3874166975081));
#76325=CARTESIAN_POINT('',(-162.515939379227,-225.002142062255,10.1125833024919));
#76326=CARTESIAN_POINT('',(-162.5175,-225.,10.));
#76327=CARTESIAN_POINT('Ctrl Pts',(-162.515939379227,-225.002142062255,
10.1125833024919));
#76328=CARTESIAN_POINT('Ctrl Pts',(-162.511202965047,-224.416895606318,
10.0756373715289));
#76329=CARTESIAN_POINT('Ctrl Pts',(-162.307732471351,-223.828679655638,
10.0386914405659));
#76330=CARTESIAN_POINT('Ctrl Pts',(-161.934544677219,-223.382377474813,
10.0017455096029));
#76331=CARTESIAN_POINT('Ctrl Pts',(-161.400011320115,-222.743119152998,
9.94882622119228));
#76332=CARTESIAN_POINT('Ctrl Pts',(-160.517284287975,-222.395012510696,
9.89590693278169));
#76333=CARTESIAN_POINT('Ctrl Pts',(-159.690299453349,-222.497351140581,
9.84298764437109));
#76334=CARTESIAN_POINT('Ctrl Pts',(-158.863314618724,-222.599689770465,
9.79006835596049));
#76335=CARTESIAN_POINT('Ctrl Pts',(-158.092071981614,-223.152473672536,
9.73714906754989));
#76336=CARTESIAN_POINT('Ctrl Pts',(-157.729492157596,-223.902748944075,
9.68422977913929));
#76337=CARTESIAN_POINT('Ctrl Pts',(-157.366912333578,-224.653024215613,
9.6313104907287));
#76338=CARTESIAN_POINT('Ctrl Pts',(-157.412995322652,-225.600790856619,
9.5783912023181));
#76339=CARTESIAN_POINT('Ctrl Pts',(-157.846653549925,-226.312350870803,
9.52547191390751));
#76340=CARTESIAN_POINT('Ctrl Pts',(-158.280311777197,-227.023910884987,
9.47255262549691));
#76341=CARTESIAN_POINT('Ctrl Pts',(-159.101545242668,-227.49926427235,9.41963333708631));
#76342=CARTESIAN_POINT('Ctrl Pts',(-159.934557528684,-227.52088933218,9.36671404867571));
#76343=CARTESIAN_POINT('Ctrl Pts',(-160.767569814701,-227.54251439201,9.31379476026511));
#76344=CARTESIAN_POINT('Ctrl Pts',(-161.612360921263,-227.110411124307,
9.26087547185452));
#76345=CARTESIAN_POINT('Ctrl Pts',(-162.082354454619,-226.422309975877,
9.20795618344392));
#76346=CARTESIAN_POINT('Ctrl Pts',(-162.364700385886,-226.008937140356,
9.1761652231266));
#76347=CARTESIAN_POINT('Ctrl Pts',(-162.511784233693,-225.503176282115,
9.14437426280927));
#76348=CARTESIAN_POINT('Ctrl Pts',(-162.514161617683,-224.998691358253,
9.11258330249195));
#76349=CARTESIAN_POINT('Ctrl Pts',(-162.519611851718,-224.998052208505,
9.38741669750806));
#76350=CARTESIAN_POINT('Ctrl Pts',(-162.513567886561,-225.705928976136,
9.43227142990595));
#76351=CARTESIAN_POINT('Ctrl Pts',(-162.201354841253,-226.418474016637,
9.47712616230385));
#76352=CARTESIAN_POINT('Ctrl Pts',(-161.6728289998,-226.887010538627,9.52198089470174));
#76353=CARTESIAN_POINT('Ctrl Pts',(-161.049278040044,-227.439786533768,
9.57490018311234));
#76354=CARTESIAN_POINT('Ctrl Pts',(-160.124638930707,-227.652924400097,
9.62781947152293));
#76355=CARTESIAN_POINT('Ctrl Pts',(-159.32202651004,-227.428892254171,9.68073875993353));
#76356=CARTESIAN_POINT('Ctrl Pts',(-158.519414089373,-227.204860108245,
9.73365804834413));
#76357=CARTESIAN_POINT('Ctrl Pts',(-157.838828357376,-226.543657950064,
9.78657733675473));
#76358=CARTESIAN_POINT('Ctrl Pts',(-157.59170533163,-225.747851874212,9.83949662516533));
#76359=CARTESIAN_POINT('Ctrl Pts',(-157.344582305884,-224.952045798359,
9.89241591357592));
#76360=CARTESIAN_POINT('Ctrl Pts',(-157.530921986389,-224.021635804835,
9.94533520198652));
#76361=CARTESIAN_POINT('Ctrl Pts',(-158.065455339009,-223.382377488383,
9.99825449039712));
#76362=CARTESIAN_POINT('Ctrl Pts',(-158.599988691629,-222.74311917193,10.0511737788077));
#76363=CARTESIAN_POINT('Ctrl Pts',(-159.482715716365,-222.395012532548,
10.1040930672183));
#76364=CARTESIAN_POINT('Ctrl Pts',(-160.309700544053,-222.497351161574,
10.1570123556289));
#76365=CARTESIAN_POINT('Ctrl Pts',(-161.136685371741,-222.5996897906,10.2099316440395));
#76366=CARTESIAN_POINT('Ctrl Pts',(-161.907928002381,-223.152473688034,
10.2628509324501));
#76367=CARTESIAN_POINT('Ctrl Pts',(-162.270507823358,-223.902748953279,
10.3157702208607));
#76368=CARTESIAN_POINT('Ctrl Pts',(-162.434137931627,-224.241343700644,
10.3396523797432));
#76369=CARTESIAN_POINT('Ctrl Pts',(-162.514537197227,-224.620160784307,
10.3635345386256));
#76370=CARTESIAN_POINT('Ctrl Pts',(-162.513643850542,-224.999337553514,
10.3874166975081));
#76371=CARTESIAN_POINT('Origin',(-160.,-225.,10.));
#76372=CARTESIAN_POINT('',(-162.517183864174,-225.002298291999,11.3874166975081));
#76373=CARTESIAN_POINT('',(-162.521737982592,-225.000045821966,11.112583302492));
#76374=CARTESIAN_POINT('',(-162.5175,-225.,10.));
#76375=CARTESIAN_POINT('Ctrl Pts',(-162.521737578137,-225.000045817593,
11.112583302492));
#76376=CARTESIAN_POINT('Ctrl Pts',(-162.521514732431,-224.169204530868,
11.0598197686592));
#76377=CARTESIAN_POINT('Ctrl Pts',(-162.070684907329,-223.338156013345,
11.0070562348264));
#76378=CARTESIAN_POINT('Ctrl Pts',(-161.374005083048,-222.885460860162,
10.9542927009936));
#76379=CARTESIAN_POINT('Ctrl Pts',(-160.675268704477,-222.431429379836,
10.901373412583));
#76380=CARTESIAN_POINT('Ctrl Pts',(-159.729228717454,-222.357988310668,
10.8484541241724));
#76381=CARTESIAN_POINT('Ctrl Pts',(-158.968793001442,-222.698744284467,
10.7955348357618));
#76382=CARTESIAN_POINT('Ctrl Pts',(-158.208357285429,-223.039500258266,
10.7426155473512));
#76383=CARTESIAN_POINT('Ctrl Pts',(-157.633525840426,-223.79445327503,10.6896962589407));
#76384=CARTESIAN_POINT('Ctrl Pts',(-157.507341524364,-224.618136849133,
10.6367769705301));
#76385=CARTESIAN_POINT('Ctrl Pts',(-157.381157208302,-225.441820423236,
10.5838576821195));
#76386=CARTESIAN_POINT('Ctrl Pts',(-157.703620021181,-226.334234554677,
10.5309383937089));
#76387=CARTESIAN_POINT('Ctrl Pts',(-158.327170986167,-226.887010554456,
10.4780191052983));
#76388=CARTESIAN_POINT('Ctrl Pts',(-158.950721951154,-227.439786554235,
10.4250998168877));
#76389=CARTESIAN_POINT('Ctrl Pts',(-159.875361068248,-227.652924422351,
10.3721805284771));
#76390=CARTESIAN_POINT('Ctrl Pts',(-160.677973495648,-227.428892274546,
10.3192612400665));
#76391=CARTESIAN_POINT('Ctrl Pts',(-161.480585923048,-227.20486012674,10.2663419516559));
#76392=CARTESIAN_POINT('Ctrl Pts',(-162.161171660753,-226.543657963013,
10.2134226632453));
#76393=CARTESIAN_POINT('Ctrl Pts',(-162.408294688572,-225.747851880485,
10.1605033748347));
#76394=CARTESIAN_POINT('Ctrl Pts',(-162.482887234606,-225.507642773429,
10.1445300173871));
#76395=CARTESIAN_POINT('Ctrl Pts',(-162.517987140231,-225.255169949006,
10.1285566599395));
#76396=CARTESIAN_POINT('Ctrl Pts',(-162.515939379227,-225.002142062255,
10.1125833024919));
#76397=CARTESIAN_POINT('Ctrl Pts',(-162.513643850542,-224.999337553514,
10.3874166975081));
#76398=CARTESIAN_POINT('Ctrl Pts',(-162.512557674726,-225.460359733951,
10.4164538270362));
#76399=CARTESIAN_POINT('Ctrl Pts',(-162.391297288662,-225.921913634613,
10.4454909565643));
#76400=CARTESIAN_POINT('Ctrl Pts',(-162.153346432012,-226.312350859794,
10.4745280860925));
#76401=CARTESIAN_POINT('Ctrl Pts',(-161.719688208377,-227.023910868009,
10.5274473745031));
#76402=CARTESIAN_POINT('Ctrl Pts',(-160.898454749795,-227.499264251384,
10.5803666629137));
#76403=CARTESIAN_POINT('Ctrl Pts',(-160.065442470767,-227.520889311033,
10.6332859513243));
#76404=CARTESIAN_POINT('Ctrl Pts',(-159.232430191738,-227.542514370681,
10.6862052397349));
#76405=CARTESIAN_POINT('Ctrl Pts',(-158.387639092262,-227.110411106604,
10.7391245281455));
#76406=CARTESIAN_POINT('Ctrl Pts',(-157.917645562849,-226.422309963946,
10.7920438165561));
#76407=CARTESIAN_POINT('Ctrl Pts',(-157.447652033437,-225.734208821288,
10.8449631049667));
#76408=CARTESIAN_POINT('Ctrl Pts',(-157.352456074086,-224.790109800049,
10.8978823933773));
#76409=CARTESIAN_POINT('Ctrl Pts',(-157.675619353926,-224.022032593786,
10.9508016817879));
#76410=CARTESIAN_POINT('Ctrl Pts',(-157.998782633765,-223.253955387523,
11.0037209701985));
#76411=CARTESIAN_POINT('Ctrl Pts',(-158.740305152795,-222.661899996236,
11.0566402586091));
#76412=CARTESIAN_POINT('Ctrl Pts',(-159.560866220885,-222.516790955336,
11.1095595470197));
#76413=CARTESIAN_POINT('Ctrl Pts',(-160.381427288976,-222.371681914436,
11.1624788354303));
#76414=CARTESIAN_POINT('Ctrl Pts',(-161.281026906129,-222.673519223924,
11.2153981238409));
#76415=CARTESIAN_POINT('Ctrl Pts',(-161.848008305222,-223.284182136912,
11.2683174122515));
#76416=CARTESIAN_POINT('Ctrl Pts',(-162.273354660738,-223.742298126085,
11.3080171740037));
#76417=CARTESIAN_POINT('Ctrl Pts',(-162.511506189725,-224.374218651919,
11.3477169357559));
#76418=CARTESIAN_POINT('Ctrl Pts',(-162.517183864174,-225.002298291999,
11.3874166975081));
#76419=CARTESIAN_POINT('Origin',(-160.,-225.,10.));
#76420=CARTESIAN_POINT('',(-162.521467614345,-224.999252277067,12.3874166975081));
#76421=CARTESIAN_POINT('',(-162.516072905486,-224.997828941168,12.1125833024919));
#76422=CARTESIAN_POINT('',(-162.5175,-225.,10.));
#76423=CARTESIAN_POINT('Ctrl Pts',(-162.516072905486,-224.997828941168,
12.1125833024919));
#76424=CARTESIAN_POINT('Ctrl Pts',(-162.518115808906,-224.749768865176,
12.0969214542));
#76425=CARTESIAN_POINT('Ctrl Pts',(-162.484398039321,-224.50225196448,12.0812596059081));
#76426=CARTESIAN_POINT('Ctrl Pts',(-162.412644390281,-224.266301977519,
12.0655977576162));
#76427=CARTESIAN_POINT('Ctrl Pts',(-162.170198417287,-223.469058562968,
12.0126784692056));
#76428=CARTESIAN_POINT('Ctrl Pts',(-161.493506842885,-222.803871551054,
11.959759180795));
#76429=CARTESIAN_POINT('Ctrl Pts',(-160.692223718217,-222.57513050535,11.9068398923844));
#76430=CARTESIAN_POINT('Ctrl Pts',(-159.89094059355,-222.346389459646,11.8539206039738));
#76431=CARTESIAN_POINT('Ctrl Pts',(-158.965065918616,-222.554094380152,
11.8010013155632));
#76432=CARTESIAN_POINT('Ctrl Pts',(-158.338279926462,-223.103199499328,
11.7480820271526));
#76433=CARTESIAN_POINT('Ctrl Pts',(-157.711493934307,-223.652304618505,
11.695162738742));
#76434=CARTESIAN_POINT('Ctrl Pts',(-157.383796624932,-224.542809936352,
11.6422434503314));
#76435=CARTESIAN_POINT('Ctrl Pts',(-157.505142280663,-225.367220236932,
11.5893241619208));
#76436=CARTESIAN_POINT('Ctrl Pts',(-157.626487936394,-226.191630537512,
11.5364048735102));
#76437=CARTESIAN_POINT('Ctrl Pts',(-158.19687655723,-226.949945820824,11.4834855850996));
#76438=CARTESIAN_POINT('Ctrl Pts',(-158.955298321493,-227.295161028136,
11.430566296689));
#76439=CARTESIAN_POINT('Ctrl Pts',(-159.713720085756,-227.640376235448,
11.3776470082784));
#76440=CARTESIAN_POINT('Ctrl Pts',(-160.660174993445,-227.572491366758,
11.3247277198678));
#76441=CARTESIAN_POINT('Ctrl Pts',(-161.361565297411,-227.122570536645,
11.2718084314572));
#76442=CARTESIAN_POINT('Ctrl Pts',(-162.062955601377,-226.672649706532,
11.2188891430466));
#76443=CARTESIAN_POINT('Ctrl Pts',(-162.51928130162,-225.840692914996,11.165969854636));
#76444=CARTESIAN_POINT('Ctrl Pts',(-162.521727766681,-225.007403573485,
11.1130505662254));
#76445=CARTESIAN_POINT('Ctrl Pts',(-162.521734967233,-225.004950996485,
11.1128948116476));
#76446=CARTESIAN_POINT('Ctrl Pts',(-162.521738235963,-225.002498407942,
11.1127390570698));
#76447=CARTESIAN_POINT('Ctrl Pts',(-162.521737578137,-225.000045817593,
11.112583302492));
#76448=CARTESIAN_POINT('Ctrl Pts',(-162.517183864174,-225.002298291999,
11.3874166975081));
#76449=CARTESIAN_POINT('Ctrl Pts',(-162.519074459115,-225.211440996619,
11.4006362241665));
#76450=CARTESIAN_POINT('Ctrl Pts',(-162.495188187366,-225.42015782109,11.4138557508248));
#76451=CARTESIAN_POINT('Ctrl Pts',(-162.443853261291,-225.621889759314,
11.4270752774832));
#76452=CARTESIAN_POINT('Ctrl Pts',(-162.238353637232,-226.429445952237,
11.4799945658938));
#76453=CARTESIAN_POINT('Ctrl Pts',(-161.592991208081,-227.125069821595,
11.5329138543044));
#76454=CARTESIAN_POINT('Ctrl Pts',(-160.803083808728,-227.390443898446,
11.585833142715));
#76455=CARTESIAN_POINT('Ctrl Pts',(-160.013176409375,-227.655817975297,
11.6387524311256));
#76456=CARTESIAN_POINT('Ctrl Pts',(-159.07872403982,-227.490942259642,11.6916717195362));
#76457=CARTESIAN_POINT('Ctrl Pts',(-158.427332085998,-226.971263875723,
11.7445910079468));
#76458=CARTESIAN_POINT('Ctrl Pts',(-157.775940132176,-226.451585491803,
11.7975102963574));
#76459=CARTESIAN_POINT('Ctrl Pts',(-157.407608594088,-225.577104439619,
11.850429584768));
#76460=CARTESIAN_POINT('Ctrl Pts',(-157.490885976319,-224.747983231456,
11.9033488731786));
#76461=CARTESIAN_POINT('Ctrl Pts',(-157.574163358551,-223.918862023293,
11.9562681615892));
#76462=CARTESIAN_POINT('Ctrl Pts',(-158.109049661103,-223.135100659151,
12.0091874499998));
#76463=CARTESIAN_POINT('Ctrl Pts',(-158.850780922444,-222.75534832385,12.0621067384104));
#76464=CARTESIAN_POINT('Ctrl Pts',(-159.592512183786,-222.37559598855,12.115026026821));
#76465=CARTESIAN_POINT('Ctrl Pts',(-160.541088403917,-222.399852682092,
12.1679453152316));
#76466=CARTESIAN_POINT('Ctrl Pts',(-161.262441123156,-222.817018541988,
12.2208646036422));
#76467=CARTESIAN_POINT('Ctrl Pts',(-161.983793842396,-223.234184401884,
12.2737838920528));
#76468=CARTESIAN_POINT('Ctrl Pts',(-162.477923060744,-224.044259428135,
12.3267031804634));
#76469=CARTESIAN_POINT('Ctrl Pts',(-162.5187152576,-224.876553304655,12.379622468874));
#76470=CARTESIAN_POINT('Ctrl Pts',(-162.520717953393,-224.917414831451,
12.3822205450854));
#76471=CARTESIAN_POINT('Ctrl Pts',(-162.521627959187,-224.95832991292,12.3848186212967));
#76472=CARTESIAN_POINT('Ctrl Pts',(-162.521467614345,-224.999252277067,
12.3874166975081));
#76473=CARTESIAN_POINT('Origin',(-160.,-225.,10.));
#76474=CARTESIAN_POINT('',(-162.514983776563,-224.998176142249,13.3874166975081));
#76475=CARTESIAN_POINT('',(-162.514086114787,-225.001240687878,13.112583302492));
#76476=CARTESIAN_POINT('',(-162.5175,-225.,10.));
#76477=CARTESIAN_POINT('Ctrl Pts',(-162.514086114787,-225.001240687878,
13.112583302492));
#76478=CARTESIAN_POINT('Ctrl Pts',(-162.511858228025,-224.501661496837,
13.0811038513303));
#76479=CARTESIAN_POINT('Ctrl Pts',(-162.367841089657,-224.000898563083,
13.0496244001686));
#76480=CARTESIAN_POINT('Ctrl Pts',(-162.090670041745,-223.589941661243,
13.0181449490069));
#76481=CARTESIAN_POINT('Ctrl Pts',(-161.624724986089,-222.899092678486,
12.9652256605963));
#76482=CARTESIAN_POINT('Ctrl Pts',(-160.782485656284,-222.462036436092,
12.9123063721857));
#76483=CARTESIAN_POINT('Ctrl Pts',(-159.949360753088,-222.478769861988,
12.8593870837751));
#76484=CARTESIAN_POINT('Ctrl Pts',(-159.116235849893,-222.495503287884,
12.8064677953645));
#76485=CARTESIAN_POINT('Ctrl Pts',(-158.292225373307,-222.966026382069,
12.7535485069539));
#76486=CARTESIAN_POINT('Ctrl Pts',(-157.854396501214,-223.675027785897,
12.7006292185434));
#76487=CARTESIAN_POINT('Ctrl Pts',(-157.416567629121,-224.384029189724,
12.6477099301328));
#76488=CARTESIAN_POINT('Ctrl Pts',(-157.364920361522,-225.331508903193,
12.5947906417222));
#76489=CARTESIAN_POINT('Ctrl Pts',(-157.723088487055,-226.083900228049,
12.5418713533116));
#76490=CARTESIAN_POINT('Ctrl Pts',(-158.081256612587,-226.836291552906,
12.488952064901));
#76491=CARTESIAN_POINT('Ctrl Pts',(-158.849240131251,-227.393594489151,
12.4360327764904));
#76492=CARTESIAN_POINT('Ctrl Pts',(-159.675609800005,-227.500787224115,
12.3831134880798));
#76493=CARTESIAN_POINT('Ctrl Pts',(-160.50197946876,-227.607979959079,12.3301941996692));
#76494=CARTESIAN_POINT('Ctrl Pts',(-161.386735287606,-227.265062492763,
12.2772749112586));
#76495=CARTESIAN_POINT('Ctrl Pts',(-161.925013011235,-226.628953851011,
12.224355622848));
#76496=CARTESIAN_POINT('Ctrl Pts',(-162.303983527613,-226.181106188262,
12.1870981827293));
#76497=CARTESIAN_POINT('Ctrl Pts',(-162.511213111775,-225.587930649141,
12.1498407426106));
#76498=CARTESIAN_POINT('Ctrl Pts',(-162.516072905486,-224.997828941168,
12.1125833024919));
#76499=CARTESIAN_POINT('Ctrl Pts',(-162.521467614345,-224.999252277067,
12.3874166975081));
#76500=CARTESIAN_POINT('Ctrl Pts',(-162.518361952259,-225.791862963762,
12.4377379097073));
#76501=CARTESIAN_POINT('Ctrl Pts',(-162.11372029147,-226.587205706412,12.4880591219065));
#76502=CARTESIAN_POINT('Ctrl Pts',(-161.469861287334,-227.049066478047,
12.5383803341058));
#76503=CARTESIAN_POINT('Ctrl Pts',(-160.792759944848,-227.534773048129,
12.5912996225164));
#76504=CARTESIAN_POINT('Ctrl Pts',(-159.851102084512,-227.651673461503,
12.644218910927));
#76505=CARTESIAN_POINT('Ctrl Pts',(-159.075790324701,-227.346274091308,
12.6971381993376));
#76506=CARTESIAN_POINT('Ctrl Pts',(-158.30047856489,-227.040874721113,12.7500574877482));
#76507=CARTESIAN_POINT('Ctrl Pts',(-157.691512905603,-226.313175567348,
12.8029767761588));
#76508=CARTESIAN_POINT('Ctrl Pts',(-157.527556020558,-225.496171748469,
12.8558960645694));
#76509=CARTESIAN_POINT('Ctrl Pts',(-157.363599135512,-224.67916792959,12.90881535298));
#76510=CARTESIAN_POINT('Ctrl Pts',(-157.644651024707,-223.772859445596,
12.9617346413906));
#76511=CARTESIAN_POINT('Ctrl Pts',(-158.242102349173,-223.191973040943,
13.0146539298012));
#76512=CARTESIAN_POINT('Ctrl Pts',(-158.83955367364,-222.61108663629,13.0675732182118));
#76513=CARTESIAN_POINT('Ctrl Pts',(-159.753404433377,-222.355622310978,
13.1204925066224));
#76514=CARTESIAN_POINT('Ctrl Pts',(-160.565476538698,-222.542480535247,
13.173411795033));
#76515=CARTESIAN_POINT('Ctrl Pts',(-161.377548644019,-222.729338759516,
13.2263310834436));
#76516=CARTESIAN_POINT('Ctrl Pts',(-162.087842094923,-223.358519533365,
13.2792503718542));
#76517=CARTESIAN_POINT('Ctrl Pts',(-162.371326622243,-224.142109747053,
13.3321696602648));
#76518=CARTESIAN_POINT('Ctrl Pts',(-162.469977988056,-224.414795687091,
13.3505853393459));
#76519=CARTESIAN_POINT('Ctrl Pts',(-162.516942395514,-224.706180754175,
13.369001018427));
#76520=CARTESIAN_POINT('Ctrl Pts',(-162.514983776563,-224.998176142249,
13.3874166975081));
#76521=CARTESIAN_POINT('Origin',(-160.,-225.,10.));
#76522=CARTESIAN_POINT('',(-162.514889488545,-225.001779462475,14.3874166975081));
#76523=CARTESIAN_POINT('',(-162.52060107169,-225.001499392296,14.112583302492));
#76524=CARTESIAN_POINT('',(-162.5175,-225.,10.));
#76525=CARTESIAN_POINT('Ctrl Pts',(-162.52060107169,-225.001499392296,14.112583302492));
#76526=CARTESIAN_POINT('Ctrl Pts',(-162.51534499077,-224.25584434795,14.0652862484605));
#76527=CARTESIAN_POINT('Ctrl Pts',(-162.163665333211,-223.505881788273,
14.0179891944291));
#76528=CARTESIAN_POINT('Ctrl Pts',(-161.584215634979,-223.038004443421,
13.9706921403977));
#76529=CARTESIAN_POINT('Ctrl Pts',(-160.935886339886,-222.514510186537,
13.9177728519871));
#76530=CARTESIAN_POINT('Ctrl Pts',(-160.002418184735,-222.344150417211,
13.8648535635765));
#76531=CARTESIAN_POINT('Ctrl Pts',(-159.210966178969,-222.604881762539,
13.8119342751659));
#76532=CARTESIAN_POINT('Ctrl Pts',(-158.419514173204,-222.865613107866,
13.7590149867553));
#76533=CARTESIAN_POINT('Ctrl Pts',(-157.770078316823,-223.557435567847,
13.7060956983447));
#76534=CARTESIAN_POINT('Ctrl Pts',(-157.559840444939,-224.363771198395,
13.6531764099341));
#76535=CARTESIAN_POINT('Ctrl Pts',(-157.349602573054,-225.170106828944,
13.6002571215235));
#76536=CARTESIAN_POINT('Ctrl Pts',(-157.578562685665,-226.090955630061,
13.5473378331129));
#76537=CARTESIAN_POINT('Ctrl Pts',(-158.141948639743,-226.704937208461,
13.4944185447023));
#76538=CARTESIAN_POINT('Ctrl Pts',(-158.705334593821,-227.318918786861,
13.4414992562917));
#76539=CARTESIAN_POINT('Ctrl Pts',(-159.603146389366,-227.626033142544,
13.3885799678811));
#76540=CARTESIAN_POINT('Ctrl Pts',(-160.424545366389,-227.485744752388,
13.3356606794705));
#76541=CARTESIAN_POINT('Ctrl Pts',(-161.245944343412,-227.345456362232,
13.2827413910599));
#76542=CARTESIAN_POINT('Ctrl Pts',(-161.990930501913,-226.757765226237,
13.2298221026493));
#76543=CARTESIAN_POINT('Ctrl Pts',(-162.31859819041,-225.991598796679,13.1769028142387));
#76544=CARTESIAN_POINT('Ctrl Pts',(-162.451350200577,-225.681192439211,
13.1554629769898));
#76545=CARTESIAN_POINT('Ctrl Pts',(-162.515603470644,-225.341491110093,
13.1340231397409));
#76546=CARTESIAN_POINT('Ctrl Pts',(-162.514086114787,-225.001240687878,
13.112583302492));
#76547=CARTESIAN_POINT('Ctrl Pts',(-162.514983776563,-224.998176142249,
13.3874166975081));
#76548=CARTESIAN_POINT('Ctrl Pts',(-162.511314108838,-225.545258590403,
13.4219203068376));
#76549=CARTESIAN_POINT('Ctrl Pts',(-162.335906246044,-226.094483494431,
13.4564239161671));
#76550=CARTESIAN_POINT('Ctrl Pts',(-162.006938674362,-226.526880084621,
13.4909275254966));
#76551=CARTESIAN_POINT('Ctrl Pts',(-161.502390595425,-227.190060554975,
13.5438468139071));
#76552=CARTESIAN_POINT('Ctrl Pts',(-160.636618833816,-227.578421842156,
13.5967661023177));
#76553=CARTESIAN_POINT('Ctrl Pts',(-159.805800530625,-227.514249828787,
13.6496853907283));
#76554=CARTESIAN_POINT('Ctrl Pts',(-158.974982227434,-227.450077815418,
13.7026046791389));
#76555=CARTESIAN_POINT('Ctrl Pts',(-158.17911738266,-226.933372501498,13.7555239675495));
#76556=CARTESIAN_POINT('Ctrl Pts',(-157.782393733624,-226.200578228517,
13.8084432559601));
#76557=CARTESIAN_POINT('Ctrl Pts',(-157.385670084588,-225.467783955537,
13.8613625443707));
#76558=CARTESIAN_POINT('Ctrl Pts',(-157.388087631289,-224.518900723497,
13.9142818327813));
#76559=CARTESIAN_POINT('Ctrl Pts',(-157.788540104405,-223.788137480721,
13.9672011211919));
#76560=CARTESIAN_POINT('Ctrl Pts',(-158.188992577521,-223.057374237944,
14.0201204096025));
#76561=CARTESIAN_POINT('Ctrl Pts',(-158.987479977051,-222.544730984433,
14.0730396980131));
#76562=CARTESIAN_POINT('Ctrl Pts',(-159.818614484671,-222.484793262913,
14.1259589864237));
#76563=CARTESIAN_POINT('Ctrl Pts',(-160.649748992291,-222.424855541393,
14.1788782748343));
#76564=CARTESIAN_POINT('Ctrl Pts',(-161.513530608,-222.817623351865,14.2317975632449));
#76565=CARTESIAN_POINT('Ctrl Pts',(-162.014692881433,-223.483366151979,
14.2847168516555));
#76566=CARTESIAN_POINT('Ctrl Pts',(-162.338892807866,-223.91403258132,14.3189501336064));
#76567=CARTESIAN_POINT('Ctrl Pts',(-162.511345757191,-224.458932104915,
14.3531834155572));
#76568=CARTESIAN_POINT('Ctrl Pts',(-162.514889488545,-225.001779462475,
14.3874166975081));
#76569=CARTESIAN_POINT('Origin',(-160.,-225.,10.));
#76570=CARTESIAN_POINT('',(-162.521411371648,-225.000821673787,15.3874166975081));
#76571=CARTESIAN_POINT('',(-162.518630481145,-224.997804626904,15.1125833024919));
#76572=CARTESIAN_POINT('',(-162.5175,-225.,10.));
#76573=CARTESIAN_POINT('Ctrl Pts',(-162.518630481145,-224.997804626904,
15.1125833024919));
#76574=CARTESIAN_POINT('Ctrl Pts',(-162.520103953586,-224.83674368871,15.1023879340014));
#76575=CARTESIAN_POINT('Ctrl Pts',(-162.505977749995,-224.675940205489,
15.0921925655108));
#76576=CARTESIAN_POINT('Ctrl Pts',(-162.47531478681,-224.51835443701,15.0819971970202));
#76577=CARTESIAN_POINT('Ctrl Pts',(-162.316157989899,-223.700401977595,
15.0290779086096));
#76578=CARTESIAN_POINT('Ctrl Pts',(-161.711475709582,-222.969139652874,
14.976158620199));
#76579=CARTESIAN_POINT('Ctrl Pts',(-160.937970545441,-222.659193088263,
14.9232393317885));
#76580=CARTESIAN_POINT('Ctrl Pts',(-160.1644653813,-222.349246523652,14.8703200433779));
#76581=CARTESIAN_POINT('Ctrl Pts',(-159.222137333336,-222.46061571915,14.8174007549673));
#76582=CARTESIAN_POINT('Ctrl Pts',(-158.542195697769,-222.942338133088,
14.7644814665567));
#76583=CARTESIAN_POINT('Ctrl Pts',(-157.862254062202,-223.424060547025,
14.7115621781461));
#76584=CARTESIAN_POINT('Ctrl Pts',(-157.444698839032,-224.276136179401,
14.6586428897355));
#76585=CARTESIAN_POINT('Ctrl Pts',(-157.480603290172,-225.108655237595,
14.6057236013249));
#76586=CARTESIAN_POINT('Ctrl Pts',(-157.516507741312,-225.941174295788,
14.5528043129143));
#76587=CARTESIAN_POINT('Ctrl Pts',(-158.005871866761,-226.754136779799,
14.4998850245037));
#76588=CARTESIAN_POINT('Ctrl Pts',(-158.724762652337,-227.175531072928,
14.4469657360931));
#76589=CARTESIAN_POINT('Ctrl Pts',(-159.443653437912,-227.596925366057,
14.3940464476825));
#76590=CARTESIAN_POINT('Ctrl Pts',(-160.392070883613,-227.626751468304,
14.3411271592719));
#76591=CARTESIAN_POINT('Ctrl Pts',(-161.136019184935,-227.251360955868,
14.2882078708613));
#76592=CARTESIAN_POINT('Ctrl Pts',(-161.879967486257,-226.875970443432,
14.2352885824507));
#76593=CARTESIAN_POINT('Ctrl Pts',(-162.4194466432,-226.095363316312,14.1823692940401));
#76594=CARTESIAN_POINT('Ctrl Pts',(-162.507591004154,-225.266745380531,
14.1294500056295));
#76595=CARTESIAN_POINT('Ctrl Pts',(-162.516955609601,-225.178711614664,
14.1238277712503));
#76596=CARTESIAN_POINT('Ctrl Pts',(-162.521225865759,-225.090135936605,
14.1182055368711));
#76597=CARTESIAN_POINT('Ctrl Pts',(-162.52060107169,-225.001499392296,14.112583302492));
#76598=CARTESIAN_POINT('Ctrl Pts',(-162.514889488545,-225.001779462475,
14.3874166975081));
#76599=CARTESIAN_POINT('Ctrl Pts',(-162.516823810444,-225.298089037601,
14.4061027039678));
#76600=CARTESIAN_POINT('Ctrl Pts',(-162.468432496996,-225.59378718038,14.4247887104276));
#76601=CARTESIAN_POINT('Ctrl Pts',(-162.366924432334,-225.869962279114,
14.4434747168873));
#76602=CARTESIAN_POINT('Ctrl Pts',(-162.079450778643,-226.652097816378,
14.4963940052979));
#76603=CARTESIAN_POINT('Ctrl Pts',(-161.365960540102,-227.277651101148,
14.5493132937085));
#76604=CARTESIAN_POINT('Ctrl Pts',(-160.55294683584,-227.460368962614,14.6022325821191));
#76605=CARTESIAN_POINT('Ctrl Pts',(-159.739933131577,-227.64308682408,14.6551518705297));
#76606=CARTESIAN_POINT('Ctrl Pts',(-158.827395961593,-227.382969262241,
14.7080711589403));
#76607=CARTESIAN_POINT('Ctrl Pts',(-158.232912316929,-226.799046068281,
14.7609904473509));
#76608=CARTESIAN_POINT('Ctrl Pts',(-157.638428672265,-226.215122874321,
14.8139097357615));
#76609=CARTESIAN_POINT('Ctrl Pts',(-157.361998552922,-225.30739404824,14.8668290241721));
#76610=CARTESIAN_POINT('Ctrl Pts',(-157.530116376076,-224.491236283003,
14.9197483125827));
#76611=CARTESIAN_POINT('Ctrl Pts',(-157.69823419923,-223.675078517767,14.9726676009933));
#76612=CARTESIAN_POINT('Ctrl Pts',(-158.310899964881,-222.950491813376,
15.0255868894039));
#76613=CARTESIAN_POINT('Ctrl Pts',(-159.087757830713,-222.649047031514,
15.0785061778145));
#76614=CARTESIAN_POINT('Ctrl Pts',(-159.864615696544,-222.347602249651,
15.1314254662251));
#76615=CARTESIAN_POINT('Ctrl Pts',(-160.805665662558,-222.469299390317,
15.1843447546357));
#76616=CARTESIAN_POINT('Ctrl Pts',(-161.480283282808,-222.958449844334,
15.2372640430463));
#76617=CARTESIAN_POINT('Ctrl Pts',(-162.118334356872,-223.421086696969,
15.2873149278669));
#76618=CARTESIAN_POINT('Ctrl Pts',(-162.518053365845,-224.212422029304,
15.3373658126875));
#76619=CARTESIAN_POINT('Ctrl Pts',(-162.521411371648,-225.000821673787,
15.3874166975081));
#76620=CARTESIAN_POINT('Origin',(-160.,-225.,10.));
#76621=CARTESIAN_POINT('',(-162.517311901221,-224.997698966112,16.3874166975081));
#76622=CARTESIAN_POINT('',(-162.513487182596,-224.999883653193,16.112583302492));
#76623=CARTESIAN_POINT('',(-162.5175,-225.,10.));
#76624=CARTESIAN_POINT('Ctrl Pts',(-162.513487182596,-224.999883653193,
16.112583302492));
#76625=CARTESIAN_POINT('Ctrl Pts',(-162.513657485401,-224.58681174506,16.0865703311316));
#76626=CARTESIAN_POINT('Ctrl Pts',(-162.417512359637,-224.17381449298,16.0605573597713));
#76627=CARTESIAN_POINT('Ctrl Pts',(-162.224617581508,-223.812463744481,
16.034544388411));
#76628=CARTESIAN_POINT('Ctrl Pts',(-161.832203571769,-223.077352625788,
15.9816251000004));
#76629=CARTESIAN_POINT('Ctrl Pts',(-161.03938641789,-222.55598307528,15.9287058115898));
#76630=CARTESIAN_POINT('Ctrl Pts',(-160.208959233887,-222.486933789028,
15.8757865231792));
#76631=CARTESIAN_POINT('Ctrl Pts',(-159.378532049883,-222.417884502776,
15.8228672347686));
#76632=CARTESIAN_POINT('Ctrl Pts',(-158.510494835754,-222.801155480781,
15.769947946358));
#76633=CARTESIAN_POINT('Ctrl Pts',(-158.002061403624,-223.461361931038,
15.7170286579474));
#76634=CARTESIAN_POINT('Ctrl Pts',(-157.493627971493,-224.121568381295,
15.6641093695368));
#76635=CARTESIAN_POINT('Ctrl Pts',(-157.344798321362,-225.058710303804,
15.6111900811262));
#76636=CARTESIAN_POINT('Ctrl Pts',(-157.6236768982,-225.843951573254,15.5582707927156));
#76637=CARTESIAN_POINT('Ctrl Pts',(-157.902555475038,-226.629192842704,
15.505351504305));
#76638=CARTESIAN_POINT('Ctrl Pts',(-158.609142278846,-227.262533459095,
15.4524322158944));
#76639=CARTESIAN_POINT('Ctrl Pts',(-159.420103202096,-227.454156768817,
15.3995129274838));
#76640=CARTESIAN_POINT('Ctrl Pts',(-160.231064125345,-227.645780078539,
15.3465936390732));
#76641=CARTESIAN_POINT('Ctrl Pts',(-161.146399168037,-227.395686081594,
15.2936743506626));
#76642=CARTESIAN_POINT('Ctrl Pts',(-161.74725103263,-226.818317786065,15.240755062252));
#76643=CARTESIAN_POINT('Ctrl Pts',(-162.232343476571,-226.352184594116,
15.198031142332));
#76644=CARTESIAN_POINT('Ctrl Pts',(-162.51245586189,-225.672734094338,15.155307222412));
#76645=CARTESIAN_POINT('Ctrl Pts',(-162.518630481145,-224.997804626904,
15.1125833024919));
#76646=CARTESIAN_POINT('Ctrl Pts',(-162.521411371648,-225.000821673787,
15.3874166975081));
#76647=CARTESIAN_POINT('Ctrl Pts',(-162.521603818114,-225.046004658637,
15.3902851010981));
#76648=CARTESIAN_POINT('Ctrl Pts',(-162.520494453647,-225.091178001493,
15.3931535046881));
#76649=CARTESIAN_POINT('Ctrl Pts',(-162.518053532688,-225.136279279337,
15.3960219082781));
#76650=CARTESIAN_POINT('Ctrl Pts',(-162.473020887832,-225.968354492954,
15.4489411966887));
#76651=CARTESIAN_POINT('Ctrl Pts',(-161.974770323632,-226.775901152821,
15.5018604850993));
#76652=CARTESIAN_POINT('Ctrl Pts',(-161.251301288472,-227.189385923252,
15.5547797735098));
#76653=CARTESIAN_POINT('Ctrl Pts',(-160.527832253312,-227.602870693684,
15.6076990619204));
#76654=CARTESIAN_POINT('Ctrl Pts',(-159.579144747191,-227.62229357468,15.660618350331));
#76655=CARTESIAN_POINT('Ctrl Pts',(-158.839358154254,-227.238766656296,
15.7135376387416));
#76656=CARTESIAN_POINT('Ctrl Pts',(-158.099571561317,-226.855239737911,
15.7664569271522));
#76657=CARTESIAN_POINT('Ctrl Pts',(-157.568685881563,-226.068763020145,
15.8193762155628));
#76658=CARTESIAN_POINT('Ctrl Pts',(-157.489634391618,-225.23922823355,15.8722955039734));
#76659=CARTESIAN_POINT('Ctrl Pts',(-157.410582901673,-224.409693446955,
15.925214792384));
#76660=CARTESIAN_POINT('Ctrl Pts',(-157.783365601536,-223.537100591531,
15.9781340807946));
#76661=CARTESIAN_POINT('Ctrl Pts',(-158.437397135063,-223.020748140834,
16.0310533692052));
#76662=CARTESIAN_POINT('Ctrl Pts',(-159.091428668591,-222.504395690137,
16.0839726576158));
#76663=CARTESIAN_POINT('Ctrl Pts',(-160.026709035783,-222.344283644167,
16.1368919460264));
#76664=CARTESIAN_POINT('Ctrl Pts',(-160.815253959035,-222.613679271864,
16.189811234437));
#76665=CARTESIAN_POINT('Ctrl Pts',(-161.603798882287,-222.88307489956,16.2427305228476));
#76666=CARTESIAN_POINT('Ctrl Pts',(-162.245608361599,-223.581978200923,
16.2956498112582));
#76667=CARTESIAN_POINT('Ctrl Pts',(-162.446990391789,-224.390571039299,
16.3485690996688));
#76668=CARTESIAN_POINT('Ctrl Pts',(-162.496268001497,-224.588431405808,
16.3615182989486));
#76669=CARTESIAN_POINT('Ctrl Pts',(-162.519174270148,-224.792859619522,
16.3744674982283));
#76670=CARTESIAN_POINT('Ctrl Pts',(-162.517311901221,-224.997698966112,
16.3874166975081));
#76671=CARTESIAN_POINT('Origin',(-160.,-225.,10.));
#76672=CARTESIAN_POINT('',(-162.513611870269,-225.000594615134,17.3874166975081));
#76673=CARTESIAN_POINT('',(-162.518203497722,-225.002256423796,17.1125833024919));
#76674=CARTESIAN_POINT('',(-162.5175,-225.,10.));
#76675=CARTESIAN_POINT('Ctrl Pts',(-162.518203497722,-225.002256423796,
17.1125833024919));
#76676=CARTESIAN_POINT('Ctrl Pts',(-162.512102188789,-224.341151222928,
17.0707527282619));
#76677=CARTESIAN_POINT('Ctrl Pts',(-162.244817978816,-223.675680014097,
17.0289221540318));
#76678=CARTESIAN_POINT('Ctrl Pts',(-161.777620829493,-223.211360872938,
16.9870915798017));
#76679=CARTESIAN_POINT('Ctrl Pts',(-161.186576093803,-222.623957066085,
16.9341722913911));
#76680=CARTESIAN_POINT('Ctrl Pts',(-160.275581999903,-222.358485772275,
16.8812530029806));
#76681=CARTESIAN_POINT('Ctrl Pts',(-159.461509426251,-222.536426651267,
16.82833371457));
#76682=CARTESIAN_POINT('Ctrl Pts',(-158.647436852599,-222.71436753026,16.7754144261594));
#76683=CARTESIAN_POINT('Ctrl Pts',(-157.930285799196,-223.335720582054,
16.7224951377488));
#76684=CARTESIAN_POINT('Ctrl Pts',(-157.638224574459,-224.116154661917,
16.6695758493382));
#76685=CARTESIAN_POINT('Ctrl Pts',(-157.346163349722,-224.89658874178,16.6166565609276));
#76686=CARTESIAN_POINT('Ctrl Pts',(-157.479191953652,-225.836103849712,
16.563737272517));
#76687=CARTESIAN_POINT('Ctrl Pts',(-157.976436499474,-226.504777891013,
16.5108179841064));
#76688=CARTESIAN_POINT('Ctrl Pts',(-158.473681045295,-227.173451932314,
16.4578986956958));
#76689=CARTESIAN_POINT('Ctrl Pts',(-159.335141533009,-227.571284906983,
16.4049794072852));
#76690=CARTESIAN_POINT('Ctrl Pts',(-160.166613660486,-227.516228453529,
16.3520601188746));
#76691=CARTESIAN_POINT('Ctrl Pts',(-160.998085787964,-227.461172000076,
16.299140830464));
#76692=CARTESIAN_POINT('Ctrl Pts',(-161.799569555205,-226.953226118501,
16.2462215420534));
#76693=CARTESIAN_POINT('Ctrl Pts',(-162.204306006026,-226.224826834275,
16.1933022536428));
#76694=CARTESIAN_POINT('Ctrl Pts',(-162.410090467508,-225.854479033516,
16.1663959365925));
#76695=CARTESIAN_POINT('Ctrl Pts',(-162.513311031199,-225.427141407443,
16.1394896195422));
#76696=CARTESIAN_POINT('Ctrl Pts',(-162.513487182596,-224.999883653193,
16.112583302492));
#76697=CARTESIAN_POINT('Ctrl Pts',(-162.517311901221,-224.997698966112,
16.3874166975081));
#76698=CARTESIAN_POINT('Ctrl Pts',(-162.511563356433,-225.629973345696,
16.4273867866389));
#76699=CARTESIAN_POINT('Ctrl Pts',(-162.269828657284,-226.266164842886,
16.4673568757698));
#76700=CARTESIAN_POINT('Ctrl Pts',(-161.839241314137,-226.725212167904,
16.5073269649006));
#76701=CARTESIAN_POINT('Ctrl Pts',(-161.269155625227,-227.332978082743,
16.5602462533112));
#76702=CARTESIAN_POINT('Ctrl Pts',(-160.368029666341,-227.630227537028,
16.6131655417218));
#76703=CARTESIAN_POINT('Ctrl Pts',(-159.548218658251,-227.48093918766,16.6660848301324));
#76704=CARTESIAN_POINT('Ctrl Pts',(-158.728407650161,-227.331650838291,
16.719004118543));
#76705=CARTESIAN_POINT('Ctrl Pts',(-157.989911592869,-226.735824685267,
16.7719234069536));
#76706=CARTESIAN_POINT('Ctrl Pts',(-157.670666268281,-225.966110761729,
16.8248426953642));
#76707=CARTESIAN_POINT('Ctrl Pts',(-157.351420943693,-225.19639683819,16.8777619837748));
#76708=CARTESIAN_POINT('Ctrl Pts',(-157.451426351811,-224.252795144137,
16.9306812721854));
#76709=CARTESIAN_POINT('Ctrl Pts',(-157.924920018577,-223.567097801959,
16.983600560596));
#76710=CARTESIAN_POINT('Ctrl Pts',(-158.398413685342,-222.881400459781,
17.0365198490066));
#76711=CARTESIAN_POINT('Ctrl Pts',(-159.245395610756,-222.45360746948,17.0894391374172));
#76712=CARTESIAN_POINT('Ctrl Pts',(-160.078286885035,-222.479476883083,
17.1423584258278));
#76713=CARTESIAN_POINT('Ctrl Pts',(-160.911178159314,-222.505346296687,
17.1952777142384));
#76714=CARTESIAN_POINT('Ctrl Pts',(-161.729978782458,-222.984878114195,
17.248197002649));
#76715=CARTESIAN_POINT('Ctrl Pts',(-162.160005599952,-223.698638610084,
17.3011162910596));
#76716=CARTESIAN_POINT('Ctrl Pts',(-162.393767178185,-224.086637156247,
17.3298830932091));
#76717=CARTESIAN_POINT('Ctrl Pts',(-162.512646706287,-224.543849909697,
17.3586498953586));
#76718=CARTESIAN_POINT('Ctrl Pts',(-162.513611870269,-225.000594615134,
17.3874166975081));
#76719=CARTESIAN_POINT('Origin',(-160.,-225.,10.));
#76720=CARTESIAN_POINT('',(-162.519491502139,-225.001988389076,18.3874166975081));
#76721=CARTESIAN_POINT('',(-162.520906603697,-224.998703157721,18.112583302492));
#76722=CARTESIAN_POINT('',(-162.5175,-225.,10.));
#76723=CARTESIAN_POINT('Ctrl Pts',(-162.520906603697,-224.998703157721,
18.112583302492));
#76724=CARTESIAN_POINT('Ctrl Pts',(-162.521374483509,-224.924174319773,
18.1078544138027));
#76725=CARTESIAN_POINT('Ctrl Pts',(-162.518355778069,-224.84968391501,18.1031255251135));
#76726=CARTESIAN_POINT('Ctrl Pts',(-162.511727091913,-224.775516150632,
18.0983966364243));
#76727=CARTESIAN_POINT('Ctrl Pts',(-162.437547854986,-223.945531439255,
18.0454773480137));
#76728=CARTESIAN_POINT('Ctrl Pts',(-161.911289246659,-223.155951116232,
17.9925580596031));
#76729=CARTESIAN_POINT('Ctrl Pts',(-161.173767361169,-222.768086967393,
17.9396387711925));
#76730=CARTESIAN_POINT('Ctrl Pts',(-160.436245475678,-222.380222818555,
17.8867194827819));
#76731=CARTESIAN_POINT('Ctrl Pts',(-159.487460313023,-222.394074843902,
17.8338001943713));
#76732=CARTESIAN_POINT('Ctrl Pts',(-158.761575865264,-222.803304431344,
17.7808809059607));
#76733=CARTESIAN_POINT('Ctrl Pts',(-158.035691417506,-223.212534018787,
17.7279616175501));
#76734=CARTESIAN_POINT('Ctrl Pts',(-157.532707684643,-224.017141168325,
17.6750423291395));
#76735=CARTESIAN_POINT('Ctrl Pts',(-157.482790051362,-224.848937628277,
17.6221230407289));
#76736=CARTESIAN_POINT('Ctrl Pts',(-157.43287241808,-225.68073408823,17.5692037523183));
#76737=CARTESIAN_POINT('Ctrl Pts',(-157.836020884379,-226.539719858598,
17.5162844639077));
#76738=CARTESIAN_POINT('Ctrl Pts',(-158.507754701494,-227.032823085037,
17.4633651754971));
#76739=CARTESIAN_POINT('Ctrl Pts',(-159.179488518608,-227.525926311476,
17.4104458870865));
#76740=CARTESIAN_POINT('Ctrl Pts',(-160.119807686538,-227.653146993986,
17.3575265986759));
#76741=CARTESIAN_POINT('Ctrl Pts',(-160.89842218145,-227.356268942422,17.3046073102653));
#76742=CARTESIAN_POINT('Ctrl Pts',(-161.677036676361,-227.059390890857,
17.2516880218547));
#76743=CARTESIAN_POINT('Ctrl Pts',(-162.293946498254,-226.338414105218,
17.1987687334441));
#76744=CARTESIAN_POINT('Ctrl Pts',(-162.466853720459,-225.523257552451,
17.1458494450335));
#76745=CARTESIAN_POINT('Ctrl Pts',(-162.503084720996,-225.35244954846,17.134760730853));
#76746=CARTESIAN_POINT('Ctrl Pts',(-162.519820871428,-225.177506387504,
17.1236720166725));
#76747=CARTESIAN_POINT('Ctrl Pts',(-162.518203497722,-225.002256423796,
17.1125833024919));
#76748=CARTESIAN_POINT('Ctrl Pts',(-162.513611870269,-225.000594615134,
17.3874166975081));
#76749=CARTESIAN_POINT('Ctrl Pts',(-162.514422217894,-225.384075551442,
17.4115691837692));
#76750=CARTESIAN_POINT('Ctrl Pts',(-162.432112241408,-225.767226550828,
17.4357216700303));
#76751=CARTESIAN_POINT('Ctrl Pts',(-162.264887269412,-226.10880625405,17.4598741562914));
#76752=CARTESIAN_POINT('Ctrl Pts',(-161.898489109535,-226.85722422786,17.512793444702));
#76753=CARTESIAN_POINT('Ctrl Pts',(-161.124439777939,-227.406071001213,
17.5657127331126));
#76754=CARTESIAN_POINT('Ctrl Pts',(-160.296944210013,-227.504194407927,
17.6186320215232));
#76755=CARTESIAN_POINT('Ctrl Pts',(-159.469448642086,-227.602317814641,
17.6715513099338));
#76756=CARTESIAN_POINT('Ctrl Pts',(-158.58850683783,-227.249717854717,17.7244705983443));
#76757=CARTESIAN_POINT('Ctrl Pts',(-158.057237798374,-226.607744041865,
17.7773898867549));
#76758=CARTESIAN_POINT('Ctrl Pts',(-157.525968758919,-225.965770229013,
17.8303091751655));
#76759=CARTESIAN_POINT('Ctrl Pts',(-157.344372484265,-225.034422563233,
17.8832284635761));
#76760=CARTESIAN_POINT('Ctrl Pts',(-157.595547324811,-224.23988617669,17.9361477519867));
#76761=CARTESIAN_POINT('Ctrl Pts',(-157.846722165357,-223.445349790147,
17.9890670403973));
#76762=CARTESIAN_POINT('Ctrl Pts',(-158.530668121103,-222.78762468284,18.0419863288079));
#76763=CARTESIAN_POINT('Ctrl Pts',(-159.334411746373,-222.567684899305,
18.0949056172185));
#76764=CARTESIAN_POINT('Ctrl Pts',(-160.138155371642,-222.34774511577,18.1478249056291));
#76765=CARTESIAN_POINT('Ctrl Pts',(-161.061696666434,-222.565590656007,
18.2007441940397));
#76766=CARTESIAN_POINT('Ctrl Pts',(-161.682422716191,-223.12153737975,18.2536634824503));
#76767=CARTESIAN_POINT('Ctrl Pts',(-162.205383293319,-223.589921491573,
18.2982478874696));
#76768=CARTESIAN_POINT('Ctrl Pts',(-162.513404637407,-224.29829090884,18.3428322924888));
#76769=CARTESIAN_POINT('Ctrl Pts',(-162.519491502139,-225.001988389076,
18.3874166975081));
#76770=CARTESIAN_POINT('Origin',(-160.,-225.,10.));
#76771=CARTESIAN_POINT('',(-162.519857325378,-224.99817643576,19.3874166975081));
#76772=CARTESIAN_POINT('',(-162.514309543052,-224.998572563953,19.1125833024919));
#76773=CARTESIAN_POINT('',(-162.5175,-225.,10.));
#76774=CARTESIAN_POINT('',(-158.086534003335,-223.364012796625,20.));
#76775=CARTESIAN_POINT('Ctrl Pts',(-162.519857325378,-224.99817643576,19.3874166975081));
#76776=CARTESIAN_POINT('Ctrl Pts',(-162.513963987124,-225.714913340689,
19.4328532664403));
#76777=CARTESIAN_POINT('Ctrl Pts',(-162.192666865723,-226.43617652876,19.4782898353725));
#76778=CARTESIAN_POINT('Ctrl Pts',(-161.652076061567,-226.905064858465,
19.5237264043047));
#76779=CARTESIAN_POINT('Ctrl Pts',(-161.022458083151,-227.451172043386,
19.5766456927153));
#76780=CARTESIAN_POINT('Ctrl Pts',(-160.095370186091,-227.654934990922,
19.6295649811259));
#76781=CARTESIAN_POINT('Ctrl Pts',(-159.295373481316,-227.421707534687,
19.6824842695365));
#76782=CARTESIAN_POINT('Ctrl Pts',(-158.49537677654,-227.188480078453,19.7354035579471));
#76783=CARTESIAN_POINT('Ctrl Pts',(-157.82247126405,-226.518262218448,19.7883228463576));
#76784=CARTESIAN_POINT('Ctrl Pts',(-157.584268441052,-225.721203069991,
19.8412421347682));
#76785=CARTESIAN_POINT('Ctrl Pts',(-157.346065618053,-224.924143921533,
19.8941614231788));
#76786=CARTESIAN_POINT('Ctrl Pts',(-157.542565484547,-224.000243484621,
19.9470807115894));
#76787=CARTESIAN_POINT('Ctrl Pts',(-158.086534003335,-223.364012796625,
20.));
#76788=CARTESIAN_POINT('',(-161.917152659427,-223.361245045743,20.));
#76789=CARTESIAN_POINT('Origin',(-160.,-225.,20.));
#76790=CARTESIAN_POINT('Ctrl Pts',(-161.91715636014,-223.361242267444,20.));
#76791=CARTESIAN_POINT('Ctrl Pts',(-161.386618601236,-222.742548953518,
19.948244384658));
#76792=CARTESIAN_POINT('Ctrl Pts',(-160.527623964281,-222.402875584563,
19.896488769316));
#76793=CARTESIAN_POINT('Ctrl Pts',(-159.717628707495,-222.49422785314,19.844733153974));
#76794=CARTESIAN_POINT('Ctrl Pts',(-158.889421520279,-222.587634085795,
19.7918138655634));
#76795=CARTESIAN_POINT('Ctrl Pts',(-158.112441887667,-223.131666210172,
19.7388945771528));
#76796=CARTESIAN_POINT('Ctrl Pts',(-157.741727813776,-223.877852582083,
19.6859752887422));
#76797=CARTESIAN_POINT('Ctrl Pts',(-157.371013739885,-224.624038953993,
19.6330560003316));
#76798=CARTESIAN_POINT('Ctrl Pts',(-157.406565224716,-225.572379573437,
19.580136711921));
#76799=CARTESIAN_POINT('Ctrl Pts',(-157.832358767884,-226.288685324508,
19.5272174235104));
#76800=CARTESIAN_POINT('Ctrl Pts',(-158.258152311052,-227.004991075579,
19.4742981350998));
#76801=CARTESIAN_POINT('Ctrl Pts',(-159.074187912558,-227.489261958278,
19.4213788466892));
#76802=CARTESIAN_POINT('Ctrl Pts',(-159.906929719594,-227.520005809176,
19.3684595582786));
#76803=CARTESIAN_POINT('Ctrl Pts',(-160.73967152663,-227.550749660074,19.315540269868));
#76804=CARTESIAN_POINT('Ctrl Pts',(-161.589119539195,-227.127966479172,
19.2626209814574));
#76805=CARTESIAN_POINT('Ctrl Pts',(-162.066623220182,-226.445068751754,
19.2097016930468));
#76806=CARTESIAN_POINT('Ctrl Pts',(-162.358730883091,-226.027313523668,
19.1773288961952));
#76807=CARTESIAN_POINT('Ctrl Pts',(-162.511647788968,-225.512217006655,
19.1449560993436));
#76808=CARTESIAN_POINT('Ctrl Pts',(-162.514309543052,-224.998572563953,
19.1125833024919));
#76809=CARTESIAN_POINT('Origin',(160.,-225.,10.));
#76810=CARTESIAN_POINT('',(157.486483996142,-224.999424946341,0.38741669750801));
#76811=CARTESIAN_POINT('',(157.484597045422,-225.003739798663,0.112583302491969));
#76812=CARTESIAN_POINT('',(157.4825,-225.,10.));
#76813=CARTESIAN_POINT('',(158.086534003335,-223.364012796625,0.));
#76814=CARTESIAN_POINT('Ctrl Pts',(157.484597045422,-225.003739798663,0.112583302491969));
#76815=CARTESIAN_POINT('Ctrl Pts',(157.489762314943,-224.411047445606,0.0750555349946397));
#76816=CARTESIAN_POINT('Ctrl Pts',(157.700778171916,-223.815196439696,0.0375277674973106));
#76817=CARTESIAN_POINT('Ctrl Pts',(158.086534003335,-223.364012796625,-1.88044024795886E-14));
#76818=CARTESIAN_POINT('',(161.917152683146,-223.361245013972,6.04505606088546E-15));
#76819=CARTESIAN_POINT('Origin',(160.,-225.,0.));
#76820=CARTESIAN_POINT('Ctrl Pts',(161.9171563836,-223.361242235853,4.27813134826349E-15));
#76821=CARTESIAN_POINT('Ctrl Pts',(161.386618632273,-222.742548965135,0.0517556153419861));
#76822=CARTESIAN_POINT('Ctrl Pts',(160.52762397761,-222.402875530323,0.103511230683966));
#76823=CARTESIAN_POINT('Ctrl Pts',(159.717628704827,-222.494227788249,0.155266846025948));
#76824=CARTESIAN_POINT('Ctrl Pts',(158.889421501254,-222.587634010013,0.208186134436545));
#76825=CARTESIAN_POINT('Ctrl Pts',(158.112441854074,-223.131666181215,0.261105422847145));
#76826=CARTESIAN_POINT('Ctrl Pts',(157.741727774883,-223.877852574113,0.314024711257743));
#76827=CARTESIAN_POINT('Ctrl Pts',(157.5703508005,-224.222806201499,0.338488706674499));
#76828=CARTESIAN_POINT('Ctrl Pts',(157.485797228021,-224.610962400354,0.362952702091254));
#76829=CARTESIAN_POINT('Ctrl Pts',(157.486483996142,-224.999424946341,0.38741669750801));
#76830=CARTESIAN_POINT('Origin',(160.,-225.,10.));
#76831=CARTESIAN_POINT('',(157.482539823067,-225.002301238291,1.38741669750801));
#76832=CARTESIAN_POINT('',(157.478271630914,-224.999864677068,1.11258330249197));
#76833=CARTESIAN_POINT('',(157.4825,-225.,10.));
#76834=CARTESIAN_POINT('Ctrl Pts',(157.478271630914,-224.999864677068,1.11258330249197));
#76835=CARTESIAN_POINT('Ctrl Pts',(157.478266758284,-224.993155409996,1.11215722053549));
#76836=CARTESIAN_POINT('Ctrl Pts',(157.478291201374,-224.986446181325,1.11173113857901));
#76837=CARTESIAN_POINT('Ctrl Pts',(157.478345066988,-224.979737190974,1.11130505662253));
#76838=CARTESIAN_POINT('Ctrl Pts',(157.485035164759,-224.14648201563,1.05838576821194));
#76839=CARTESIAN_POINT('Ctrl Pts',(157.945584954632,-223.316903059734,1.00546647980134));
#76840=CARTESIAN_POINT('Ctrl Pts',(158.649263628601,-222.870539628389,0.952547191390737));
#76841=CARTESIAN_POINT('Ctrl Pts',(159.35294230257,-222.424176197045,0.89962790298014));
#76842=CARTESIAN_POINT('Ctrl Pts',(160.299749860634,-222.361028290252,0.846708614569545));
#76843=CARTESIAN_POINT('Ctrl Pts',(161.056392406879,-222.710150110404,0.793789326158948));
#76844=CARTESIAN_POINT('Ctrl Pts',(161.813034953124,-223.059271930555,0.74087003774835));
#76845=CARTESIAN_POINT('Ctrl Pts',(162.37951248755,-223.820663477651,0.687950749337751));
#76846=CARTESIAN_POINT('Ctrl Pts',(162.496677191016,-224.645584853209,0.635031460927153));
#76847=CARTESIAN_POINT('Ctrl Pts',(162.613841894483,-225.470506228767,0.582112172516556));
#76848=CARTESIAN_POINT('Ctrl Pts',(162.281693766989,-226.358957432787,0.529192884105958));
#76849=CARTESIAN_POINT('Ctrl Pts',(161.652075880165,-226.90506461644,0.476273595695361));
#76850=CARTESIAN_POINT('Ctrl Pts',(161.02245799334,-227.451171800092,0.423354307284765));
#76851=CARTESIAN_POINT('Ctrl Pts',(160.095370347186,-227.654934963376,0.370435018874168));
#76852=CARTESIAN_POINT('Ctrl Pts',(159.295373478101,-227.421707341511,0.317515730463572));
#76853=CARTESIAN_POINT('Ctrl Pts',(158.495376609015,-227.188479719646,0.264596442052972));
#76854=CARTESIAN_POINT('Ctrl Pts',(157.822470517,-226.518261312633,0.211677153642375));
#76855=CARTESIAN_POINT('Ctrl Pts',(157.584267735883,-225.721202253877,0.158757865231775));
#76856=CARTESIAN_POINT('Ctrl Pts',(157.514986700607,-225.489378441796,0.143366344318507));
#76857=CARTESIAN_POINT('Ctrl Pts',(157.482478577974,-225.246824782278,0.127974823405238));
#76858=CARTESIAN_POINT('Ctrl Pts',(157.484597045422,-225.003739798663,0.112583302491969));
#76859=CARTESIAN_POINT('Ctrl Pts',(157.486483996142,-224.999424946341,0.38741669750801));
#76860=CARTESIAN_POINT('Ctrl Pts',(157.487282810391,-225.451265104701,0.415871990501851));
#76861=CARTESIAN_POINT('Ctrl Pts',(157.603404782612,-225.90351972549,0.444327283495692));
#76862=CARTESIAN_POINT('Ctrl Pts',(157.832358734819,-226.28868533952,0.472782576489532));
#76863=CARTESIAN_POINT('Ctrl Pts',(158.258152285151,-227.004991097435,0.52570186490013));
#76864=CARTESIAN_POINT('Ctrl Pts',(159.074187897019,-227.489261998672,0.578621153310728));
#76865=CARTESIAN_POINT('Ctrl Pts',(159.906929716988,-227.520005852602,0.631540441721327));
#76866=CARTESIAN_POINT('Ctrl Pts',(160.739671536957,-227.550749706533,0.684459730131924));
#76867=CARTESIAN_POINT('Ctrl Pts',(161.589119565027,-227.127966513156,0.737379018542522));
#76868=CARTESIAN_POINT('Ctrl Pts',(162.066623254035,-226.445068773419,0.790298306953119));
#76869=CARTESIAN_POINT('Ctrl Pts',(162.544126943043,-225.762171033683,0.843217595363718));
#76870=CARTESIAN_POINT('Ctrl Pts',(162.649686292989,-224.819158747586,0.896136883774314));
#76871=CARTESIAN_POINT('Ctrl Pts',(162.334969949118,-224.047579899124,0.949056172184912));
#76872=CARTESIAN_POINT('Ctrl Pts',(162.020253605247,-223.276001050662,1.00197546059551));
#76873=CARTESIAN_POINT('Ctrl Pts',(161.285261567559,-222.675855639836,1.05489474900611));
#76874=CARTESIAN_POINT('Ctrl Pts',(160.466339381582,-222.521757867424,1.1078140374167));
#76875=CARTESIAN_POINT('Ctrl Pts',(159.647417195605,-222.367660095012,1.1607333258273));
#76876=CARTESIAN_POINT('Ctrl Pts',(158.74456486134,-222.659609961014,1.2136526142379));
#76877=CARTESIAN_POINT('Ctrl Pts',(158.170921226274,-223.264017153202,1.26657190264849));
#76878=CARTESIAN_POINT('Ctrl Pts',(157.734269805566,-223.724085465692,1.306853500935));
#76879=CARTESIAN_POINT('Ctrl Pts',(157.488364938267,-224.365194431732,1.3471350992215));
#76880=CARTESIAN_POINT('Ctrl Pts',(157.482539823067,-225.002301238291,1.38741669750801));
#76881=CARTESIAN_POINT('Origin',(160.,-225.,10.));
#76882=CARTESIAN_POINT('',(157.478659134318,-224.999094471329,2.38741669750801));
#76883=CARTESIAN_POINT('',(157.484174852024,-224.997885174718,2.11258330249197));
#76884=CARTESIAN_POINT('',(157.4825,-225.,10.));
#76885=CARTESIAN_POINT('Ctrl Pts',(157.484174852024,-224.997885174718,2.11258330249197));
#76886=CARTESIAN_POINT('Ctrl Pts',(157.482125749745,-224.740545664016,2.09633961766574));
#76887=CARTESIAN_POINT('Ctrl Pts',(157.518448874547,-224.483770799219,2.08009593283951));
#76888=CARTESIAN_POINT('Ctrl Pts',(157.595547504626,-224.239886233381,2.06385224801329));
#76889=CARTESIAN_POINT('Ctrl Pts',(157.846722326401,-223.445349906401,2.01093295960269));
#76890=CARTESIAN_POINT('Ctrl Pts',(158.53066823104,-222.787624848871,1.95801367119209));
#76891=CARTESIAN_POINT('Ctrl Pts',(159.334411796167,-222.567685081513,1.9050943827815));
#76892=CARTESIAN_POINT('Ctrl Pts',(160.138155361294,-222.347745314154,1.8521750943709));
#76893=CARTESIAN_POINT('Ctrl Pts',(161.061696586909,-222.565590836967,1.7992558059603));
#76894=CARTESIAN_POINT('Ctrl Pts',(161.682422590323,-223.12153751965,1.7463365175497));
#76895=CARTESIAN_POINT('Ctrl Pts',(162.303148593736,-223.677484202334,1.6934172291391));
#76896=CARTESIAN_POINT('Ctrl Pts',(162.621059374948,-224.571532044889,1.64049794072851));
#76897=CARTESIAN_POINT('Ctrl Pts',(162.490679871376,-225.39456067087,1.58757865231791));
#76898=CARTESIAN_POINT('Ctrl Pts',(162.360300367805,-226.217589296851,1.53465936390731));
#76899=CARTESIAN_POINT('Ctrl Pts',(161.781630579449,-226.969598706259,1.48174007549671));
#76900=CARTESIAN_POINT('Ctrl Pts',(161.019467913069,-227.306477917669,1.42882078708612));
#76901=CARTESIAN_POINT('Ctrl Pts',(160.257305246689,-227.643357129078,1.37590149867552));
#76902=CARTESIAN_POINT('Ctrl Pts',(159.311649702285,-227.565106142489,1.32298221026492));
#76903=CARTESIAN_POINT('Ctrl Pts',(158.615237132917,-227.107514951799,1.27006292185432));
#76904=CARTESIAN_POINT('Ctrl Pts',(157.924431759696,-226.653608076519,1.2175697154002));
#76905=CARTESIAN_POINT('Ctrl Pts',(157.478871937926,-225.826444953881,1.16507650894609));
#76906=CARTESIAN_POINT('Ctrl Pts',(157.478271630914,-224.999864677068,1.11258330249197));
#76907=CARTESIAN_POINT('Ctrl Pts',(157.482539823067,-225.002301238291,1.38741669750801));
#76908=CARTESIAN_POINT('Ctrl Pts',(157.480712288809,-225.202183038908,1.4000543876321));
#76909=CARTESIAN_POINT('Ctrl Pts',(157.502515506984,-225.401670911927,1.41269207775619));
#76910=CARTESIAN_POINT('Ctrl Pts',(157.549472906877,-225.595050659854,1.42532976788029));
#76911=CARTESIAN_POINT('Ctrl Pts',(157.746103158413,-226.404812455942,1.47824905629089));
#76912=CARTESIAN_POINT('Ctrl Pts',(158.383798597353,-227.107471529744,1.53116834470148));
#76913=CARTESIAN_POINT('Ctrl Pts',(159.170748325666,-227.381492482561,1.58408763311208));
#76914=CARTESIAN_POINT('Ctrl Pts',(159.95769805398,-227.655513435377,1.63700692152268));
#76915=CARTESIAN_POINT('Ctrl Pts',(160.893902071666,-227.500896267209,1.68992620993327));
#76916=CARTESIAN_POINT('Ctrl Pts',(161.550954150764,-226.988393126299,1.74284549834387));
#76917=CARTESIAN_POINT('Ctrl Pts',(162.208006229861,-226.475889985388,1.79576478675447));
#76918=CARTESIAN_POINT('Ctrl Pts',(162.585906370371,-225.605500871734,1.84868407516507));
#76919=CARTESIAN_POINT('Ctrl Pts',(162.511727132244,-224.775516147041,1.90160336357567));
#76920=CARTESIAN_POINT('Ctrl Pts',(162.437547894118,-223.945531422348,1.95452265198626));
#76921=CARTESIAN_POINT('Ctrl Pts',(161.911289277357,-223.155951086614,2.00744194039686));
#76922=CARTESIAN_POINT('Ctrl Pts',(161.173767380025,-222.768086931539,2.06036122880746));
#76923=CARTESIAN_POINT('Ctrl Pts',(160.436245482693,-222.380222776464,2.11328051721805));
#76924=CARTESIAN_POINT('Ctrl Pts',(159.487460304791,-222.394074802048,2.16619980562865));
#76925=CARTESIAN_POINT('Ctrl Pts',(158.761575845372,-222.803304396067,2.21911909403925));
#76926=CARTESIAN_POINT('Ctrl Pts',(158.035691385952,-223.212533990086,2.27203838244985));
#76927=CARTESIAN_POINT('Ctrl Pts',(157.532707645016,-224.017141152539,2.32495767086044));
#76928=CARTESIAN_POINT('Ctrl Pts',(157.482790010934,-224.84893762585,2.37787695927104));
#76929=CARTESIAN_POINT('Ctrl Pts',(157.479790467183,-224.898920161267,2.3810568720167));
#76930=CARTESIAN_POINT('Ctrl Pts',(157.478426850695,-224.949000871619,2.38423678476235));
#76931=CARTESIAN_POINT('Ctrl Pts',(157.478659134318,-224.999094471329,2.38741669750801));
#76932=CARTESIAN_POINT('Origin',(160.,-225.,10.));
#76933=CARTESIAN_POINT('',(157.485215918653,-224.99827376338,3.38741669750801));
#76934=CARTESIAN_POINT('',(157.485769737505,-225.001366316787,3.11258330249197));
#76935=CARTESIAN_POINT('',(157.4825,-225.,10.));
#76936=CARTESIAN_POINT('Ctrl Pts',(157.485769737505,-225.001366316787,3.11258330249197));
#76937=CARTESIAN_POINT('Ctrl Pts',(157.488277094539,-224.492626544162,3.080522014796));
#76938=CARTESIAN_POINT('Ctrl Pts',(157.638052833085,-223.982529385542,3.04846072710002));
#76939=CARTESIAN_POINT('Ctrl Pts',(157.924920173766,-223.567097909119,3.01639943940404));
#76940=CARTESIAN_POINT('Ctrl Pts',(158.39841380512,-222.881400618225,2.96348015099344));
#76941=CARTESIAN_POINT('Ctrl Pts',(159.24539566719,-222.453607659927,2.91056086258285));
#76942=CARTESIAN_POINT('Ctrl Pts',(160.07828687918,-222.479477071591,2.85764157417225));
#76943=CARTESIAN_POINT('Ctrl Pts',(160.911178091169,-222.505346483254,2.80472228576165));
#76944=CARTESIAN_POINT('Ctrl Pts',(161.729978653078,-222.98487826488,2.75180299735105));
#76945=CARTESIAN_POINT('Ctrl Pts',(162.160005438412,-223.698638707398,2.69888370894046));
#76946=CARTESIAN_POINT('Ctrl Pts',(162.590032223745,-224.412399149916,2.64596442052986));
#76947=CARTESIAN_POINT('Ctrl Pts',(162.631285232503,-225.360388253327,2.59304513211926));
#76948=CARTESIAN_POINT('Ctrl Pts',(162.264887100028,-226.108806171146,2.54012584370867));
#76949=CARTESIAN_POINT('Ctrl Pts',(161.898488967552,-226.857224088965,2.48720655529807));
#76950=CARTESIAN_POINT('Ctrl Pts',(161.124439693843,-227.406070821191,2.43428726688747));
#76951=CARTESIAN_POINT('Ctrl Pts',(160.296944187805,-227.504194220605,2.38136797847687));
#76952=CARTESIAN_POINT('Ctrl Pts',(159.469448681766,-227.602317620019,2.32844869006627));
#76953=CARTESIAN_POINT('Ctrl Pts',(158.588506943398,-227.249717686621,2.27552940165568));
#76954=CARTESIAN_POINT('Ctrl Pts',(158.05723794367,-226.607743921706,2.22261011324508));
#76955=CARTESIAN_POINT('Ctrl Pts',(157.68904306018,-226.162825329247,2.18593450966071));
#76956=CARTESIAN_POINT('Ctrl Pts',(157.48880139235,-225.578916017294,2.14925890607634));
#76957=CARTESIAN_POINT('Ctrl Pts',(157.484174852024,-224.997885174718,2.11258330249197));
#76958=CARTESIAN_POINT('Ctrl Pts',(157.478659134318,-224.999094471329,2.38741669750801));
#76959=CARTESIAN_POINT('Ctrl Pts',(157.482292454888,-225.782645648265,2.43715607317295));
#76960=CARTESIAN_POINT('Ctrl Pts',(157.876385242744,-226.569350388705,2.48689544883789));
#76961=CARTESIAN_POINT('Ctrl Pts',(158.507754677526,-227.032823117687,2.53663482450284));
#76962=CARTESIAN_POINT('Ctrl Pts',(159.179488505429,-227.525926352046,2.58955411291343));
#76963=CARTESIAN_POINT('Ctrl Pts',(160.119807688463,-227.653147036598,2.64247340132403));
#76964=CARTESIAN_POINT('Ctrl Pts',(160.89842219588,-227.356268980265,2.69539268973463));
#76965=CARTESIAN_POINT('Ctrl Pts',(161.677036703297,-227.059390923932,2.74831197814522));
#76966=CARTESIAN_POINT('Ctrl Pts',(162.293946535097,-226.338414126714,2.80123126655582));
#76967=CARTESIAN_POINT('Ctrl Pts',(162.466853760079,-225.523257560855,2.85415055496642));
#76968=CARTESIAN_POINT('Ctrl Pts',(162.639760985062,-224.708100994996,2.90706984337702));
#76969=CARTESIAN_POINT('Ctrl Pts',(162.368665603227,-223.798764660497,2.95998913178761));
#76970=CARTESIAN_POINT('Ctrl Pts',(161.777620858044,-223.21136084421,3.01290842019821));
#76971=CARTESIAN_POINT('Ctrl Pts',(161.186576112861,-222.623957027924,3.06582770860881));
#76972=CARTESIAN_POINT('Ctrl Pts',(160.275582004329,-222.35848572985,3.1187469970194));
#76973=CARTESIAN_POINT('Ctrl Pts',(159.461509417602,-222.5364266117,3.17166628543));
#76974=CARTESIAN_POINT('Ctrl Pts',(158.647436830876,-222.71436749355,3.2245855738406));
#76975=CARTESIAN_POINT('Ctrl Pts',(157.930285765954,-223.335720555324,3.2775048622512));
#76976=CARTESIAN_POINT('Ctrl Pts',(157.638224536527,-224.116154647722,3.3304241506618));
#76977=CARTESIAN_POINT('Ctrl Pts',(157.533377363911,-224.39632298147,3.3494216662772));
#76978=CARTESIAN_POINT('Ctrl Pts',(157.483313259179,-224.696992739086,3.3684191818926));
#76979=CARTESIAN_POINT('Ctrl Pts',(157.485215918653,-224.99827376338,3.38741669750801));
#76980=CARTESIAN_POINT('Origin',(160.,-225.,10.));
#76981=CARTESIAN_POINT('',(157.484904423017,-225.001872886231,4.38741669750801));
#76982=CARTESIAN_POINT('',(157.47919603435,-225.001369558219,4.11258330249197));
#76983=CARTESIAN_POINT('',(157.4825,-225.,10.));
#76984=CARTESIAN_POINT('Ctrl Pts',(157.47919603435,-225.001369558219,4.11258330249197));
#76985=CARTESIAN_POINT('Ctrl Pts',(157.4841473595,-224.246701787719,4.06470441192625));
#76986=CARTESIAN_POINT('Ctrl Pts',(157.845660234688,-223.487919737563,4.01682552136052));
#76987=CARTESIAN_POINT('Ctrl Pts',(158.437397251925,-223.020748288856,3.9689466307948));
#76988=CARTESIAN_POINT('Ctrl Pts',(159.09142873654,-222.504395876775,3.9160273423842));
#76989=CARTESIAN_POINT('Ctrl Pts',(160.026709033785,-222.34428384278,3.8631080539736));
#76990=CARTESIAN_POINT('Ctrl Pts',(160.815253898065,-222.613679450329,3.810188765563));
#76991=CARTESIAN_POINT('Ctrl Pts',(161.603798762344,-222.883075057879,3.75726947715241));
#76992=CARTESIAN_POINT('Ctrl Pts',(162.245608193657,-223.581978306972,3.70435018874181));
#76993=CARTESIAN_POINT('Ctrl Pts',(162.446990208786,-224.390571084876,3.65143090033121));
#76994=CARTESIAN_POINT('Ctrl Pts',(162.648372223916,-225.199163862781,3.59851161192062));
#76995=CARTESIAN_POINT('Ctrl Pts',(162.40932682286,-226.117446169496,3.54559232351002));
#76996=CARTESIAN_POINT('Ctrl Pts',(161.839241176586,-226.725212038881,3.49267303509942));
#76997=CARTESIAN_POINT('Ctrl Pts',(161.269155530311,-227.332977908266,3.43975374668882));
#76998=CARTESIAN_POINT('Ctrl Pts',(160.368029638817,-227.630227340321,3.38683445827822));
#76999=CARTESIAN_POINT('Ctrl Pts',(159.548218692039,-227.480939002117,3.33391516986763));
#77000=CARTESIAN_POINT('Ctrl Pts',(158.72840774526,-227.331650663914,3.28099588145703));
#77001=CARTESIAN_POINT('Ctrl Pts',(157.989911743197,-226.735824555453,3.22807659304643));
#77002=CARTESIAN_POINT('Ctrl Pts',(157.670666442485,-225.966110689478,3.17515730463584));
#77003=CARTESIAN_POINT('Ctrl Pts',(157.544836732555,-225.662729959147,3.15429930392121));
#77004=CARTESIAN_POINT('Ctrl Pts',(157.484138534938,-225.332335385827,3.13344130320659));
#77005=CARTESIAN_POINT('Ctrl Pts',(157.485769737505,-225.001366316787,3.11258330249197));
#77006=CARTESIAN_POINT('Ctrl Pts',(157.485215918653,-224.99827376338,3.38741669750801));
#77007=CARTESIAN_POINT('Ctrl Pts',(157.488613288272,-225.536238129905,3.4213384703032));
#77008=CARTESIAN_POINT('Ctrl Pts',(157.657697925989,-226.076151417195,3.45526024309839));
#77009=CARTESIAN_POINT('Ctrl Pts',(157.976436466973,-226.504777915181,3.48918201589359));
#77010=CARTESIAN_POINT('Ctrl Pts',(158.473681020781,-227.173451967221,3.54210130430419));
#77011=CARTESIAN_POINT('Ctrl Pts',(159.335141522331,-227.57128494828,3.59502059271478));
#77012=CARTESIAN_POINT('Ctrl Pts',(160.166613663162,-227.516228493942,3.64793988112538));
#77013=CARTESIAN_POINT('Ctrl Pts',(160.998085803994,-227.461172039605,3.70085916953598));
#77014=CARTESIAN_POINT('Ctrl Pts',(161.799569584108,-226.953226149871,3.75377845794658));
#77015=CARTESIAN_POINT('Ctrl Pts',(162.20430604143,-226.224826853947,3.80669774635717));
#77016=CARTESIAN_POINT('Ctrl Pts',(162.609042498751,-225.496427558022,3.85961703476777));
#77017=CARTESIAN_POINT('Ctrl Pts',(162.617031633279,-224.547574855907,3.91253632317837));
#77018=CARTESIAN_POINT('Ctrl Pts',(162.224617617237,-223.812463725408,3.96545561158897));
#77019=CARTESIAN_POINT('Ctrl Pts',(161.832203601196,-223.077352594909,4.01837489999956));
#77020=CARTESIAN_POINT('Ctrl Pts',(161.039386434584,-222.555983036026,4.07129418841016));
#77021=CARTESIAN_POINT('Ctrl Pts',(160.208959237243,-222.486933748666,4.12421347682076));
#77022=CARTESIAN_POINT('Ctrl Pts',(159.378532039902,-222.417884461305,4.17713276523136));
#77023=CARTESIAN_POINT('Ctrl Pts',(158.510494811831,-222.801155445465,4.23005205364195));
#77024=CARTESIAN_POINT('Ctrl Pts',(158.002061371535,-223.461361906326,4.28297134205255));
#77025=CARTESIAN_POINT('Ctrl Pts',(157.667567635935,-223.895705731609,4.3177864605377));
#77026=CARTESIAN_POINT('Ctrl Pts',(157.488717770492,-224.44991289216,4.35260157902286));
#77027=CARTESIAN_POINT('Ctrl Pts',(157.484904423017,-225.001872886231,4.38741669750801));
#77028=CARTESIAN_POINT('Origin',(160.,-225.,10.));
#77029=CARTESIAN_POINT('',(157.478473497091,-225.000661269082,5.38741669750801));
#77030=CARTESIAN_POINT('',(157.481647327547,-224.997761948287,5.11258330249197));
#77031=CARTESIAN_POINT('',(157.4825,-225.,10.));
#77032=CARTESIAN_POINT('Ctrl Pts',(157.481647327547,-224.997761948287,5.11258330249197));
#77033=CARTESIAN_POINT('Ctrl Pts',(157.480078492543,-224.827461165568,5.1018060974671));
#77034=CARTESIAN_POINT('Ctrl Pts',(157.495878758897,-224.657449797744,5.09102889244222));
#77035=CARTESIAN_POINT('Ctrl Pts',(157.530116560791,-224.491236321052,5.08025168741734));
#77036=CARTESIAN_POINT('Ctrl Pts',(157.698234371372,-223.675078616854,5.02733239900675));
#77037=CARTESIAN_POINT('Ctrl Pts',(158.310900091203,-222.950491966653,4.97441311059615));
#77038=CARTESIAN_POINT('Ctrl Pts',(159.087757898936,-222.649047207334,4.92149382218555));
#77039=CARTESIAN_POINT('Ctrl Pts',(159.864615706669,-222.347602448016,4.86857453377496));
#77040=CARTESIAN_POINT('Ctrl Pts',(160.805665602304,-222.469299579581,4.81565524536436));
#77041=CARTESIAN_POINT('Ctrl Pts',(161.480283172102,-222.958449997016,4.76273595695376));
#77042=CARTESIAN_POINT('Ctrl Pts',(162.154900741899,-223.447600414451,4.70981666854316));
#77043=CARTESIAN_POINT('Ctrl Pts',(162.563085985859,-224.304204117755,4.65689738013256));
#77044=CARTESIAN_POINT('Ctrl Pts',(162.518053344371,-225.136279269145,4.60397809172197));
#77045=CARTESIAN_POINT('Ctrl Pts',(162.473020702882,-225.968354420534,4.55105880331137));
#77046=CARTESIAN_POINT('Ctrl Pts',(161.974770175945,-226.775901020007,4.49813951490078));
#77047=CARTESIAN_POINT('Ctrl Pts',(161.251301194891,-227.189385759515,4.44522022649018));
#77048=CARTESIAN_POINT('Ctrl Pts',(160.527832213837,-227.602870499024,4.39230093807958));
#77049=CARTESIAN_POINT('Ctrl Pts',(159.579144778666,-227.622293378567,4.33938164966898));
#77050=CARTESIAN_POINT('Ctrl Pts',(158.839358241055,-227.238766488865,4.28646236125838));
#77051=CARTESIAN_POINT('Ctrl Pts',(158.099571703444,-226.855239599163,4.23354307284778));
#77052=CARTESIAN_POINT('Ctrl Pts',(157.568686063394,-226.068762940216,4.18062378443719));
#77053=CARTESIAN_POINT('Ctrl Pts',(157.489634579361,-225.239228215659,4.12770449602659));
#77054=CARTESIAN_POINT('Ctrl Pts',(157.482105171054,-225.16021760982,4.12266409818172));
#77055=CARTESIAN_POINT('Ctrl Pts',(157.47867478901,-225.080816382468,4.11762370033685));
#77056=CARTESIAN_POINT('Ctrl Pts',(157.47919603435,-225.001369558219,4.11258330249197));
#77057=CARTESIAN_POINT('Ctrl Pts',(157.484904423017,-225.001872886231,4.38741669750801));
#77058=CARTESIAN_POINT('Ctrl Pts',(157.482921448559,-225.288896971155,4.40552086743346));
#77059=CARTESIAN_POINT('Ctrl Pts',(157.528269960652,-225.575313401567,4.4236250373589));
#77060=CARTESIAN_POINT('Ctrl Pts',(157.623676860034,-225.843951586809,4.44172920728434));
#77061=CARTESIAN_POINT('Ctrl Pts',(157.902555441351,-226.629192868871,4.49464849569494));
#77062=CARTESIAN_POINT('Ctrl Pts',(158.609142256508,-227.262533495433,4.54756778410554));
#77063=CARTESIAN_POINT('Ctrl Pts',(159.420103192782,-227.454156808233,4.60048707251614));
#77064=CARTESIAN_POINT('Ctrl Pts',(160.231064129057,-227.645780121033,4.65340636092673));
#77065=CARTESIAN_POINT('Ctrl Pts',(161.146399186449,-227.395686120071,4.70632564933733));
#77066=CARTESIAN_POINT('Ctrl Pts',(161.747251060693,-226.818317815269,4.75924493774793));
#77067=CARTESIAN_POINT('Ctrl Pts',(162.348102934937,-226.240949510468,4.81216422615853));
#77068=CARTESIAN_POINT('Ctrl Pts',(162.634471626033,-225.336306901827,4.86508351456912));
#77069=CARTESIAN_POINT('Ctrl Pts',(162.475314826566,-224.518354429275,4.91800280297972));
#77070=CARTESIAN_POINT('Ctrl Pts',(162.316158027099,-223.700401956722,4.97092209139032));
#77071=CARTESIAN_POINT('Ctrl Pts',(161.71147573707,-222.969139620257,5.02384137980092));
#77072=CARTESIAN_POINT('Ctrl Pts',(160.937970560506,-222.659193050668,5.07676066821151));
#77073=CARTESIAN_POINT('Ctrl Pts',(160.164465383941,-222.349246481079,5.12967995662211));
#77074=CARTESIAN_POINT('Ctrl Pts',(159.222137320843,-222.460615678366,5.18259924503271));
#77075=CARTESIAN_POINT('Ctrl Pts',(158.542195674355,-222.94233810004,5.23551853344331));
#77076=CARTESIAN_POINT('Ctrl Pts',(157.891633337668,-223.403245982205,5.28615125479821));
#77077=CARTESIAN_POINT('Ctrl Pts',(157.481272601586,-224.203193660849,5.33678397615311));
#77078=CARTESIAN_POINT('Ctrl Pts',(157.478473497091,-225.000661269082,5.38741669750801));
#77079=CARTESIAN_POINT('Origin',(160.,-225.,10.));
#77080=CARTESIAN_POINT('',(157.482962712505,-224.997707731329,6.38741669750801));
#77081=CARTESIAN_POINT('',(157.48651745684,-225.000035219866,6.11258330249197));
#77082=CARTESIAN_POINT('',(157.4825,-225.,10.));
#77083=CARTESIAN_POINT('Ctrl Pts',(157.48651745684,-225.000035219866,6.11258330249197));
#77084=CARTESIAN_POINT('Ctrl Pts',(157.486570157899,-224.577722240852,6.08598849459735));
#77085=CARTESIAN_POINT('Ctrl Pts',(157.587291233443,-224.155385642676,6.05939368670272));
#77086=CARTESIAN_POINT('Ctrl Pts',(157.788540269793,-223.788137571352,6.0327988788081));
#77087=CARTESIAN_POINT('Ctrl Pts',(158.18899271296,-223.057374383227,5.9798795903975));
#77088=CARTESIAN_POINT('Ctrl Pts',(158.987480052774,-222.544731168055,5.92696030198691));
#77089=CARTESIAN_POINT('Ctrl Pts',(159.818614498236,-222.484793451018,5.87404101357631));
#77090=CARTESIAN_POINT('Ctrl Pts',(160.649748943698,-222.42485573398,5.82112172516571));
#77091=CARTESIAN_POINT('Ctrl Pts',(161.513530494807,-222.817623515078,5.76820243675511));
#77092=CARTESIAN_POINT('Ctrl Pts',(162.01469273076,-223.483366265404,5.71528314834452));
#77093=CARTESIAN_POINT('Ctrl Pts',(162.515854966714,-224.149109015729,5.66236385993392));
#77094=CARTESIAN_POINT('Ctrl Pts',(162.654397887511,-225.087826735282,5.60944457152332));
#77095=CARTESIAN_POINT('Ctrl Pts',(162.366924255319,-225.869962214052,5.55652528311273));
#77096=CARTESIAN_POINT('Ctrl Pts',(162.079450623127,-226.652097692822,5.50360599470213));
#77097=CARTESIAN_POINT('Ctrl Pts',(161.365960437946,-227.27765093081,5.45068670629153));
#77098=CARTESIAN_POINT('Ctrl Pts',(160.552946794486,-227.460368778611,5.39776741788093));
#77099=CARTESIAN_POINT('Ctrl Pts',(159.739933151027,-227.643086626412,5.34484812947033));
#77100=CARTESIAN_POINT('Ctrl Pts',(158.827396049288,-227.382969084027,5.29192884105974));
#77101=CARTESIAN_POINT('Ctrl Pts',(158.232912449084,-226.799045933736,5.23900955264914));
#77102=CARTESIAN_POINT('Ctrl Pts',(157.759497590274,-226.334040850912,5.19686746926341));
#77103=CARTESIAN_POINT('Ctrl Pts',(157.487781939944,-225.663688760426,5.15472538587769));
#77104=CARTESIAN_POINT('Ctrl Pts',(157.481647327547,-224.997761948287,5.11258330249197));
#77105=CARTESIAN_POINT('Ctrl Pts',(157.478473497091,-225.000661269082,5.38741669750801));
#77106=CARTESIAN_POINT('Ctrl Pts',(157.478347089899,-225.036674801679,5.38970326456371));
#77107=CARTESIAN_POINT('Ctrl Pts',(157.479051869504,-225.072683276385,5.3919898316194));
#77108=CARTESIAN_POINT('Ctrl Pts',(157.480603249708,-225.10865523934,5.3942763986751));
#77109=CARTESIAN_POINT('Ctrl Pts',(157.516507701425,-225.941174310904,5.4471956870857));
#77110=CARTESIAN_POINT('Ctrl Pts',(158.005871834734,-226.754136807972,5.50011497549629));
#77111=CARTESIAN_POINT('Ctrl Pts',(158.724762631855,-227.175531107869,5.55303426390689));
#77112=CARTESIAN_POINT('Ctrl Pts',(159.443653428977,-227.596925407766,5.60595355231749));
#77113=CARTESIAN_POINT('Ctrl Pts',(160.392070889911,-227.626751510492,5.65887284072808));
#77114=CARTESIAN_POINT('Ctrl Pts',(161.136019203181,-227.251360992027,5.71179212913868));
#77115=CARTESIAN_POINT('Ctrl Pts',(161.879967516452,-226.875970473562,5.76471141754928));
#77116=CARTESIAN_POINT('Ctrl Pts',(162.419446682059,-226.095363333905,5.81763070595988));
#77117=CARTESIAN_POINT('Ctrl Pts',(162.507591044428,-225.266745384815,5.87054999437047));
#77118=CARTESIAN_POINT('Ctrl Pts',(162.595735406798,-224.438127435725,5.92346928278107));
#77119=CARTESIAN_POINT('Ctrl Pts',(162.232544965929,-223.561498677202,5.97638857119167));
#77120=CARTESIAN_POINT('Ctrl Pts',(161.584215660423,-223.03800441191,6.02930785960226));
#77121=CARTESIAN_POINT('Ctrl Pts',(160.935886354917,-222.514510146617,6.08222714801286));
#77122=CARTESIAN_POINT('Ctrl Pts',(160.002418184774,-222.344150374556,6.13514643642346));
#77123=CARTESIAN_POINT('Ctrl Pts',(159.210966166297,-222.604881724071,6.18806572483406));
#77124=CARTESIAN_POINT('Ctrl Pts',(158.419514147819,-222.865613073586,6.24098501324466));
#77125=CARTESIAN_POINT('Ctrl Pts',(157.770078281009,-223.557435544678,6.29390430165525));
#77126=CARTESIAN_POINT('Ctrl Pts',(157.559840405747,-224.363771188177,6.34682359006585));
#77127=CARTESIAN_POINT('Ctrl Pts',(157.506084274381,-224.569944717679,6.36035462587991));
#77128=CARTESIAN_POINT('Ctrl Pts',(157.48104219227,-224.783604931856,6.37388566169396));
#77129=CARTESIAN_POINT('Ctrl Pts',(157.482962712505,-224.997707731329,6.38741669750801));
#77130=CARTESIAN_POINT('Origin',(160.,-225.,10.));
#77131=CARTESIAN_POINT('',(157.486314949328,-225.000739875386,7.38741669750801));
#77132=CARTESIAN_POINT('',(157.481518068703,-225.002219574922,7.11258330249198));
#77133=CARTESIAN_POINT('',(157.4825,-225.,10.));
#77134=CARTESIAN_POINT('Ctrl Pts',(157.481518068703,-225.002219574922,7.11258330249198));
#77135=CARTESIAN_POINT('Ctrl Pts',(157.487674948651,-224.33210956248,7.0701708917276));
#77136=CARTESIAN_POINT('Ctrl Pts',(157.763272363098,-223.657527262373,7.02775848096323));
#77137=CARTESIAN_POINT('Ctrl Pts',(158.242102480641,-223.191973176159,6.98534607019885));
#77138=CARTESIAN_POINT('Ctrl Pts',(158.839553760426,-222.611086814949,6.93242678178826));
#77139=CARTESIAN_POINT('Ctrl Pts',(159.753404451819,-222.355622508743,6.87950749337766));
#77140=CARTESIAN_POINT('Ctrl Pts',(160.565476496408,-222.542480719037,6.82658820496706));
#77141=CARTESIAN_POINT('Ctrl Pts',(161.377548540996,-222.729338929331,6.77366891655647));
#77142=CARTESIAN_POINT('Ctrl Pts',(162.08784193878,-223.358519656126,6.72074962814587));
#77143=CARTESIAN_POINT('Ctrl Pts',(162.371326444899,-224.142109811212,6.66783033973527));
#77144=CARTESIAN_POINT('Ctrl Pts',(162.654810951018,-224.925699966298,6.61491105132467));
#77145=CARTESIAN_POINT('Ctrl Pts',(162.511486565472,-225.863699549674,6.56199176291407));
#77146=CARTESIAN_POINT('Ctrl Pts',(162.006938524269,-226.52687997043,6.50907247450348));
#77147=CARTESIAN_POINT('Ctrl Pts',(161.502390483066,-227.190060391187,6.45615318609288));
#77148=CARTESIAN_POINT('Ctrl Pts',(160.636618786206,-227.578421649324,6.40323389768228));
#77149=CARTESIAN_POINT('Ctrl Pts',(159.805800545149,-227.514249640754,6.35031460927169));
#77150=CARTESIAN_POINT('Ctrl Pts',(158.974982304092,-227.450077632184,6.29739532086109));
#77151=CARTESIAN_POINT('Ctrl Pts',(158.179117518839,-226.933372356907,6.24447603245049));
#77152=CARTESIAN_POINT('Ctrl Pts',(157.782393899472,-226.20057813873,6.19155674403989));
#77153=CARTESIAN_POINT('Ctrl Pts',(157.585045380588,-225.836052694455,6.16523226352392));
#77154=CARTESIAN_POINT('Ctrl Pts',(157.486465291471,-225.41805552788,6.13890778300795));
#77155=CARTESIAN_POINT('Ctrl Pts',(157.48651745684,-225.000035219866,6.11258330249197));
#77156=CARTESIAN_POINT('Ctrl Pts',(157.482962712505,-224.997707731329,6.38741669750801));
#77157=CARTESIAN_POINT('Ctrl Pts',(157.488553262792,-225.62095160291,6.42680495010456));
#77158=CARTESIAN_POINT('Ctrl Pts',(157.722615899816,-226.247945794455,6.4661932027011));
#77159=CARTESIAN_POINT('Ctrl Pts',(158.141948609901,-226.704937235844,6.50558145529765));
#77160=CARTESIAN_POINT('Ctrl Pts',(158.705334573027,-227.318918824106,6.55850074370824));
#77161=CARTESIAN_POINT('Ctrl Pts',(159.603146382992,-227.626033184721,6.61142003211884));
#77162=CARTESIAN_POINT('Ctrl Pts',(160.424545373207,-227.485744792312,6.66433932052944));
#77163=CARTESIAN_POINT('Ctrl Pts',(161.245944363423,-227.345456399903,6.71725860894004));
#77164=CARTESIAN_POINT('Ctrl Pts',(161.990930533889,-226.757765254469,6.77017789735064));
#77165=CARTESIAN_POINT('Ctrl Pts',(162.318598227649,-225.991598812605,6.82309718576123));
#77166=CARTESIAN_POINT('Ctrl Pts',(162.646265921409,-225.225432370742,6.87601647417183));
#77167=CARTESIAN_POINT('Ctrl Pts',(162.556615138462,-224.280790632449,6.92893576258242));
#77168=CARTESIAN_POINT('Ctrl Pts',(162.090670075323,-223.589941638596,6.98185505099302));
#77169=CARTESIAN_POINT('Ctrl Pts',(161.624725012184,-222.899092644743,7.03477433940362));
#77170=CARTESIAN_POINT('Ctrl Pts',(160.782485668852,-222.46203639533,7.08769362781422));
#77171=CARTESIAN_POINT('Ctrl Pts',(159.949360752275,-222.478769821494,7.14061291622481));
#77172=CARTESIAN_POINT('Ctrl Pts',(159.116235835699,-222.495503247659,7.19353220463541));
#77173=CARTESIAN_POINT('Ctrl Pts',(158.292225345878,-222.966026349402,7.24645149304601));
#77174=CARTESIAN_POINT('Ctrl Pts',(157.854396466754,-223.675027764616,7.29937078145661));
#77175=CARTESIAN_POINT('Ctrl Pts',(157.611579868785,-224.068234608215,7.32871942014041));
#77176=CARTESIAN_POINT('Ctrl Pts',(157.487542231623,-224.534790895352,7.35806805882421));
#77177=CARTESIAN_POINT('Ctrl Pts',(157.486314949328,-225.000739875386,7.38741669750801));
#77178=CARTESIAN_POINT('Origin',(160.,-225.,10.));
#77179=CARTESIAN_POINT('',(157.480251899882,-225.00189995361,8.38741669750802));
#77180=CARTESIAN_POINT('',(157.479288544104,-224.998569117391,8.11258330249198));
#77181=CARTESIAN_POINT('',(157.4825,-225.,10.));
#77182=CARTESIAN_POINT('Ctrl Pts',(157.479288544104,-224.998569117391,8.11258330249198));
#77183=CARTESIAN_POINT('Ctrl Pts',(157.478719757445,-224.914853296399,8.10727257726845));
#77184=CARTESIAN_POINT('Ctrl Pts',(157.482528847107,-224.831189860152,8.10196185204493));
#77185=CARTESIAN_POINT('Ctrl Pts',(157.490886163968,-224.747983250304,8.0966511268214));
#77186=CARTESIAN_POINT('Ctrl Pts',(157.574163539971,-223.918862104148,8.04373183841081));
#77187=CARTESIAN_POINT('Ctrl Pts',(158.109049802521,-223.135100798621,7.99081255000021));
#77188=CARTESIAN_POINT('Ctrl Pts',(158.850781008391,-222.755348491721,7.93789326158961));
#77189=CARTESIAN_POINT('Ctrl Pts',(159.59251221426,-222.375596184821,7.88497397317902));
#77190=CARTESIAN_POINT('Ctrl Pts',(160.54108836345,-222.399852876549,7.83205468476842));
#77191=CARTESIAN_POINT('Ctrl Pts',(161.262441028742,-222.817018705246,7.77913539635782));
#77192=CARTESIAN_POINT('Ctrl Pts',(161.983793694034,-223.234184533944,7.72621610794722));
#77193=CARTESIAN_POINT('Ctrl Pts',(162.477922875428,-224.044259499611,7.67329681953662));
#77194=CARTESIAN_POINT('Ctrl Pts',(162.518715069233,-224.876553313887,7.62037753112602));
#77195=CARTESIAN_POINT('Ctrl Pts',(162.559507263039,-225.708847128162,7.56745824271543));
#77196=CARTESIAN_POINT('Ctrl Pts',(162.146962469256,-226.563359791046,7.51453895430483));
#77197=CARTESIAN_POINT('Ctrl Pts',(161.469861177408,-227.049066324803,7.46161966589423));
#77198=CARTESIAN_POINT('Ctrl Pts',(160.79275988556,-227.534772858561,7.40870037748364));
#77199=CARTESIAN_POINT('Ctrl Pts',(159.851102095648,-227.651673263193,7.35578108907304));
#77200=CARTESIAN_POINT('Ctrl Pts',(159.07579039382,-227.346273915838,7.30286180066244));
#77201=CARTESIAN_POINT('Ctrl Pts',(158.300478691992,-227.040874568482,7.24994251225184));
#77202=CARTESIAN_POINT('Ctrl Pts',(157.691513078248,-226.31317546914,7.19702322384125));
#77203=CARTESIAN_POINT('Ctrl Pts',(157.527556205464,-225.496171711362,7.14410393543065));
#77204=CARTESIAN_POINT('Ctrl Pts',(157.495003333849,-225.333959429654,7.13359705778443));
#77205=CARTESIAN_POINT('Ctrl Pts',(157.479992817412,-225.168226736112,7.1230901801382));
#77206=CARTESIAN_POINT('Ctrl Pts',(157.481518068703,-225.002219574922,7.11258330249198));
#77207=CARTESIAN_POINT('Ctrl Pts',(157.486314949328,-225.000739875386,7.38741669750801));
#77208=CARTESIAN_POINT('Ctrl Pts',(157.48532928722,-225.374955535516,7.41098734723481));
#77209=CARTESIAN_POINT('Ctrl Pts',(157.563557666543,-225.748779475827,7.4345579969616));
#77210=CARTESIAN_POINT('Ctrl Pts',(157.723088450485,-226.083900245458,7.4581286466884));
#77211=CARTESIAN_POINT('Ctrl Pts',(158.08125658177,-226.836291582399,7.511047935099));
#77212=CARTESIAN_POINT('Ctrl Pts',(158.849240112769,-227.393594527594,7.5639672235096));
#77213=CARTESIAN_POINT('Ctrl Pts',(159.675609794796,-227.50078726428,7.6168865119202));
#77214=CARTESIAN_POINT('Ctrl Pts',(160.501979476823,-227.607980000966,7.66980580033079));
#77215=CARTESIAN_POINT('Ctrl Pts',(161.386735309878,-227.265062529142,7.72272508874138));
#77216=CARTESIAN_POINT('Ctrl Pts',(161.925013042153,-226.628953877174,7.77564437715198));
#77217=CARTESIAN_POINT('Ctrl Pts',(162.463290774427,-225.992845225205,7.82856366556258));
#77218=CARTESIAN_POINT('Ctrl Pts',(162.655090405919,-225.063545393091,7.88148295397318));
#77219=CARTESIAN_POINT('Ctrl Pts',(162.412644429031,-224.266301965735,7.93440224238378));
#77220=CARTESIAN_POINT('Ctrl Pts',(162.170198452142,-223.46905853838,7.98732153079438));
#77221=CARTESIAN_POINT('Ctrl Pts',(161.493506866872,-222.803871515782,8.04024081920497));
#77222=CARTESIAN_POINT('Ctrl Pts',(160.692223729335,-222.575130466404,8.09316010761557));
#77223=CARTESIAN_POINT('Ctrl Pts',(159.890940591798,-222.346389417026,8.14607939602616));
#77224=CARTESIAN_POINT('Ctrl Pts',(158.965065901994,-222.554094340868,8.19899868443676));
#77225=CARTESIAN_POINT('Ctrl Pts',(158.338279899773,-223.103199468864,8.25191797284736));
#77226=CARTESIAN_POINT('Ctrl Pts',(157.803322442313,-223.571856844922,8.29708421440091));
#77227=CARTESIAN_POINT('Ctrl Pts',(157.486236222901,-224.289207295096,8.34225045595446));
#77228=CARTESIAN_POINT('Ctrl Pts',(157.480251899882,-225.00189995361,8.38741669750802));
#77229=CARTESIAN_POINT('Origin',(160.,-225.,10.));
#77230=CARTESIAN_POINT('',(157.480388086678,-224.998052208457,9.38741669750802));
#77231=CARTESIAN_POINT('',(157.485838591434,-224.998691358362,9.11258330249198));
#77232=CARTESIAN_POINT('',(157.4825,-225.,10.));
#77233=CARTESIAN_POINT('Ctrl Pts',(157.485838591434,-224.998691358362,9.11258330249198));
#77234=CARTESIAN_POINT('Ctrl Pts',(157.484258577989,-224.663409819317,9.0914549743987));
#77235=CARTESIAN_POINT('Ctrl Pts',(157.54659475251,-224.328691854693,9.07032664630543));
#77236=CARTESIAN_POINT('Ctrl Pts',(157.675619527759,-224.022032666926,9.04919831821216));
#77237=CARTESIAN_POINT('Ctrl Pts',(157.99878278343,-223.253955518105,8.99627902980156));
#77238=CARTESIAN_POINT('Ctrl Pts',(158.740305247003,-222.661900171095,8.94335974139096));
#77239=CARTESIAN_POINT('Ctrl Pts',(159.560866253727,-222.516791141048,8.89044045298036));
#77240=CARTESIAN_POINT('Ctrl Pts',(160.38142726045,-222.371682111,8.83752116456977));
#77241=CARTESIAN_POINT('Ctrl Pts',(161.281026810325,-222.673519397914,8.78460187615917));
#77242=CARTESIAN_POINT('Ctrl Pts',(161.848008167015,-223.284182265233,8.73168258774857));
#77243=CARTESIAN_POINT('Ctrl Pts',(162.414989523706,-223.894845132552,8.67876329933798));
#77244=CARTESIAN_POINT('Ctrl Pts',(162.649352687212,-224.814333580276,8.62584401092738));
#77245=CARTESIAN_POINT('Ctrl Pts',(162.443853078522,-225.621889712804,8.57292472251678));
#77246=CARTESIAN_POINT('Ctrl Pts',(162.238353469833,-226.429445845333,8.52000543410618));
#77247=CARTESIAN_POINT('Ctrl Pts',(161.592991088946,-227.125069662667,8.46708614569559));
#77248=CARTESIAN_POINT('Ctrl Pts',(160.803083748668,-227.390443719672,8.41416685728499));
#77249=CARTESIAN_POINT('Ctrl Pts',(160.01317640839,-227.655817776677,8.36124756887439));
#77250=CARTESIAN_POINT('Ctrl Pts',(159.07872410872,-227.490942073352,8.30832828046379));
#77251=CARTESIAN_POINT('Ctrl Pts',(158.427332203613,-226.971263728298,8.25540899205319));
#77252=CARTESIAN_POINT('Ctrl Pts',(157.841310856667,-226.503737802108,8.20780042886612));
#77253=CARTESIAN_POINT('Ctrl Pts',(157.484387492819,-225.749048531349,8.16019186567905));
#77254=CARTESIAN_POINT('Ctrl Pts',(157.479288544104,-224.998569117391,8.11258330249198));
#77255=CARTESIAN_POINT('Ctrl Pts',(157.480251899882,-225.00189995361,8.38741669750802));
#77256=CARTESIAN_POINT('Ctrl Pts',(157.479224656189,-225.124237774648,8.39516974436506));
#77257=CARTESIAN_POINT('Ctrl Pts',(157.487364250787,-225.246438350547,8.40292279122211));
#77258=CARTESIAN_POINT('Ctrl Pts',(157.505142240593,-225.36722024283,8.41067583807915));
#77259=CARTESIAN_POINT('Ctrl Pts',(157.626487898273,-226.19163055665,8.46359512648975));
#77260=CARTESIAN_POINT('Ctrl Pts',(158.196876528271,-226.949945852142,8.51651441490035));
#77261=CARTESIAN_POINT('Ctrl Pts',(158.955298304715,-227.295161064999,8.56943370331095));
#77262=CARTESIAN_POINT('Ctrl Pts',(159.713720081158,-227.640376277855,8.62235299172154));
#77263=CARTESIAN_POINT('Ctrl Pts',(160.660175004048,-227.572491408075,8.67527228013214));
#77264=CARTESIAN_POINT('Ctrl Pts',(161.361565319279,-227.122570570736,8.72819156854274));
#77265=CARTESIAN_POINT('Ctrl Pts',(162.06295563451,-226.672649733396,8.78111085695333));
#77266=CARTESIAN_POINT('Ctrl Pts',(162.519281342082,-225.840692928498,8.83403014536393));
#77267=CARTESIAN_POINT('Ctrl Pts',(162.521727807182,-225.007403573603,8.88694943377453));
#77268=CARTESIAN_POINT('Ctrl Pts',(162.524174272282,-224.174114218709,8.93986872218513));
#77269=CARTESIAN_POINT('Ctrl Pts',(162.07274149491,-223.339492313819,8.99278801059573));
#77270=CARTESIAN_POINT('Ctrl Pts',(161.374005105116,-222.885460826201,9.04570729900632));
#77271=CARTESIAN_POINT('Ctrl Pts',(160.675268715322,-222.431429338582,9.09862658741692));
#77272=CARTESIAN_POINT('Ctrl Pts',(159.729228713105,-222.357988268235,9.15154587582752));
#77273=CARTESIAN_POINT('Ctrl Pts',(158.968792984879,-222.698744247507,9.20446516423812));
#77274=CARTESIAN_POINT('Ctrl Pts',(158.208357256654,-223.039500226778,9.25738445264872));
#77275=CARTESIAN_POINT('Ctrl Pts',(157.633525802418,-223.794453255668,9.31030374105931));
#77276=CARTESIAN_POINT('Ctrl Pts',(157.50734148433,-224.618136843,9.36322302946991));
#77277=CARTESIAN_POINT('Ctrl Pts',(157.488111813416,-224.743660874526,9.37128758548261));
#77278=CARTESIAN_POINT('Ctrl Pts',(157.479301425492,-224.870781089513,9.37935214149532));
#77279=CARTESIAN_POINT('Ctrl Pts',(157.480388086678,-224.998052208457,9.38741669750802));
#77280=CARTESIAN_POINT('Origin',(160.,-225.,10.));
#77281=CARTESIAN_POINT('',(157.486356088001,-224.999337553498,10.387416697508));
#77282=CARTESIAN_POINT('',(157.484060830038,-225.002142062077,10.112583302492));
#77283=CARTESIAN_POINT('',(157.4825,-225.,10.));
#77284=CARTESIAN_POINT('Ctrl Pts',(157.484060830038,-225.002142062077,10.112583302492));
#77285=CARTESIAN_POINT('Ctrl Pts',(157.488797243823,-224.416895654818,10.075637371529));
#77286=CARTESIAN_POINT('Ctrl Pts',(157.692267720596,-223.828679753063,10.0386914405659));
#77287=CARTESIAN_POINT('Ctrl Pts',(158.065455483688,-223.38237760936,10.0017455096029));
#77288=CARTESIAN_POINT('Ctrl Pts',(158.599988796332,-222.743119340715,9.94882622119231));
#77289=CARTESIAN_POINT('Ctrl Pts',(159.482715755051,-222.395012727367,9.89590693278172));
#77290=CARTESIAN_POINT('Ctrl Pts',(160.309700520891,-222.49735134874,9.84298764437112));
#77291=CARTESIAN_POINT('Ctrl Pts',(161.136685286731,-222.599689970112,9.79006835596052));
#77292=CARTESIAN_POINT('Ctrl Pts',(161.907927859693,-223.152473826205,9.73714906754993));
#77293=CARTESIAN_POINT('Ctrl Pts',(162.270507653554,-223.902749035339,9.68422977913933));
#77294=CARTESIAN_POINT('Ctrl Pts',(162.633087447414,-224.653024244473,9.63131049072873));
#77295=CARTESIAN_POINT('Ctrl Pts',(162.587004462172,-225.600790806648,9.57839120231814));
#77296=CARTESIAN_POINT('Ctrl Pts',(162.153346270969,-226.312350761648,9.52547191390754));
#77297=CARTESIAN_POINT('Ctrl Pts',(161.719688079767,-227.023910716647,9.47255262549694));
#77298=CARTESIAN_POINT('Ctrl Pts',(160.898454682603,-227.499264064472,9.41963333708634));
#77299=CARTESIAN_POINT('Ctrl Pts',(160.065442465872,-227.520889122503,9.36671404867574));
#77300=CARTESIAN_POINT('Ctrl Pts',(159.232430249142,-227.542514180535,9.31379476026514));
#77301=CARTESIAN_POINT('Ctrl Pts',(158.387639212846,-227.110410948773,9.26087547185455));
#77302=CARTESIAN_POINT('Ctrl Pts',(157.917645718582,-226.422309857576,9.20795618344395));
#77303=CARTESIAN_POINT('Ctrl Pts',(157.635299810799,-226.008937056437,9.17616522312663));
#77304=CARTESIAN_POINT('Ctrl Pts',(157.488215975226,-225.503176240263,9.1443742628093));
#77305=CARTESIAN_POINT('Ctrl Pts',(157.485838591434,-224.998691358362,9.11258330249198));
#77306=CARTESIAN_POINT('Ctrl Pts',(157.480388086678,-224.998052208457,9.38741669750802));
#77307=CARTESIAN_POINT('Ctrl Pts',(157.486432051983,-225.705928993396,9.43227142990591));
#77308=CARTESIAN_POINT('Ctrl Pts',(157.798645104925,-226.418474051318,9.47712616230381));
#77309=CARTESIAN_POINT('Ctrl Pts',(158.3271709593,-226.887010584763,9.5219808947017));
#77310=CARTESIAN_POINT('Ctrl Pts',(158.950721934301,-227.43978659342,9.5749001831123));
#77311=CARTESIAN_POINT('Ctrl Pts',(159.875361066246,-227.65292446496,9.62781947152289));
#77312=CARTESIAN_POINT('Ctrl Pts',(160.677973506536,-227.428892313556,9.68073875993349));
#77313=CARTESIAN_POINT('Ctrl Pts',(161.480585946827,-227.204860162152,9.73365804834408));
#77314=CARTESIAN_POINT('Ctrl Pts',(162.161171695463,-226.543657987806,9.78657733675469));
#77315=CARTESIAN_POINT('Ctrl Pts',(162.408294727251,-225.747851892496,9.83949662516529));
#77316=CARTESIAN_POINT('Ctrl Pts',(162.655417759039,-224.952045797187,9.89241591357588));
#77317=CARTESIAN_POINT('Ctrl Pts',(162.469078073979,-224.021635780915,9.94533520198648));
#77318=CARTESIAN_POINT('Ctrl Pts',(161.93454470829,-223.382377448833,9.99825449039708));
#77319=CARTESIAN_POINT('Ctrl Pts',(161.400011342601,-222.74311911675,10.0511737788077));
#77320=CARTESIAN_POINT('Ctrl Pts',(160.517284296283,-222.395012468857,10.1040930672183));
#77321=CARTESIAN_POINT('Ctrl Pts',(159.690299448375,-222.497351100386,10.1570123556289));
#77322=CARTESIAN_POINT('Ctrl Pts',(158.863314600468,-222.599689731914,10.2099316440395));
#77323=CARTESIAN_POINT('Ctrl Pts',(158.092071950971,-223.152473642863,10.2628509324501));
#77324=CARTESIAN_POINT('Ctrl Pts',(157.729492121129,-223.902748926452,10.3157702208607));
#77325=CARTESIAN_POINT('Ctrl Pts',(157.56586200886,-224.241343682096,10.3396523797431));
#77326=CARTESIAN_POINT('Ctrl Pts',(157.485462741294,-224.620160775021,10.3635345386256));
#77327=CARTESIAN_POINT('Ctrl Pts',(157.486356088001,-224.999337553498,10.387416697508));
#77328=CARTESIAN_POINT('Origin',(160.,-225.,10.));
#77329=CARTESIAN_POINT('',(157.482816074282,-225.002298292055,11.387416697508));
#77330=CARTESIAN_POINT('',(157.478262227161,-225.000045821962,11.112583302492));
#77331=CARTESIAN_POINT('',(157.4825,-225.,10.));
#77332=CARTESIAN_POINT('Ctrl Pts',(157.47826263161,-225.000045817589,11.112583302492));
#77333=CARTESIAN_POINT('Ctrl Pts',(157.478485477297,-224.16920459997,11.0598197686592));
#77334=CARTESIAN_POINT('Ctrl Pts',(157.929315264901,-223.338156151569,11.0070562348264));
#77335=CARTESIAN_POINT('Ctrl Pts',(158.625995031235,-222.88546103604,10.9542927009937));
#77336=CARTESIAN_POINT('Ctrl Pts',(159.324731351689,-222.431429593478,10.9013734125831));
#77337=CARTESIAN_POINT('Ctrl Pts',(160.270771260024,-222.357988530419,10.8484541241725));
#77338=CARTESIAN_POINT('Ctrl Pts',(161.031206912787,-222.698744475875,10.7955348357619));
#77339=CARTESIAN_POINT('Ctrl Pts',(161.79164256555,-223.039500421331,10.7426155473513));
#77340=CARTESIAN_POINT('Ctrl Pts',(162.366473962741,-223.794453375302,10.6896962589407));
#77341=CARTESIAN_POINT('Ctrl Pts',(162.492658268308,-224.618136880895,10.6367769705301));
#77342=CARTESIAN_POINT('Ctrl Pts',(162.618842573874,-225.441820386487,10.5838576821195));
#77343=CARTESIAN_POINT('Ctrl Pts',(162.296379787816,-226.334234443702,10.5309383937089));
#77344=CARTESIAN_POINT('Ctrl Pts',(161.672828874694,-226.887010397503,10.4780191052983));
#77345=CARTESIAN_POINT('Ctrl Pts',(161.049277961572,-227.439786351304,10.4250998168877));
#77346=CARTESIAN_POINT('Ctrl Pts',(160.124638921385,-227.652924201693,10.3721805284771));
#77347=CARTESIAN_POINT('Ctrl Pts',(159.322026560743,-227.428892072521,10.3192612400665));
#77348=CARTESIAN_POINT('Ctrl Pts',(158.519414200101,-227.20485994335,10.2663419516559));
#77349=CARTESIAN_POINT('Ctrl Pts',(157.838828519004,-226.543657834619,10.2134226632453));
#77350=CARTESIAN_POINT('Ctrl Pts',(157.591705511739,-225.747851818282,10.1605033748347));
#77351=CARTESIAN_POINT('Ctrl Pts',(157.517112971909,-225.507642731205,10.1445300173871));
#77352=CARTESIAN_POINT('Ctrl Pts',(157.482013069203,-225.255169927782,10.1285566599396));
#77353=CARTESIAN_POINT('Ctrl Pts',(157.484060830038,-225.002142062077,10.112583302492));
#77354=CARTESIAN_POINT('Ctrl Pts',(157.486356088001,-224.999337553498,10.387416697508));
#77355=CARTESIAN_POINT('Ctrl Pts',(157.487442263843,-225.460359745206,10.4164538270362));
#77356=CARTESIAN_POINT('Ctrl Pts',(157.608702652872,-225.921913657154,10.4454909565643));
#77357=CARTESIAN_POINT('Ctrl Pts',(157.84665351534,-226.312350891881,10.4745280860925));
#77358=CARTESIAN_POINT('Ctrl Pts',(158.280311749578,-227.023910917493,10.527447374503));
#77359=CARTESIAN_POINT('Ctrl Pts',(159.101545228238,-227.49926431249,10.5803666629137));
#77360=CARTESIAN_POINT('Ctrl Pts',(159.934557527633,-227.520889372667,10.6332859513243));
#77361=CARTESIAN_POINT('Ctrl Pts',(160.767569827029,-227.542514432845,10.6862052397348));
#77362=CARTESIAN_POINT('Ctrl Pts',(161.612360947159,-227.110411158202,10.7391245281454));
#77363=CARTESIAN_POINT('Ctrl Pts',(162.082354488063,-226.422309998721,10.792043816556));
#77364=CARTESIAN_POINT('Ctrl Pts',(162.552348028967,-225.734208839239,10.8449631049666));
#77365=CARTESIAN_POINT('Ctrl Pts',(162.647543990645,-224.790109794918,10.8978823933772));
#77366=CARTESIAN_POINT('Ctrl Pts',(162.324380702904,-224.022032569876,10.9508016817878));
#77367=CARTESIAN_POINT('Ctrl Pts',(162.001217415163,-223.253955344834,11.0037209701984));
#77368=CARTESIAN_POINT('Ctrl Pts',(161.259694878004,-222.661899939071,11.056640258609));
#77369=CARTESIAN_POINT('Ctrl Pts',(160.439133789851,-222.516790894623,11.1095595470196));
#77370=CARTESIAN_POINT('Ctrl Pts',(159.618572701698,-222.371681850175,11.1624788354302));
#77371=CARTESIAN_POINT('Ctrl Pts',(158.718973062551,-222.673519167043,11.2153981238408));
#77372=CARTESIAN_POINT('Ctrl Pts',(158.151991649595,-223.284182094961,11.2683174122514));
#77373=CARTESIAN_POINT('Ctrl Pts',(157.72664528368,-223.742298095335,11.3080171740036));
#77374=CARTESIAN_POINT('Ctrl Pts',(157.48849374887,-224.374218636619,11.3477169357558));
#77375=CARTESIAN_POINT('Ctrl Pts',(157.482816074282,-225.002298292055,11.387416697508));
#77376=CARTESIAN_POINT('Origin',(160.,-225.,10.));
#77377=CARTESIAN_POINT('',(157.478532324006,-224.999252277049,12.387416697508));
#77378=CARTESIAN_POINT('',(157.483927303789,-224.997828941348,12.112583302492));
#77379=CARTESIAN_POINT('',(157.4825,-225.,10.));
#77380=CARTESIAN_POINT('Ctrl Pts',(157.483927303789,-224.997828941348,12.112583302492));
#77381=CARTESIAN_POINT('Ctrl Pts',(157.481884400539,-224.74976888599,12.0969214542001));
#77382=CARTESIAN_POINT('Ctrl Pts',(157.51560216732,-224.50225200588,12.0812596059081));
#77383=CARTESIAN_POINT('Ctrl Pts',(157.587355810392,-224.266302038545,12.0655977576162));
#77384=CARTESIAN_POINT('Ctrl Pts',(157.829801763221,-223.469058690305,12.0126784692056));
#77385=CARTESIAN_POINT('Ctrl Pts',(158.506493281338,-222.803871733718,11.959759180795));
#77386=CARTESIAN_POINT('Ctrl Pts',(159.307776339359,-222.575130707039,11.9068398923844));
#77387=CARTESIAN_POINT('Ctrl Pts',(160.109059397379,-222.346389680361,11.8539206039738));
#77388=CARTESIAN_POINT('Ctrl Pts',(161.034933995303,-222.554094583591,11.8010013155632));
#77389=CARTESIAN_POINT('Ctrl Pts',(161.661719935324,-223.103199657096,11.7480820271526));
#77390=CARTESIAN_POINT('Ctrl Pts',(162.288505875345,-223.6523047306,11.695162738742));
#77391=CARTESIAN_POINT('Ctrl Pts',(162.616203157464,-224.542809974379,11.6422434503314));
#77392=CARTESIAN_POINT('Ctrl Pts',(162.494857511826,-225.367220206388,11.5893241619208));
#77393=CARTESIAN_POINT('Ctrl Pts',(162.373511866188,-226.191630438397,11.5364048735102));
#77394=CARTESIAN_POINT('Ctrl Pts',(161.803123292794,-226.949945658637,11.4834855850996));
#77395=CARTESIAN_POINT('Ctrl Pts',(161.044701591613,-227.295160837235,11.430566296689));
#77396=CARTESIAN_POINT('Ctrl Pts',(160.286279890432,-227.640376015833,11.3776470082784));
#77397=CARTESIAN_POINT('Ctrl Pts',(159.339825061465,-227.57249115279,11.3247277198679));
#77398=CARTESIAN_POINT('Ctrl Pts',(158.638434815837,-227.122570360099,11.2718084314573));
#77399=CARTESIAN_POINT('Ctrl Pts',(157.93704457021,-226.672649567409,11.2188891430467));
#77400=CARTESIAN_POINT('Ctrl Pts',(157.480718907923,-225.84069284507,11.1659698546361));
#77401=CARTESIAN_POINT('Ctrl Pts',(157.478272443065,-225.007403572869,11.1130505662255));
#77402=CARTESIAN_POINT('Ctrl Pts',(157.478265242513,-225.004950996073,11.1128948116476));
#77403=CARTESIAN_POINT('Ctrl Pts',(157.478261973784,-225.002498407734,11.1127390570698));
#77404=CARTESIAN_POINT('Ctrl Pts',(157.47826263161,-225.000045817589,11.112583302492));
#77405=CARTESIAN_POINT('Ctrl Pts',(157.482816074282,-225.002298292055,11.387416697508));
#77406=CARTESIAN_POINT('Ctrl Pts',(157.480925479294,-225.211441001789,11.4006362241664));
#77407=CARTESIAN_POINT('Ctrl Pts',(157.504811751628,-225.420157831362,11.4138557508248));
#77408=CARTESIAN_POINT('Ctrl Pts',(157.556146678958,-225.621889774519,11.4270752774832));
#77409=CARTESIAN_POINT('Ctrl Pts',(157.761646308041,-226.429445987186,11.4799945658938));
#77410=CARTESIAN_POINT('Ctrl Pts',(158.407008752971,-227.125069873552,11.5329138543044));
#77411=CARTESIAN_POINT('Ctrl Pts',(159.196916171637,-227.390443956891,11.585833142715));
#77412=CARTESIAN_POINT('Ctrl Pts',(159.986823590303,-227.655818040231,11.6387524311256));
#77413=CARTESIAN_POINT('Ctrl Pts',(160.921275982705,-227.490942320545,11.6916717195362));
#77414=CARTESIAN_POINT('Ctrl Pts',(161.572667952453,-226.971263923919,11.7445910079468));
#77415=CARTESIAN_POINT('Ctrl Pts',(162.224059922201,-226.451585527294,11.7975102963574));
#77416=CARTESIAN_POINT('Ctrl Pts',(162.592391469295,-225.577104453729,11.850429584768));
#77417=CARTESIAN_POINT('Ctrl Pts',(162.509114085028,-224.747983225294,11.9033488731786));
#77418=CARTESIAN_POINT('Ctrl Pts',(162.42583670076,-223.91886199686,11.9562681615892));
#77419=CARTESIAN_POINT('Ctrl Pts',(161.89095038513,-223.135100613555,12.0091874499998));
#77420=CARTESIAN_POINT('Ctrl Pts',(161.149219105654,-222.75534826897,12.0621067384104));
#77421=CARTESIAN_POINT('Ctrl Pts',(160.407487826177,-222.375595924385,12.115026026821));
#77422=CARTESIAN_POINT('Ctrl Pts',(159.458911582854,-222.39985261852,12.1679453152316));
#77423=CARTESIAN_POINT('Ctrl Pts',(158.737558845978,-222.817018488615,12.2208646036422));
#77424=CARTESIAN_POINT('Ctrl Pts',(158.016206109101,-223.234184358711,12.2737838920528));
#77425=CARTESIAN_POINT('Ctrl Pts',(157.522076878672,-224.044259404767,12.3267031804634));
#77426=CARTESIAN_POINT('Ctrl Pts',(157.481284680818,-224.876553301636,12.379622468874));
#77427=CARTESIAN_POINT('Ctrl Pts',(157.479281984977,-224.917414829432,12.3822205450853));
#77428=CARTESIAN_POINT('Ctrl Pts',(157.478371979161,-224.958329911901,12.3848186212967));
#77429=CARTESIAN_POINT('Ctrl Pts',(157.478532324006,-224.999252277049,12.387416697508));
#77430=CARTESIAN_POINT('Origin',(160.,-225.,10.));
#77431=CARTESIAN_POINT('',(157.485016161947,-224.998176142204,13.387416697508));
#77432=CARTESIAN_POINT('',(157.485914094323,-225.001240687775,13.112583302492));
#77433=CARTESIAN_POINT('',(157.4825,-225.,10.));
#77434=CARTESIAN_POINT('Ctrl Pts',(157.485914094323,-225.001240687775,13.112583302492));
#77435=CARTESIAN_POINT('Ctrl Pts',(157.4881419809,-224.501661538287,13.0811038513303));
#77436=CARTESIAN_POINT('Ctrl Pts',(157.632159107289,-224.000898646184,13.0496244001686));
#77437=CARTESIAN_POINT('Ctrl Pts',(157.909330132147,-223.589941778525,13.018144949007));
#77438=CARTESIAN_POINT('Ctrl Pts',(158.375275149048,-222.899092853229,12.9652256605964));
#77439=CARTESIAN_POINT('Ctrl Pts',(159.2175144088,-222.462036647188,12.9123063721858));
#77440=CARTESIAN_POINT('Ctrl Pts',(160.0506392427,-222.478770071692,12.8593870837752));
#77441=CARTESIAN_POINT('Ctrl Pts',(160.8837640766,-222.495503496197,12.8064677953646));
#77442=CARTESIAN_POINT('Ctrl Pts',(161.707774484648,-222.966026551246,12.753548506954));
#77443=CARTESIAN_POINT('Ctrl Pts',(162.145603320324,-223.675027896102,12.7006292185434));
#77444=CARTESIAN_POINT('Ctrl Pts',(162.583432156,-224.384029240958,12.6477099301328));
#77445=CARTESIAN_POINT('Ctrl Pts',(162.635079419304,-225.331508875619,12.5947906417222));
#77446=CARTESIAN_POINT('Ctrl Pts',(162.276911323562,-226.083900137896,12.5418713533116));
#77447=CARTESIAN_POINT('Ctrl Pts',(161.91874322782,-226.836291400172,12.488952064901));
#77448=CARTESIAN_POINT('Ctrl Pts',(161.150759773034,-227.393594290062,12.4360327764904));
#77449=CARTESIAN_POINT('Ctrl Pts',(160.324390173013,-227.500787016111,12.3831134880798));
#77450=CARTESIAN_POINT('Ctrl Pts',(159.498020572992,-227.607979742159,12.3301941996692));
#77451=CARTESIAN_POINT('Ctrl Pts',(158.613264827736,-227.265062304366,12.2772749112586));
#77452=CARTESIAN_POINT('Ctrl Pts',(158.074987148879,-226.628953715522,12.224355622848));
#77453=CARTESIAN_POINT('Ctrl Pts',(157.696016664022,-226.181106090023,12.1870981827293));
#77454=CARTESIAN_POINT('Ctrl Pts',(157.488787097096,-225.58793060024,12.1498407426107));
#77455=CARTESIAN_POINT('Ctrl Pts',(157.483927303789,-224.997828941348,12.112583302492));
#77456=CARTESIAN_POINT('Ctrl Pts',(157.478532324006,-224.999252277049,12.387416697508));
#77457=CARTESIAN_POINT('Ctrl Pts',(157.481637986168,-225.791862983123,12.4377379097073));
#77458=CARTESIAN_POINT('Ctrl Pts',(157.88627965685,-226.587205745219,12.4880591219065));
#77459=CARTESIAN_POINT('Ctrl Pts',(158.530138676728,-227.049066528146,12.5383803341058));
#77460=CARTESIAN_POINT('Ctrl Pts',(159.207240035769,-227.534773110103,12.5912996225164));
#77461=CARTESIAN_POINT('Ctrl Pts',(160.148897919128,-227.651673526335,12.644218910927));
#77462=CARTESIAN_POINT('Ctrl Pts',(160.924209697895,-227.346274148673,12.6971381993375));
#77463=CARTESIAN_POINT('Ctrl Pts',(161.699521476663,-227.040874771011,12.7500574877481));
#77464=CARTESIAN_POINT('Ctrl Pts',(162.308487150838,-226.313175599455,12.8029767761587));
#77465=CARTESIAN_POINT('Ctrl Pts',(162.472444039893,-225.4961717606,12.8558960645693));
#77466=CARTESIAN_POINT('Ctrl Pts',(162.636400928947,-224.679167921746,12.9088153529799));
#77467=CARTESIAN_POINT('Ctrl Pts',(162.35534903288,-223.772859415593,12.9617346413905));
#77468=CARTESIAN_POINT('Ctrl Pts',(161.757897693807,-223.191972996737,13.0146539298011));
#77469=CARTESIAN_POINT('Ctrl Pts',(161.160446354733,-222.611086577882,13.0675732182117));
#77470=CARTESIAN_POINT('Ctrl Pts',(160.246595572652,-222.355622246324,13.1204925066223));
#77471=CARTESIAN_POINT('Ctrl Pts',(159.434523447476,-222.542480475161,13.1734117950329));
#77472=CARTESIAN_POINT('Ctrl Pts',(158.622451322301,-222.729338703999,13.2263310834435));
#77473=CARTESIAN_POINT('Ctrl Pts',(157.91215785403,-223.358519493232,13.2792503718541));
#77474=CARTESIAN_POINT('Ctrl Pts',(157.628673319779,-224.142109726078,13.3321696602647));
#77475=CARTESIAN_POINT('Ctrl Pts',(157.530021951554,-224.414795672783,13.3505853393458));
#77476=CARTESIAN_POINT('Ctrl Pts',(157.483057542947,-224.706180746991,13.3690010184269));
#77477=CARTESIAN_POINT('Ctrl Pts',(157.485016161947,-224.998176142204,13.387416697508));
#77478=CARTESIAN_POINT('Origin',(160.,-225.,10.));
#77479=CARTESIAN_POINT('',(157.485110449967,-225.001779462518,14.387416697508));
#77480=CARTESIAN_POINT('',(157.479399137962,-225.001499392172,14.112583302492));
#77481=CARTESIAN_POINT('',(157.4825,-225.,10.));
#77482=CARTESIAN_POINT('Ctrl Pts',(157.479399137962,-225.001499392172,14.112583302492));
#77483=CARTESIAN_POINT('Ctrl Pts',(157.484655218445,-224.255844409846,14.0652862484606));
#77484=CARTESIAN_POINT('Ctrl Pts',(157.836334846753,-223.505881912547,14.0179891944291));
#77485=CARTESIAN_POINT('Ctrl Pts',(158.415784496789,-223.038004606611,13.9706921403977));
#77486=CARTESIAN_POINT('Ctrl Pts',(159.064113737957,-222.514510393269,13.9177728519871));
#77487=CARTESIAN_POINT('Ctrl Pts',(159.997581815466,-222.344150638113,13.8648535635765));
#77488=CARTESIAN_POINT('Ctrl Pts',(160.789033755402,-222.604881961754,13.8119342751659));
#77489=CARTESIAN_POINT('Ctrl Pts',(161.580485695339,-222.865613285395,13.7590149867553));
#77490=CARTESIAN_POINT('Ctrl Pts',(162.229921497702,-223.557435687833,13.7060956983447));
#77491=CARTESIAN_POINT('Ctrl Pts',(162.4401593521,-224.363771251314,13.6531764099341));
#77492=CARTESIAN_POINT('Ctrl Pts',(162.650397206498,-225.170106814795,13.6002571215235));
#77493=CARTESIAN_POINT('Ctrl Pts',(162.421437112931,-226.09095553932,13.5473378331129));
#77494=CARTESIAN_POINT('Ctrl Pts',(161.858051205713,-226.704937066652,13.4944185447023));
#77495=CARTESIAN_POINT('Ctrl Pts',(161.294665298495,-227.318918593984,13.4414992562917));
#77496=CARTESIAN_POINT('Ctrl Pts',(160.396853577626,-227.626032924123,13.3885799678811));
#77497=CARTESIAN_POINT('Ctrl Pts',(159.575454668923,-227.485744545635,13.3356606794706));
#77498=CARTESIAN_POINT('Ctrl Pts',(158.75405576022,-227.345456167148,13.28274139106));
#77499=CARTESIAN_POINT('Ctrl Pts',(158.009069663684,-226.757765080034,13.2298221026494));
#77500=CARTESIAN_POINT('Ctrl Pts',(157.68140200244,-225.991598714202,13.1769028142388));
#77501=CARTESIAN_POINT('Ctrl Pts',(157.548650003315,-225.681192382553,13.1554629769898));
#77502=CARTESIAN_POINT('Ctrl Pts',(157.484396738593,-225.341491081689,13.1340231397409));
#77503=CARTESIAN_POINT('Ctrl Pts',(157.485914094323,-225.001240687775,13.112583302492));
#77504=CARTESIAN_POINT('Ctrl Pts',(157.485016161947,-224.998176142204,13.387416697508));
#77505=CARTESIAN_POINT('Ctrl Pts',(157.488685829761,-225.545258603735,13.4219203068375));
#77506=CARTESIAN_POINT('Ctrl Pts',(157.664093696845,-226.09448352119,13.456423916167));
#77507=CARTESIAN_POINT('Ctrl Pts',(157.99306127657,-226.526880121952,13.4909275254965));
#77508=CARTESIAN_POINT('Ctrl Pts',(158.497609367842,-227.190060608521,13.5438468139071));
#77509=CARTESIAN_POINT('Ctrl Pts',(159.363381150619,-227.578421905197,13.5967661023177));
#77510=CARTESIAN_POINT('Ctrl Pts',(160.194199474123,-227.514249890259,13.6496853907283));
#77511=CARTESIAN_POINT('Ctrl Pts',(161.025017797627,-227.450077875321,13.7026046791389));
#77512=CARTESIAN_POINT('Ctrl Pts',(161.820882661859,-226.933372548768,13.7555239675495));
#77513=CARTESIAN_POINT('Ctrl Pts',(162.217606320595,-226.200578257871,13.8084432559601));
#77514=CARTESIAN_POINT('Ctrl Pts',(162.614329979331,-225.467783966974,13.8613625443707));
#77515=CARTESIAN_POINT('Ctrl Pts',(162.611912432571,-224.518900711734,13.9142818327813));
#77516=CARTESIAN_POINT('Ctrl Pts',(162.211459949664,-223.788137451091,13.9672011211919));
#77517=CARTESIAN_POINT('Ctrl Pts',(161.811007466758,-223.057374190448,14.0201204096025));
#77518=CARTESIAN_POINT('Ctrl Pts',(161.012520047705,-222.544730924403,14.0730396980131));
#77519=CARTESIAN_POINT('Ctrl Pts',(160.181385519764,-222.484793201417,14.1259589864237));
#77520=CARTESIAN_POINT('Ctrl Pts',(159.350250991823,-222.424855478432,14.1788782748343));
#77521=CARTESIAN_POINT('Ctrl Pts',(158.486469354995,-222.817623298507,14.2317975632449));
#77522=CARTESIAN_POINT('Ctrl Pts',(157.985307069309,-223.483366114898,14.2847168516555));
#77523=CARTESIAN_POINT('Ctrl Pts',(157.661107134949,-223.914032554769,14.3189501336063));
#77524=CARTESIAN_POINT('Ctrl Pts',(157.488654181408,-224.458932091686,14.3531834155572));
#77525=CARTESIAN_POINT('Ctrl Pts',(157.485110449967,-225.001779462518,14.387416697508));
#77526=CARTESIAN_POINT('Origin',(160.,-225.,10.));
#77527=CARTESIAN_POINT('',(157.478588566705,-225.000821673807,15.387416697508));
#77528=CARTESIAN_POINT('',(157.481369728344,-224.997804627087,15.112583302492));
#77529=CARTESIAN_POINT('',(157.4825,-225.,10.));
#77530=CARTESIAN_POINT('Ctrl Pts',(157.481369728344,-224.997804627087,15.112583302492));
#77531=CARTESIAN_POINT('Ctrl Pts',(157.479896256025,-224.836743702289,15.1023879340014));
#77532=CARTESIAN_POINT('Ctrl Pts',(157.494022458441,-224.675940232443,15.0921925655108));
#77533=CARTESIAN_POINT('Ctrl Pts',(157.524685419075,-224.518354477072,15.0819971970203));
#77534=CARTESIAN_POINT('Ctrl Pts',(157.683842202748,-223.70040208569,15.0290779086097));
#77535=CARTESIAN_POINT('Ctrl Pts',(158.288524432771,-222.969139821792,14.9761586201991));
#77536=CARTESIAN_POINT('Ctrl Pts',(159.062029532575,-222.659193282961,14.9232393317885));
#77537=CARTESIAN_POINT('Ctrl Pts',(159.835534632379,-222.34924674413,14.8703200433779));
#77538=CARTESIAN_POINT('Ctrl Pts',(160.777862601965,-222.460615930365,14.8174007549673));
#77539=CARTESIAN_POINT('Ctrl Pts',(161.457804180978,-222.942338304235,14.7644814665567));
#77540=CARTESIAN_POINT('Ctrl Pts',(162.13774575999,-223.424060678104,14.7115621781461));
#77541=CARTESIAN_POINT('Ctrl Pts',(162.555300948429,-224.276136239609,14.6586428897355));
#77542=CARTESIAN_POINT('Ctrl Pts',(162.519396500276,-225.108655228557,14.6057236013249));
#77543=CARTESIAN_POINT('Ctrl Pts',(162.483492052122,-225.941174217505,14.5528043129143));
#77544=CARTESIAN_POINT('Ctrl Pts',(161.994127967376,-226.754136633897,14.4998850245037));
#77545=CARTESIAN_POINT('Ctrl Pts',(161.275237241595,-227.175530891977,14.4469657360931));
#77546=CARTESIAN_POINT('Ctrl Pts',(160.556346515813,-227.596925150056,14.3940464476825));
#77547=CARTESIAN_POINT('Ctrl Pts',(159.607929148997,-227.626751249823,14.3411271592719));
#77548=CARTESIAN_POINT('Ctrl Pts',(158.863980909553,-227.25136076861,14.2882078708613));
#77549=CARTESIAN_POINT('Ctrl Pts',(158.12003267011,-226.875970287397,14.2352885824507));
#77550=CARTESIAN_POINT('Ctrl Pts',(157.580553558038,-226.095363225205,14.1823692940401));
#77551=CARTESIAN_POINT('Ctrl Pts',(157.492409204416,-225.266745358344,14.1294500056295));
#77552=CARTESIAN_POINT('Ctrl Pts',(157.483044599748,-225.1787115998,14.1238277712503));
#77553=CARTESIAN_POINT('Ctrl Pts',(157.478774343945,-225.090135929108,14.1182055368712));
#77554=CARTESIAN_POINT('Ctrl Pts',(157.479399137962,-225.001499392172,14.112583302492));
#77555=CARTESIAN_POINT('Ctrl Pts',(157.485110449967,-225.001779462518,14.387416697508));
#77556=CARTESIAN_POINT('Ctrl Pts',(157.483176128021,-225.298089044889,14.4061027039678));
#77557=CARTESIAN_POINT('Ctrl Pts',(157.531567442652,-225.593787194898,14.4247887104275));
#77558=CARTESIAN_POINT('Ctrl Pts',(157.633075509796,-225.869962300384,14.4434747168873));
#77559=CARTESIAN_POINT('Ctrl Pts',(157.920549170516,-226.652097856771,14.4963940052979));
#77560=CARTESIAN_POINT('Ctrl Pts',(158.634039426501,-227.277651156836,14.5493132937085));
#77561=CARTESIAN_POINT('Ctrl Pts',(159.447053150641,-227.460369022769,14.6022325821191));
#77562=CARTESIAN_POINT('Ctrl Pts',(160.260066874781,-227.643086888702,14.6551518705297));
#77563=CARTESIAN_POINT('Ctrl Pts',(161.172604067077,-227.382969320504,14.7080711589403));
#77564=CARTESIAN_POINT('Ctrl Pts',(161.767087726275,-226.799046112267,14.7609904473509));
#77565=CARTESIAN_POINT('Ctrl Pts',(162.361571385474,-226.21512290403,14.8139097357615));
#77566=CARTESIAN_POINT('Ctrl Pts',(162.638001511576,-225.307394055755,14.866829024172));
#77567=CARTESIAN_POINT('Ctrl Pts',(162.469883684311,-224.491236270564,14.9197483125826));
#77568=CARTESIAN_POINT('Ctrl Pts',(162.301765857047,-223.675078485373,14.9726676009932));
#77569=CARTESIAN_POINT('Ctrl Pts',(161.689100076417,-222.950491763267,15.0255868894038));
#77570=CARTESIAN_POINT('Ctrl Pts',(160.912242191591,-222.649046974034,15.0785061778144));
#77571=CARTESIAN_POINT('Ctrl Pts',(160.135384306766,-222.347602184801,15.131425466225));
#77572=CARTESIAN_POINT('Ctrl Pts',(159.194334317744,-222.469299328443,15.1843447546356));
#77573=CARTESIAN_POINT('Ctrl Pts',(158.519716681,-222.95844979442,15.2372640430462));
#77574=CARTESIAN_POINT('Ctrl Pts',(157.881665591336,-223.421086658366,15.2873149278668));
#77575=CARTESIAN_POINT('Ctrl Pts',(157.481946572589,-224.212422010048,15.3373658126874));
#77576=CARTESIAN_POINT('Ctrl Pts',(157.478588566705,-225.000821673807,15.387416697508));
#77577=CARTESIAN_POINT('Origin',(160.,-225.,10.));
#77578=CARTESIAN_POINT('',(157.482688037232,-224.997698966056,16.387416697508));
#77579=CARTESIAN_POINT('',(157.486513026464,-224.999883653202,16.112583302492));
#77580=CARTESIAN_POINT('',(157.4825,-225.,10.));
#77581=CARTESIAN_POINT('Ctrl Pts',(157.486513026464,-224.999883653202,16.112583302492));
#77582=CARTESIAN_POINT('Ctrl Pts',(157.486342723674,-224.586811779428,16.0865703311317));
#77583=CARTESIAN_POINT('Ctrl Pts',(157.58248784144,-224.173814561698,16.0605573597713));
#77584=CARTESIAN_POINT('Ctrl Pts',(157.775382603526,-223.812463843255,16.034544388411));
#77585=CARTESIAN_POINT('Ctrl Pts',(158.167796580626,-223.077352785706,15.9816251000004));
#77586=CARTESIAN_POINT('Ctrl Pts',(158.960613668561,-222.555983278562,15.9287058115898));
#77587=CARTESIAN_POINT('Ctrl Pts',(159.791040783494,-222.486933998053,15.8757865231792));
#77588=CARTESIAN_POINT('Ctrl Pts',(160.621467898426,-222.417884717545,15.8228672347686));
#77589=CARTESIAN_POINT('Ctrl Pts',(161.489505040356,-222.801155663671,15.769947946358));
#77590=CARTESIAN_POINT('Ctrl Pts',(161.997938430197,-223.461362059015,15.7170286579474));
#77591=CARTESIAN_POINT('Ctrl Pts',(162.506371820038,-224.121568454359,15.6641093695368));
#77592=CARTESIAN_POINT('Ctrl Pts',(162.65520145779,-225.058710298921,15.6111900811262));
#77593=CARTESIAN_POINT('Ctrl Pts',(162.376322904148,-225.843951503058,15.5582707927156));
#77594=CARTESIAN_POINT('Ctrl Pts',(162.097444350506,-226.629192707195,15.505351504305));
#77595=CARTESIAN_POINT('Ctrl Pts',(161.390857605468,-227.262533270907,15.4524322158945));
#77596=CARTESIAN_POINT('Ctrl Pts',(160.579896749671,-227.454156564691,15.3995129274839));
#77597=CARTESIAN_POINT('Ctrl Pts',(159.768935893874,-227.645779858475,15.3465936390733));
#77598=CARTESIAN_POINT('Ctrl Pts',(158.853600927316,-227.395685882331,15.2936743506627));
#77599=CARTESIAN_POINT('Ctrl Pts',(158.252749112698,-226.818317634826,15.2407550622521));
#77600=CARTESIAN_POINT('Ctrl Pts',(157.767656709105,-226.352184481647,15.198031142332));
#77601=CARTESIAN_POINT('Ctrl Pts',(157.487544347085,-225.672734038383,15.155307222412));
#77602=CARTESIAN_POINT('Ctrl Pts',(157.481369728344,-224.997804627087,15.112583302492));
#77603=CARTESIAN_POINT('Ctrl Pts',(157.478588566705,-225.000821673807,15.387416697508));
#77604=CARTESIAN_POINT('Ctrl Pts',(157.478396120234,-225.046004659762,15.390285101098));
#77605=CARTESIAN_POINT('Ctrl Pts',(157.479505484729,-225.091178003722,15.393153504688));
#77606=CARTESIAN_POINT('Ctrl Pts',(157.481946405746,-225.136279282669,15.396021908278));
#77607=CARTESIAN_POINT('Ctrl Pts',(157.526979051704,-225.96835451663,15.4489411966886));
#77608=CARTESIAN_POINT('Ctrl Pts',(158.025229628086,-226.775901196241,15.5018604850992));
#77609=CARTESIAN_POINT('Ctrl Pts',(158.748698680934,-227.189385976782,15.5547797735098));
#77610=CARTESIAN_POINT('Ctrl Pts',(159.472167733783,-227.602870757323,15.6076990619204));
#77611=CARTESIAN_POINT('Ctrl Pts',(160.420855263099,-227.622293638794,15.660618350331));
#77612=CARTESIAN_POINT('Ctrl Pts',(161.160641874123,-227.238766711032,15.7135376387416));
#77613=CARTESIAN_POINT('Ctrl Pts',(161.900428485148,-226.855239783271,15.7664569271522));
#77614=CARTESIAN_POINT('Ctrl Pts',(162.431314177881,-226.068763046276,15.8193762155628));
#77615=CARTESIAN_POINT('Ctrl Pts',(162.510365669759,-225.2392282394,15.8722955039734));
#77616=CARTESIAN_POINT('Ctrl Pts',(162.589417161637,-224.409693432523,15.925214792384));
#77617=CARTESIAN_POINT('Ctrl Pts',(162.21663445266,-223.537100555763,15.9781340807946));
#77618=CARTESIAN_POINT('Ctrl Pts',(161.562602903142,-223.020748092442,16.0310533692052));
#77619=CARTESIAN_POINT('Ctrl Pts',(160.908571353624,-222.50439562912,16.0839726576158));
#77620=CARTESIAN_POINT('Ctrl Pts',(159.973290963564,-222.344283579236,16.1368919460264));
#77621=CARTESIAN_POINT('Ctrl Pts',(159.184746021032,-222.613679213519,16.189811234437));
#77622=CARTESIAN_POINT('Ctrl Pts',(158.396201078501,-222.883074847802,16.2427305228476));
#77623=CARTESIAN_POINT('Ctrl Pts',(157.754391583496,-223.581978166253,16.2956498112582));
#77624=CARTESIAN_POINT('Ctrl Pts',(157.553009548383,-224.390571024399,16.3485690996688));
#77625=CARTESIAN_POINT('Ctrl Pts',(157.503731937471,-224.588431395745,16.3615182989485));
#77626=CARTESIAN_POINT('Ctrl Pts',(157.480825668259,-224.792859614458,16.3744674982283));
#77627=CARTESIAN_POINT('Ctrl Pts',(157.482688037232,-224.997698966056,16.387416697508));
#77628=CARTESIAN_POINT('Origin',(160.,-225.,10.));
#77629=CARTESIAN_POINT('',(157.486388068275,-225.000594615142,17.387416697508));
#77630=CARTESIAN_POINT('',(157.48179671173,-225.002256423607,17.112583302492));
#77631=CARTESIAN_POINT('',(157.4825,-225.,10.));
#77632=CARTESIAN_POINT('Ctrl Pts',(157.48179671173,-225.002256423607,17.112583302492));
#77633=CARTESIAN_POINT('Ctrl Pts',(157.487898020156,-224.341151277727,17.0707527282619));
#77634=CARTESIAN_POINT('Ctrl Pts',(157.755182207898,-223.675680124248,17.0289221540319));
#77635=CARTESIAN_POINT('Ctrl Pts',(158.222379318362,-223.211361021709,16.9870915798018));
#77636=CARTESIAN_POINT('Ctrl Pts',(158.813424004892,-222.623957263715,16.9341722913912));
#77637=CARTESIAN_POINT('Ctrl Pts',(159.724418023019,-222.358485991985,16.8812530029806));
#77638=CARTESIAN_POINT('Ctrl Pts',(160.53849052896,-222.536426856176,16.82833371457));
#77639=CARTESIAN_POINT('Ctrl Pts',(161.3525630349,-222.714367720367,16.7754144261594));
#77640=CARTESIAN_POINT('Ctrl Pts',(162.069714028654,-223.335720720481,16.7224951377488));
#77641=CARTESIAN_POINT('Ctrl Pts',(162.361775229099,-224.116154735432,16.6695758493382));
#77642=CARTESIAN_POINT('Ctrl Pts',(162.653836429543,-224.896588750382,16.6166565609276));
#77643=CARTESIAN_POINT('Ctrl Pts',(162.520807836678,-225.836103780169,16.563737272517));
#77644=CARTESIAN_POINT('Ctrl Pts',(162.023563332215,-226.504777765852,16.5108179841064));
#77645=CARTESIAN_POINT('Ctrl Pts',(161.526318827752,-227.173451751535,16.4578986956958));
#77646=CARTESIAN_POINT('Ctrl Pts',(160.664858411691,-227.571284693115,16.4049794072852));
#77647=CARTESIAN_POINT('Ctrl Pts',(159.833386353372,-227.516228244241,16.3520601188746));
#77648=CARTESIAN_POINT('Ctrl Pts',(159.001914295052,-227.461171795367,16.299140830464));
#77649=CARTESIAN_POINT('Ctrl Pts',(158.200430594475,-226.95322595604,16.2462215420534));
#77650=CARTESIAN_POINT('Ctrl Pts',(157.795694177318,-226.224826732399,16.1933022536428));
#77651=CARTESIAN_POINT('Ctrl Pts',(157.589909732952,-225.854478962444,16.1663959365925));
#77652=CARTESIAN_POINT('Ctrl Pts',(157.486689177846,-225.427141371915,16.1394896195423));
#77653=CARTESIAN_POINT('Ctrl Pts',(157.486513026464,-224.999883653202,16.112583302492));
#77654=CARTESIAN_POINT('Ctrl Pts',(157.482688037232,-224.997698966056,16.387416697508));
#77655=CARTESIAN_POINT('Ctrl Pts',(157.488436582161,-225.629973361099,16.4273867866389));
#77656=CARTESIAN_POINT('Ctrl Pts',(157.73017128722,-226.266164873843,16.4673568757697));
#77657=CARTESIAN_POINT('Ctrl Pts',(158.160758640894,-226.725212210085,16.5073269649006));
#77658=CARTESIAN_POINT('Ctrl Pts',(158.730844343742,-227.332978139783,16.5602462533112));
#77659=CARTESIAN_POINT('Ctrl Pts',(159.631970324661,-227.630227601337,16.6131655417218));
#77660=CARTESIAN_POINT('Ctrl Pts',(160.451781352795,-227.480939248318,16.6660848301324));
#77661=CARTESIAN_POINT('Ctrl Pts',(161.271592380928,-227.331650895299,16.719004118543));
#77662=CARTESIAN_POINT('Ctrl Pts',(162.010088456277,-226.735824727707,16.7719234069535));
#77663=CARTESIAN_POINT('Ctrl Pts',(162.32933378867,-225.966110785349,16.8248426953641));
#77664=CARTESIAN_POINT('Ctrl Pts',(162.648579121063,-225.196396842992,16.8777619837747));
#77665=CARTESIAN_POINT('Ctrl Pts',(162.5485737105,-224.252795125869,16.9306812721853));
#77666=CARTESIAN_POINT('Ctrl Pts',(162.075080032158,-223.567097766926,16.9836005605959));
#77667=CARTESIAN_POINT('Ctrl Pts',(161.601586353816,-222.881400407983,17.0365198490065));
#77668=CARTESIAN_POINT('Ctrl Pts',(160.754604407694,-222.453607407218,17.0894391374171));
#77669=CARTESIAN_POINT('Ctrl Pts',(159.921713113051,-222.479476821456,17.1423584258277));
#77670=CARTESIAN_POINT('Ctrl Pts',(159.088821818408,-222.505346235694,17.1952777142383));
#77671=CARTESIAN_POINT('Ctrl Pts',(158.270021175245,-222.984878064933,17.2481970026489));
#77672=CARTESIAN_POINT('Ctrl Pts',(157.839994347237,-223.698638578269,17.3011162910595));
#77673=CARTESIAN_POINT('Ctrl Pts',(157.606232763289,-224.086637133918,17.329883093209));
#77674=CARTESIAN_POINT('Ctrl Pts',(157.48735323228,-224.543849898541,17.3586498953585));
#77675=CARTESIAN_POINT('Ctrl Pts',(157.486388068275,-225.000594615142,17.387416697508));
#77676=CARTESIAN_POINT('Origin',(160.,-225.,10.));
#77677=CARTESIAN_POINT('',(157.480508436316,-225.001988388677,18.387416697508));
#77678=CARTESIAN_POINT('',(157.479093605947,-224.998703157778,18.112583302492));
#77679=CARTESIAN_POINT('',(157.4825,-225.,10.));
#77680=CARTESIAN_POINT('Ctrl Pts',(157.479093605947,-224.998703157778,18.112583302492));
#77681=CARTESIAN_POINT('Ctrl Pts',(157.478625726168,-224.92417432602,18.1078544138028));
#77682=CARTESIAN_POINT('Ctrl Pts',(157.481644431352,-224.849683927444,18.1031255251135));
#77683=CARTESIAN_POINT('Ctrl Pts',(157.488273116953,-224.775516169229,18.0983966364243));
#77684=CARTESIAN_POINT('Ctrl Pts',(157.562452347668,-223.945531526816,18.0454773480137));
#77685=CARTESIAN_POINT('Ctrl Pts',(158.088710912316,-223.155951269613,17.9925580596031));
#77686=CARTESIAN_POINT('Ctrl Pts',(158.826232736485,-222.768087153071,17.9396387711925));
#77687=CARTESIAN_POINT('Ctrl Pts',(159.563754560655,-222.38022303653,17.8867194827819));
#77688=CARTESIAN_POINT('Ctrl Pts',(160.512539644345,-222.39407506065,17.8338001943713));
#77689=CARTESIAN_POINT('Ctrl Pts',(161.238424031716,-222.803304614037,17.7808809059607));
#77690=CARTESIAN_POINT('Ctrl Pts',(161.964308419087,-223.212534167423,17.7279616175502));
#77691=CARTESIAN_POINT('Ctrl Pts',(162.467292110139,-224.017141250075,17.6750423291395));
#77692=CARTESIAN_POINT('Ctrl Pts',(162.517209739275,-224.848937640852,17.6221230407289));
#77693=CARTESIAN_POINT('Ctrl Pts',(162.567127368411,-225.680734031629,17.5692037523183));
#77694=CARTESIAN_POINT('Ctrl Pts',(162.16397893563,-226.539719730531,17.5162844639078));
#77695=CARTESIAN_POINT('Ctrl Pts',(161.492245174384,-227.032822915951,17.4633651754972));
#77696=CARTESIAN_POINT('Ctrl Pts',(160.820511413138,-227.525926101371,17.4104458870866));
#77697=CARTESIAN_POINT('Ctrl Pts',(159.880192323427,-227.653146773309,17.357526598676));
#77698=CARTESIAN_POINT('Ctrl Pts',(159.101577893279,-227.35626874644,17.3046073102654));
#77699=CARTESIAN_POINT('Ctrl Pts',(158.322963463131,-227.059390719571,17.2516880218548));
#77700=CARTESIAN_POINT('Ctrl Pts',(157.706053692547,-226.338413993894,17.1987687334442));
#77701=CARTESIAN_POINT('Ctrl Pts',(157.533146484722,-225.523257508927,17.1458494450336));
#77702=CARTESIAN_POINT('Ctrl Pts',(157.496915487198,-225.352449519144,17.134760730853));
#77703=CARTESIAN_POINT('Ctrl Pts',(157.480179338158,-225.177506372738,17.1236720166725));
#77704=CARTESIAN_POINT('Ctrl Pts',(157.48179671173,-225.002256423607,17.112583302492));
#77705=CARTESIAN_POINT('Ctrl Pts',(157.486388068275,-225.000594615142,17.387416697508));
#77706=CARTESIAN_POINT('Ctrl Pts',(157.48557772063,-225.384075560824,17.4115691837691));
#77707=CARTESIAN_POINT('Ctrl Pts',(157.567887699128,-225.767226569576,17.4357216700302));
#77708=CARTESIAN_POINT('Ctrl Pts',(157.735112675213,-226.108806281153,17.4598741562913));
#77709=CARTESIAN_POINT('Ctrl Pts',(158.101510844047,-226.857224273268,17.5127934447019));
#77710=CARTESIAN_POINT('Ctrl Pts',(158.875560194568,-227.406071060066,17.5657127331125));
#77711=CARTESIAN_POINT('Ctrl Pts',(159.703055782727,-227.504194469167,17.6186320215231));
#77712=CARTESIAN_POINT('Ctrl Pts',(160.530551370886,-227.602317878268,17.6715513099337));
#77713=CARTESIAN_POINT('Ctrl Pts',(161.411493196683,-227.249717909671,17.7244705983443));
#77714=CARTESIAN_POINT('Ctrl Pts',(161.942762249126,-226.607744081147,17.7773898867549));
#77715=CARTESIAN_POINT('Ctrl Pts',(162.474031301569,-225.965770252623,17.8303091751655));
#77716=CARTESIAN_POINT('Ctrl Pts',(162.655627580658,-225.034422564172,17.8832284635761));
#77717=CARTESIAN_POINT('Ctrl Pts',(162.404452733975,-224.239886158156,17.9361477519867));
#77718=CARTESIAN_POINT('Ctrl Pts',(162.153277887292,-223.445349752141,17.9890670403973));
#77719=CARTESIAN_POINT('Ctrl Pts',(161.469331914838,-222.787624628562,18.0419863288079));
#77720=CARTESIAN_POINT('Ctrl Pts',(160.665588269906,-222.567684839738,18.0949056172185));
#77721=CARTESIAN_POINT('Ctrl Pts',(159.861844624975,-222.347745050914,18.1478249056291));
#77722=CARTESIAN_POINT('Ctrl Pts',(158.938303307568,-222.565590596846,18.2007441940397));
#77723=CARTESIAN_POINT('Ctrl Pts',(158.317577242659,-223.121537334013,18.2536634824503));
#77724=CARTESIAN_POINT('Ctrl Pts',(157.794616652767,-223.589921457145,18.2982478874695));
#77725=CARTESIAN_POINT('Ctrl Pts',(157.486595301213,-224.298290891207,18.3428322924888));
#77726=CARTESIAN_POINT('Ctrl Pts',(157.480508436316,-225.001988388677,18.387416697508));
#77727=CARTESIAN_POINT('Origin',(160.,-225.,10.));
#77728=CARTESIAN_POINT('',(157.48014261364,-224.998176427436,19.387416697508));
#77729=CARTESIAN_POINT('',(157.485690666959,-224.998572567547,19.112583302492));
#77730=CARTESIAN_POINT('',(157.4825,-225.,10.));
#77731=CARTESIAN_POINT('',(161.913465996665,-223.364012796625,20.));
#77732=CARTESIAN_POINT('Ctrl Pts',(157.48014261364,-224.998176427436,19.387416697508));
#77733=CARTESIAN_POINT('Ctrl Pts',(157.486035940553,-225.714913366798,19.4328532664402));
#77734=CARTESIAN_POINT('Ctrl Pts',(157.807333049291,-226.436176607492,19.4782898353724));
#77735=CARTESIAN_POINT('Ctrl Pts',(158.347923879131,-226.905064937574,19.5237264043046));
#77736=CARTESIAN_POINT('Ctrl Pts',(158.97754188746,-227.451172122934,19.5766456927152));
#77737=CARTESIAN_POINT('Ctrl Pts',(159.904629866452,-227.654935000039,19.6295649811258));
#77738=CARTESIAN_POINT('Ctrl Pts',(160.704626517538,-227.421707597932,19.6824842695364));
#77739=CARTESIAN_POINT('Ctrl Pts',(161.504623168624,-227.188480195825,19.735403557947));
#77740=CARTESIAN_POINT('Ctrl Pts',(162.177528491803,-226.518262514506,19.7883228463576));
#77741=CARTESIAN_POINT('Ctrl Pts',(162.41573132851,-225.721203336705,19.8412421347682));
#77742=CARTESIAN_POINT('Ctrl Pts',(162.653934165218,-224.924144158904,19.8941614231788));
#77743=CARTESIAN_POINT('Ctrl Pts',(162.457434515453,-224.000243484621,19.9470807115894));
#77744=CARTESIAN_POINT('Ctrl Pts',(161.913465996665,-223.364012796625,20.));
#77745=CARTESIAN_POINT('',(158.082847463497,-223.361245209821,20.));
#77746=CARTESIAN_POINT('Origin',(160.,-225.,20.));
#77747=CARTESIAN_POINT('Ctrl Pts',(158.082843761452,-223.361242430594,20.));
#77748=CARTESIAN_POINT('Ctrl Pts',(158.613381559625,-222.742548892826,19.948244384658));
#77749=CARTESIAN_POINT('Ctrl Pts',(159.472376104806,-222.40287586538,19.896488769316));
#77750=CARTESIAN_POINT('Ctrl Pts',(160.282371278711,-222.494228189242,19.844733153974));
#77751=CARTESIAN_POINT('Ctrl Pts',(161.110578381185,-222.587634478424,19.7918138655634));
#77752=CARTESIAN_POINT('Ctrl Pts',(161.887557938352,-223.131666360088,19.7388945771528));
#77753=CARTESIAN_POINT('Ctrl Pts',(162.258271984796,-223.877852623269,19.6859752887422));
#77754=CARTESIAN_POINT('Ctrl Pts',(162.62898603124,-224.62403888645,19.6330560003316));
#77755=CARTESIAN_POINT('Ctrl Pts',(162.59343456696,-225.572379531148,19.5801367119211));
#77756=CARTESIAN_POINT('Ctrl Pts',(162.167641060891,-226.288685246806,19.5272174235105));
#77757=CARTESIAN_POINT('Ctrl Pts',(161.741847554822,-227.004990962463,19.4742981350999));
#77758=CARTESIAN_POINT('Ctrl Pts',(160.925812006964,-227.489261749081,19.4213788466893));
#77759=CARTESIAN_POINT('Ctrl Pts',(160.093070266903,-227.520005584259,19.3684595582787));
#77760=CARTESIAN_POINT('Ctrl Pts',(159.260328526843,-227.550749419438,19.3155402698681));
#77761=CARTESIAN_POINT('Ctrl Pts',(158.410880594581,-227.127966303179,19.2626209814575));
#77762=CARTESIAN_POINT('Ctrl Pts',(157.933376955139,-226.445068639568,19.2097016930469));
#77763=CARTESIAN_POINT('Ctrl Pts',(157.641269317644,-226.027313450515,19.1773288961952));
#77764=CARTESIAN_POINT('Ctrl Pts',(157.488352422676,-225.512216972223,19.1449560993436));
#77765=CARTESIAN_POINT('Ctrl Pts',(157.485690666959,-224.998572567547,19.112583302492));
#77766=CARTESIAN_POINT('Origin',(0.,225.,10.));
#77767=CARTESIAN_POINT('',(-2.51347389046773,225.0005858313,0.387416697508012));
#77768=CARTESIAN_POINT('',(-2.51553408751311,224.996405665924,0.112583302491965));
#77769=CARTESIAN_POINT('',(-2.5175,225.,10.));
#77770=CARTESIAN_POINT('',(-1.91346599666507,226.635987203375,0.));
#77771=CARTESIAN_POINT('Ctrl Pts',(-2.51553408751311,224.996405665924,0.112583302491965));
#77772=CARTESIAN_POINT('Ctrl Pts',(-2.51031901166848,225.589040573862,0.0750555349946381));
#77773=CARTESIAN_POINT('Ctrl Pts',(-2.29922182808404,226.184803560304,0.0375277674973117));
#77774=CARTESIAN_POINT('Ctrl Pts',(-1.91346599666503,226.635987203375,-1.50573997714787E-14));
#77775=CARTESIAN_POINT('',(1.91712510374251,226.63873942345,1.67669336393566E-15));
#77776=CARTESIAN_POINT('Origin',(0.,225.,0.));
#77777=CARTESIAN_POINT('Ctrl Pts',(1.91712867315962,226.638742108209,1.44285430635494E-15));
#77778=CARTESIAN_POINT('Ctrl Pts',(1.38658202527179,227.257482867444,0.0517556153419835));
#77779=CARTESIAN_POINT('Ctrl Pts',(0.527608291324034,227.597070351188,0.103511230683964));
#77780=CARTESIAN_POINT('Ctrl Pts',(-0.282369177537283,227.505702430347,
0.155266846025946));
#77781=CARTESIAN_POINT('Ctrl Pts',(-1.1105581768861,227.412280193503,0.208186134436544));
#77782=CARTESIAN_POINT('Ctrl Pts',(-1.88752287836714,226.868305491623,0.261105422847144));
#77783=CARTESIAN_POINT('Ctrl Pts',(-2.25823175842065,226.122142534186,0.314024711257743));
#77784=CARTESIAN_POINT('Ctrl Pts',(-2.42960632929949,225.777199740752,0.338488706674499));
#77785=CARTESIAN_POINT('Ctrl Pts',(-2.51415958122241,225.389047102439,0.362952702091256));
#77786=CARTESIAN_POINT('Ctrl Pts',(-2.51347389046773,225.0005858313,0.387416697508012));
#77787=CARTESIAN_POINT('Origin',(0.,225.,10.));
#77788=CARTESIAN_POINT('',(-2.51741847158745,224.997698802423,1.38741669750801));
#77789=CARTESIAN_POINT('',(-2.52168717967801,225.000137595091,1.11258330249197));
#77790=CARTESIAN_POINT('',(-2.5175,225.,10.));
#77791=CARTESIAN_POINT('Ctrl Pts',(-2.52168717967801,225.000137595091,1.11258330249197));
#77792=CARTESIAN_POINT('Ctrl Pts',(-2.52169204710937,225.006846738092,1.11215722053549));
#77793=CARTESIAN_POINT('Ctrl Pts',(-2.52166759919164,225.013555842314,1.11173113857901));
#77794=CARTESIAN_POINT('Ctrl Pts',(-2.52161372912346,225.020264707836,1.11130505662253));
#77795=CARTESIAN_POINT('Ctrl Pts',(-2.51492307810834,225.853504379485,1.05838576821194));
#77796=CARTESIAN_POINT('Ctrl Pts',(-2.05437847998888,226.683061975931,1.00546647980134));
#77797=CARTESIAN_POINT('Ctrl Pts',(-1.3507129006363,227.129421042381,0.952547191390737));
#77798=CARTESIAN_POINT('Ctrl Pts',(-0.647047321283738,227.575780108832,
0.899627902980141));
#77799=CARTESIAN_POINT('Ctrl Pts',(0.299739239301934,227.638940645286,0.846708614569544));
#77800=CARTESIAN_POINT('Ctrl Pts',(1.05637242882409,227.289819467046,0.793789326158948));
#77801=CARTESIAN_POINT('Ctrl Pts',(1.81300561834626,226.940698288805,0.740870037748351));
#77802=CARTESIAN_POINT('Ctrl Pts',(2.37948543680491,226.179295395871,0.687950749337752));
#77803=CARTESIAN_POINT('Ctrl Pts',(2.49664115114991,225.35439625556,0.635031460927153));
#77804=CARTESIAN_POINT('Ctrl Pts',(2.61379686549491,224.52949711525,0.582112172516556));
#77805=CARTESIAN_POINT('Ctrl Pts',(2.28162847572628,223.641101727564,0.529192884105959));
#77806=CARTESIAN_POINT('Ctrl Pts',(1.65203466276087,223.094991627842,0.476273595695361));
#77807=CARTESIAN_POINT('Ctrl Pts',(1.02244084979547,222.548881528121,0.423354307284765));
#77808=CARTESIAN_POINT('Ctrl Pts',(0.0954216136332989,222.345056716363,
0.370435018874169));
#77809=CARTESIAN_POINT('Ctrl Pts',(-0.704614902137573,222.578323517273,
0.317515730463573));
#77810=CARTESIAN_POINT('Ctrl Pts',(-1.50465141790847,222.811590318182,0.264596442052974));
#77811=CARTESIAN_POINT('Ctrl Pts',(-2.17770521328806,223.48194873176,0.211677153642374));
#77812=CARTESIAN_POINT('Ctrl Pts',(-2.41590098767414,224.278990281059,0.158757865231776));
#77813=CARTESIAN_POINT('Ctrl Pts',(-2.48517998504973,224.510809000532,0.143366344318505));
#77814=CARTESIAN_POINT('Ctrl Pts',(-2.51767298237096,224.75334424267,0.127974823405235));
#77815=CARTESIAN_POINT('Ctrl Pts',(-2.51553408751311,224.996405665924,0.112583302491965));
#77816=CARTESIAN_POINT('Ctrl Pts',(-2.51347389046773,225.0005858313,0.387416697508012));
#77817=CARTESIAN_POINT('Ctrl Pts',(-2.51267632935821,224.54874715578,0.415871990501853));
#77818=CARTESIAN_POINT('Ctrl Pts',(-2.39655750155179,224.096490925473,0.444327283495693));
#77819=CARTESIAN_POINT('Ctrl Pts',(-2.16760750705151,223.711328458468,0.472782576489533));
#77820=CARTESIAN_POINT('Ctrl Pts',(-1.74182131700286,222.995028553183,0.525701864900131));
#77821=CARTESIAN_POINT('Ctrl Pts',(-0.925795878279577,222.510779955607,
0.578621153310729));
#77822=CARTESIAN_POINT('Ctrl Pts',(-0.0930673453572587,222.480039920553,
0.631540441721328));
#77823=CARTESIAN_POINT('Ctrl Pts',(0.739661187565012,222.449299885498,0.684459730131924));
#77824=CARTESIAN_POINT('Ctrl Pts',(1.5890928146863,222.872068412965,0.73737901854252));
#77825=CARTESIAN_POINT('Ctrl Pts',(2.06658816412527,223.554953044849,0.790298306953116));
#77826=CARTESIAN_POINT('Ctrl Pts',(2.54408351356428,224.237837676734,0.843217595363715));
#77827=CARTESIAN_POINT('Ctrl Pts',(2.64964258532089,225.180838413036,0.896136883774315));
#77828=CARTESIAN_POINT('Ctrl Pts',(2.33493175115268,225.952405437576,0.949056172184913));
#77829=CARTESIAN_POINT('Ctrl Pts',(2.02022091698448,226.723972462116,1.00197546059551));
#77830=CARTESIAN_POINT('Ctrl Pts',(1.28524017689151,227.324105774894,1.05489474900611));
#77831=CARTESIAN_POINT('Ctrl Pts',(0.466331374739214,227.478200482608,1.1078140374167));
#77832=CARTESIAN_POINT('Ctrl Pts',(-0.352577427413085,227.632295190321,
1.1607333258273));
#77833=CARTESIAN_POINT('Ctrl Pts',(-1.2554142916247,227.34035129297,1.2136526142379));
#77834=CARTESIAN_POINT('Ctrl Pts',(-1.82904831020792,226.735954385945,1.2665719026485));
#77835=CARTESIAN_POINT('Ctrl Pts',(-2.26569241095164,226.275893902412,1.306853500935));
#77836=CARTESIAN_POINT('Ctrl Pts',(-2.5115933498986,225.634795266357,1.34713509922151));
#77837=CARTESIAN_POINT('Ctrl Pts',(-2.51741847158745,224.997698802423,1.38741669750801));
#77838=CARTESIAN_POINT('Origin',(0.,225.,10.));
#77839=CARTESIAN_POINT('',(-2.52129908879481,225.000905510379,2.38741669750801));
#77840=CARTESIAN_POINT('',(-2.51578353683605,225.002114845881,2.11258330249197));
#77841=CARTESIAN_POINT('',(-2.5175,225.,10.));
#77842=CARTESIAN_POINT('Ctrl Pts',(-2.51578353683605,225.002114845881,2.11258330249197));
#77843=CARTESIAN_POINT('Ctrl Pts',(-2.51783260554419,225.259450106344,2.09633961766574));
#77844=CARTESIAN_POINT('Ctrl Pts',(-2.48151008120921,225.516220723336,2.08009593283951));
#77845=CARTESIAN_POINT('Ctrl Pts',(-2.40441272483833,225.760101241637,2.06385224801329));
#77846=CARTESIAN_POINT('Ctrl Pts',(-2.15324205259667,226.554624382399,2.01093295960269));
#77847=CARTESIAN_POINT('Ctrl Pts',(-1.46930744293435,227.21233837926,1.95801367119209));
#77848=CARTESIAN_POINT('Ctrl Pts',(-0.665577185407848,227.432274590025,
1.9050943827815));
#77849=CARTESIAN_POINT('Ctrl Pts',(0.138153072118675,227.65221080079,1.8521750943709));
#77850=CARTESIAN_POINT('Ctrl Pts',(1.06167897750938,227.434369225459,1.7992558059603));
#77851=CARTESIAN_POINT('Ctrl Pts',(1.68239474048309,226.878431585785,1.7463365175497));
#77852=CARTESIAN_POINT('Ctrl Pts',(2.30311050345679,226.322493946112,1.6934172291391));
#77853=CARTESIAN_POINT('Ctrl Pts',(2.62101612401351,225.428460242096,1.64049794072851));
#77854=CARTESIAN_POINT('Ctrl Pts',(2.49063871562429,224.605445516318,1.58757865231791));
#77855=CARTESIAN_POINT('Ctrl Pts',(2.36026130723508,223.78243079054,1.53465936390731));
#77856=CARTESIAN_POINT('Ctrl Pts',(1.78160086989994,223.030435043,1.48174007549672));
#77857=CARTESIAN_POINT('Ctrl Pts',(1.01945094781155,222.693560877067,1.42882078708612));
#77858=CARTESIAN_POINT('Ctrl Pts',(0.257301025723131,222.356686711134,1.37590149867552));
#77859=CARTESIAN_POINT('Ctrl Pts',(-0.688338381118543,222.434934126809,
1.32298221026492));
#77860=CARTESIAN_POINT('Ctrl Pts',(-1.38473973258398,222.892518708072,1.27006292185432));
#77861=CARTESIAN_POINT('Ctrl Pts',(-2.07553397822393,223.346419027141,1.2175697154002));
#77862=CARTESIAN_POINT('Ctrl Pts',(-2.52108751316975,224.173572603789,1.16507650894609));
#77863=CARTESIAN_POINT('Ctrl Pts',(-2.52168717967801,225.000137595091,1.11258330249197));
#77864=CARTESIAN_POINT('Ctrl Pts',(-2.51741847158745,224.997698802423,1.38741669750801));
#77865=CARTESIAN_POINT('Ctrl Pts',(-2.5192460078812,224.797820246635,1.4000543876321));
#77866=CARTESIAN_POINT('Ctrl Pts',(-2.49744317904368,224.598335619689,1.4126920777562));
#77867=CARTESIAN_POINT('Ctrl Pts',(-2.45048657256469,224.404959042237,1.42532976788029));
#77868=CARTESIAN_POINT('Ctrl Pts',(-2.25385964338344,223.595210522252,1.47824905629088));
#77869=CARTESIAN_POINT('Ctrl Pts',(-1.61617461206615,222.892563398979,1.53116834470149));
#77870=CARTESIAN_POINT('Ctrl Pts',(-0.829237887491455,222.618547060792,
1.58408763311208));
#77871=CARTESIAN_POINT('Ctrl Pts',(-0.0423011629167494,222.344530722605,
1.63700692152268));
#77872=CARTESIAN_POINT('Ctrl Pts',(0.893887254915367,222.499145169502,1.68992620993328));
#77873=CARTESIAN_POINT('Ctrl Pts',(1.55092842656392,223.011639779642,1.74284549834387));
#77874=CARTESIAN_POINT('Ctrl Pts',(2.20796959821247,223.524134389781,1.79576478675447));
#77875=CARTESIAN_POINT('Ctrl Pts',(2.58586352367745,224.394509163162,1.84868407516507));
#77876=CARTESIAN_POINT('Ctrl Pts',(2.5116855256137,225.224480154825,1.90160336357567));
#77877=CARTESIAN_POINT('Ctrl Pts',(2.43750752754995,226.054451146488,1.95452265198626));
#77878=CARTESIAN_POINT('Ctrl Pts',(1.91125760595749,226.844018356432,2.00744194039686));
#77879=CARTESIAN_POINT('Ctrl Pts',(1.17374792360493,227.231876074238,2.06036122880746));
#77880=CARTESIAN_POINT('Ctrl Pts',(0.436238241252373,227.619733792044,2.11328051721805));
#77881=CARTESIAN_POINT('Ctrl Pts',(-0.512531201860274,227.60588201771,2.16619980562865));
#77882=CARTESIAN_POINT('Ctrl Pts',(-1.23840363011865,227.196659209991,2.21911909403925));
#77883=CARTESIAN_POINT('Ctrl Pts',(-1.96427605837704,226.787436402272,2.27203838244985));
#77884=CARTESIAN_POINT('Ctrl Pts',(-2.46725147178114,225.982842561167,2.32495767086044));
#77885=CARTESIAN_POINT('Ctrl Pts',(-2.51716828038405,225.151059868138,2.37787695927104));
#77886=CARTESIAN_POINT('Ctrl Pts',(-2.52016777453195,225.101078160775,2.3810568720167));
#77887=CARTESIAN_POINT('Ctrl Pts',(-2.52153136850561,225.050998280136,2.38423678476236));
#77888=CARTESIAN_POINT('Ctrl Pts',(-2.52129908879481,225.000905510379,2.38741669750801));
#77889=CARTESIAN_POINT('Origin',(0.,225.,10.));
#77890=CARTESIAN_POINT('',(-2.51474241101028,225.001726207962,3.38741669750801));
#77891=CARTESIAN_POINT('',(-2.51418867251095,224.99863370625,3.11258330249198));
#77892=CARTESIAN_POINT('',(-2.5175,225.,10.));
#77893=CARTESIAN_POINT('Ctrl Pts',(-2.51418867251095,224.99863370625,3.11258330249198));
#77894=CARTESIAN_POINT('Ctrl Pts',(-2.51168135695882,225.507365063915,3.080522014796));
#77895=CARTESIAN_POINT('Ctrl Pts',(-2.36190809597984,226.01745378504,3.04846072710002));
#77896=CARTESIAN_POINT('Ctrl Pts',(-2.07504550059781,226.432878388949,3.01639943940404));
#77897=CARTESIAN_POINT('Ctrl Pts',(-1.60155970167469,227.118564336299,2.96348015099344));
#77898=CARTESIAN_POINT('Ctrl Pts',(-0.754591850175153,227.546350214638,
2.91056086258285));
#77899=CARTESIAN_POINT('Ctrl Pts',(0.0782855841932958,227.520481232549,
2.85764157417225));
#77900=CARTESIAN_POINT('Ctrl Pts',(0.911163018561756,227.49461225046,2.80472228576165));
#77901=CARTESIAN_POINT('Ctrl Pts',(1.72995003579915,227.015088407943,2.75180299735105));
#77902=CARTESIAN_POINT('Ctrl Pts',(2.15996970786875,226.301339769147,2.69888370894046));
#77903=CARTESIAN_POINT('Ctrl Pts',(2.58998937993835,225.58759113035,2.64596442052986));
#77904=CARTESIAN_POINT('Ctrl Pts',(2.63124170684017,224.639617695274,2.59304513211926));
#77905=CARTESIAN_POINT('Ctrl Pts',(2.26484963484653,223.891212163822,2.54012584370866));
#77906=CARTESIAN_POINT('Ctrl Pts',(1.89845756285288,223.14280663237,2.48720655529807));
#77907=CARTESIAN_POINT('Ctrl Pts',(1.12442109196377,222.593969004542,2.43428726688747));
#77908=CARTESIAN_POINT('Ctrl Pts',(0.296939275219781,222.495847216434,2.38136797847687));
#77909=CARTESIAN_POINT('Ctrl Pts',(-0.530542541524199,222.397725428326,
2.32844869006628));
#77910=CARTESIAN_POINT('Ctrl Pts',(-1.41146970412308,222.750319479939,2.27552940165568));
#77911=CARTESIAN_POINT('Ctrl Pts',(-1.94272991801202,223.392282648076,2.22261011324508));
#77912=CARTESIAN_POINT('Ctrl Pts',(-2.31091871249395,223.83719389646,2.18593450966071));
#77913=CARTESIAN_POINT('Ctrl Pts',(-2.51115707230781,224.421093599656,2.14925890607634));
#77914=CARTESIAN_POINT('Ctrl Pts',(-2.51578353683605,225.002114845881,2.11258330249197));
#77915=CARTESIAN_POINT('Ctrl Pts',(-2.52129908879481,225.000905510379,2.38741669750801));
#77916=CARTESIAN_POINT('Ctrl Pts',(-2.51766582941986,224.217367315361,2.43715607317295));
#77917=CARTESIAN_POINT('Ctrl Pts',(-2.12357956846045,223.430675615842,2.4868954488379));
#77918=CARTESIAN_POINT('Ctrl Pts',(-1.49222059474684,222.967210567987,2.53663482450284));
#77919=CARTESIAN_POINT('Ctrl Pts',(-0.820497896705034,222.474115505819,
2.58955411291343));
#77920=CARTESIAN_POINT('Ctrl Pts',(0.119805703180309,222.346896926438,2.64247340132403));
#77921=CARTESIAN_POINT('Ctrl Pts',(0.898407308371105,222.643770062743,2.69539268973463));
#77922=CARTESIAN_POINT('Ctrl Pts',(1.67700891356191,222.940643199048,2.74831197814523));
#77923=CARTESIAN_POINT('Ctrl Pts',(2.29390852405818,223.661608051039,2.80123126655583));
#77924=CARTESIAN_POINT('Ctrl Pts',(2.46681288417962,224.476751109985,2.85415055496642));
#77925=CARTESIAN_POINT('Ctrl Pts',(2.63971724430104,225.291894168932,2.90706984337702));
#77926=CARTESIAN_POINT('Ctrl Pts',(2.3686263540477,226.201215434834,2.95998913178762));
#77927=CARTESIAN_POINT('Ctrl Pts',(1.7775914024464,226.78860951756,3.01290842019821));
#77928=CARTESIAN_POINT('Ctrl Pts',(1.18655645084507,227.376003600287,3.06582770860881));
#77929=CARTESIAN_POINT('Ctrl Pts',(0.275577437895753,227.641470499838,3.11874699701941));
#77930=CARTESIAN_POINT('Ctrl Pts',(-0.538481659453402,227.463532566591,
3.17166628543));
#77931=CARTESIAN_POINT('Ctrl Pts',(-1.35254075680253,227.285594633344,3.2245855738406));
#77932=CARTESIAN_POINT('Ctrl Pts',(-2.06967993855152,226.664251867297,3.2775048622512));
#77933=CARTESIAN_POINT('Ctrl Pts',(-2.36173632851075,225.88383070677,3.33042415066179));
#77934=CARTESIAN_POINT('Ctrl Pts',(-2.46658176380421,225.603667015439,3.3494216662772));
#77935=CARTESIAN_POINT('Ctrl Pts',(-2.51664503896433,225.30300223997,3.36841918189261));
#77936=CARTESIAN_POINT('Ctrl Pts',(-2.51474241101028,225.001726207962,3.38741669750801));
#77937=CARTESIAN_POINT('Origin',(0.,225.,10.));
#77938=CARTESIAN_POINT('',(-2.5150539014468,224.998127144802,4.38741669750802));
#77939=CARTESIAN_POINT('',(-2.52076226691227,224.998630464431,4.11258330249197));
#77940=CARTESIAN_POINT('',(-2.5175,225.,10.));
#77941=CARTESIAN_POINT('Ctrl Pts',(-2.52076226691227,224.998630464431,4.11258330249197));
#77942=CARTESIAN_POINT('Ctrl Pts',(-2.51581102366626,225.753285751347,4.06470441192625));
#77943=CARTESIAN_POINT('Ctrl Pts',(-2.15430412856549,226.512055249875,4.01682552136052));
#77944=CARTESIAN_POINT('Ctrl Pts',(-1.56257689974821,226.979218970693,3.9689466307948));
#77945=CARTESIAN_POINT('Ctrl Pts',(-0.908556234018705,227.495562841339,
3.9160273423842));
#77946=CARTESIAN_POINT('Ctrl Pts',(0.0267085919674362,227.655672226725,
3.8631080539736));
#77947=CARTESIAN_POINT('Ctrl Pts',(0.815240412263574,227.386281075505,3.810188765563));
#77948=CARTESIAN_POINT('Ctrl Pts',(1.60377223255971,227.116889924285,3.75726947715241));
#77949=CARTESIAN_POINT('Ctrl Pts',(2.24557104716584,226.417998236458,3.70435018874181));
#77950=CARTESIAN_POINT('Ctrl Pts',(2.44694973106533,225.609418834108,3.65143090033121));
#77951=CARTESIAN_POINT('Ctrl Pts',(2.64832841496483,224.800839431759,3.59851161192062));
#77952=CARTESIAN_POINT('Ctrl Pts',(2.40928696815766,223.882572314887,3.54559232351002));
#77953=CARTESIAN_POINT('Ctrl Pts',(1.83921075214889,223.274816499182,3.49267303509942));
#77954=CARTESIAN_POINT('Ctrl Pts',(1.26913453614011,222.667060683477,3.43975374668882));
#77955=CARTESIAN_POINT('Ctrl Pts',(0.368023550929722,222.36981616894,3.38683445827822));
#77956=CARTESIAN_POINT('Ctrl Pts',(-0.451773834664424,222.519102037416,
3.33391516986763));
#77957=CARTESIAN_POINT('Ctrl Pts',(-1.27157122025857,222.668387905892,3.28099588145703));
#77958=CARTESIAN_POINT('Ctrl Pts',(-2.01005500623649,223.264204157383,3.22807659304643));
#77959=CARTESIAN_POINT('Ctrl Pts',(-2.32929502605208,224.033905291309,3.17515730463584));
#77960=CARTESIAN_POINT('Ctrl Pts',(-2.45512265453008,224.337281003336,3.15429930392122));
#77961=CARTESIAN_POINT('Ctrl Pts',(-2.51581984809172,224.667670111702,3.1334413032066));
#77962=CARTESIAN_POINT('Ctrl Pts',(-2.51418867251095,224.99863370625,3.11258330249198));
#77963=CARTESIAN_POINT('Ctrl Pts',(-2.51474241101028,225.001726207962,3.38741669750801));
#77964=CARTESIAN_POINT('Ctrl Pts',(-2.51134509767322,224.46377075561,3.4213384703032));
#77965=CARTESIAN_POINT('Ctrl Pts',(-2.34226326168293,223.923866414815,3.4552602430984));
#77966=CARTESIAN_POINT('Ctrl Pts',(-2.02353000223652,223.495247019255,3.48918201589359));
#77967=CARTESIAN_POINT('Ctrl Pts',(-1.52629368783361,222.826584047275,3.54210130430419));
#77968=CARTESIAN_POINT('Ctrl Pts',(-0.664847460858349,222.428757658323,
3.59502059271478));
#77969=CARTESIAN_POINT('Ctrl Pts',(0.166610902338107,222.483813200354,3.64793988112538));
#77970=CARTESIAN_POINT('Ctrl Pts',(0.998069265534564,222.538868742386,3.70085916953598));
#77971=CARTESIAN_POINT('Ctrl Pts',(1.79953976495221,223.046806215399,3.75377845794658));
#77972=CARTESIAN_POINT('Ctrl Pts',(2.20426951572994,223.775193441637,3.80669774635718));
#77973=CARTESIAN_POINT('Ctrl Pts',(2.60899926650765,224.503580667874,3.85961703476777));
#77974=CARTESIAN_POINT('Ctrl Pts',(2.61698826864545,225.452417647336,3.91253632317837));
#77975=CARTESIAN_POINT('Ctrl Pts',(2.22458075496457,226.187516596923,3.96545561158897));
#77976=CARTESIAN_POINT('Ctrl Pts',(1.83217324128368,226.922615546509,4.01837489999956));
#77977=CARTESIAN_POINT('Ctrl Pts',(1.0393692117841,227.443976466221,4.07129418841016));
#77978=CARTESIAN_POINT('Ctrl Pts',(0.208955774755814,227.513024609426,4.12421347682076));
#77979=CARTESIAN_POINT('Ctrl Pts',(-0.621457662272467,227.58207275263,4.17713276523136));
#77980=CARTESIAN_POINT('Ctrl Pts',(-1.48948050682944,227.198808119328,4.23005205364195));
#77981=CARTESIAN_POINT('Ctrl Pts',(-1.99790552230265,226.538612598193,4.28297134205255));
#77982=CARTESIAN_POINT('Ctrl Pts',(-2.33239371528771,226.104275970056,4.3177864605377));
#77983=CARTESIAN_POINT('Ctrl Pts',(-2.51124061715918,225.550077992808,4.35260157902286));
#77984=CARTESIAN_POINT('Ctrl Pts',(-2.5150539014468,224.998127144802,4.38741669750802));
#77985=CARTESIAN_POINT('Origin',(0.,225.,10.));
#77986=CARTESIAN_POINT('',(-2.52148472081105,224.999338741875,5.38741669750802));
#77987=CARTESIAN_POINT('',(-2.51831101426404,225.002238014691,5.11258330249197));
#77988=CARTESIAN_POINT('',(-2.5175,225.,10.));
#77989=CARTESIAN_POINT('Ctrl Pts',(-2.51831101426404,225.002238014691,5.11258330249197));
#77990=CARTESIAN_POINT('Ctrl Pts',(-2.51987982331657,225.172535980322,5.1018060974671));
#77991=CARTESIAN_POINT('Ctrl Pts',(-2.50407981832776,225.342544535845,5.09102889244222));
#77992=CARTESIAN_POINT('Ctrl Pts',(-2.46984258279024,225.50875526306,5.08025168741734));
#77993=CARTESIAN_POINT('Ctrl Pts',(-2.3017275531875,226.324899466508,5.02733239900675));
#77994=CARTESIAN_POINT('Ctrl Pts',(-1.68907196797494,227.049474130712,4.97441311059615));
#77995=CARTESIAN_POINT('Ctrl Pts',(-0.912227010900041,227.350913903579,
4.92149382218555));
#77996=CARTESIAN_POINT('Ctrl Pts',(-0.135382053825148,227.652353676446,
4.86857453377495));
#77997=CARTESIAN_POINT('Ctrl Pts',(0.805652275112092,227.530658557975,4.81565524536436));
#77998=CARTESIAN_POINT('Ctrl Pts',(1.48025868549315,227.041516231988,4.76273595695376));
#77999=CARTESIAN_POINT('Ctrl Pts',(2.15486509587421,226.552373906002,4.70981666854316));
#78000=CARTESIAN_POINT('Ctrl Pts',(2.56304358769908,225.695784372502,4.65689738013257));
#78001=CARTESIAN_POINT('Ctrl Pts',(2.51801169113329,224.863722985166,4.60397809172197));
#78002=CARTESIAN_POINT('Ctrl Pts',(2.4729797945675,224.031661597831,4.55105880331137));
#78003=CARTESIAN_POINT('Ctrl Pts',(1.97473750961105,223.224128356661,4.49813951490077));
#78004=CARTESIAN_POINT('Ctrl Pts',(1.25128049606563,222.810650456954,4.44522022649017));
#78005=CARTESIAN_POINT('Ctrl Pts',(0.527823482520219,222.397172557246,4.39230093807958));
#78006=CARTESIAN_POINT('Ctrl Pts',(-0.420848259614152,222.377749999001,
4.33938164966898));
#78007=CARTESIAN_POINT('Ctrl Pts',(-1.16062255979383,222.761270544458,4.28646236125838));
#78008=CARTESIAN_POINT('Ctrl Pts',(-1.90039685997351,223.144791089915,4.23354307284779));
#78009=CARTESIAN_POINT('Ctrl Pts',(-2.43127371819849,223.931254739075,4.18062378443719));
#78010=CARTESIAN_POINT('Ctrl Pts',(-2.51032389457454,224.760775741608,4.12770449602659));
#78011=CARTESIAN_POINT('Ctrl Pts',(-2.51785317833117,224.839785040467,4.12266409818172));
#78012=CARTESIAN_POINT('Ctrl Pts',(-2.52128350363041,224.919184954378,4.11762370033684));
#78013=CARTESIAN_POINT('Ctrl Pts',(-2.52076226691227,224.998630464431,4.11258330249197));
#78014=CARTESIAN_POINT('Ctrl Pts',(-2.5150539014468,224.998127144802,4.38741669750802));
#78015=CARTESIAN_POINT('Ctrl Pts',(-2.51703684304577,224.711107815914,4.40552086743346));
#78016=CARTESIAN_POINT('Ctrl Pts',(-2.47168908238452,224.424696131468,4.4236250373589));
#78017=CARTESIAN_POINT('Ctrl Pts',(-2.37628376391044,224.156062397605,4.44172920728435));
#78018=CARTESIAN_POINT('Ctrl Pts',(-2.0974098036556,223.370834127117,4.49464849569494));
#78019=CARTESIAN_POINT('Ctrl Pts',(-1.39083469675649,222.73750399511,4.54756778410554));
#78020=CARTESIAN_POINT('Ctrl Pts',(-0.579887198234946,222.545883857538,
4.60048707251614));
#78021=CARTESIAN_POINT('Ctrl Pts',(0.231060300286584,222.354263719967,4.65340636092673));
#78022=CARTESIAN_POINT('Ctrl Pts',(1.14638019043053,222.604353576832,4.70632564933733));
#78023=CARTESIAN_POINT('Ctrl Pts',(1.74722210846285,223.181712314548,4.75924493774793));
#78024=CARTESIAN_POINT('Ctrl Pts',(2.34806402649518,223.759071052265,4.81216422615853));
#78025=CARTESIAN_POINT('Ctrl Pts',(2.63442797241588,224.663698670832,4.86508351456912));
#78026=CARTESIAN_POINT('Ctrl Pts',(2.47527381020271,225.481637589781,4.91800280297972));
#78027=CARTESIAN_POINT('Ctrl Pts',(2.31611964798954,226.29957650873,4.97092209139032));
#78028=CARTESIAN_POINT('Ctrl Pts',(1.71144737764256,227.030826728061,5.02384137980092));
#78029=CARTESIAN_POINT('Ctrl Pts',(0.937955018183124,227.340768161786,5.07676066821151));
#78030=CARTESIAN_POINT('Ctrl Pts',(0.164462658723686,227.650709595511,5.12967995662211));
#78031=CARTESIAN_POINT('Ctrl Pts',(-0.777849789848224,227.539342243629,
5.18259924503271));
#78032=CARTESIAN_POINT('Ctrl Pts',(-1.45778016959366,227.057627804173,5.23551853344331));
#78033=CARTESIAN_POINT('Ctrl Pts',(-2.10833172635816,226.596727559325,5.28615125479821));
#78034=CARTESIAN_POINT('Ctrl Pts',(-2.51868566269795,225.796793135942,5.33678397615311));
#78035=CARTESIAN_POINT('Ctrl Pts',(-2.52148472081105,224.999338741875,5.38741669750802));
#78036=CARTESIAN_POINT('Origin',(0.,225.,10.));
#78037=CARTESIAN_POINT('',(-2.51699557978349,225.002292230688,6.38741669750802));
#78038=CARTESIAN_POINT('',(-2.51344096553148,224.999964780717,6.11258330249198));
#78039=CARTESIAN_POINT('',(-2.5175,225.,10.));
#78040=CARTESIAN_POINT('Ctrl Pts',(-2.51344096553148,224.999964780717,6.11258330249198));
#78041=CARTESIAN_POINT('Ctrl Pts',(-2.5133882653449,225.422270773897,6.08598849459735));
#78042=CARTESIAN_POINT('Ctrl Pts',(-2.41266885591251,225.844600385848,6.05939368670273));
#78043=CARTESIAN_POINT('Ctrl Pts',(-2.21142314859194,226.211842382213,6.0327988788081));
#78044=CARTESIAN_POINT('Ctrl Pts',(-1.8109773296453,226.942593482169,5.9798795903975));
#78045=CARTESIAN_POINT('Ctrl Pts',(-1.01250319828182,227.455228217279,5.9269603019869));
#78046=CARTESIAN_POINT('Ctrl Pts',(-0.181382501313819,227.515164942836,
5.87404101357631));
#78047=CARTESIAN_POINT('Ctrl Pts',(0.649738195654195,227.575101668393,5.82112172516571));
#78048=CARTESIAN_POINT('Ctrl Pts',(1.51350545822674,227.182340384398,5.76820243675511));
#78049=CARTESIAN_POINT('Ctrl Pts',(2.01465940403403,226.516608646683,5.71528314834452));
#78050=CARTESIAN_POINT('Ctrl Pts',(2.51581334984132,225.850876908968,5.66236385993392));
#78051=CARTESIAN_POINT('Ctrl Pts',(2.65435397888336,224.912174717534,5.60944457152332));
#78052=CARTESIAN_POINT('Ctrl Pts',(2.36688510203449,224.130052176724,5.55652528311272));
#78053=CARTESIAN_POINT('Ctrl Pts',(2.07941622518562,223.347929635915,5.50360599470212));
#78054=CARTESIAN_POINT('Ctrl Pts',(1.36593784244583,222.722386745729,5.45068670629153));
#78055=CARTESIAN_POINT('Ctrl Pts',(0.552937647728462,222.539671920418,5.39776741788093));
#78056=CARTESIAN_POINT('Ctrl Pts',(-0.260062546988908,222.356957095107,
5.34484812947033));
#78057=CARTESIAN_POINT('Ctrl Pts',(-1.17258455368387,222.617070334669,5.29192884105973));
#78058=CARTESIAN_POINT('Ctrl Pts',(-1.76705832003488,223.200983825795,5.23900955264914));
#78059=CARTESIAN_POINT('Ctrl Pts',(-2.24046534769195,223.66598121658,5.19686746926341));
#78060=CARTESIAN_POINT('Ctrl Pts',(-2.51217650334442,224.336322218207,5.15472538587769));
#78061=CARTESIAN_POINT('Ctrl Pts',(-2.51831101426404,225.002238014691,5.11258330249197));
#78062=CARTESIAN_POINT('Ctrl Pts',(-2.52148472081105,224.999338741875,5.38741669750802));
#78063=CARTESIAN_POINT('Ctrl Pts',(-2.52161112590833,224.963325806029,5.38970326456371));
#78064=CARTESIAN_POINT('Ctrl Pts',(-2.52090635798137,224.927317927988,5.39198983161941));
#78065=CARTESIAN_POINT('Ctrl Pts',(-2.51935500348403,224.891346561095,5.3942763986751));
#78066=CARTESIAN_POINT('Ctrl Pts',(-2.48345114670998,224.058841284505,5.4471956870857));
#78067=CARTESIAN_POINT('Ctrl Pts',(-1.99409512224288,223.245892258356,5.50011497549629));
#78068=CARTESIAN_POINT('Ctrl Pts',(-1.2752162372571,222.82450494103,5.55303426390689));
#78069=CARTESIAN_POINT('Ctrl Pts',(-0.556337352271339,222.403117623704,
5.60595355231749));
#78070=CARTESIAN_POINT('Ctrl Pts',(0.392064393233094,222.373292015201,5.65887284072809));
#78071=CARTESIAN_POINT('Ctrl Pts',(1.13600037916085,222.748676313385,5.71179212913868));
#78072=CARTESIAN_POINT('Ctrl Pts',(1.87993636508862,223.124060611569,5.76471141754928));
#78073=CARTESIAN_POINT('Ctrl Pts',(2.41940659143971,223.904654816441,5.81763070595988));
#78074=CARTESIAN_POINT('Ctrl Pts',(2.50754949324294,224.733259035199,5.87054999437047));
#78075=CARTESIAN_POINT('Ctrl Pts',(2.59569239504618,225.561863253957,5.92346928278107));
#78076=CARTESIAN_POINT('Ctrl Pts',(2.23250797230156,226.438477486601,5.97638857119167));
#78077=CARTESIAN_POINT('Ctrl Pts',(1.58418940971608,226.961963077509,6.02930785960227));
#78078=CARTESIAN_POINT('Ctrl Pts',(0.935870847130601,227.485448668418,6.08222714801287));
#78079=CARTESIAN_POINT('Ctrl Pts',(0.00241814470426038,227.65580561759,
6.13514643642346));
#78080=CARTESIAN_POINT('Ctrl Pts',(-0.789020759286212,227.395078588435,
6.18806572483406));
#78081=CARTESIAN_POINT('Ctrl Pts',(-1.58045966327668,227.13435155928,6.24098501324466));
#78082=CARTESIAN_POINT('Ctrl Pts',(-2.22988476883129,226.442540551798,6.29390430165526));
#78083=CARTESIAN_POINT('Ctrl Pts',(-2.44011916041725,225.63621826941,6.34682359006585));
#78084=CARTESIAN_POINT('Ctrl Pts',(-2.4938744010362,225.430048156236,6.36035462587991));
#78085=CARTESIAN_POINT('Ctrl Pts',(-2.51891606819546,225.216391482443,6.37388566169396));
#78086=CARTESIAN_POINT('Ctrl Pts',(-2.51699557978349,225.002292230688,6.38741669750802));
#78087=CARTESIAN_POINT('Origin',(0.,225.,10.));
#78088=CARTESIAN_POINT('',(-2.51364339850779,224.999260136873,7.38741669750802));
#78089=CARTESIAN_POINT('',(-2.51844027096952,224.997780461794,7.11258330249198));
#78090=CARTESIAN_POINT('',(-2.5175,225.,10.));
#78091=CARTESIAN_POINT('Ctrl Pts',(-2.51844027096952,224.997780461794,7.11258330249198));
#78092=CARTESIAN_POINT('Ctrl Pts',(-2.51228349286758,225.667879389382,7.0701708917276));
#78093=CARTESIAN_POINT('Ctrl Pts',(-2.23669063730925,226.342450530656,7.02775848096323));
#78094=CARTESIAN_POINT('Ctrl Pts',(-1.75786844049796,226.807996915748,6.98534607019885));
#78095=CARTESIAN_POINT('Ctrl Pts',(-1.1604270436572,227.388873668029,6.93242678178825));
#78096=CARTESIAN_POINT('Ctrl Pts',(-0.246591469036519,227.644333748386,
6.87950749337766));
#78097=CARTESIAN_POINT('Ctrl Pts',(0.565467142385517,227.45747862907,6.82658820496706));
#78098=CARTESIAN_POINT('Ctrl Pts',(1.37752575380754,227.270623509755,6.77366891655647));
#78099=CARTESIAN_POINT('Ctrl Pts',(2.08780740203091,226.641453190767,6.72074962814587));
#78100=CARTESIAN_POINT('Ctrl Pts',(2.37128721879421,225.857875997705,6.66783033973527));
#78101=CARTESIAN_POINT('Ctrl Pts',(2.65476703555751,225.074298804643,6.61491105132467));
#78102=CARTESIAN_POINT('Ctrl Pts',(2.51144502086071,224.136314737507,6.56199176291408));
#78103=CARTESIAN_POINT('Ctrl Pts',(2.00690532581108,223.473145286975,6.50907247450348));
#78104=CARTESIAN_POINT('Ctrl Pts',(1.50236563076145,222.809975836444,6.45615318609288));
#78105=CARTESIAN_POINT('Ctrl Pts',(0.63660825535895,222.421621002517,6.40323389768228));
#78106=CARTESIAN_POINT('Ctrl Pts',(-0.194196242434726,222.485791949564,
6.35031460927168));
#78107=CARTESIAN_POINT('Ctrl Pts',(-1.02500074022841,222.549962896611,6.29739532086108));
#78108=CARTESIAN_POINT('Ctrl Pts',(-1.8208523604133,223.066659624631,6.24447603245049));
#78109=CARTESIAN_POINT('Ctrl Pts',(-2.21756941724085,223.799441721043,6.19155674403989));
#78110=CARTESIAN_POINT('Ctrl Pts',(-2.4149146716173,224.163961135396,6.16523226352392));
#78111=CARTESIAN_POINT('Ctrl Pts',(-2.51349313003819,224.581951387528,6.13890778300795));
#78112=CARTESIAN_POINT('Ctrl Pts',(-2.51344096553148,224.999964780717,6.11258330249198));
#78113=CARTESIAN_POINT('Ctrl Pts',(-2.51699557978349,225.002292230688,6.38741669750802));
#78114=CARTESIAN_POINT('Ctrl Pts',(-2.51140512213347,224.379058686358,6.42680495010456));
#78115=CARTESIAN_POINT('Ctrl Pts',(-2.27734636356429,223.752074884207,6.4661932027011));
#78116=CARTESIAN_POINT('Ctrl Pts',(-1.85802060188977,223.295091015239,6.50558145529765));
#78117=CARTESIAN_POINT('Ctrl Pts',(-1.29464397415902,222.681119600751,6.55850074370824));
#78118=CARTESIAN_POINT('Ctrl Pts',(-0.396847041080206,222.37401032907,6.61142003211884));
#78119=CARTESIAN_POINT('Ctrl Pts',(0.424538338422313,222.514296396878,6.66433932052944));
#78120=CARTESIAN_POINT('Ctrl Pts',(1.24592371792485,222.654582464686,6.71725860894004));
#78121=CARTESIAN_POINT('Ctrl Pts',(1.99089754385111,223.242263871983,6.77017789735063));
#78122=CARTESIAN_POINT('Ctrl Pts',(2.31855980810489,224.008417618346,6.82309718576123));
#78123=CARTESIAN_POINT('Ctrl Pts',(2.64622207235867,224.774571364709,6.87601647417183));
#78124=CARTESIAN_POINT('Ctrl Pts',(2.55657277494001,225.719197450137,6.92893576258243));
#78125=CARTESIAN_POINT('Ctrl Pts',(2.090635432585,226.410034996511,6.98185505099302));
#78126=CARTESIAN_POINT('Ctrl Pts',(1.62469809022998,227.100872542886,7.03477433940362));
#78127=CARTESIAN_POINT('Ctrl Pts',(0.782472702938629,227.537921550207,7.08769362781422));
#78128=CARTESIAN_POINT('Ctrl Pts',(-0.0506384086244314,227.521188401318,
7.14061291622481));
#78129=CARTESIAN_POINT('Ctrl Pts',(-0.88374952018748,227.504455252428,7.19353220463541));
#78130=CARTESIAN_POINT('Ctrl Pts',(-1.70774635602222,227.033939947329,7.246451493046));
#78131=CARTESIAN_POINT('Ctrl Pts',(-2.14556798025209,226.324950280381,7.2993707814566));
#78132=CARTESIAN_POINT('Ctrl Pts',(-2.38838055471039,225.931749952283,7.32871942014041));
#78133=CARTESIAN_POINT('Ctrl Pts',(-2.51241613654943,225.465201396059,7.35806805882421));
#78134=CARTESIAN_POINT('Ctrl Pts',(-2.51364339850779,224.999260136873,7.38741669750802));
#78135=CARTESIAN_POINT('Origin',(0.,225.,10.));
#78136=CARTESIAN_POINT('',(-2.51970634748832,224.998100077872,8.38741669750802));
#78137=CARTESIAN_POINT('',(-2.5206697586887,225.00143085894,8.11258330249197));
#78138=CARTESIAN_POINT('',(-2.5175,225.,10.));
#78139=CARTESIAN_POINT('Ctrl Pts',(-2.5206697586887,225.00143085894,8.11258330249197));
#78140=CARTESIAN_POINT('Ctrl Pts',(-2.52123853593806,225.085145295118,8.10727257726845));
#78141=CARTESIAN_POINT('Ctrl Pts',(-2.51742950928565,225.168807347417,8.10196185204492));
#78142=CARTESIAN_POINT('Ctrl Pts',(-2.50907233067035,225.252012580876,8.0966511268214));
#78143=CARTESIAN_POINT('Ctrl Pts',(-2.42579633222796,226.081120011841,8.0437318384108));
#78144=CARTESIAN_POINT('Ctrl Pts',(-1.89091891768193,226.864868352514,7.99081255000021));
#78145=CARTESIAN_POINT('Ctrl Pts',(-1.14919998141176,227.244614377611,7.93789326158961));
#78146=CARTESIAN_POINT('Ctrl Pts',(-0.407481045141574,227.624360402708,
7.88497397317902));
#78147=CARTESIAN_POINT('Ctrl Pts',(0.541079412852777,227.600104112231,7.83205468476842));
#78148=CARTESIAN_POINT('Ctrl Pts',(1.26242014564368,227.182945184224,7.77913539635782));
#78149=CARTESIAN_POINT('Ctrl Pts',(1.9837608784346,226.765786256217,7.72621610794722));
#78150=CARTESIAN_POINT('Ctrl Pts',(2.47788188602208,225.955724690681,7.67329681953662));
#78151=CARTESIAN_POINT('Ctrl Pts',(2.51867340504949,225.123444644078,7.62037753112602));
#78152=CARTESIAN_POINT('Ctrl Pts',(2.5594649240769,224.291164597474,7.56745824271542));
#78153=CARTESIAN_POINT('Ctrl Pts',(2.14692695454429,223.436666069803,7.51453895430482));
#78154=CARTESIAN_POINT('Ctrl Pts',(1.46983686319842,222.950967570526,7.46161966589423));
#78155=CARTESIAN_POINT('Ctrl Pts',(0.792746771852553,222.465269071248,7.40870037748363));
#78156=CARTESIAN_POINT('Ctrl Pts',(-0.148895441306572,222.348370600364,
7.35578108907304));
#78157=CARTESIAN_POINT('Ctrl Pts',(-0.924194318051915,222.653764895852,
7.30286180066244));
#78158=CARTESIAN_POINT('Ctrl Pts',(-1.69949319479726,222.95915919134,7.24994251225184));
#78159=CARTESIAN_POINT('Ctrl Pts',(-2.30844873512883,223.686846253199,7.19702322384125));
#78160=CARTESIAN_POINT('Ctrl Pts',(-2.4724028957642,224.503836496231,7.14410393543065));
#78161=CARTESIAN_POINT('Ctrl Pts',(-2.50495522889496,224.66604609465,7.13359705778442));
#78162=CARTESIAN_POINT('Ctrl Pts',(-2.51996549703062,224.831776046668,7.1230901801382));
#78163=CARTESIAN_POINT('Ctrl Pts',(-2.51844027096952,224.997780461794,7.11258330249198));
#78164=CARTESIAN_POINT('Ctrl Pts',(-2.51364339850779,224.999260136873,7.38741669750802));
#78165=CARTESIAN_POINT('Ctrl Pts',(-2.51462904428357,224.625050677558,7.41098734723481));
#78166=CARTESIAN_POINT('Ctrl Pts',(-2.4364019612172,224.251232931569,7.43455799696161));
#78167=CARTESIAN_POINT('Ctrl Pts',(-2.27687382072545,223.916117714943,7.4581286466884));
#78168=CARTESIAN_POINT('Ctrl Pts',(-1.91871162434389,223.163738845247,7.511047935099));
#78169=CARTESIAN_POINT('Ctrl Pts',(-1.15074081895573,222.606445134651,7.5639672235096));
#78170=CARTESIAN_POINT('Ctrl Pts',(-0.324384830006751,222.499254174166,
7.61688651192019));
#78171=CARTESIAN_POINT('Ctrl Pts',(0.501971158942218,222.392063213681,7.66980580033079));
#78172=CARTESIAN_POINT('Ctrl Pts',(1.38671233145202,222.734975003306,7.72272508874139));
#78173=CARTESIAN_POINT('Ctrl Pts',(1.92498114437798,223.371073114853,7.77564437715199));
#78174=CARTESIAN_POINT('Ctrl Pts',(2.46324995730394,224.007171226399,7.82856366556258));
#78175=CARTESIAN_POINT('Ctrl Pts',(2.65504641064604,224.936455659866,7.88148295397317));
#78176=CARTESIAN_POINT('Ctrl Pts',(2.41260445112607,225.733685876771,7.93440224238377));
#78177=CARTESIAN_POINT('Ctrl Pts',(2.17016249160608,226.530916093675,7.98732153079437));
#78178=CARTESIAN_POINT('Ctrl Pts',(1.49348211922398,227.196092094017,8.04024081920497));
#78179=CARTESIAN_POINT('Ctrl Pts',(0.692212259076926,227.424829353119,8.09316010761557));
#78180=CARTESIAN_POINT('Ctrl Pts',(-0.109057601070118,227.653566612221,
8.14607939602617));
#78181=CARTESIAN_POINT('Ctrl Pts',(-1.03491694898213,227.445865130083,8.19899868443676));
#78182=CARTESIAN_POINT('Ctrl Pts',(-1.66169256525882,226.896769100847,8.25191797284736));
#78183=CARTESIAN_POINT('Ctrl Pts',(-2.19664115838768,226.428119490518,8.29708421440091));
#78184=CARTESIAN_POINT('Ctrl Pts',(-2.51372212363046,225.710780926955,8.34225045595447));
#78185=CARTESIAN_POINT('Ctrl Pts',(-2.51970634748832,224.998100077872,8.38741669750802));
#78186=CARTESIAN_POINT('Origin',(0.,225.,10.));
#78187=CARTESIAN_POINT('',(-2.51957016294845,225.001947759268,9.38741669750802));
#78188=CARTESIAN_POINT('',(-2.51411981970798,225.001308619991,9.11258330249198));
#78189=CARTESIAN_POINT('',(-2.5175,225.,10.));
#78190=CARTESIAN_POINT('Ctrl Pts',(-2.51411981970798,225.001308619991,9.11258330249198));
#78191=CARTESIAN_POINT('Ctrl Pts',(-2.51569980701715,225.336584612862,9.0914549743987));
#78192=CARTESIAN_POINT('Ctrl Pts',(-2.45336466365061,225.671297040634,9.07032664630543));
#78193=CARTESIAN_POINT('Ctrl Pts',(-2.324342022709,225.977951155695,9.04919831821216));
#78194=CARTESIAN_POINT('Ctrl Pts',(-2.00118411275304,226.746015599105,8.99627902980156));
#78195=CARTESIAN_POINT('Ctrl Pts',(-1.25967391532669,227.338061152429,8.94335974139096));
#78196=CARTESIAN_POINT('Ctrl Pts',(-0.43912648219266,227.483167782107,8.89044045298036));
#78197=CARTESIAN_POINT('Ctrl Pts',(0.381420950941362,227.628274411784,8.83752116456977));
#78198=CARTESIAN_POINT('Ctrl Pts',(1.28100561978306,227.326442117814,8.78460187615917));
#78199=CARTESIAN_POINT('Ctrl Pts',(1.84797759755815,226.715789351983,8.73168258774857));
#78200=CARTESIAN_POINT('Ctrl Pts',(2.41494957533325,226.105136586152,8.67876329933797));
#78201=CARTESIAN_POINT('Ctrl Pts',(2.64930886204171,225.18566334846,8.62584401092738));
#78202=CARTESIAN_POINT('Ctrl Pts',(2.44381265269372,224.378120574396,8.57292472251678));
#78203=CARTESIAN_POINT('Ctrl Pts',(2.23831644334573,223.570577800332,8.52000543410618));
#78204=CARTESIAN_POINT('Ctrl Pts',(1.59296473794131,222.874965489897,8.46708614569558));
#78205=CARTESIAN_POINT('Ctrl Pts',(0.803070464184594,222.609595822667,8.41416685728498));
#78206=CARTESIAN_POINT('Ctrl Pts',(0.0131761904278596,222.344226155438,
8.36124756887439));
#78207=CARTESIAN_POINT('Ctrl Pts',(-0.921260651681179,222.509099131415,
8.30832828046379));
#78208=CARTESIAN_POINT('Ctrl Pts',(-1.57264178156633,223.028768880033,8.25540899205319));
#78209=CARTESIAN_POINT('Ctrl Pts',(-2.1586534346405,223.496287072483,8.20780042886612));
#78210=CARTESIAN_POINT('Ctrl Pts',(-2.51557089431972,224.250963859292,8.16019186567905));
#78211=CARTESIAN_POINT('Ctrl Pts',(-2.5206697586887,225.00143085894,8.11258330249197));
#78212=CARTESIAN_POINT('Ctrl Pts',(-2.51970634748832,224.998100077872,8.38741669750802));
#78213=CARTESIAN_POINT('Ctrl Pts',(-2.52073357415978,224.875764283992,8.39516974436507));
#78214=CARTESIAN_POINT('Ctrl Pts',(-2.51259411443575,224.753565732976,8.40292279122211));
#78215=CARTESIAN_POINT('Ctrl Pts',(-2.49481641921416,224.632785842068,8.41067583807916));
#78216=CARTESIAN_POINT('Ctrl Pts',(-2.37347277225141,223.808389188859,8.46359512648976));
#78217=CARTESIAN_POINT('Ctrl Pts',(-1.80309359368457,223.050086458773,8.51651441490035));
#78218=CARTESIAN_POINT('Ctrl Pts',(-1.044684384411,222.704876966188,8.56943370331095));
#78219=CARTESIAN_POINT('Ctrl Pts',(-0.286275175137409,222.359667473603,
8.62235299172154));
#78220=CARTESIAN_POINT('Ctrl Pts',(0.660164064842918,222.42755121852,8.67527228013214));
#78221=CARTESIAN_POINT('Ctrl Pts',(1.3615427579239,222.877464600599,8.72819156854274));
#78222=CARTESIAN_POINT('Ctrl Pts',(2.06292145100487,223.327377982678,8.78111085695334));
#78223=CARTESIAN_POINT('Ctrl Pts',(2.51923959718651,224.159321001919,8.83403014536394));
#78224=CARTESIAN_POINT('Ctrl Pts',(2.52168602174821,224.992596549075,8.88694943377453));
#78225=CARTESIAN_POINT('Ctrl Pts',(2.52413244630992,225.825872096231,8.93986872218513));
#78226=CARTESIAN_POINT('Ctrl Pts',(2.0727071492517,226.660480171302,8.99278801059573));
#78227=CARTESIAN_POINT('Ctrl Pts',(1.37398233763145,227.114504135546,9.04570729900633));
#78228=CARTESIAN_POINT('Ctrl Pts',(0.675257526011217,227.56852809979,9.09862658741692));
#78229=CARTESIAN_POINT('Ctrl Pts',(-0.270766800171062,227.641967953207,
9.15154587582752));
#78230=CARTESIAN_POINT('Ctrl Pts',(-1.03118992785508,227.301217620317,9.20446516423812));
#78231=CARTESIAN_POINT('Ctrl Pts',(-1.79161305553911,226.960467287426,9.25738445264872));
#78232=CARTESIAN_POINT('Ctrl Pts',(-2.3664349847249,226.205526768229,9.31030374105931));
#78233=CARTESIAN_POINT('Ctrl Pts',(-2.4926172119192,225.381856829466,9.36322302946991));
#78234=CARTESIAN_POINT('Ctrl Pts',(-2.51184656419469,225.256334877894,9.37128758548261));
#78235=CARTESIAN_POINT('Ctrl Pts',(-2.52065680612908,225.129216769309,9.37935214149532));
#78236=CARTESIAN_POINT('Ctrl Pts',(-2.51957016294845,225.001947759268,9.38741669750802));
#78237=CARTESIAN_POINT('Origin',(0.,225.,10.));
#78238=CARTESIAN_POINT('',(-2.51360226051679,225.000662435525,10.387416697508));
#78239=CARTESIAN_POINT('',(-2.5158975516969,224.997857973357,10.112583302492));
#78240=CARTESIAN_POINT('',(-2.5175,225.,10.));
#78241=CARTESIAN_POINT('Ctrl Pts',(-2.5158975516969,224.997857973357,10.112583302492));
#78242=CARTESIAN_POINT('Ctrl Pts',(-2.51116121626031,225.583094699563,10.075637371529));
#78243=CARTESIAN_POINT('Ctrl Pts',(-2.30769410526437,226.171300871144,10.0386914405659));
#78244=CARTESIAN_POINT('Ctrl Pts',(-1.93451251538482,226.617595632188,10.0017455096029));
#78245=CARTESIAN_POINT('Ctrl Pts',(-1.39998804490588,227.256843326324,9.94882622119231));
#78246=CARTESIAN_POINT('Ctrl Pts',(-0.517275688115731,227.604944181348,
9.89590693278172));
#78247=CARTESIAN_POINT('Ctrl Pts',(0.30969539787435,227.502607252845,9.84298764437112));
#78248=CARTESIAN_POINT('Ctrl Pts',(1.13666648386443,227.400270324341,9.79006835596052));
#78249=CARTESIAN_POINT('Ctrl Pts',(1.90789629905445,226.847495612311,9.73714906754992));
#78250=CARTESIAN_POINT('Ctrl Pts',(2.27047009517739,226.09723281411,9.68422977913933));
#78251=CARTESIAN_POINT('Ctrl Pts',(2.63304389130033,225.346970015909,9.63131049072872));
#78252=CARTESIAN_POINT('Ctrl Pts',(2.5869616683562,224.399219131538,9.57839120231813));
#78253=CARTESIAN_POINT('Ctrl Pts',(2.15331065065815,223.68767094705,9.52547191390753));
#78254=CARTESIAN_POINT('Ctrl Pts',(1.7196596329601,222.976122762562,9.47255262549694));
#78255=CARTESIAN_POINT('Ctrl Pts',(0.898439820508138,222.500777277956,9.41963333708634));
#78256=CARTESIAN_POINT('Ctrl Pts',(0.0654413833334434,222.479152577643,
9.36671404867574));
#78257=CARTESIAN_POINT('Ctrl Pts',(-0.767557053841252,222.45752787733,9.31379476026514));
#78258=CARTESIAN_POINT('Ctrl Pts',(-1.61233411573868,222.889623961309,9.26087547185455));
#78259=CARTESIAN_POINT('Ctrl Pts',(-2.08231983544461,223.577713670048,9.20795618344395));
#78260=CARTESIAN_POINT('Ctrl Pts',(-2.36466107270674,223.991079633239,9.17616522312662));
#78261=CARTESIAN_POINT('Ctrl Pts',(-2.51174247524297,224.496832083198,9.1443742628093));
#78262=CARTESIAN_POINT('Ctrl Pts',(-2.51411981970798,225.001308619991,9.11258330249198));
#78263=CARTESIAN_POINT('Ctrl Pts',(-2.51957016294845,225.001947759268,9.38741669750802));
#78264=CARTESIAN_POINT('Ctrl Pts',(-2.51352629779302,224.294082703961,9.43227142990591));
#78265=CARTESIAN_POINT('Ctrl Pts',(-2.20131841827154,223.581549453024,9.4771261623038));
#78266=CARTESIAN_POINT('Ctrl Pts',(-1.6728013216547,223.113020683305,9.5219808947017));
#78267=CARTESIAN_POINT('Ctrl Pts',(-1.04926067899306,222.560253834235,9.57490018311229));
#78268=CARTESIAN_POINT('Ctrl Pts',(-0.124636868466955,222.347119494424,
9.62781947152289));
#78269=CARTESIAN_POINT('Ctrl Pts',(0.677962272406855,222.571147933579,9.68073875993349));
#78270=CARTESIAN_POINT('Ctrl Pts',(1.48056141328067,222.795176372734,9.73365804834409));
#78271=CARTESIAN_POINT('Ctrl Pts',(2.16113588450219,223.456367590855,9.78657733675469));
#78272=CARTESIAN_POINT('Ctrl Pts',(2.40825482142189,224.252160499529,9.83949662516529));
#78273=CARTESIAN_POINT('Ctrl Pts',(2.65537375834158,225.047953408204,9.89241591357588));
#78274=CARTESIAN_POINT('Ctrl Pts',(2.46903716095948,225.978348007433,9.94533520198648));
#78275=CARTESIAN_POINT('Ctrl Pts',(1.93451265257388,226.617595746903,9.99825449039708));
#78276=CARTESIAN_POINT('Ctrl Pts',(1.39998814418828,227.256843486372,10.0511737788077));
#78277=CARTESIAN_POINT('Ctrl Pts',(0.517275724799156,227.604944366082,10.1040930672183));
#78278=CARTESIAN_POINT('Ctrl Pts',(-0.309695419836912,227.502607430321,
10.1570123556289));
#78279=CARTESIAN_POINT('Ctrl Pts',(-1.13666656447296,227.40027049456,10.2099316440395));
#78280=CARTESIAN_POINT('Ctrl Pts',(-1.90789643435596,226.847495743329,10.2628509324501));
#78281=CARTESIAN_POINT('Ctrl Pts',(-2.27047025619141,226.097232891922,10.3157702208607));
#78282=CARTESIAN_POINT('Ctrl Pts',(-2.43409765708363,225.758643746847,10.3396523797431));
#78283=CARTESIAN_POINT('Ctrl Pts',(-2.51449559242104,225.379832930983,10.3635345386256));
#78284=CARTESIAN_POINT('Ctrl Pts',(-2.51360226051679,225.000662435525,10.387416697508));
#78285=CARTESIAN_POINT('Origin',(0.,225.,10.));
#78286=CARTESIAN_POINT('',(-2.51714221557728,224.997701746028,11.387416697508));
#78287=CARTESIAN_POINT('',(-2.52169605742446,224.999954178766,11.112583302492));
#78288=CARTESIAN_POINT('',(-2.5175,225.,10.));
#78289=CARTESIAN_POINT('Ctrl Pts',(-2.52169565421209,224.999954183169,11.112583302492));
#78290=CARTESIAN_POINT('Ctrl Pts',(-2.52147281221073,225.830781657145,11.0598197686592));
#78291=CARTESIAN_POINT('Ctrl Pts',(-2.07065048216162,226.661816358474,11.0070562348264));
#78292=CARTESIAN_POINT('Ctrl Pts',(-1.37398224019328,227.114503985593,10.9542927009937));
#78293=CARTESIAN_POINT('Ctrl Pts',(-0.675257478124223,227.568527917639,
10.9013734125831));
#78294=CARTESIAN_POINT('Ctrl Pts',(0.270766780969211,227.641967765848,10.8484541241725));
#78295=CARTESIAN_POINT('Ctrl Pts',(1.03118985472662,227.301217457122,10.7955348357619));
#78296=CARTESIAN_POINT('Ctrl Pts',(1.79161292848402,226.960467148397,10.7426155473513));
#78297=CARTESIAN_POINT('Ctrl Pts',(2.36643481690539,226.205526682737,10.6896962589407));
#78298=CARTESIAN_POINT('Ctrl Pts',(2.49261703515127,225.381856802386,10.6367769705301));
#78299=CARTESIAN_POINT('Ctrl Pts',(2.61879925339715,224.558186922035,10.5838576821195));
#78300=CARTESIAN_POINT('Ctrl Pts',(2.29634180146753,223.665787626992,10.5309383937089));
#78301=CARTESIAN_POINT('Ctrl Pts',(1.67280120302526,223.113020817123,10.4780191052983));
#78302=CARTESIAN_POINT('Ctrl Pts',(1.04926060458298,222.560254007253,10.4250998168877));
#78303=CARTESIAN_POINT('Ctrl Pts',(0.124636859628036,222.347119682557,10.3721805284771));
#78304=CARTESIAN_POINT('Ctrl Pts',(-0.677962224328165,222.571148105825,
10.3192612400665));
#78305=CARTESIAN_POINT('Ctrl Pts',(-1.48056130828437,222.795176529092,10.2663419516559));
#78306=CARTESIAN_POINT('Ctrl Pts',(-2.16113573124182,223.456367700324,10.2134226632453));
#78307=CARTESIAN_POINT('Ctrl Pts',(-2.40825465063667,224.252160552564,10.1605033748347));
#78308=CARTESIAN_POINT('Ctrl Pts',(-2.48284595656893,224.49236566614,10.1445300173871));
#78309=CARTESIAN_POINT('Ctrl Pts',(-2.51794527865757,224.744834293198,10.1285566599396));
#78310=CARTESIAN_POINT('Ctrl Pts',(-2.5158975516969,224.997857973357,10.112583302492));
#78311=CARTESIAN_POINT('Ctrl Pts',(-2.51360226051679,225.000662435525,10.387416697508));
#78312=CARTESIAN_POINT('Ctrl Pts',(-2.51251610267223,224.539647883028,10.4164538270362));
#78313=CARTESIAN_POINT('Ctrl Pts',(-2.39125772294784,224.078101619103,10.4454909565643));
#78314=CARTESIAN_POINT('Ctrl Pts',(-2.15331080336361,223.687670853984,10.4745280860925));
#78315=CARTESIAN_POINT('Ctrl Pts',(-1.71965975491251,222.976122619035,10.5274473745031));
#78316=CARTESIAN_POINT('Ctrl Pts',(-0.898439884222463,222.50077710072,10.5803666629137));
#78317=CARTESIAN_POINT('Ctrl Pts',(-0.0654413879743779,222.479152398873,
10.6332859513243));
#78318=CARTESIAN_POINT('Ctrl Pts',(0.767557108273737,222.457527697027,10.6862052397348));
#78319=CARTESIAN_POINT('Ctrl Pts',(1.61233423007989,222.889623811649,10.7391245281454));
#78320=CARTESIAN_POINT('Ctrl Pts',(2.08231998311562,223.577713569184,10.792043816556));
#78321=CARTESIAN_POINT('Ctrl Pts',(2.55230573615135,224.265803326719,10.8449631049666));
#78322=CARTESIAN_POINT('Ctrl Pts',(2.64750012041665,225.209886727168,10.8978823933772));
#78323=CARTESIAN_POINT('Ctrl Pts',(2.32434218754344,225.977951225047,10.9508016817878));
#78324=CARTESIAN_POINT('Ctrl Pts',(2.00118425467023,226.746015722927,11.0037209701984));
#78325=CARTESIAN_POINT('Ctrl Pts',(1.2596740046585,227.338061318237,11.056640258609));
#78326=CARTESIAN_POINT('Ctrl Pts',(0.439126513334034,227.483167958204,11.1095595470196));
#78327=CARTESIAN_POINT('Ctrl Pts',(-0.381420977990437,227.628274598172,
11.1624788354302));
#78328=CARTESIAN_POINT('Ctrl Pts',(-1.28100571062764,227.326442282797,11.2153981238408));
#78329=CARTESIAN_POINT('Ctrl Pts',(-1.84797772861045,226.715789473661,11.2683174122514));
#78330=CARTESIAN_POINT('Ctrl Pts',(-2.27331704646822,226.257681064343,11.3080171740036));
#78331=CARTESIAN_POINT('Ctrl Pts',(-2.51146463506934,225.625770994084,11.3477169357558));
#78332=CARTESIAN_POINT('Ctrl Pts',(-2.51714221557728,224.997701746028,11.387416697508));
#78333=CARTESIAN_POINT('Origin',(0.,225.,10.));
#78334=CARTESIAN_POINT('',(-2.52142589487062,225.000747710561,12.387416697508));
#78335=CARTESIAN_POINT('',(-2.51603107573661,225.002171022738,12.112583302492));
#78336=CARTESIAN_POINT('',(-2.5175,225.,10.));
#78337=CARTESIAN_POINT('Ctrl Pts',(-2.51603107573661,225.002171022738,12.112583302492));
#78338=CARTESIAN_POINT('Ctrl Pts',(-2.51807394519329,225.250226974727,12.0969214542001));
#78339=CARTESIAN_POINT('Ctrl Pts',(-2.48435673616632,225.497739760452,12.0812596059081));
#78340=CARTESIAN_POINT('Ctrl Pts',(-2.41260428003234,225.73368582474,12.0655977576162));
#78341=CARTESIAN_POINT('Ctrl Pts',(-2.17016233770549,226.530915985108,12.0126784692056));
#78342=CARTESIAN_POINT('Ctrl Pts',(-1.49348201331126,227.196091938278,11.959759180795));
#78343=CARTESIAN_POINT('Ctrl Pts',(-0.692212209987538,227.424829181159,
11.9068398923844));
#78344=CARTESIAN_POINT('Ctrl Pts',(0.109057593336183,227.65356642404,11.8539206039738));
#78345=CARTESIAN_POINT('Ctrl Pts',(1.03491687558939,227.445864956631,11.8010013155632));
#78346=CARTESIAN_POINT('Ctrl Pts',(1.66169244741728,226.896768966335,11.7480820271526));
#78347=CARTESIAN_POINT('Ctrl Pts',(2.28846801924516,226.347672976039,11.695162738742));
#78348=CARTESIAN_POINT('Ctrl Pts',(2.61615988064774,225.457182462856,11.6422434503314));
#78349=CARTESIAN_POINT('Ctrl Pts',(2.49481624229027,224.63278586811,11.5893241619208));
#78350=CARTESIAN_POINT('Ctrl Pts',(2.37347260393281,223.808389273364,11.5364048735102));
#78351=CARTESIAN_POINT('Ctrl Pts',(1.8030934658153,223.050086597054,11.4834855850996));
#78352=CARTESIAN_POINT('Ctrl Pts',(1.04468431032549,222.70487712895,11.430566296689));
#78353=CARTESIAN_POINT('Ctrl Pts',(0.286275154835696,222.359667660847,11.3776470082784));
#78354=CARTESIAN_POINT('Ctrl Pts',(-0.660164018026388,222.427551400949,
11.3247277198678));
#78355=CARTESIAN_POINT('Ctrl Pts',(-1.36154266136797,222.877464751122,11.2718084314572));
#78356=CARTESIAN_POINT('Ctrl Pts',(-2.06292130470955,223.327378101294,11.2188891430466));
#78357=CARTESIAN_POINT('Ctrl Pts',(-2.51923941853063,224.159321061537,11.1659698546361));
#78358=CARTESIAN_POINT('Ctrl Pts',(-2.52168584291883,224.9925965496,11.1130505662255));
#78359=CARTESIAN_POINT('Ctrl Pts',(-2.52169304335196,224.995049085825,11.1128948116476));
#78360=CARTESIAN_POINT('Ctrl Pts',(-2.52169631202743,224.997501633594,11.1127390570698));
#78361=CARTESIAN_POINT('Ctrl Pts',(-2.52169565421209,224.999954183169,11.112583302492));
#78362=CARTESIAN_POINT('Ctrl Pts',(-2.51714221557728,224.997701746028,11.387416697508));
#78363=CARTESIAN_POINT('Ctrl Pts',(-2.51903277923729,224.788562501822,11.4006362241664));
#78364=CARTESIAN_POINT('Ctrl Pts',(-2.49514690270336,224.57984913072,11.4138557508248));
#78365=CARTESIAN_POINT('Ctrl Pts',(-2.44381282600061,224.378120530295,11.4270752774832));
#78366=CARTESIAN_POINT('Ctrl Pts',(-2.23831660207953,223.570577698963,11.4799945658938));
#78367=CARTESIAN_POINT('Ctrl Pts',(-1.59296485090897,222.874965339197,11.5329138543044));
#78368=CARTESIAN_POINT('Ctrl Pts',(-0.803070521135639,222.609595653148,
11.585833142715));
#78369=CARTESIAN_POINT('Ctrl Pts',(-0.0131761913623006,222.3442259671,11.6387524311256));
#78370=CARTESIAN_POINT('Ctrl Pts',(0.921260717013809,222.509098954769,11.6916717195362));
#78371=CARTESIAN_POINT('Ctrl Pts',(1.5726418930927,223.02876874024,11.7445910079468));
#78372=CARTESIAN_POINT('Ctrl Pts',(2.22402306917158,223.548438525711,11.7975102963574));
#78373=CARTESIAN_POINT('Ctrl Pts',(2.59234851295325,224.422905108984,11.850429584768));
#78374=CARTESIAN_POINT('Ctrl Pts',(2.50907250860523,225.252012598747,11.9033488731786));
#78375=CARTESIAN_POINT('Ctrl Pts',(2.42579650425721,226.081120088511,11.9562681615892));
#78376=CARTESIAN_POINT('Ctrl Pts',(1.8909190517795,226.864868484764,12.0091874499998));
#78377=CARTESIAN_POINT('Ctrl Pts',(1.14920006290913,227.244614536791,12.0621067384104));
#78378=CARTESIAN_POINT('Ctrl Pts',(0.407481074038757,227.624360588819,12.115026026821));
#78379=CARTESIAN_POINT('Ctrl Pts',(-0.541079451224263,227.600104296622,
12.1679453152316));
#78380=CARTESIAN_POINT('Ctrl Pts',(-1.26242023517021,227.182945339031,12.2208646036422));
#78381=CARTESIAN_POINT('Ctrl Pts',(-1.98376101911615,226.765786381441,12.2737838920528));
#78382=CARTESIAN_POINT('Ctrl Pts',(-2.47788206174501,225.955724758458,12.3267031804634));
#78383=CARTESIAN_POINT('Ctrl Pts',(-2.51867358366524,225.123444652832,12.379622468874));
#78384=CARTESIAN_POINT('Ctrl Pts',(-2.52067624632207,225.082583802119,12.3822205450853));
#78385=CARTESIAN_POINT('Ctrl Pts',(-2.52158623705894,225.041669397619,12.3848186212967));
#78386=CARTESIAN_POINT('Ctrl Pts',(-2.52142589487062,225.000747710561,12.387416697508));
#78387=CARTESIAN_POINT('Origin',(0.,225.,10.));
#78388=CARTESIAN_POINT('',(-2.5149421643676,225.001823827574,13.387416697508));
#78389=CARTESIAN_POINT('',(-2.51404431806768,224.998759332749,13.112583302492));
#78390=CARTESIAN_POINT('',(-2.5175,225.,10.));
#78391=CARTESIAN_POINT('Ctrl Pts',(-2.51404431806768,224.998759332749,13.112583302492));
#78392=CARTESIAN_POINT('Ctrl Pts',(-2.51181646834445,225.498330218278,13.0811038513303));
#78393=CARTESIAN_POINT('Ctrl Pts',(-2.36780172426376,225.999084826841,13.0496244001686));
#78394=CARTESIAN_POINT('Ctrl Pts',(-2.09063528432425,226.410034896516,13.018144949007));
#78395=CARTESIAN_POINT('Ctrl Pts',(-1.62469797501192,227.100872393899,12.9652256605964));
#78396=CARTESIAN_POINT('Ctrl Pts',(-0.782472647448307,227.537921370226,
12.9123063721858));
#78397=CARTESIAN_POINT('Ctrl Pts',(0.0506384050333455,227.521188222523,
12.8593870837752));
#78398=CARTESIAN_POINT('Ctrl Pts',(0.883749457514986,227.504455074821,12.8064677953646));
#78399=CARTESIAN_POINT('Ctrl Pts',(1.70774623491467,227.033939803089,12.753548506954));
#78400=CARTESIAN_POINT('Ctrl Pts',(2.14556782809573,226.324950186421,12.7006292185434));
#78401=CARTESIAN_POINT('Ctrl Pts',(2.58338942127679,225.615960569752,12.6477099301328));
#78402=CARTESIAN_POINT('Ctrl Pts',(2.63503583023922,224.668496608148,12.5947906417222));
#78403=CARTESIAN_POINT('Ctrl Pts',(2.2768736592573,223.916117791808,12.5418713533116));
#78404=CARTESIAN_POINT('Ctrl Pts',(1.91871148827538,223.163738975468,12.488952064901));
#78405=CARTESIAN_POINT('Ctrl Pts',(1.15074073734909,222.606445304394,12.4360327764904));
#78406=CARTESIAN_POINT('Ctrl Pts',(0.324384807002465,222.49925435151,12.3831134880798));
#78407=CARTESIAN_POINT('Ctrl Pts',(-0.501971123344163,222.392063398627,
12.3301941996692));
#78408=CARTESIAN_POINT('Ctrl Pts',(-1.38671223311115,222.734975163934,12.2772749112586));
#78409=CARTESIAN_POINT('Ctrl Pts',(-1.9249810078649,223.371073230371,12.224355622848));
#78410=CARTESIAN_POINT('Ctrl Pts',(-2.30394522385243,223.818913447646,12.1870981827293));
#78411=CARTESIAN_POINT('Ctrl Pts',(-2.51117136281936,224.412079125215,12.1498407426107));
#78412=CARTESIAN_POINT('Ctrl Pts',(-2.51603107573661,225.002171022738,12.112583302492));
#78413=CARTESIAN_POINT('Ctrl Pts',(-2.52142589487062,225.000747710561,12.387416697508));
#78414=CARTESIAN_POINT('Ctrl Pts',(-2.51832028417003,224.208150138174,12.4377379097073));
#78415=CARTESIAN_POINT('Ctrl Pts',(-2.11368531846519,223.412820555035,12.4880591219065));
#78416=CARTESIAN_POINT('Ctrl Pts',(-1.4698369674343,222.950967425215,12.5383803341058));
#78417=CARTESIAN_POINT('Ctrl Pts',(-0.792746828071511,222.465268891494,
12.5912996225164));
#78418=CARTESIAN_POINT('Ctrl Pts',(0.148895451865672,222.34837041232,12.644218910927));
#78419=CARTESIAN_POINT('Ctrl Pts',(0.924194383592584,222.653764729465,12.6971381993376));
#78420=CARTESIAN_POINT('Ctrl Pts',(1.6994933153195,222.959159046611,12.7500574877481));
#78421=CARTESIAN_POINT('Ctrl Pts',(2.30844889883614,223.686846160075,12.8029767761587));
#78422=CARTESIAN_POINT('Ctrl Pts',(2.47240307109859,224.503836461045,12.8558960645693));
#78423=CARTESIAN_POINT('Ctrl Pts',(2.63635724336105,225.320826762015,12.9088153529799));
#78424=CARTESIAN_POINT('Ctrl Pts',(2.35531000436931,226.227120250491,12.9617346413905));
#78425=CARTESIAN_POINT('Ctrl Pts',(1.75786856516005,226.807997043965,13.0146539298011));
#78426=CARTESIAN_POINT('Ctrl Pts',(1.16042712595079,227.38887383744,13.0675732182117));
#78427=CARTESIAN_POINT('Ctrl Pts',(0.246591486524002,227.644333935913,13.1204925066223));
#78428=CARTESIAN_POINT('Ctrl Pts',(-0.565467182486472,227.457478803346,
13.1734117950329));
#78429=CARTESIAN_POINT('Ctrl Pts',(-1.37752585149693,227.27062367078,13.2263310834435));
#78430=CARTESIAN_POINT('Ctrl Pts',(-2.08780755009108,226.641453307173,13.2792503718541));
#78431=CARTESIAN_POINT('Ctrl Pts',(-2.37128738695782,225.857876058543,13.3321696602647));
#78432=CARTESIAN_POINT('Ctrl Pts',(-2.46993712051424,225.585194630288,13.3505853393458));
#78433=CARTESIAN_POINT('Ctrl Pts',(-2.51690075091277,225.293814384377,13.3690010184269));
#78434=CARTESIAN_POINT('Ctrl Pts',(-2.5149421643676,225.001823827574,13.387416697508));
#78435=CARTESIAN_POINT('Origin',(0.,225.,10.));
#78436=CARTESIAN_POINT('',(-2.51484787790986,224.998220566968,14.387416697508));
#78437=CARTESIAN_POINT('',(-2.52055916665943,224.998500632631,14.112583302492));
#78438=CARTESIAN_POINT('',(-2.5175,225.,10.));
#78439=CARTESIAN_POINT('Ctrl Pts',(-2.52055916665943,224.998500632631,14.112583302492));
#78440=CARTESIAN_POINT('Ctrl Pts',(-2.51530317312179,225.744143280451,14.0652862484606));
#78441=CARTESIAN_POINT('Ctrl Pts',(-2.16362936224286,226.494093371989,14.0179891944291));
#78442=CARTESIAN_POINT('Ctrl Pts',(-1.58418929737073,226.961962938373,13.9706921403977));
#78443=CARTESIAN_POINT('Ctrl Pts',(-0.935870780761794,227.485448492158,
13.9177728519871));
#78444=CARTESIAN_POINT('Ctrl Pts',(-0.00241814453275091,227.655805429249,
13.8648535635765));
#78445=CARTESIAN_POINT('Ctrl Pts',(0.789020703331562,227.395078418584,13.8119342751659));
#78446=CARTESIAN_POINT('Ctrl Pts',(1.58045955119587,227.134351407919,13.7590149867553));
#78447=CARTESIAN_POINT('Ctrl Pts',(2.22988461069546,226.442540449498,13.7060956983447));
#78448=CARTESIAN_POINT('Ctrl Pts',(2.44011898737231,225.636218224291,13.6531764099341));
#78449=CARTESIAN_POINT('Ctrl Pts',(2.65035336404916,224.829895999084,13.6002571215235));
#78450=CARTESIAN_POINT('Ctrl Pts',(2.42139705790327,223.909062507092,13.5473378331129));
#78451=CARTESIAN_POINT('Ctrl Pts',(1.85802047012526,223.295091136145,13.4944185447023));
#78452=CARTESIAN_POINT('Ctrl Pts',(1.29464388234725,222.681119765198,13.4414992562917));
#78453=CARTESIAN_POINT('Ctrl Pts',(0.396847012937123,222.374010515296,13.3885799678811));
#78454=CARTESIAN_POINT('Ctrl Pts',(-0.424538308315552,222.514296573155,
13.3356606794705));
#78455=CARTESIAN_POINT('Ctrl Pts',(-1.24592362956823,222.654582631015,13.28274139106));
#78456=CARTESIAN_POINT('Ctrl Pts',(-1.99089740266345,223.242263996636,13.2298221026494));
#78457=CARTESIAN_POINT('Ctrl Pts',(-2.31855964368053,224.008417688666,13.1769028142388));
#78458=CARTESIAN_POINT('Ctrl Pts',(-2.45130944684338,224.318818885623,13.1554629769898));
#78459=CARTESIAN_POINT('Ctrl Pts',(-2.51556164869825,224.658514567202,13.1340231397409));
#78460=CARTESIAN_POINT('Ctrl Pts',(-2.51404431806768,224.998759332749,13.112583302492));
#78461=CARTESIAN_POINT('Ctrl Pts',(-2.5149421643676,225.001823827574,13.387416697508));
#78462=CARTESIAN_POINT('Ctrl Pts',(-2.51127255736073,224.454750431288,13.4219203068375));
#78463=CARTESIAN_POINT('Ctrl Pts',(-2.33586759681367,223.905534614577,13.456423916167));
#78464=CARTESIAN_POINT('Ctrl Pts',(-2.00690546813401,223.473145178696,13.4909275254965));
#78465=CARTESIAN_POINT('Ctrl Pts',(-1.50236573730415,222.809975681135,13.5438468139071));
#78466=CARTESIAN_POINT('Ctrl Pts',(-0.636608300505109,222.421620819667,
13.5967661023177));
#78467=CARTESIAN_POINT('Ctrl Pts',(0.19419625620641,222.485791771264,13.6496853907283));
#78468=CARTESIAN_POINT('Ctrl Pts',(1.02500081291792,222.549962722862,13.7026046791389));
#78469=CARTESIAN_POINT('Ctrl Pts',(1.82085248954192,223.066659487525,13.7555239675495));
#78470=CARTESIAN_POINT('Ctrl Pts',(2.21756957450331,223.799441635903,13.8084432559601));
#78471=CARTESIAN_POINT('Ctrl Pts',(2.61428665946469,224.532223784281,13.8613625443707));
#78472=CARTESIAN_POINT('Ctrl Pts',(2.61186915276347,225.481091316374,13.9142818327813));
#78473=CARTESIAN_POINT('Ctrl Pts',(2.21142330541858,226.211842468152,13.9672011211919));
#78474=CARTESIAN_POINT('Ctrl Pts',(1.81097745807369,226.942593619931,14.0201204096025));
#78475=CARTESIAN_POINT('Ctrl Pts',(1.01250327008514,227.455228391396,14.0730396980131));
#78476=CARTESIAN_POINT('Ctrl Pts',(0.181382514176868,227.515165121203,14.1259589864237));
#78477=CARTESIAN_POINT('Ctrl Pts',(-0.64973824173139,227.575101851011,14.1788782748343));
#78478=CARTESIAN_POINT('Ctrl Pts',(-1.51350556555936,227.182340539162,14.2317975632449));
#78479=CARTESIAN_POINT('Ctrl Pts',(-2.01465954690679,226.516608754235,14.2847168516555));
#78480=CARTESIAN_POINT('Ctrl Pts',(-2.33885410922109,226.085949450577,14.3189501336063));
#78481=CARTESIAN_POINT('Ctrl Pts',(-2.51130420518947,225.541058942732,14.3531834155572));
#78482=CARTESIAN_POINT('Ctrl Pts',(-2.51484787790986,224.998220566968,14.387416697508));
#78483=CARTESIAN_POINT('Origin',(0.,225.,10.));
#78484=CARTESIAN_POINT('',(-2.52136965310386,224.999178339809,15.387416697508));
#78485=CARTESIAN_POINT('',(-2.51858860887527,225.002195336597,15.112583302492));
#78486=CARTESIAN_POINT('',(-2.5175,225.,10.));
#78487=CARTESIAN_POINT('Ctrl Pts',(-2.51858860887527,225.002195336597,15.112583302492));
#78488=CARTESIAN_POINT('Ctrl Pts',(-2.52006205682024,225.163253597151,15.1023879340014));
#78489=CARTESIAN_POINT('Ctrl Pts',(-2.50593608807698,225.324054407012,15.0921925655108));
#78490=CARTESIAN_POINT('Ctrl Pts',(-2.47527363466472,225.481637555625,15.0819971970203));
#78491=CARTESIAN_POINT('Ctrl Pts',(-2.31611948373823,226.299576416568,15.0290779086097));
#78492=CARTESIAN_POINT('Ctrl Pts',(-1.71144725627252,227.030826584042,14.9761586201991));
#78493=CARTESIAN_POINT('Ctrl Pts',(-0.937954951666531,227.340767995787,
14.9232393317885));
#78494=CARTESIAN_POINT('Ctrl Pts',(-0.164462647060536,227.650709407532,
14.8703200433779));
#78495=CARTESIAN_POINT('Ctrl Pts',(0.777849734685748,227.539342063548,14.8174007549673));
#78496=CARTESIAN_POINT('Ctrl Pts',(1.45778006621284,227.057627658253,14.7644814665567));
#78497=CARTESIAN_POINT('Ctrl Pts',(2.13771039773993,226.575913252958,14.7115621781461));
#78498=CARTESIAN_POINT('Ctrl Pts',(2.55525867904782,225.723851786352,14.6586428897355));
#78499=CARTESIAN_POINT('Ctrl Pts',(2.51935482481995,224.8913465688,14.6057236013249));
#78500=CARTESIAN_POINT('Ctrl Pts',(2.48345097059207,224.058841351249,14.5528043129143));
#78501=CARTESIAN_POINT('Ctrl Pts',(1.99409498082843,223.245892382752,14.4998850245037));
#78502=CARTESIAN_POINT('Ctrl Pts',(1.27521614682309,222.824505095309,14.4469657360931));
#78503=CARTESIAN_POINT('Ctrl Pts',(0.55633731281776,222.403117807866,14.3940464476825));
#78504=CARTESIAN_POINT('Ctrl Pts',(-0.392064365429268,222.373292201478,
14.3411271592719));
#78505=CARTESIAN_POINT('Ctrl Pts',(-1.13600029859962,222.748676473042,14.2882078708613));
#78506=CARTESIAN_POINT('Ctrl Pts',(-1.87993623176996,223.124060744605,14.2352885824507));
#78507=CARTESIAN_POINT('Ctrl Pts',(-2.41940641986364,223.904654894119,14.1823692940401));
#78508=CARTESIAN_POINT('Ctrl Pts',(-2.50754931541607,224.733259054115,14.1294500056295));
#78509=CARTESIAN_POINT('Ctrl Pts',(-2.51691376517606,224.821291356419,14.1238277712503));
#78510=CARTESIAN_POINT('Ctrl Pts',(-2.5211839503414,224.909865561906,14.1182055368712));
#78511=CARTESIAN_POINT('Ctrl Pts',(-2.52055916665943,224.998500632631,14.112583302492));
#78512=CARTESIAN_POINT('Ctrl Pts',(-2.51484787790986,224.998220566968,14.387416697508));
#78513=CARTESIAN_POINT('Ctrl Pts',(-2.51678216780468,224.701915894494,14.4061027039678));
#78514=CARTESIAN_POINT('Ctrl Pts',(-2.46839165502543,224.406222644251,14.4247887104275));
#78515=CARTESIAN_POINT('Ctrl Pts',(-2.36688526988595,224.130052115031,14.4434747168873));
#78516=CARTESIAN_POINT('Ctrl Pts',(-2.07941637265078,223.347929518756,14.4963940052979));
#78517=CARTESIAN_POINT('Ctrl Pts',(-1.36593793931355,222.722386584209,14.5493132937085));
#78518=CARTESIAN_POINT('Ctrl Pts',(-0.552937686940973,222.53967174594,14.6022325821191));
#78519=CARTESIAN_POINT('Ctrl Pts',(0.260062565431603,222.356956907671,14.6551518705297));
#78520=CARTESIAN_POINT('Ctrl Pts',(1.17258463683953,222.61707016568,14.7080711589403));
#78521=CARTESIAN_POINT('Ctrl Pts',(1.76705844534861,223.200983698215,14.7609904473509));
#78522=CARTESIAN_POINT('Ctrl Pts',(2.3615322538577,223.784897230751,14.8139097357615));
#78523=CARTESIAN_POINT('Ctrl Pts',(2.63795779946796,224.692611037813,14.866829024172));
#78524=CARTESIAN_POINT('Ctrl Pts',(2.46984275794309,225.508755299139,14.9197483125826));
#78525=CARTESIAN_POINT('Ctrl Pts',(2.30172771641822,226.324899560465,14.9726676009932));
#78526=CARTESIAN_POINT('Ctrl Pts',(1.68907208775825,227.049474276054,15.0255868894038));
#78527=CARTESIAN_POINT('Ctrl Pts',(0.912227075592163,227.350914070298,15.0785061778144));
#78528=CARTESIAN_POINT('Ctrl Pts',(0.135382063426061,227.652353864542,15.131425466225));
#78529=CARTESIAN_POINT('Ctrl Pts',(-0.805652332246163,227.53065873744,15.1843447546356));
#78530=CARTESIAN_POINT('Ctrl Pts',(-1.48025879046803,227.041516376766,15.2372640430462));
#78531=CARTESIAN_POINT('Ctrl Pts',(-2.1182993075233,226.578887178787,15.2873149278668));
#78532=CARTESIAN_POINT('Ctrl Pts',(-2.51801170286182,225.787564939661,15.3373658126874));
#78533=CARTESIAN_POINT('Ctrl Pts',(-2.52136965310386,224.999178339809,15.387416697508));
#78534=CARTESIAN_POINT('Origin',(0.,225.,10.));
#78535=CARTESIAN_POINT('',(-2.51727025050597,225.002300995809,16.387416697508));
#78536=CARTESIAN_POINT('',(-2.51344539583794,225.000116344878,16.112583302492));
#78537=CARTESIAN_POINT('',(-2.5175,225.,10.));
#78538=CARTESIAN_POINT('Ctrl Pts',(-2.51344539583794,225.000116344878,16.112583302492));
#78539=CARTESIAN_POINT('Ctrl Pts',(-2.5136156958088,225.413181385681,16.0865703311317));
#78540=CARTESIAN_POINT('Ctrl Pts',(-2.41747216845691,225.826171771672,16.0605573597713));
#78541=CARTESIAN_POINT('Ctrl Pts',(-2.22458059720485,226.187516512708,16.034544388411));
#78542=CARTESIAN_POINT('Ctrl Pts',(-1.83217311135215,226.922615410164,15.9816251000004));
#78543=CARTESIAN_POINT('Ctrl Pts',(-1.03936913807555,227.443976292902,15.9287058115898));
#78544=CARTESIAN_POINT('Ctrl Pts',(-0.208955759937372,227.51302443121,15.8757865231792));
#78545=CARTESIAN_POINT('Ctrl Pts',(0.621457618200808,227.582072569518,15.8228672347686));
#78546=CARTESIAN_POINT('Ctrl Pts',(1.48948040120057,227.198807963396,15.769947946358));
#78547=CARTESIAN_POINT('Ctrl Pts',(1.99790538061801,226.53861248908,15.7170286579474));
#78548=CARTESIAN_POINT('Ctrl Pts',(2.50633036003544,225.878417014764,15.6641093695368));
#78549=CARTESIAN_POINT('Ctrl Pts',(2.65515753587054,224.941290672255,15.6111900811262));
#78550=CARTESIAN_POINT('Ctrl Pts',(2.37628359539248,224.156062457454,15.5582707927156));
#78551=CARTESIAN_POINT('Ctrl Pts',(2.09740965491442,223.370834242652,15.505351504305));
#78552=CARTESIAN_POINT('Ctrl Pts',(1.3908345981232,222.737504155558,15.4524322158944));
#78553=CARTESIAN_POINT('Ctrl Pts',(0.579887157111302,222.545884031576,15.3995129274838));
#78554=CARTESIAN_POINT('Ctrl Pts',(-0.231060283900595,222.354263907594,
15.3465936390732));
#78555=CARTESIAN_POINT('Ctrl Pts',(-1.14638010913316,222.604353746723,15.2936743506627));
#78556=CARTESIAN_POINT('Ctrl Pts',(-1.74722198455582,223.181712443495,15.2407550622521));
#78557=CARTESIAN_POINT('Ctrl Pts',(-2.23230636382754,223.647837885973,15.198031142332));
#78558=CARTESIAN_POINT('Ctrl Pts',(-2.51241409227338,224.327277089876,15.155307222412));
#78559=CARTESIAN_POINT('Ctrl Pts',(-2.51858860887527,225.002195336597,15.112583302492));
#78560=CARTESIAN_POINT('Ctrl Pts',(-2.52136965310386,224.999178339809,15.387416697508));
#78561=CARTESIAN_POINT('Ctrl Pts',(-2.52156209638561,224.953996102544,15.390285101098));
#78562=CARTESIAN_POINT('Ctrl Pts',(-2.52045275027353,224.908823507113,15.393153504688));
#78563=CARTESIAN_POINT('Ctrl Pts',(-2.51801186970213,224.863722975502,15.396021908278));
#78564=CARTESIAN_POINT('Ctrl Pts',(-2.47297996994284,224.03166152916,15.4489411966886));
#78565=CARTESIAN_POINT('Ctrl Pts',(-1.97473764965276,223.224128230723,15.5018604850992));
#78566=CARTESIAN_POINT('Ctrl Pts',(-1.25128058480224,222.810650301693,15.5547797735098));
#78567=CARTESIAN_POINT('Ctrl Pts',(-0.527823519951722,222.397172372662,
15.6076990619204));
#78568=CARTESIAN_POINT('Ctrl Pts',(0.420848289459224,222.37774981304,15.660618350331));
#78569=CARTESIAN_POINT('Ctrl Pts',(1.16062264210119,222.761270385695,15.7135376387416));
#78570=CARTESIAN_POINT('Ctrl Pts',(1.90039699474315,223.14479095835,15.7664569271522));
#78571=CARTESIAN_POINT('Ctrl Pts',(2.43127389061612,223.931254663283,15.8193762155628));
#78572=CARTESIAN_POINT('Ctrl Pts',(2.51032407259816,224.760775724643,15.8722955039734));
#78573=CARTESIAN_POINT('Ctrl Pts',(2.5893742545802,225.590296786003,15.925214792384));
#78574=CARTESIAN_POINT('Ctrl Pts',(2.21659772267131,226.462875203789,15.9781340807946));
#78575=CARTESIAN_POINT('Ctrl Pts',(1.56257701056091,226.979219111052,16.0310533692052));
#78576=CARTESIAN_POINT('Ctrl Pts',(0.908556298450499,227.495563018316,16.0839726576158));
#78577=CARTESIAN_POINT('Ctrl Pts',(-0.026708593861423,227.655672415057,
16.1368919460264));
#78578=CARTESIAN_POINT('Ctrl Pts',(-0.815240470077567,227.386281244732,
16.189811234437));
#78579=CARTESIAN_POINT('Ctrl Pts',(-1.60377234629372,227.116890074407,16.2427305228476));
#78580=CARTESIAN_POINT('Ctrl Pts',(-2.24557120641408,226.417998337017,16.2956498112582));
#78581=CARTESIAN_POINT('Ctrl Pts',(-2.44694990459468,225.609418877326,16.3485690996688));
#78582=CARTESIAN_POINT('Ctrl Pts',(-2.49622669896886,225.411561784543,16.3615182989485));
#78583=CARTESIAN_POINT('Ctrl Pts',(-2.5191325886196,225.207136953215,16.3744674982283));
#78584=CARTESIAN_POINT('Ctrl Pts',(-2.51727025050597,225.002300995809,16.387416697508));
#78585=CARTESIAN_POINT('Origin',(0.,225.,10.));
#78586=CARTESIAN_POINT('',(-2.51357028108852,224.999405388847,17.387416697508));
#78587=CARTESIAN_POINT('',(-2.51816163287682,224.997743614195,17.112583302492));
#78588=CARTESIAN_POINT('',(-2.5175,225.,10.));
#78589=CARTESIAN_POINT('Ctrl Pts',(-2.51816163287682,224.997743614195,17.112583302492));
#78590=CARTESIAN_POINT('Ctrl Pts',(-2.51206042535773,225.658837824156,17.0707527282619));
#78591=CARTESIAN_POINT('Ctrl Pts',(-2.24478065864621,226.324297969017,17.0289221540318));
#78592=CARTESIAN_POINT('Ctrl Pts',(-1.77759127638479,226.788609390717,16.9870915798018));
#78593=CARTESIAN_POINT('Ctrl Pts',(-1.18655636669689,227.376003431787,16.9341722913912));
#78594=CARTESIAN_POINT('Ctrl Pts',(-0.275577418352753,227.641470312515,
16.8812530029806));
#78595=CARTESIAN_POINT('Ctrl Pts',(0.538481621265696,227.463532391886,16.82833371457));
#78596=CARTESIAN_POINT('Ctrl Pts',(1.35254066088415,227.285594471258,16.7754144261594));
#78597=CARTESIAN_POINT('Ctrl Pts',(2.06967979177691,226.664251749274,16.7224951377488));
#78598=CARTESIAN_POINT('Ctrl Pts',(2.36173616102469,225.883830644091,16.6695758493382));
#78599=CARTESIAN_POINT('Ctrl Pts',(2.65379253027246,225.103409538909,16.6166565609276));
#78600=CARTESIAN_POINT('Ctrl Pts',(2.52076613787524,224.163910050527,16.563737272517));
#78601=CARTESIAN_POINT('Ctrl Pts',(2.02352985873453,223.495247125967,16.5108179841064));
#78602=CARTESIAN_POINT('Ctrl Pts',(1.52629357959382,222.826584201406,16.4578986956958));
#78603=CARTESIAN_POINT('Ctrl Pts',(0.66484741370963,222.428757840667,16.4049794072852));
#78604=CARTESIAN_POINT('Ctrl Pts',(-0.16661089052257,222.483813378794,16.3520601188746));
#78605=CARTESIAN_POINT('Ctrl Pts',(-0.998069194754779,222.53886891692,16.299140830464));
#78606=CARTESIAN_POINT('Ctrl Pts',(-1.79953963733499,223.046806353913,16.2462215420534));
#78607=CARTESIAN_POINT('Ctrl Pts',(-2.20426935941068,223.775193528496,16.1933022536428));
#78608=CARTESIAN_POINT('Ctrl Pts',(-2.41005039972525,224.14553517222,16.1663959365925));
#78609=CARTESIAN_POINT('Ctrl Pts',(-2.51326924737162,224.572865693797,16.1394896195423));
#78610=CARTESIAN_POINT('Ctrl Pts',(-2.51344539583794,225.000116344878,16.112583302492));
#78611=CARTESIAN_POINT('Ctrl Pts',(-2.51727025050597,225.002300995809,16.387416697508));
#78612=CARTESIAN_POINT('Ctrl Pts',(-2.51152180083078,224.370037077569,16.4273867866389));
#78613=CARTESIAN_POINT('Ctrl Pts',(-2.26979110135257,223.733856106507,16.4673568757697));
#78614=CARTESIAN_POINT('Ctrl Pts',(-1.83921088257949,223.274816376839,16.5073269649006));
#78615=CARTESIAN_POINT('Ctrl Pts',(-1.26913462614288,222.667060518033,16.5602462533112));
#78616=CARTESIAN_POINT('Ctrl Pts',(-0.368023577028847,222.369815982413,
16.6131655417218));
#78617=CARTESIAN_POINT('Ctrl Pts',(0.451773866702606,222.519101861478,16.6660848301324));
#78618=CARTESIAN_POINT('Ctrl Pts',(1.27157131043406,222.668387740542,16.719004118543));
#78619=CARTESIAN_POINT('Ctrl Pts',(2.01005514878293,223.264204034292,16.7719234069536));
#78620=CARTESIAN_POINT('Ctrl Pts',(2.32929519123782,224.0339052228,16.8248426953642));
#78621=CARTESIAN_POINT('Ctrl Pts',(2.64853523369271,224.803606411309,16.8777619837748));
#78622=CARTESIAN_POINT('Ctrl Pts',(2.54853148025362,225.747192494575,16.9306812721853));
#78623=CARTESIAN_POINT('Ctrl Pts',(2.07504564775282,226.432878490558,16.9836005605959));
#78624=CARTESIAN_POINT('Ctrl Pts',(1.60155981525203,227.11856448654,17.0365198490065));
#78625=CARTESIAN_POINT('Ctrl Pts',(0.754591903689518,227.546350395238,17.0894391374172));
#78626=CARTESIAN_POINT('Ctrl Pts',(-0.078285589744484,227.520481411304,
17.1423584258277));
#78627=CARTESIAN_POINT('Ctrl Pts',(-0.911163083178489,227.494612427371,
17.1952777142383));
#78628=CARTESIAN_POINT('Ctrl Pts',(-1.72995015848399,227.015088550806,17.2481970026489));
#78629=CARTESIAN_POINT('Ctrl Pts',(-2.15996986104755,226.301339861412,17.3011162910595));
#78630=CARTESIAN_POINT('Ctrl Pts',(-2.3937275716209,225.913347733231,17.329883093209));
#78631=CARTESIAN_POINT('Ctrl Pts',(-2.5126051329784,225.456142540028,17.3586498953585));
#78632=CARTESIAN_POINT('Ctrl Pts',(-2.51357028108852,224.999405388847,17.387416697508));
#78633=CARTESIAN_POINT('Origin',(0.,225.,10.));
#78634=CARTESIAN_POINT('',(-2.51944987787367,224.998011234297,18.387416697508));
#78635=CARTESIAN_POINT('',(-2.52086470301557,225.001296835693,18.112583302492));
#78636=CARTESIAN_POINT('',(-2.5175,225.,10.));
#78637=CARTESIAN_POINT('Ctrl Pts',(-2.52086470301557,225.001296835693,18.112583302492));
#78638=CARTESIAN_POINT('Ctrl Pts',(-2.52133257653149,225.075824437259,18.1078544138028));
#78639=CARTESIAN_POINT('Ctrl Pts',(-2.51831392254458,225.15031360591,18.1031255251135));
#78640=CARTESIAN_POINT('Ctrl Pts',(-2.51168534756933,225.224480139039,18.0983966364243));
#78641=CARTESIAN_POINT('Ctrl Pts',(-2.43750735482731,226.054451071963,18.0454773480137));
#78642=CARTESIAN_POINT('Ctrl Pts',(-1.91125747041057,226.844018225654,17.9925580596031));
#78643=CARTESIAN_POINT('Ctrl Pts',(-1.17374784032625,227.231875915892,17.9396387711925));
#78644=CARTESIAN_POINT('Ctrl Pts',(-0.436238210241938,227.619733606129,
17.8867194827819));
#78645=CARTESIAN_POINT('Ctrl Pts',(0.512531165509953,227.605881832913,17.8338001943713));
#78646=CARTESIAN_POINT('Ctrl Pts',(1.23840354227387,227.196659054247,17.7808809059607));
#78647=CARTESIAN_POINT('Ctrl Pts',(1.96427591903778,226.787436275581,17.7279616175501));
#78648=CARTESIAN_POINT('Ctrl Pts',(2.46725129681372,225.982842491466,17.6750423291396));
#78649=CARTESIAN_POINT('Ctrl Pts',(2.51716810188636,225.151059857407,17.622123040729));
#78650=CARTESIAN_POINT('Ctrl Pts',(2.56708490695901,224.319277223348,17.5692037523184));
#78651=CARTESIAN_POINT('Ctrl Pts',(2.16394313932837,223.460305739345,17.5162844639078));
#78652=CARTESIAN_POINT('Ctrl Pts',(1.49222048891769,222.967210712155,17.4633651754972));
#78653=CARTESIAN_POINT('Ctrl Pts',(0.820497838507012,222.474115684964,17.4104458870866));
#78654=CARTESIAN_POINT('Ctrl Pts',(-0.119805694683712,222.346897114587,
17.357526598676));
#78655=CARTESIAN_POINT('Ctrl Pts',(-0.898407244656005,222.643770229834,
17.3046073102654));
#78656=CARTESIAN_POINT('Ctrl Pts',(-1.67700879462829,222.940643345081,17.2516880218548));
#78657=CARTESIAN_POINT('Ctrl Pts',(-2.29390836138215,223.661608145953,17.1987687334442));
#78658=CARTESIAN_POINT('Ctrl Pts',(-2.46681270924325,224.476751147095,17.1458494450336));
#78659=CARTESIAN_POINT('Ctrl Pts',(-2.5030431074891,224.647556311476,17.134760730853));
#78660=CARTESIAN_POINT('Ctrl Pts',(-2.51977897969982,224.822496564027,17.1236720166725));
#78661=CARTESIAN_POINT('Ctrl Pts',(-2.51816163287682,224.997743614195,17.112583302492));
#78662=CARTESIAN_POINT('Ctrl Pts',(-2.51357028108852,224.999405388847,17.387416697508));
#78663=CARTESIAN_POINT('Ctrl Pts',(-2.51438061538806,224.61593079506,17.4115691837691));
#78664=CARTESIAN_POINT('Ctrl Pts',(-2.43207200078867,224.232786133973,17.4357216700302));
#78665=CARTESIAN_POINT('Ctrl Pts',(-2.26484979545939,223.891212085232,17.4598741562913));
#78666=CARTESIAN_POINT('Ctrl Pts',(-1.89845769748606,223.142806500668,17.5127934447019));
#78667=CARTESIAN_POINT('Ctrl Pts',(-1.12442117171776,222.593968833764,17.5657127331125));
#78668=CARTESIAN_POINT('Ctrl Pts',(-0.296939296283662,222.495847038768,
17.6186320215231));
#78669=CARTESIAN_POINT('Ctrl Pts',(0.530542579150434,222.397725243773,17.6715513099337));
#78670=CARTESIAN_POINT('Ctrl Pts',(1.41146980425034,222.750319320686,17.7244705983443));
#78671=CARTESIAN_POINT('Ctrl Pts',(1.94273005579705,223.392282534215,17.7773898867549));
#78672=CARTESIAN_POINT('Ctrl Pts',(2.47399030734377,224.034245747745,17.8303091751655));
#78673=CARTESIAN_POINT('Ctrl Pts',(2.65558358533729,224.965578097891,17.8832284635761));
#78674=CARTESIAN_POINT('Ctrl Pts',(2.40441289532158,225.760101295249,17.9361477519867));
#78675=CARTESIAN_POINT('Ctrl Pts',(2.15324220530586,226.554624492607,17.9890670403973));
#78676=CARTESIAN_POINT('Ctrl Pts',(1.46930754728092,227.212338537177,18.0419863288079));
#78677=CARTESIAN_POINT('Ctrl Pts',(0.665577232673735,227.432274763069,18.0949056172185));
#78678=CARTESIAN_POINT('Ctrl Pts',(-0.138153081933449,227.65221098896,18.1478249056291));
#78679=CARTESIAN_POINT('Ctrl Pts',(-1.06167905312287,227.434369396173,18.2007441940397));
#78680=CARTESIAN_POINT('Ctrl Pts',(-1.68239485993616,226.878431717949,18.2536634824503));
#78681=CARTESIAN_POINT('Ctrl Pts',(-2.20534680740171,226.410055226959,18.2982478874695));
#78682=CARTESIAN_POINT('Ctrl Pts',(-2.51336312809547,225.701697049152,18.3428322924888));
#78683=CARTESIAN_POINT('Ctrl Pts',(-2.51944987787367,224.998011234297,18.387416697508));
#78684=CARTESIAN_POINT('Origin',(0.,225.,10.));
#78685=CARTESIAN_POINT('',(-2.51981693572124,225.001815876221,19.387416697508));
#78686=CARTESIAN_POINT('',(-2.51426753931457,225.001426524072,19.112583302492));
#78687=CARTESIAN_POINT('',(-2.5175,225.,10.));
#78688=CARTESIAN_POINT('',(1.91346599666508,226.635987203375,20.));
#78689=CARTESIAN_POINT('Ctrl Pts',(-2.51981693572124,225.001815876221,19.387416697508));
#78690=CARTESIAN_POINT('Ctrl Pts',(-2.51391411286498,224.285104614356,19.4328532664402));
#78691=CARTESIAN_POINT('Ctrl Pts',(-2.19260500873154,223.563882178275,19.4782898353724));
#78692=CARTESIAN_POINT('Ctrl Pts',(-1.6520348486382,223.0949913699,19.5237264043046));
#78693=CARTESIAN_POINT('Ctrl Pts',(-1.02244091405153,222.54888129811,19.5766456927152));
#78694=CARTESIAN_POINT('Ctrl Pts',(-0.0954213187754091,222.3450568217,19.6295649811258));
#78695=CARTESIAN_POINT('Ctrl Pts',(0.704615011959953,222.5783234432,19.6824842695364));
#78696=CARTESIAN_POINT('Ctrl Pts',(1.50465134269532,222.811590064701,19.735403557947));
#78697=CARTESIAN_POINT('Ctrl Pts',(2.17770440888991,223.481947784111,19.7883228463576));
#78698=CARTESIAN_POINT('Ctrl Pts',(2.41590020207929,224.27898939678,19.8412421347682));
#78699=CARTESIAN_POINT('Ctrl Pts',(2.65409599526866,225.07603100945,19.8941614231788));
#78700=CARTESIAN_POINT('Ctrl Pts',(2.45743451545281,225.999756515378,19.9470807115894));
#78701=CARTESIAN_POINT('Ctrl Pts',(1.91346599666508,226.635987203375,20.));
#78702=CARTESIAN_POINT('',(-1.91712497064688,226.638739441994,20.));
#78703=CARTESIAN_POINT('Origin',(0.,225.,20.));
#78704=CARTESIAN_POINT('Ctrl Pts',(-1.91712853756764,226.638742124992,20.));
#78705=CARTESIAN_POINT('Ctrl Pts',(-1.38658184659742,227.25748310036,19.948244384658));
#78706=CARTESIAN_POINT('Ctrl Pts',(-0.527608215846001,227.597070123218,
19.896488769316));
#78707=CARTESIAN_POINT('Ctrl Pts',(0.282369170464696,227.505702112488,19.844733153974));
#78708=CARTESIAN_POINT('Ctrl Pts',(1.11055808540672,227.412279783734,19.7918138655634));
#78709=CARTESIAN_POINT('Ctrl Pts',(1.88752272406553,226.868305377813,19.7388945771528));
#78710=CARTESIAN_POINT('Ctrl Pts',(2.25823158349443,226.122142530554,19.6859752887422));
#78711=CARTESIAN_POINT('Ctrl Pts',(2.62894044292332,225.375979683295,19.6330560003316));
#78712=CARTESIAN_POINT('Ctrl Pts',(2.5933935231223,224.427628394699,19.580136711921));
#78713=CARTESIAN_POINT('Ctrl Pts',(2.16760736434175,223.711328508078,19.5272174235105));
#78714=CARTESIAN_POINT('Ctrl Pts',(1.7418212055612,222.995028621457,19.4742981350999));
#78715=CARTESIAN_POINT('Ctrl Pts',(0.925795807801111,222.510780136812,19.4213788466893));
#78716=CARTESIAN_POINT('Ctrl Pts',(0.0930673314969442,222.480040121849,
19.3684595582787));
#78717=CARTESIAN_POINT('Ctrl Pts',(-0.73966114480722,222.449300106886,19.3155402698681));
#78718=CARTESIAN_POINT('Ctrl Pts',(-1.58909269965547,222.872068561606,19.2626209814575));
#78719=CARTESIAN_POINT('Ctrl Pts',(-2.0665880130911,223.554953135211,19.2097016930469));
#78720=CARTESIAN_POINT('Ctrl Pts',(-2.35869055724325,223.972700316596,19.1773288961952));
#78721=CARTESIAN_POINT('Ctrl Pts',(-2.51160537190243,224.487789375327,19.1449560993436));
#78722=CARTESIAN_POINT('Ctrl Pts',(-2.51426753931457,225.001426524072,19.112583302492));
#78723=CARTESIAN_POINT('Origin',(0.,225.,22.2084234471774));
#78724=CARTESIAN_POINT('',(-3.07861193515008,225.000167983521,0.791576552822533));
#78725=CARTESIAN_POINT('',(-3.06858470798512,225.000715214498,0.708423447177441));
#78726=CARTESIAN_POINT('',(-3.0735,225.,22.2084234471774));
#78727=CARTESIAN_POINT('',(0.793799282532883,222.030777046254,0.));
#78728=CARTESIAN_POINT('Ctrl Pts',(-3.06858470798512,225.000715214498,0.708423447177441));
#78729=CARTESIAN_POINT('Ctrl Pts',(-3.06942183630073,225.474969719701,0.683959451760685));
#78730=CARTESIAN_POINT('Ctrl Pts',(-2.74289880307249,226.973915933301,0.60657616793333));
#78731=CARTESIAN_POINT('Ctrl Pts',(-0.407268936110244,228.609155678633,
0.476273595695376));
#78732=CARTESIAN_POINT('Ctrl Pts',(2.8136368462077,227.3011440524,0.317515730463589));
#78733=CARTESIAN_POINT('Ctrl Pts',(3.45438708523699,223.881452722834,0.158757865231792));
#78734=CARTESIAN_POINT('Ctrl Pts',(1.7810709486973,222.29471665351,0.0529192884105984));
#78735=CARTESIAN_POINT('Ctrl Pts',(0.793799282532894,222.030777046254,0.));
#78736=CARTESIAN_POINT('',(-0.79379928253288,222.030777046254,0.));
#78737=CARTESIAN_POINT('Origin',(0.,225.,0.));
#78738=CARTESIAN_POINT('Ctrl Pts',(-3.07861193515008,225.000167983521,0.791576552822533));
#78739=CARTESIAN_POINT('Ctrl Pts',(-3.07861787757322,225.008358867736,0.79115047086606));
#78740=CARTESIAN_POINT('Ctrl Pts',(-3.0748809971153,226.033849902817,0.737805100498988));
#78741=CARTESIAN_POINT('Ctrl Pts',(-1.94583850483642,228.067541710309,0.631540441721317));
#78742=CARTESIAN_POINT('Ctrl Pts',(1.52182603612892,228.298871095165,0.472782576489527));
#78743=CARTESIAN_POINT('Ctrl Pts',(3.59659353011021,225.51018574291,0.314024711257735));
#78744=CARTESIAN_POINT('Ctrl Pts',(2.38892360237163,222.280232421953,0.156430519094557));
#78745=CARTESIAN_POINT('Ctrl Pts',(0.166093927952955,221.76984766752,0.0517556153419845));
#78746=CARTESIAN_POINT('Ctrl Pts',(-0.795579049799779,222.025472494795,
5.56033084159191E-15));
#78747=CARTESIAN_POINT('Origin',(0.,225.,22.2084234471774));
#78748=CARTESIAN_POINT('',(-3.07140444904293,225.0025819181,1.79157655282252));
#78749=CARTESIAN_POINT('',(-3.07340046570963,224.997190573684,1.70842344717744));
#78750=CARTESIAN_POINT('',(-3.0735,225.,22.2084234471774));
#78751=CARTESIAN_POINT('Ctrl Pts',(-3.07340046570963,224.997190573684,1.70842344717744));
#78752=CARTESIAN_POINT('Ctrl Pts',(-3.06628884246803,225.774992353981,1.66814184889093));
#78753=CARTESIAN_POINT('Ctrl Pts',(-2.37168484978274,227.585923512749,1.57494096219383));
#78754=CARTESIAN_POINT('Ctrl Pts',(0.671786446474784,228.570069051027,1.42882078708613));
#78755=CARTESIAN_POINT('Ctrl Pts',(3.36369902404275,226.372043545379,1.27006292185434));
#78756=CARTESIAN_POINT('Ctrl Pts',(2.97708237215331,222.918244820821,1.11130505662255));
#78757=CARTESIAN_POINT('Ctrl Pts',(-0.134013682612229,221.369828849617,
0.952547191390754));
#78758=CARTESIAN_POINT('Ctrl Pts',(-2.66220321452624,222.870115699926,0.81825332157572));
#78759=CARTESIAN_POINT('Ctrl Pts',(-3.0676110022969,224.449086150263,0.736878740171281));
#78760=CARTESIAN_POINT('Ctrl Pts',(-3.06858470798512,225.000715214498,0.708423447177441));
#78761=CARTESIAN_POINT('Ctrl Pts',(-3.07140444904293,225.0025819181,1.79157655282252));
#78762=CARTESIAN_POINT('Ctrl Pts',(-3.07390606281625,225.316750705799,1.7753328679963));
#78763=CARTESIAN_POINT('Ctrl Pts',(-2.88509438037845,226.651495277729,1.70616989475949));
#78764=CARTESIAN_POINT('Ctrl Pts',(-0.958825582149559,228.5039149863,1.58408763311207));
#78765=CARTESIAN_POINT('Ctrl Pts',(2.42364536547895,227.706056696193,1.42532976788028));
#78766=CARTESIAN_POINT('Ctrl Pts',(3.58799443175235,224.431602766551,1.26657190264849));
#78767=CARTESIAN_POINT('Ctrl Pts',(1.46861466513916,221.677371668161,1.1078140374167));
#78768=CARTESIAN_POINT('Ctrl Pts',(-1.98555294623619,221.963188531272,0.949482254141378));
#78769=CARTESIAN_POINT('Ctrl Pts',(-3.07787982988179,223.991052789571,0.844069759276657));
#78770=CARTESIAN_POINT('Ctrl Pts',(-3.07861193515008,225.000167983521,0.791576552822533));
#78771=CARTESIAN_POINT('Origin',(0.,225.,22.2084234471774));
#78772=CARTESIAN_POINT('',(-3.06945735251731,224.998331954781,2.79157655282253));
#78773=CARTESIAN_POINT('',(-3.07813813283449,225.001105495988,2.70842344717744));
#78774=CARTESIAN_POINT('',(-3.0735,225.,22.2084234471774));
#78775=CARTESIAN_POINT('Ctrl Pts',(-3.07813813283449,225.001105495988,2.70842344717744));
#78776=CARTESIAN_POINT('Ctrl Pts',(-3.07842171245361,225.062261455412,2.70524353443178));
#78777=CARTESIAN_POINT('Ctrl Pts',(-3.04905263632461,226.140881525194,2.64914433327553));
#78778=CARTESIAN_POINT('Ctrl Pts',(-1.78403476954297,228.164490547375,2.54012584370868));
#78779=CARTESIAN_POINT('Ctrl Pts',(1.69089220174611,228.21522353059,2.38136797847689));
#78780=CARTESIAN_POINT('Ctrl Pts',(3.61831520156474,225.323384619251,2.22261011324509));
#78781=CARTESIAN_POINT('Ctrl Pts',(2.23425524535826,222.135582991462,2.0638522480133));
#78782=CARTESIAN_POINT('Ctrl Pts',(-1.19459293999268,221.56929798347,1.90509438278151));
#78783=CARTESIAN_POINT('Ctrl Pts',(-2.9375525643654,223.489815960057,1.78661811583622));
#78784=CARTESIAN_POINT('Ctrl Pts',(-3.07563162074394,224.753168034969,1.72106113730153));
#78785=CARTESIAN_POINT('Ctrl Pts',(-3.07340046570963,224.997190573684,1.70842344717744));
#78786=CARTESIAN_POINT('Ctrl Pts',(-3.06945735251731,224.998331954781,2.79157655282253));
#78787=CARTESIAN_POINT('Ctrl Pts',(-3.06639628624136,225.619418678826,2.75951526512656));
#78788=CARTESIAN_POINT('Ctrl Pts',(-2.58173678204169,227.270042729222,2.67453468901999));
#78789=CARTESIAN_POINT('Ctrl Pts',(0.112777612738978,228.630986010631,2.53663482450283));
#78790=CARTESIAN_POINT('Ctrl Pts',(3.11163588183028,226.874700175507,2.37787695927104));
#78791=CARTESIAN_POINT('Ctrl Pts',(3.26272508945618,223.402688633055,2.21911909403925));
#78792=CARTESIAN_POINT('Ctrl Pts',(0.42776847383237,221.392536757232,2.06036122880745));
#78793=CARTESIAN_POINT('Ctrl Pts',(-2.46856006320185,222.551801968966,1.91784704840188));
#78794=CARTESIAN_POINT('Ctrl Pts',(-3.06575621121678,224.293239792867,1.8282521564069));
#78795=CARTESIAN_POINT('Ctrl Pts',(-3.07140444904293,225.0025819181,1.79157655282252));
#78796=CARTESIAN_POINT('Origin',(0.,225.,22.2084234471774));
#78797=CARTESIAN_POINT('',(-3.07748275168016,224.998327996994,3.79157655282253));
#78798=CARTESIAN_POINT('',(-3.07013338639129,225.002107447932,3.70842344717744));
#78799=CARTESIAN_POINT('',(-3.0735,225.,22.2084234471774));
#78800=CARTESIAN_POINT('Ctrl Pts',(-3.07013338639129,225.002107447932,3.70842344717744));
#78801=CARTESIAN_POINT('Ctrl Pts',(-3.07245621738108,225.369921503297,3.68942593156204));
#78802=CARTESIAN_POINT('Ctrl Pts',(-2.84108114631271,226.759489676162,3.61750912753603));
#78803=CARTESIAN_POINT('Ctrl Pts',(-0.77573256839211,228.548946215303,3.49267303509943));
#78804=CARTESIAN_POINT('Ctrl Pts',(2.56078460694016,227.576657219349,3.33391516986764));
#78805=CARTESIAN_POINT('Ctrl Pts',(3.55367181789592,224.246211645467,3.17515730463585));
#78806=CARTESIAN_POINT('Ctrl Pts',(1.2942387062452,221.605633127976,3.01639943940405));
#78807=CARTESIAN_POINT('Ctrl Pts',(-2.08070002352559,222.062246195024,2.86082148691792));
#78808=CARTESIAN_POINT('Ctrl Pts',(-3.07370245351417,224.04451973933,2.75816282284238));
#78809=CARTESIAN_POINT('Ctrl Pts',(-3.07813813283449,225.001105495988,2.70842344717744));
#78810=CARTESIAN_POINT('Ctrl Pts',(-3.07748275168016,224.998327996994,3.79157655282253));
#78811=CARTESIAN_POINT('Ctrl Pts',(-3.07143800644999,225.919651939133,3.74369766225681));
#78812=CARTESIAN_POINT('Ctrl Pts',(-2.14228137459996,227.869865672693,3.6428994832805));
#78813=CARTESIAN_POINT('Ctrl Pts',(1.17442911621855,228.437658305789,3.48918201589358));
#78814=CARTESIAN_POINT('Ctrl Pts',(3.52505710830432,225.877924122033,3.33042415066179));
#78815=CARTESIAN_POINT('Ctrl Pts',(2.64955297313634,222.514713813743,3.17166628543));
#78816=CARTESIAN_POINT('Ctrl Pts',(-0.650821938137665,221.426037330607,
3.01290842019821));
#78817=CARTESIAN_POINT('Ctrl Pts',(-2.80933951944355,223.167551333338,2.88621184266238));
#78818=CARTESIAN_POINT('Ctrl Pts',(-3.07144877978551,224.594273719291,2.81243455353716));
#78819=CARTESIAN_POINT('Ctrl Pts',(-3.06945735251731,224.998331954781,2.79157655282253));
#78820=CARTESIAN_POINT('Origin',(0.,225.,22.2084234471774));
#78821=CARTESIAN_POINT('',(-3.07449013002601,225.002732289237,4.79157655282253));
#78822=CARTESIAN_POINT('',(-3.07051367074349,224.9977135172,4.70842344717744));
#78823=CARTESIAN_POINT('',(-3.0735,225.,22.2084234471774));
#78824=CARTESIAN_POINT('Ctrl Pts',(-3.07051367074349,224.9977135172,4.70842344717744));
#78825=CARTESIAN_POINT('Ctrl Pts',(-3.06585820728449,225.671564929849,4.67360832869228));
#78826=CARTESIAN_POINT('Ctrl Pts',(-2.51562445587184,227.376589891734,4.58587392179654));
#78827=CARTESIAN_POINT('Ctrl Pts',(0.301020094439488,228.620244073749,4.44522022649019));
#78828=CARTESIAN_POINT('Ctrl Pts',(3.20471405829287,226.710727346758,4.28646236125839));
#78829=CARTESIAN_POINT('Ctrl Pts',(3.17545384212145,223.235553019399,4.12770449602661));
#78830=CARTESIAN_POINT('Ctrl Pts',(0.24001839430402,221.375200499072,3.96894663079481));
#78831=CARTESIAN_POINT('Ctrl Pts',(-2.53753165970314,222.657907037816,3.82918628117842));
#78832=CARTESIAN_POINT('Ctrl Pts',(-3.06598576274026,224.345342370355,3.74234521997263));
#78833=CARTESIAN_POINT('Ctrl Pts',(-3.07013338639129,225.002107447932,3.70842344717744));
#78834=CARTESIAN_POINT('Ctrl Pts',(-3.07449013002601,225.002732289237,4.79157655282253));
#78835=CARTESIAN_POINT('Ctrl Pts',(-3.07640541686727,225.210641245489,4.78079934779766));
#78836=CARTESIAN_POINT('Ctrl Pts',(-2.96239872551369,226.437356865561,4.71710285436219));
#78837=CARTESIAN_POINT('Ctrl Pts',(-1.31414727007755,228.386708628075,4.60048707251613));
#78838=CARTESIAN_POINT('Ctrl Pts',(2.13244936546002,227.9409927036,4.44172920728434));
#78839=CARTESIAN_POINT('Ctrl Pts',(3.62742842558762,224.80368037246,4.28297134205255));
#78840=CARTESIAN_POINT('Ctrl Pts',(1.80258513325755,221.846039756688,4.12421347682075));
#78841=CARTESIAN_POINT('Ctrl Pts',(-1.67198400213467,221.774903431643,3.96545561158896));
#78842=CARTESIAN_POINT('Ctrl Pts',(-3.0299620136904,223.786670051152,3.85457663692289));
#78843=CARTESIAN_POINT('Ctrl Pts',(-3.07811910562385,224.901336626527,3.79661695066741));
#78844=CARTESIAN_POINT('Ctrl Pts',(-3.07748275168016,224.998327996994,3.79157655282253));
#78845=CARTESIAN_POINT('Origin',(0.,225.,22.2084234471774));
#78846=CARTESIAN_POINT('',(-3.06854451144427,224.999957002397,5.79157655282253));
#78847=CARTESIAN_POINT('',(-3.0783647624281,224.999192700359,5.70842344717744));
#78848=CARTESIAN_POINT('',(-3.0735,225.,22.2084234471774));
#78849=CARTESIAN_POINT('Ctrl Pts',(-3.0783647624281,224.999192700359,5.70842344717744));
#78850=CARTESIAN_POINT('Ctrl Pts',(-3.07494752107333,225.972768104595,5.65779072582254));
#78851=CARTESIAN_POINT('Ctrl Pts',(-2.05035872108597,227.970077691126,5.55423871605705));
#78852=CARTESIAN_POINT('Ctrl Pts',(1.35121084102199,228.372092749875,5.39776741788093));
#78853=CARTESIAN_POINT('Ctrl Pts',(3.56586056047961,225.693843436134,5.23900955264916));
#78854=CARTESIAN_POINT('Ctrl Pts',(2.51703483521181,222.380588636929,5.08025168741735));
#78855=CARTESIAN_POINT('Ctrl Pts',(-0.835381072264795,221.464619014198,
4.92149382218557));
#78856=CARTESIAN_POINT('Ctrl Pts',(-2.85574307416149,223.275546289828,4.79755107543892));
#78857=CARTESIAN_POINT('Ctrl Pts',(-3.07293455296969,224.647304815178,4.72652761710288));
#78858=CARTESIAN_POINT('Ctrl Pts',(-3.07051367074349,224.9977135172,4.70842344717744));
#78859=CARTESIAN_POINT('Ctrl Pts',(-3.06854451144427,224.999957002397,5.79157655282253));
#78860=CARTESIAN_POINT('Ctrl Pts',(-3.06848017220945,225.51553097262,5.76498174492791));
#78861=CARTESIAN_POINT('Ctrl Pts',(-2.70083896904008,227.057098457445,5.6854676486227));
#78862=CARTESIAN_POINT('Ctrl Pts',(-0.261298247139434,228.623327421715,
5.55303426390689));
#78863=CARTESIAN_POINT('Ctrl Pts',(2.9023029622151,227.184814842139,5.39427639867509));
#78864=CARTESIAN_POINT('Ctrl Pts',(3.40971661468071,223.746759804953,5.2355185334433));
#78865=CARTESIAN_POINT('Ctrl Pts',(0.796557755474301,221.455670144991,5.07676066821152));
#78866=CARTESIAN_POINT('Ctrl Pts',(-2.31872915212835,222.343678723149,4.92878000800458));
#78867=CARTESIAN_POINT('Ctrl Pts',(-3.06700078769786,224.189746310888,4.83371863620826));
#78868=CARTESIAN_POINT('Ctrl Pts',(-3.07449013002601,225.002732289237,4.79157655282253));
#78869=CARTESIAN_POINT('Origin',(0.,225.,22.2084234471774));
#78870=CARTESIAN_POINT('',(-3.07464793359474,224.997290267855,6.79157655282253));
#78871=CARTESIAN_POINT('',(-3.07288417654997,225.002798479054,6.70842344717745));
#78872=CARTESIAN_POINT('',(-3.0735,225.,22.2084234471774));
#78873=CARTESIAN_POINT('Ctrl Pts',(-3.07288417654997,225.002798479054,6.70842344717745));
#78874=CARTESIAN_POINT('Ctrl Pts',(-3.07522881255163,225.264182411633,6.69489241136339));
#78875=CARTESIAN_POINT('Ctrl Pts',(-2.92508997887231,226.545173952939,6.62844208713874));
#78876=CARTESIAN_POINT('Ctrl Pts',(-1.13665728427362,228.450331936026,6.50907247450349));
#78877=CARTESIAN_POINT('Ctrl Pts',(2.28217117361002,227.826389036385,6.3503146092717));
#78878=CARTESIAN_POINT('Ctrl Pts',(3.61235666314995,224.615735001789,6.1915567440399));
#78879=CARTESIAN_POINT('Ctrl Pts',(1.63651347662755,221.756760278445,6.03279887880811));
#78880=CARTESIAN_POINT('Ctrl Pts',(-1.83706677935009,221.865998420731,5.87404101357633));
#78881=CARTESIAN_POINT('Ctrl Pts',(-3.05774551774456,223.893866766071,5.76591586969943));
#78882=CARTESIAN_POINT('Ctrl Pts',(-3.0785190845995,224.955226162792,5.71071001423313));
#78883=CARTESIAN_POINT('Ctrl Pts',(-3.0783647624281,224.999192700359,5.70842344717744));
#78884=CARTESIAN_POINT('Ctrl Pts',(-3.07464793359474,224.997290267855,6.79157655282253));
#78885=CARTESIAN_POINT('Ctrl Pts',(-3.06713140628724,225.815383238637,6.74916414205817));
#78886=CARTESIAN_POINT('Ctrl Pts',(-2.31086280809112,227.66650877076,6.65383244288321));
#78887=CARTESIAN_POINT('Ctrl Pts',(0.814607649856128,228.540224958348,6.50558145529764));
#78888=CARTESIAN_POINT('Ctrl Pts',(3.41605827048919,226.235849615258,6.34682359006585));
#78889=CARTESIAN_POINT('Ctrl Pts',(2.89113249630378,222.800424752883,6.18806572483406));
#78890=CARTESIAN_POINT('Ctrl Pts',(-0.279757624807835,221.378051070173,
6.02930785960226));
#78891=CARTESIAN_POINT('Ctrl Pts',(-2.70632259531143,222.95346808107,5.89714480226509));
#78892=CARTESIAN_POINT('Ctrl Pts',(-3.06860819669216,224.489623670136,5.81790103333851));
#78893=CARTESIAN_POINT('Ctrl Pts',(-3.06854451144427,224.999957002397,5.79157655282253));
#78894=CARTESIAN_POINT('Origin',(0.,225.,22.2084234471774));
#78895=CARTESIAN_POINT('',(-3.07736981264336,225.001746869892,7.79157655282253));
#78896=CARTESIAN_POINT('',(-3.06879165255757,224.999096735126,7.70842344717744));
#78897=CARTESIAN_POINT('',(-3.0735,225.,22.2084234471774));
#78898=CARTESIAN_POINT('Ctrl Pts',(-3.06879165255757,224.999096735126,7.70842344717744));
#78899=CARTESIAN_POINT('Ctrl Pts',(-3.06729334485985,225.567942995347,7.67907480849364));
#78900=CARTESIAN_POINT('Ctrl Pts',(-2.64281785384595,227.164568935651,7.59680688139924));
#78901=CARTESIAN_POINT('Ctrl Pts',(-0.0729493050082294,228.632004770035,
7.46161966589425));
#78902=CARTESIAN_POINT('Ctrl Pts',(3.01175344912091,227.031285655038,7.30286180066245));
#78903=CARTESIAN_POINT('Ctrl Pts',(3.3400995650489,223.571533988429,7.14410393543066));
#78904=CARTESIAN_POINT('Ctrl Pts',(0.611586690390379,221.419114359437,6.98534607019887));
#78905=CARTESIAN_POINT('Ctrl Pts',(-2.39639172809182,222.448053117521,6.84011924078113));
#78906=CARTESIAN_POINT('Ctrl Pts',(-3.06605904384397,224.241921299909,6.74781169977399));
#78907=CARTESIAN_POINT('Ctrl Pts',(-3.07288417654997,225.002798479054,6.70842344717745));
#78908=CARTESIAN_POINT('Ctrl Pts',(-3.07736981264336,225.001746869892,7.79157655282253));
#78909=CARTESIAN_POINT('Ctrl Pts',(-3.07806420663577,225.103949975987,7.78626582759902));
#78910=CARTESIAN_POINT('Ctrl Pts',(-3.02707587405751,226.223865622706,7.7280358139649));
#78911=CARTESIAN_POINT('Ctrl Pts',(-1.65552872289502,228.233574342207,7.61688651192019));
#78912=CARTESIAN_POINT('Ctrl Pts',(1.81863282742744,228.144734172854,7.4581286466884));
#78913=CARTESIAN_POINT('Ctrl Pts',(3.62838168560431,225.177833412168,7.2993707814566));
#78914=CARTESIAN_POINT('Ctrl Pts',(2.11743576779875,222.048179519659,7.14061291622482));
#78915=CARTESIAN_POINT('Ctrl Pts',(-1.33138728143009,221.620031614681,6.98185505099302));
#78916=CARTESIAN_POINT('Ctrl Pts',(-2.96588661920454,223.573218574879,6.86550959652559));
#78917=CARTESIAN_POINT('Ctrl Pts',(-3.07651001196569,224.794623110004,6.80208343046876));
#78918=CARTESIAN_POINT('Ctrl Pts',(-3.07464793359474,224.997290267855,6.79157655282253));
#78919=CARTESIAN_POINT('Origin',(0.,225.,22.2084234471774));
#78920=CARTESIAN_POINT('',(-3.06937329329591,225.001597633979,8.79157655282253));
#78921=CARTESIAN_POINT('',(-3.07619362820471,224.997680472429,8.70842344717745));
#78922=CARTESIAN_POINT('',(-3.0735,225.,22.2084234471774));
#78923=CARTESIAN_POINT('Ctrl Pts',(-3.07619362820471,224.997680472429,8.70842344717745));
#78924=CARTESIAN_POINT('Ctrl Pts',(-3.06888776444019,225.867759753325,8.66325720562389));
#78925=CARTESIAN_POINT('Ctrl Pts',(-2.22821902191904,227.769621341675,8.56517167565974));
#78926=CARTESIAN_POINT('Ctrl Pts',(0.997195697683612,228.493190660582,8.41416685728499));
#78927=CARTESIAN_POINT('Ctrl Pts',(3.47557956006656,226.05694227482,8.25540899205321));
#78928=CARTESIAN_POINT('Ctrl Pts',(2.77311314575043,222.653380360706,8.09665112682141));
#78929=CARTESIAN_POINT('Ctrl Pts',(-0.467306310506461,221.397444648195,
7.93789326158963));
#78930=CARTESIAN_POINT('Ctrl Pts',(-2.76007210838313,223.061237008611,7.80848403504163));
#78931=CARTESIAN_POINT('Ctrl Pts',(-3.06999498216705,224.542241611707,7.73199409690424));
#78932=CARTESIAN_POINT('Ctrl Pts',(-3.06879165255757,224.999096735126,7.70842344717744));
#78933=CARTESIAN_POINT('Ctrl Pts',(-3.06937329329591,225.001597633979,8.79157655282253));
#78934=CARTESIAN_POINT('Ctrl Pts',(-3.0713022271567,225.410920678304,8.77044822472927));
#78935=CARTESIAN_POINT('Ctrl Pts',(-2.80459016801079,226.843047661762,8.6964006082254));
#78936=CARTESIAN_POINT('Ctrl Pts',(-0.632602258973873,228.57723255616,8.56943370331094));
#78937=CARTESIAN_POINT('Ctrl Pts',(2.66218242386824,227.471753046111,8.41067583807915));
#78938=CARTESIAN_POINT('Ctrl Pts',(3.52053785707391,224.10412524546,8.25191797284736));
#78939=CARTESIAN_POINT('Ctrl Pts',(1.15689718192732,221.556401984935,8.09316010761557));
#78940=CARTESIAN_POINT('Ctrl Pts',(-2.1510494467117,222.140059414158,7.93971296760729));
#78941=CARTESIAN_POINT('Ctrl Pts',(-3.07114484357178,224.085536215108,7.83918511600961));
#78942=CARTESIAN_POINT('Ctrl Pts',(-3.07736981264336,225.001746869892,7.79157655282253));
#78943=CARTESIAN_POINT('Origin',(0.,225.,22.2084234471774));
#78944=CARTESIAN_POINT('',(-3.07154364454433,224.997384898158,9.79157655282253));
#78945=CARTESIAN_POINT('',(-3.07602736676149,225.002377929736,9.70842344717745));
#78946=CARTESIAN_POINT('',(-3.0735,225.,22.2084234471774));
#78947=CARTESIAN_POINT('Ctrl Pts',(-3.07602736676149,225.002377929736,9.70842344717745));
#78948=CARTESIAN_POINT('Ctrl Pts',(-3.07735399945888,225.157754812501,9.70035889116475));
#78949=CARTESIAN_POINT('Ctrl Pts',(-2.99601741917923,226.331315348169,9.63937504674145));
#78950=CARTESIAN_POINT('Ctrl Pts',(-1.48552434035628,228.315116541671,9.52547191390755));
#78951=CARTESIAN_POINT('Ctrl Pts',(1.97934846979805,228.046138520449,9.36671404867575));
#78952=CARTESIAN_POINT('Ctrl Pts',(3.63272163822919,224.989334645098,9.20795618344396));
#78953=CARTESIAN_POINT('Ctrl Pts',(1.96142810620627,221.942291702134,9.04919831821217));
#78954=CARTESIAN_POINT('Ctrl Pts',(-1.50496435148532,221.693663273135,8.89044045298037));
#78955=CARTESIAN_POINT('Ctrl Pts',(-2.99968389613058,223.680849962287,8.77684882930214));
#78956=CARTESIAN_POINT('Ctrl Pts',(-3.0774477220179,224.848326326454,8.71617649403449));
#78957=CARTESIAN_POINT('Ctrl Pts',(-3.07619362820471,224.997680472429,8.70842344717745));
#78958=CARTESIAN_POINT('Ctrl Pts',(-3.07154364454433,224.997384898158,9.79157655282253));
#78959=CARTESIAN_POINT('Ctrl Pts',(-3.06576127037765,225.711873509079,9.75463062185952));
#78960=CARTESIAN_POINT('Ctrl Pts',(-2.46155812568994,227.45857358682,9.6647654024859));
#78961=CARTESIAN_POINT('Ctrl Pts',(0.446144826681538,228.60523690935,9.5219808947017));
#78962=CARTESIAN_POINT('Ctrl Pts',(3.27082189161085,226.580665218277,9.36322302946991));
#78963=CARTESIAN_POINT('Ctrl Pts',(3.10204288995985,223.109468781596,9.20446516423812));
#78964=CARTESIAN_POINT('Ctrl Pts',(0.094274357402458,221.368486441654,9.04570729900631));
#78965=CARTESIAN_POINT('Ctrl Pts',(-2.58800189649888,222.74044730297,8.90807776186779));
#78966=CARTESIAN_POINT('Ctrl Pts',(-3.06647090274457,224.385705425108,8.82336751313986));
#78967=CARTESIAN_POINT('Ctrl Pts',(-3.06937329329591,225.001597633979,8.79157655282253));
#78968=CARTESIAN_POINT('Origin',(0.,225.,22.2084234471774));
#78969=CARTESIAN_POINT('',(-3.07862277358246,224.999944058962,10.7915765528225));
#78970=CARTESIAN_POINT('',(-3.06874142907581,225.000808737075,10.7084234471774));
#78971=CARTESIAN_POINT('',(-3.0735,225.,22.2084234471774));
#78972=CARTESIAN_POINT('Ctrl Pts',(-3.06874142907581,225.000808737075,10.7084234471774));
#78973=CARTESIAN_POINT('Ctrl Pts',(-3.06983205692395,225.46372056142,10.684541288295));
#78974=CARTESIAN_POINT('Ctrl Pts',(-2.75418302977163,226.950963548454,10.6077398410019));
#78975=CARTESIAN_POINT('Ctrl Pts',(-0.446144858320614,228.605237165021,
10.4780191052983));
#78976=CARTESIAN_POINT('Ctrl Pts',(2.78684416371602,227.330296088014,10.3192612400665));
#78977=CARTESIAN_POINT('Ctrl Pts',(3.46931351670972,223.922668122894,10.1605033748347));
#78978=CARTESIAN_POINT('Ctrl Pts',(0.976667275638124,221.501014249336,10.0017455096029));
#78979=CARTESIAN_POINT('Ctrl Pts',(-2.23779834748522,222.241978304803,9.85105220038384));
#78980=CARTESIAN_POINT('Ctrl Pts',(-3.06864868967899,224.138178030039,9.75327817957534));
#78981=CARTESIAN_POINT('Ctrl Pts',(-3.07602736676149,225.002377929736,9.70842344717745));
#78982=CARTESIAN_POINT('Ctrl Pts',(-3.07862228131909,224.999944064338,10.7915765528225));
#78983=CARTESIAN_POINT('Ctrl Pts',(-3.07835022376532,226.014263127402,10.7388130189898));
#78984=CARTESIAN_POINT('Ctrl Pts',(-1.97594900327483,228.046402194062,10.6331301967464));
#78985=CARTESIAN_POINT('Ctrl Pts',(1.48552423500794,228.315116306574,10.4745280860925));
#78986=CARTESIAN_POINT('Ctrl Pts',(3.59084507798282,225.550099995309,10.3157702208607));
#78987=CARTESIAN_POINT('Ctrl Pts',(2.40982464679436,222.281632189969,10.1570123556289));
#78988=CARTESIAN_POINT('Ctrl Pts',(-0.976667206376252,221.501014497472,
9.99825449039707));
#78989=CARTESIAN_POINT('Ctrl Pts',(-2.88922780988848,223.35910399192,9.8764425561283));
#78990=CARTESIAN_POINT('Ctrl Pts',(-3.07404362023996,224.688479920614,9.80754991027012));
#78991=CARTESIAN_POINT('Ctrl Pts',(-3.07154364454433,224.997384898158,9.79157655282253));
#78992=CARTESIAN_POINT('Origin',(0.,225.,22.2084234471774));
#78993=CARTESIAN_POINT('',(-3.07170665790524,225.002650501842,11.7915765528225));
#78994=CARTESIAN_POINT('',(-3.07306319744856,224.997194167395,11.7084234471774));
#78995=CARTESIAN_POINT('',(-3.0735,225.,22.2084234471774));
#78996=CARTESIAN_POINT('Ctrl Pts',(-3.07306319744856,224.997194167395,11.7084234471774));
#78997=CARTESIAN_POINT('Ctrl Pts',(-3.0661317004511,225.763975034882,11.6687236854252));
#78998=CARTESIAN_POINT('Ctrl Pts',(-2.38783086968629,227.563804830108,11.5761046352624));
#78999=CARTESIAN_POINT('Ctrl Pts',(0.632602303835877,228.577232809845,11.430566296689));
#79000=CARTESIAN_POINT('Ctrl Pts',(3.34842961673882,226.408829071393,11.2718084314573));
#79001=CARTESIAN_POINT('Ctrl Pts',(2.99977427607618,222.951065022201,11.1130505662255));
#79002=CARTESIAN_POINT('Ctrl Pts',(-0.0942743640881148,221.36848618412,
10.9542927009937));
#79003=CARTESIAN_POINT('Ctrl Pts',(-2.64958041800097,222.847570317374,10.8194169946443));
#79004=CARTESIAN_POINT('Ctrl Pts',(-3.06741538890292,224.437977266529,10.7374605767056));
#79005=CARTESIAN_POINT('Ctrl Pts',(-3.06874142907581,225.000808737075,10.7084234471774));
#79006=CARTESIAN_POINT('Ctrl Pts',(-3.07170665790524,225.002650501842,11.7915765528225));
#79007=CARTESIAN_POINT('Ctrl Pts',(-3.07420070329748,225.305490608471,11.7759147045306));
#79008=CARTESIAN_POINT('Ctrl Pts',(-2.89394997723761,226.628683144966,11.7073335678281));
#79009=CARTESIAN_POINT('Ctrl Pts',(-0.997195626965866,228.493190412856,
11.585833142715));
#79010=CARTESIAN_POINT('Ctrl Pts',(2.39382145824392,227.732470897368,11.4270752774832));
#79011=CARTESIAN_POINT('Ctrl Pts',(3.59401323900362,224.47099412406,11.2683174122514));
#79012=CARTESIAN_POINT('Ctrl Pts',(1.50496424475834,221.69366350761,11.1095595470196));
#79013=CARTESIAN_POINT('Ctrl Pts',(-1.9614279671085,221.942291918976,10.9508016817878));
#79014=CARTESIAN_POINT('Ctrl Pts',(-3.07726325298195,223.97664313747,10.8448073503888));
#79015=CARTESIAN_POINT('Ctrl Pts',(-3.07862308441559,224.996949859326,10.7917323074004));
#79016=CARTESIAN_POINT('Ctrl Pts',(-3.07862228131909,224.999944064338,10.7915765528225));
#79017=CARTESIAN_POINT('Origin',(0.,225.,22.2084234471774));
#79018=CARTESIAN_POINT('',(-3.06928111681468,224.998485326397,12.7915765528225));
#79019=CARTESIAN_POINT('',(-3.07829294454214,225.000912845446,12.7084234471774));
#79020=CARTESIAN_POINT('',(-3.0735,225.,22.2084234471774));
#79021=CARTESIAN_POINT('Ctrl Pts',(-3.07829294454214,225.000912845446,12.7084234471774));
#79022=CARTESIAN_POINT('Ctrl Pts',(-3.07848869894762,225.050872251671,12.7058253709661));
#79023=CARTESIAN_POINT('Ctrl Pts',(-3.05474886562024,226.118247010729,12.6503080063441));
#79024=CARTESIAN_POINT('Ctrl Pts',(-1.81863295639868,228.144734395868,12.5418713533116));
#79025=CARTESIAN_POINT('Ctrl Pts',(1.65552884029951,228.233574571522,12.3831134880798));
#79026=CARTESIAN_POINT('Ctrl Pts',(3.6145507074577,225.363047426476,12.224355622848));
#79027=CARTESIAN_POINT('Ctrl Pts',(2.26553590928934,222.160259290996,12.0655977576162));
#79028=CARTESIAN_POINT('Ctrl Pts',(-1.15689726397057,221.556401740727,11.9068398923844));
#79029=CARTESIAN_POINT('Ctrl Pts',(-2.9294746139871,223.467029101815,11.7877817889048));
#79030=CARTESIAN_POINT('Ctrl Pts',(-3.07537129969644,224.74186567998,11.7216429738358));
#79031=CARTESIAN_POINT('Ctrl Pts',(-3.07306319744856,224.997194167395,11.7084234471774));
#79032=CARTESIAN_POINT('Ctrl Pts',(-3.06928111681467,224.998485326397,12.7915765528225));
#79033=CARTESIAN_POINT('Ctrl Pts',(-3.06656123751991,225.608388451192,12.7600971016609));
#79034=CARTESIAN_POINT('Ctrl Pts',(-2.59517217214773,227.247458453491,12.6756983620886));
#79035=CARTESIAN_POINT('Ctrl Pts',(0.0729492998349137,228.632004512465,
12.5383803341058));
#79036=CARTESIAN_POINT('Ctrl Pts',(3.09088863886716,226.908713126961,12.3796224688739));
#79037=CARTESIAN_POINT('Ctrl Pts',(3.28004681715442,223.438567562721,12.2208646036422));
#79038=CARTESIAN_POINT('Ctrl Pts',(0.46730627736665,221.397444903677,12.0621067384104));
#79039=CARTESIAN_POINT('Ctrl Pts',(-2.45343773644609,222.529479433023,11.9190107214705));
#79040=CARTESIAN_POINT('Ctrl Pts',(-3.0657736578453,224.282234435491,11.8288339929412));
#79041=CARTESIAN_POINT('Ctrl Pts',(-3.07170665790524,225.002650501842,11.7915765528225));
#79042=CARTESIAN_POINT('Origin',(0.,225.,22.2084234471774));
#79043=CARTESIAN_POINT('',(-3.07723479591964,224.998169491318,13.7915765528225));
#79044=CARTESIAN_POINT('',(-3.07037725608096,225.002226627229,13.7084234471775));
#79045=CARTESIAN_POINT('',(-3.0735,225.,22.2084234471774));
#79046=CARTESIAN_POINT('Ctrl Pts',(-3.07037725608096,225.002226627229,13.7084234471775));
#79047=CARTESIAN_POINT('Ctrl Pts',(-3.07276840434177,225.358704472843,13.6900077680964));
#79048=CARTESIAN_POINT('Ctrl Pts',(-2.85067271507903,226.736670699133,13.6186728006047));
#79049=CARTESIAN_POINT('Ctrl Pts',(-0.814607707625303,228.540225209408,
13.4944185447024));
#79050=CARTESIAN_POINT('Ctrl Pts',(2.53237203947883,227.604586743482,13.3356606794706));
#79051=CARTESIAN_POINT('Ctrl Pts',(3.56172499563507,224.285230592343,13.1769028142388));
#79052=CARTESIAN_POINT('Ctrl Pts',(1.33138737584751,221.620031374985,13.018144949007));
#79053=CARTESIAN_POINT('Ctrl Pts',(-2.06099584336155,222.041172659259,12.8619851599865));
#79054=CARTESIAN_POINT('Ctrl Pts',(-3.07450144722803,224.033266911491,12.7587446593767));
#79055=CARTESIAN_POINT('Ctrl Pts',(-3.07829294454214,225.000912845446,12.7084234471774));
#79056=CARTESIAN_POINT('Ctrl Pts',(-3.07723479591964,224.998169491318,13.7915765528225));
#79057=CARTESIAN_POINT('Ctrl Pts',(-3.07081799507026,225.908490316769,13.7442794987911));
#79058=CARTESIAN_POINT('Ctrl Pts',(-2.1610969881185,227.848485082751,13.6440631563491));
#79059=CARTESIAN_POINT('Ctrl Pts',(1.13665720366575,228.45033169134,13.4909275254965));
#79060=CARTESIAN_POINT('Ctrl Pts',(3.51521679100075,225.9165311185,13.3321696602647));
#79061=CARTESIAN_POINT('Ctrl Pts',(2.6766501094444,222.54392130205,13.1734117950329));
#79062=CARTESIAN_POINT('Ctrl Pts',(-0.611586647018769,221.419114613381,
13.0146539298011));
#79063=CARTESIAN_POINT('Ctrl Pts',(-2.79907365008124,223.144739589274,12.887375515731));
#79064=CARTESIAN_POINT('Ctrl Pts',(-3.07113355601754,224.583096135967,12.8130163900715));
#79065=CARTESIAN_POINT('Ctrl Pts',(-3.06928111681467,224.998485326397,12.7915765528225));
#79066=CARTESIAN_POINT('Origin',(0.,225.,22.2084234471774));
#79067=CARTESIAN_POINT('',(-3.07482903252357,225.002680185515,14.7915765528225));
#79068=CARTESIAN_POINT('',(-3.07026214607982,224.997827572026,14.7084234471775));
#79069=CARTESIAN_POINT('',(-3.0735,225.,22.2084234471774));
#79070=CARTESIAN_POINT('Ctrl Pts',(-3.07026214607981,224.997827572026,14.7084234471775));
#79071=CARTESIAN_POINT('Ctrl Pts',(-3.06593583898703,225.660553986291,14.6741901652266));
#79072=CARTESIAN_POINT('Ctrl Pts',(-2.52994317982435,227.354129803758,14.5870375948652));
#79073=CARTESIAN_POINT('Ctrl Pts',(0.261298265669851,228.62332767867,14.4469657360931));
#79074=CARTESIAN_POINT('Ctrl Pts',(3.18575953691054,226.745771011226,14.2882078708613));
#79075=CARTESIAN_POINT('Ctrl Pts',(3.19461380524764,223.270484782959,14.1294500056295));
#79076=CARTESIAN_POINT('Ctrl Pts',(0.279757644647243,221.378050813317,13.9706921403977));
#79077=CARTESIAN_POINT('Ctrl Pts',(-2.52331408064506,222.6354313281,13.830349954247));
#79078=CARTESIAN_POINT('Ctrl Pts',(-3.065897201608,224.334329871127,13.7429270565069));
#79079=CARTESIAN_POINT('Ctrl Pts',(-3.07037725608096,225.002226627229,13.7084234471775));
#79080=CARTESIAN_POINT('Ctrl Pts',(-3.07482903252357,225.002680185515,14.7915765528225));
#79081=CARTESIAN_POINT('Ctrl Pts',(-3.07662789737314,225.199308810663,14.781381184332));
#79082=CARTESIAN_POINT('Ctrl Pts',(-2.96986772218245,226.414596975574,14.7182665274308));
#79083=CARTESIAN_POINT('Ctrl Pts',(-1.35121074519871,228.372092510738,14.6022325821191));
#79084=CARTESIAN_POINT('Ctrl Pts',(2.10006683807499,227.964202701323,14.4434747168873));
#79085=CARTESIAN_POINT('Ctrl Pts',(3.62936333372522,224.843474696222,14.2847168516555));
#79086=CARTESIAN_POINT('Ctrl Pts',(1.83706664907154,221.865998642983,14.1259589864237));
#79087=CARTESIAN_POINT('Ctrl Pts',(-1.6365133605716,221.756760508445,13.9672011211919));
#79088=CARTESIAN_POINT('Ctrl Pts',(-3.02371435647241,223.763990945825,13.8557403099915));
#79089=CARTESIAN_POINT('Ctrl Pts',(-3.07799756559058,224.889959008746,13.7971987872017));
#79090=CARTESIAN_POINT('Ctrl Pts',(-3.07723479591964,224.998169491318,13.7915765528225));
#79091=CARTESIAN_POINT('Origin',(0.,225.,22.2084234471774));
#79092=CARTESIAN_POINT('',(-3.06854992020173,225.000142040112,15.7915765528225));
#79093=CARTESIAN_POINT('',(-3.078224281555,224.998996872852,15.7084234471775));
#79094=CARTESIAN_POINT('',(-3.0735,225.,22.2084234471774));
#79095=CARTESIAN_POINT('Ctrl Pts',(-3.078224281555,224.998996872852,15.7084234471775));
#79096=CARTESIAN_POINT('Ctrl Pts',(-3.07412471449684,225.96150182405,15.6583725623569));
#79097=CARTESIAN_POINT('Ctrl Pts',(-2.07017713194897,227.949046013955,15.5554023891256));
#79098=CARTESIAN_POINT('Ctrl Pts',(1.31414736327247,228.386708868249,15.3995129274839));
#79099=CARTESIAN_POINT('Ctrl Pts',(3.55803662804284,225.732909001281,15.2407550622521));
#79100=CARTESIAN_POINT('Ctrl Pts',(2.54561091074421,222.408350845166,15.0819971970203));
#79101=CARTESIAN_POINT('Ctrl Pts',(-0.796557811963526,221.455669893639,
14.9232393317885));
#79102=CARTESIAN_POINT('Ctrl Pts',(-2.84623604737516,223.252727349544,14.7987147485075));
#79103=CARTESIAN_POINT('Ctrl Pts',(-3.07262363167733,224.636082820945,14.7271094536372));
#79104=CARTESIAN_POINT('Ctrl Pts',(-3.07026214607981,224.997827572026,14.7084234471775));
#79105=CARTESIAN_POINT('Ctrl Pts',(-3.06854992020173,225.000142040112,15.7915765528225));
#79106=CARTESIAN_POINT('Ctrl Pts',(-3.06875783160601,225.504434156461,15.7655635814622));
#79107=CARTESIAN_POINT('Ctrl Pts',(-2.71259519013905,227.034352506937,15.6866313216913));
#79108=CARTESIAN_POINT('Ctrl Pts',(-0.301020073092202,228.620243817014,
15.5547797735098));
#79109=CARTESIAN_POINT('Ctrl Pts',(2.87816724394823,227.216513409565,15.396021908278));
#79110=CARTESIAN_POINT('Ctrl Pts',(3.4232560124835,223.784230016872,15.2372640430462));
#79111=CARTESIAN_POINT('Ctrl Pts',(0.835381013022407,221.464619264915,15.0785061778144));
#79112=CARTESIAN_POINT('Ctrl Pts',(-2.30174382348909,222.321765613181,14.9299436810732));
#79113=CARTESIAN_POINT('Ctrl Pts',(-3.06729084909732,224.178703529587,14.8343004727426));
#79114=CARTESIAN_POINT('Ctrl Pts',(-3.07482903252357,225.002680185515,14.7915765528225));
#79115=CARTESIAN_POINT('Origin',(0.,225.,22.2084234471774));
#79116=CARTESIAN_POINT('',(-3.07430775715862,224.997245282316,16.7915765528225));
#79117=CARTESIAN_POINT('',(-3.07321950940619,225.002809179988,16.7084234471775));
#79118=CARTESIAN_POINT('',(-3.0735,225.,22.2084234471774));
#79119=CARTESIAN_POINT('Ctrl Pts',(-3.07321950940619,225.002809179988,16.7084234471775));
#79120=CARTESIAN_POINT('Ctrl Pts',(-3.07549315238226,225.252883982405,16.6954742478977));
#79121=CARTESIAN_POINT('Ctrl Pts',(-2.93324531242376,226.5223824011,16.6296057602074));
#79122=CARTESIAN_POINT('Ctrl Pts',(-1.174429199505,228.437658549578,16.5108179841064));
#79123=CARTESIAN_POINT('Ctrl Pts',(2.25103651630915,227.851247946737,16.3520601188746));
#79124=CARTESIAN_POINT('Ctrl Pts',(3.61635370100267,224.655375334543,16.1933022536428));
#79125=CARTESIAN_POINT('Ctrl Pts',(1.67198412070606,221.77490320293,16.034544388411));
#79126=CARTESIAN_POINT('Ctrl Pts',(-1.80258526109082,221.84603953302,15.8757865231792));
#79127=CARTESIAN_POINT('Ctrl Pts',(-3.0521184279115,223.871238113346,15.7670795427681));
#79128=CARTESIAN_POINT('Ctrl Pts',(-3.0784592267095,224.94383595677,15.7112918507675));
#79129=CARTESIAN_POINT('Ctrl Pts',(-3.078224281555,224.998996872852,15.7084234471775));
#79130=CARTESIAN_POINT('Ctrl Pts',(-3.07430775715862,224.997245282316,16.7915765528225));
#79131=CARTESIAN_POINT('Ctrl Pts',(-3.06685907342071,225.804344807366,16.7497459785925));
#79132=CARTESIAN_POINT('Ctrl Pts',(-2.3277397025553,227.644568216933,16.6549961159518));
#79133=CARTESIAN_POINT('Ctrl Pts',(0.77573251337774,228.548945963627,16.5073269649006));
#79134=CARTESIAN_POINT('Ctrl Pts',(3.40229908990077,226.273239680388,16.3485690996688));
#79135=CARTESIAN_POINT('Ctrl Pts',(2.91508167139093,222.832264493646,16.189811234437));
#79136=CARTESIAN_POINT('Ctrl Pts',(-0.24001837728243,221.37520075613,16.0310533692052));
#79137=CARTESIAN_POINT('Ctrl Pts',(-2.69447339772875,222.930728603527,15.8983084753337));
#79138=CARTESIAN_POINT('Ctrl Pts',(-3.06833486863825,224.478531364404,15.8184828698728));
#79139=CARTESIAN_POINT('Ctrl Pts',(-3.06854992020173,225.000142040112,15.7915765528225));
#79140=CARTESIAN_POINT('Origin',(0.,225.,22.2084234471774));
#79141=CARTESIAN_POINT('',(-3.07760781120887,225.001583247072,17.7915765528225));
#79142=CARTESIAN_POINT('',(-3.06870238686219,224.999274066583,17.7084234471775));
#79143=CARTESIAN_POINT('',(-3.0735,225.,22.2084234471774));
#79144=CARTESIAN_POINT('Ctrl Pts',(-3.06870238686219,224.999274066583,17.7084234471775));
#79145=CARTESIAN_POINT('Ctrl Pts',(-3.06752408191027,225.556883454529,17.679656645028));
#79146=CARTESIAN_POINT('Ctrl Pts',(-2.65540744149069,227.141891306754,17.5979705544679));
#79147=CARTESIAN_POINT('Ctrl Pts',(-0.112777620733934,228.630986268181,
17.4633651754972));
#79148=CARTESIAN_POINT('Ctrl Pts',(2.98929492288558,227.064193826811,17.3046073102654));
#79149=CARTESIAN_POINT('Ctrl Pts',(3.35556487664332,223.608251232666,17.1458494450336));
#79150=CARTESIAN_POINT('Ctrl Pts',(0.650821984291496,221.426037077147,16.9870915798018));
#79151=CARTESIAN_POINT('Ctrl Pts',(-2.38035569234535,222.425914952088,16.8412829138497));
#79152=CARTESIAN_POINT('Ctrl Pts',(-3.06620149150084,224.230907232535,16.7483935363083));
#79153=CARTESIAN_POINT('Ctrl Pts',(-3.07321950940619,225.002809179988,16.7084234471775));
#79154=CARTESIAN_POINT('Ctrl Pts',(-3.07760781120886,225.001583247072,17.7915765528225));
#79155=CARTESIAN_POINT('Ctrl Pts',(-3.07817901647247,225.092570569182,17.7868476641333));
#79156=CARTESIAN_POINT('Ctrl Pts',(-3.03325241567471,226.201192212555,17.7291994870335));
#79157=CARTESIAN_POINT('Ctrl Pts',(-1.69089208164927,228.215223302252,17.6186320215231));
#79158=CARTESIAN_POINT('Ctrl Pts',(1.7840346429268,228.164490323129,17.4598741562913));
#79159=CARTESIAN_POINT('Ctrl Pts',(3.6262131814702,225.217615651258,17.3011162910595));
#79160=CARTESIAN_POINT('Ctrl Pts',(2.14968143631101,222.071579278568,17.1423584258277));
#79161=CARTESIAN_POINT('Ctrl Pts',(-1.29423861444767,221.60563336867,16.9836005605959));
#79162=CARTESIAN_POINT('Ctrl Pts',(-2.95834120127935,223.550454624517,16.8666732695942));
#79163=CARTESIAN_POINT('Ctrl Pts',(-3.07628230153224,224.783294216301,16.8026652670031));
#79164=CARTESIAN_POINT('Ctrl Pts',(-3.07430775715862,224.997245282316,16.7915765528225));
#79165=CARTESIAN_POINT('Origin',(0.,225.,22.2084234471774));
#79166=CARTESIAN_POINT('',(-3.06955363737172,225.001741577652,18.7915765528225));
#79167=CARTESIAN_POINT('',(-3.07588051624417,224.997572007392,18.7084234471775));
#79168=CARTESIAN_POINT('',(-3.0735,225.,22.2084234471774));
#79169=CARTESIAN_POINT('Ctrl Pts',(-3.07588051624417,224.997572007392,18.7084234471775));
#79170=CARTESIAN_POINT('Ctrl Pts',(-3.06844948329747,225.856669664575,18.6638390421582));
#79171=CARTESIAN_POINT('Ctrl Pts',(-2.24606376672136,227.747944926667,18.5663353487284));
#79172=CARTESIAN_POINT('Ctrl Pts',(0.958825650497796,228.503915237338,18.4159123668879));
#79173=CARTESIAN_POINT('Ctrl Pts',(3.46377878428887,226.094996727722,18.2571545016561));
#79174=CARTESIAN_POINT('Ctrl Pts',(2.79868213295254,222.683934191666,18.0983966364244));
#79175=CARTESIAN_POINT('Ctrl Pts',(-0.427768504200867,221.39253650103,17.9396387711925));
#79176=CARTESIAN_POINT('Ctrl Pts',(-2.74903334262051,223.038450531923,17.8096477081103));
#79177=CARTESIAN_POINT('Ctrl Pts',(-3.06969168675082,224.531107566481,17.7325759334386));
#79178=CARTESIAN_POINT('Ctrl Pts',(-3.06870238686219,224.999274066583,17.7084234471775));
#79179=CARTESIAN_POINT('Ctrl Pts',(-3.06955363737172,225.001741577652,18.7915765528225));
#79180=CARTESIAN_POINT('Ctrl Pts',(-3.07161643466669,225.39973657835,18.7710300612636));
#79181=CARTESIAN_POINT('Ctrl Pts',(-2.81478278977398,226.820249470738,18.697564281294));
#79182=CARTESIAN_POINT('Ctrl Pts',(-0.671786392406203,228.570068782136,
18.5711792129139));
#79183=CARTESIAN_POINT('Ctrl Pts',(2.6349094131999,227.500806238298,18.4124213476821));
#79184=CARTESIAN_POINT('Ctrl Pts',(3.53015369719777,224.142786739032,18.2536634824503));
#79185=CARTESIAN_POINT('Ctrl Pts',(1.19459285411968,221.569298229067,18.0949056172185));
#79186=CARTESIAN_POINT('Ctrl Pts',(-2.13212068041073,222.118715376741,17.9408766406759));
#79187=CARTESIAN_POINT('Ctrl Pts',(-3.07178686430458,224.074364251189,17.8397669525439));
#79188=CARTESIAN_POINT('Ctrl Pts',(-3.07760781120886,225.001583247072,17.7915765528225));
#79189=CARTESIAN_POINT('Origin',(0.,225.,22.2084234471774));
#79190=CARTESIAN_POINT('',(-3.07038312444426,224.996706709974,19.7915765528225));
#79191=CARTESIAN_POINT('',(-3.07632864029364,225.002216919788,19.7084234471775));
#79192=CARTESIAN_POINT('',(-3.0735,225.,22.2084234471774));
#79193=CARTESIAN_POINT('',(-0.793799282532889,222.030777046254,20.));
#79194=CARTESIAN_POINT('Ctrl Pts',(-0.793799282532863,222.030777046254,
20.));
#79195=CARTESIAN_POINT('Ctrl Pts',(-1.78107094869726,222.29471665351,19.9470807115894));
#79196=CARTESIAN_POINT('Ctrl Pts',(-2.87946818977925,223.336279021215,19.8776062291969));
#79197=CARTESIAN_POINT('Ctrl Pts',(-3.07279576536299,224.676472836184,19.8081317468044));
#79198=CARTESIAN_POINT('Ctrl Pts',(-3.07038312444426,224.996706709974,19.7915765528225));
#79199=CARTESIAN_POINT('',(0.795577463231005,222.025477587473,20.));
#79200=CARTESIAN_POINT('Origin',(0.,225.,20.));
#79201=CARTESIAN_POINT('Ctrl Pts',(0.795579197825938,222.025472417912,20.));
#79202=CARTESIAN_POINT('Ctrl Pts',(-0.166093587115772,221.769847778298,
19.948244384658));
#79203=CARTESIAN_POINT('Ctrl Pts',(-2.23002435410521,222.243746776087,19.8510522003838));
#79204=CARTESIAN_POINT('Ctrl Pts',(-3.06912215526932,224.127217093236,19.7538600161097));
#79205=CARTESIAN_POINT('Ctrl Pts',(-3.07632864029364,225.002216919788,19.7084234471775));
#79206=CARTESIAN_POINT('Origin',(160.,225.,22.2084234471774));
#79207=CARTESIAN_POINT('',(156.921337686793,225.000165205707,0.791576552822524));
#79208=CARTESIAN_POINT('',(156.931363809071,225.000702042684,0.708423447177432));
#79209=CARTESIAN_POINT('',(156.9265,225.,22.2084234471774));
#79210=CARTESIAN_POINT('',(160.793799282533,222.030777046254,0.));
#79211=CARTESIAN_POINT('Ctrl Pts',(156.931363809071,225.000702042684,0.708423447177431));
#79212=CARTESIAN_POINT('Ctrl Pts',(156.93052536392,225.474958108265,0.683959451760675));
#79213=CARTESIAN_POINT('Ctrl Pts',(157.257049637554,226.973918093966,0.606576167933322));
#79214=CARTESIAN_POINT('Ctrl Pts',(159.592724492903,228.609330790972,0.47627359569537));
#79215=CARTESIAN_POINT('Ctrl Pts',(162.813708975205,227.300991022112,0.317515730463582));
#79216=CARTESIAN_POINT('Ctrl Pts',(163.454303623542,223.882029725929,0.158757865231786));
#79217=CARTESIAN_POINT('Ctrl Pts',(161.781070948697,222.29471665351,0.0529192884105924));
#79218=CARTESIAN_POINT('Ctrl Pts',(160.793799282533,222.030777046254,-4.44089209850063E-15));
#79219=CARTESIAN_POINT('',(159.206200717467,222.030777046254,0.));
#79220=CARTESIAN_POINT('Origin',(160.,225.,0.));
#79221=CARTESIAN_POINT('Ctrl Pts',(156.921337686793,225.000165205707,0.791576552822524));
#79222=CARTESIAN_POINT('Ctrl Pts',(156.921331738014,225.008356241664,0.791150470866056));
#79223=CARTESIAN_POINT('Ctrl Pts',(156.925067879715,226.033866332656,0.73780510049899));
#79224=CARTESIAN_POINT('Ctrl Pts',(158.05412312597,228.067610591205,0.631540441721325));
#79225=CARTESIAN_POINT('Ctrl Pts',(161.521864702141,228.298893654481,0.472782576489533));
#79226=CARTESIAN_POINT('Ctrl Pts',(163.59662383415,225.510249900124,0.314024711257741));
#79227=CARTESIAN_POINT('Ctrl Pts',(162.389027673369,222.280093327593,0.156430519094562));
#79228=CARTESIAN_POINT('Ctrl Pts',(160.166034912224,221.769854531922,0.0517556153419853));
#79229=CARTESIAN_POINT('Ctrl Pts',(159.204403756969,222.025437709964,5.35135087284533E-15));
#79230=CARTESIAN_POINT('Origin',(160.,225.,22.2084234471774));
#79231=CARTESIAN_POINT('',(156.928544657468,225.00258189294,1.79157655282252));
#79232=CARTESIAN_POINT('',(156.926548550309,224.997190523908,1.70842344717743));
#79233=CARTESIAN_POINT('',(156.9265,225.,22.2084234471774));
#79234=CARTESIAN_POINT('Ctrl Pts',(156.926548550309,224.997190523908,1.70842344717743));
#79235=CARTESIAN_POINT('Ctrl Pts',(156.933660165655,225.775004947959,1.66814184889092));
#79236=CARTESIAN_POINT('Ctrl Pts',(157.628275269786,227.585965325339,1.57494096219383));
#79237=CARTESIAN_POINT('Ctrl Pts',(160.671798784727,228.570131009447,1.42882078708613));
#79238=CARTESIAN_POINT('Ctrl Pts',(163.363752796435,226.372061137603,1.27006292185433));
#79239=CARTESIAN_POINT('Ctrl Pts',(162.977135122943,222.918220049959,1.11130505662254));
#79240=CARTESIAN_POINT('Ctrl Pts',(159.865978920635,221.369750301164,0.952547191390749));
#79241=CARTESIAN_POINT('Ctrl Pts',(157.337757826407,222.870106331044,0.818253321575712));
#79242=CARTESIAN_POINT('Ctrl Pts',(156.932339046436,224.449071163496,0.736878740171274));
#79243=CARTESIAN_POINT('Ctrl Pts',(156.931363809071,225.000702042684,0.708423447177431));
#79244=CARTESIAN_POINT('Ctrl Pts',(156.928544657468,225.00258189294,1.79157655282252));
#79245=CARTESIAN_POINT('Ctrl Pts',(156.926043002634,225.316755878999,1.7753328679963));
#79246=CARTESIAN_POINT('Ctrl Pts',(157.114857812095,226.651522572006,1.70616989475949));
#79247=CARTESIAN_POINT('Ctrl Pts',(159.041158479961,228.50397348879,1.58408763311208));
#79248=CARTESIAN_POINT('Ctrl Pts',(162.423685640744,227.706100715127,1.42532976788028));
#79249=CARTESIAN_POINT('Ctrl Pts',(163.588053642863,224.431594906927,1.2665719026485));
#79250=CARTESIAN_POINT('Ctrl Pts',(161.468639564753,221.677313682196,1.1078140374167));
#79251=CARTESIAN_POINT('Ctrl Pts',(158.014412901123,221.963143608921,0.949482254141379));
#79252=CARTESIAN_POINT('Ctrl Pts',(156.922070575081,223.99103131721,0.844069759276654));
#79253=CARTESIAN_POINT('Ctrl Pts',(156.921337686793,225.000165205707,0.791576552822524));
#79254=CARTESIAN_POINT('Origin',(160.,225.,22.2084234471774));
#79255=CARTESIAN_POINT('',(156.930491779875,224.998331926605,2.79157655282252));
#79256=CARTESIAN_POINT('',(156.921810795731,225.001105518347,2.70842344717743));
#79257=CARTESIAN_POINT('',(156.9265,225.,22.2084234471774));
#79258=CARTESIAN_POINT('Ctrl Pts',(156.921810795731,225.001105518347,2.70842344717743));
#79259=CARTESIAN_POINT('Ctrl Pts',(156.92152721133,225.062262492373,2.70524353443178));
#79260=CARTESIAN_POINT('Ctrl Pts',(156.950896773024,226.140900456302,2.64914433327553));
#79261=CARTESIAN_POINT('Ctrl Pts',(158.215935612034,228.164543027245,2.54012584370868));
#79262=CARTESIAN_POINT('Ctrl Pts',(161.69092028973,228.215276931872,2.38136797847688));
#79263=CARTESIAN_POINT('Ctrl Pts',(163.618375178607,225.323389882532,2.22261011324509));
#79264=CARTESIAN_POINT('Ctrl Pts',(162.23429242903,222.135535662507,2.0638522480133));
#79265=CARTESIAN_POINT('Ctrl Pts',(158.805387032225,221.569240674643,1.90509438278151));
#79266=CARTESIAN_POINT('Ctrl Pts',(157.062398923068,223.489791358345,1.78661811583621));
#79267=CARTESIAN_POINT('Ctrl Pts',(156.924317397752,224.753164018422,1.72106113730152));
#79268=CARTESIAN_POINT('Ctrl Pts',(156.926548550309,224.997190523908,1.70842344717743));
#79269=CARTESIAN_POINT('Ctrl Pts',(156.930491779875,224.998331926605,2.79157655282252));
#79270=CARTESIAN_POINT('Ctrl Pts',(156.933552896885,225.619428942765,2.75951526512655));
#79271=CARTESIAN_POINT('Ctrl Pts',(157.418220432956,227.270080346152,2.67453468901999));
#79272=CARTESIAN_POINT('Ctrl Pts',(160.112779481517,228.63104619244,2.53663482450283));
#79273=CARTESIAN_POINT('Ctrl Pts',(163.111687448995,226.874731226991,2.37787695927104));
#79274=CARTESIAN_POINT('Ctrl Pts',(163.262779158505,223.402662193936,2.21911909403925));
#79275=CARTESIAN_POINT('Ctrl Pts',(160.427775566504,221.392476912117,2.06036122880746));
#79276=CARTESIAN_POINT('Ctrl Pts',(157.531399019878,222.551761497166,1.91784704840188));
#79277=CARTESIAN_POINT('Ctrl Pts',(156.934192988001,224.293228030656,1.8282521564069));
#79278=CARTESIAN_POINT('Ctrl Pts',(156.928544657468,225.00258189294,1.79157655282252));
#79279=CARTESIAN_POINT('Origin',(160.,225.,22.2084234471774));
#79280=CARTESIAN_POINT('',(156.922466247698,224.998327969291,3.79157655282252));
#79281=CARTESIAN_POINT('',(156.929815672431,225.002107482967,3.70842344717743));
#79282=CARTESIAN_POINT('',(156.9265,225.,22.2084234471774));
#79283=CARTESIAN_POINT('Ctrl Pts',(156.929815672431,225.002107482967,3.70842344717743));
#79284=CARTESIAN_POINT('Ctrl Pts',(156.927492802909,225.369927641302,3.68942593156203));
#79285=CARTESIAN_POINT('Ctrl Pts',(157.158871713077,226.759518870601,3.61750912753603));
#79286=CARTESIAN_POINT('Ctrl Pts',(159.224254559927,228.549005100767,3.49267303509943));
#79287=CARTESIAN_POINT('Ctrl Pts',(162.560827097429,227.576699973488,3.33391516986764));
#79288=CARTESIAN_POINT('Ctrl Pts',(163.553730780998,224.246199136404,3.17515730463585));
#79289=CARTESIAN_POINT('Ctrl Pts',(161.29426018331,221.605576810485,3.01639943940405));
#79290=CARTESIAN_POINT('Ctrl Pts',(157.919265447971,222.062197443487,2.86082148691792));
#79291=CARTESIAN_POINT('Ctrl Pts',(156.92624654986,224.044503891545,2.75816282284237));
#79292=CARTESIAN_POINT('Ctrl Pts',(156.921810795731,225.001105518347,2.70842344717743));
#79293=CARTESIAN_POINT('Ctrl Pts',(156.922466247698,224.998327969291,3.79157655282252));
#79294=CARTESIAN_POINT('Ctrl Pts',(156.928511093102,225.919667179771,3.74369766225681));
#79295=CARTESIAN_POINT('Ctrl Pts',(157.857683123109,227.869913232578,3.6428994832805));
#79296=CARTESIAN_POINT('Ctrl Pts',(161.174448579081,228.437715275457,3.48918201589359));
#79297=CARTESIAN_POINT('Ctrl Pts',(163.525115526208,225.877938670865,3.3304241506618));
#79298=CARTESIAN_POINT('Ctrl Pts',(162.649596882032,222.514672627688,3.17166628543));
#79299=CARTESIAN_POINT('Ctrl Pts',(159.349167276316,221.4259781011,3.01290842019821));
#79300=CARTESIAN_POINT('Ctrl Pts',(157.190613923645,223.167520967189,2.88621184266239));
#79301=CARTESIAN_POINT('Ctrl Pts',(156.928500319601,224.594266995409,2.81243455353715));
#79302=CARTESIAN_POINT('Ctrl Pts',(156.930491779875,224.998331926605,2.79157655282252));
#79303=CARTESIAN_POINT('Origin',(160.,225.,22.2084234471774));
#79304=CARTESIAN_POINT('',(156.925458918946,225.002732334518,4.79157655282252));
#79305=CARTESIAN_POINT('',(156.929435381723,224.997713479262,4.70842344717743));
#79306=CARTESIAN_POINT('',(156.9265,225.,22.2084234471774));
#79307=CARTESIAN_POINT('Ctrl Pts',(156.929435381723,224.997713479262,4.70842344717743));
#79308=CARTESIAN_POINT('Ctrl Pts',(156.934090922428,225.671576072799,4.67360832869228));
#79309=CARTESIAN_POINT('Ctrl Pts',(157.484333803602,227.376629325332,4.58587392179653));
#79310=CARTESIAN_POINT('Ctrl Pts',(160.301025089113,228.620304142684,4.44522022649019));
#79311=CARTESIAN_POINT('Ctrl Pts',(163.20476723256,226.710755732037,4.28646236125839));
#79312=CARTESIAN_POINT('Ctrl Pts',(163.175506530854,223.235523742761,4.1277044960266));
#79313=CARTESIAN_POINT('Ctrl Pts',(160.240022376856,221.375140354604,3.96894663079481));
#79314=CARTESIAN_POINT('Ctrl Pts',(157.462426236202,222.657868176513,3.82918628117842));
#79315=CARTESIAN_POINT('Ctrl Pts',(156.933963364886,224.345331507984,3.74234521997263));
#79316=CARTESIAN_POINT('Ctrl Pts',(156.929815672431,225.002107482967,3.70842344717743));
#79317=CARTESIAN_POINT('Ctrl Pts',(156.925458918946,225.002732334518,4.79157655282252));
#79318=CARTESIAN_POINT('Ctrl Pts',(156.923543600364,225.210644736276,4.78079934779765));
#79319=CARTESIAN_POINT('Ctrl Pts',(157.037552181058,226.437380685709,4.71710285436219));
#79320=CARTESIAN_POINT('Ctrl Pts',(158.685830951627,228.386764753245,4.60048707251613));
#79321=CARTESIAN_POINT('Ctrl Pts',(162.132484704811,227.941041442286,4.44172920728434));
#79322=CARTESIAN_POINT('Ctrl Pts',(163.627488540013,224.80367711901,4.28297134205255));
#79323=CARTESIAN_POINT('Ctrl Pts',(161.802615006038,221.845987488677,4.12421347682076));
#79324=CARTESIAN_POINT('Ctrl Pts',(158.327988289432,221.774849984717,3.96545561158897));
#79325=CARTESIAN_POINT('Ctrl Pts',(156.969987773211,223.786649943641,3.85457663692288));
#79326=CARTESIAN_POINT('Ctrl Pts',(156.921829883209,224.901334991466,3.7966169506674));
#79327=CARTESIAN_POINT('Ctrl Pts',(156.922466247698,224.998327969291,3.79157655282252));
#79328=CARTESIAN_POINT('Origin',(160.,225.,22.2084234471774));
#79329=CARTESIAN_POINT('',(156.93140463606,224.999957001684,5.79157655282252));
#79330=CARTESIAN_POINT('',(156.921584159768,224.999192686964,5.70842344717744));
#79331=CARTESIAN_POINT('',(156.9265,225.,22.2084234471774));
#79332=CARTESIAN_POINT('Ctrl Pts',(156.921584159768,224.999192686964,5.70842344717744));
#79333=CARTESIAN_POINT('Ctrl Pts',(156.925001457824,225.972784245262,5.65779072582253));
#79334=CARTESIAN_POINT('Ctrl Pts',(157.949607258313,227.970126972175,5.55423871605704));
#79335=CARTESIAN_POINT('Ctrl Pts',(161.351233261004,228.372148701364,5.39776741788094));
#79336=CARTESIAN_POINT('Ctrl Pts',(163.565919727063,225.69385494874,5.23900955264914));
#79337=CARTESIAN_POINT('Ctrl Pts',(162.517076599142,222.380545174315,5.08025168741736));
#79338=CARTESIAN_POINT('Ctrl Pts',(159.164605066666,221.464560353348,4.92149382218556));
#79339=CARTESIAN_POINT('Ctrl Pts',(157.144209541887,223.275517676808,4.79755107543892));
#79340=CARTESIAN_POINT('Ctrl Pts',(156.927014459328,224.647298963079,4.72652761710288));
#79341=CARTESIAN_POINT('Ctrl Pts',(156.929435381723,224.997713479262,4.70842344717743));
#79342=CARTESIAN_POINT('Ctrl Pts',(156.93140463606,224.999957001684,5.79157655282252));
#79343=CARTESIAN_POINT('Ctrl Pts',(156.931468976361,225.515539516096,5.76498174492791));
#79344=CARTESIAN_POINT('Ctrl Pts',(157.299116272149,227.057132548067,5.6854676486227));
#79345=CARTESIAN_POINT('Ctrl Pts',(159.738697422576,228.623387468178,5.55303426390689));
#79346=CARTESIAN_POINT('Ctrl Pts',(162.902351059725,227.184851049301,5.3942763986751));
#79347=CARTESIAN_POINT('Ctrl Pts',(163.409773121145,223.746739036021,5.2355185334433));
#79348=CARTESIAN_POINT('Ctrl Pts',(160.796570956179,221.455611407691,5.07676066821152));
#79349=CARTESIAN_POINT('Ctrl Pts',(157.681232421457,222.343634702093,4.92878000800458));
#79350=CARTESIAN_POINT('Ctrl Pts',(156.932948385389,224.189732883212,4.83371863620825));
#79351=CARTESIAN_POINT('Ctrl Pts',(156.925458918946,225.002732334518,4.79157655282252));
#79352=CARTESIAN_POINT('Origin',(160.,225.,22.2084234471774));
#79353=CARTESIAN_POINT('',(156.925301112762,224.997290222949,6.79157655282252));
#79354=CARTESIAN_POINT('',(156.927064836583,225.002798525488,6.70842344717744));
#79355=CARTESIAN_POINT('',(156.9265,225.,22.2084234471774));
#79356=CARTESIAN_POINT('Ctrl Pts',(156.927064836583,225.002798525488,6.70842344717744));
#79357=CARTESIAN_POINT('Ctrl Pts',(156.924720161678,225.264186795083,6.69489241136339));
#79358=CARTESIAN_POINT('Ctrl Pts',(157.074861486538,226.545199591255,6.62844208713874));
#79359=CARTESIAN_POINT('Ctrl Pts',(158.863323855727,228.450389185699,6.50907247450349));
#79360=CARTESIAN_POINT('Ctrl Pts',(162.282209040562,227.826435933279,6.35031460927169));
#79361=CARTESIAN_POINT('Ctrl Pts',(163.612416601221,224.615728625868,6.1915567440399));
#79362=CARTESIAN_POINT('Ctrl Pts',(161.636540630497,221.756706464952,6.03279887880811));
#79363=CARTESIAN_POINT('Ctrl Pts',(158.162902739098,221.865946419773,5.87404101357632));
#79364=CARTESIAN_POINT('Ctrl Pts',(156.942203746577,223.893848412542,5.76591586969943));
#79365=CARTESIAN_POINT('Ctrl Pts',(156.921429835036,224.955225419882,5.71071001423313));
#79366=CARTESIAN_POINT('Ctrl Pts',(156.921584159768,224.999192686964,5.70842344717744));
#79367=CARTESIAN_POINT('Ctrl Pts',(156.925301112762,224.997290222949,6.79157655282253));
#79368=CARTESIAN_POINT('Ctrl Pts',(156.932817764635,225.815396751321,6.74916414205816));
#79369=CARTESIAN_POINT('Ctrl Pts',(157.689098895856,227.666552960644,6.6538324428832));
#79370=CARTESIAN_POINT('Ctrl Pts',(160.814621149687,228.540283627621,6.50558145529764));
#79371=CARTESIAN_POINT('Ctrl Pts',(163.416114882048,226.235870095991,6.34682359006586));
#79372=CARTESIAN_POINT('Ctrl Pts',(162.891180408695,222.800388301109,6.18806572483405));
#79373=CARTESIAN_POINT('Ctrl Pts',(159.720237738997,221.377991046555,6.02930785960227));
#79374=CARTESIAN_POINT('Ctrl Pts',(157.293632555002,222.953434165558,5.89714480226508));
#79375=CARTESIAN_POINT('Ctrl Pts',(156.931340949756,224.489615212083,5.8179010333385));
#79376=CARTESIAN_POINT('Ctrl Pts',(156.93140463606,224.999957001684,5.79157655282252));
#79377=CARTESIAN_POINT('Origin',(160.,225.,22.2084234471774));
#79378=CARTESIAN_POINT('',(156.922579188606,225.001746898842,7.79157655282252));
#79379=CARTESIAN_POINT('',(156.931157428481,224.999096720139,7.70842344717743));
#79380=CARTESIAN_POINT('',(156.9265,225.,22.2084234471774));
#79381=CARTESIAN_POINT('Ctrl Pts',(156.931157428481,224.999096720139,7.70842344717743));
#79382=CARTESIAN_POINT('Ctrl Pts',(156.932655761039,225.567952418948,7.67907480849363));
#79383=CARTESIAN_POINT('Ctrl Pts',(157.357138295168,227.164604851287,7.59680688139924));
#79384=CARTESIAN_POINT('Ctrl Pts',(159.927049484579,228.632065034116,7.46161966589424));
#79385=CARTESIAN_POINT('Ctrl Pts',(163.011803421676,227.031319359169,7.30286180066245));
#79386=CARTESIAN_POINT('Ctrl Pts',(163.34015498569,223.57151028659,7.14410393543066));
#79387=CARTESIAN_POINT('Ctrl Pts',(160.61159683815,221.41905494355,6.98534607019886));
#79388=CARTESIAN_POINT('Ctrl Pts',(157.60356850975,222.448010774312,6.84011924078113));
#79389=CARTESIAN_POINT('Ctrl Pts',(156.933890082535,224.241908721479,6.74781169977398));
#79390=CARTESIAN_POINT('Ctrl Pts',(156.927064836583,225.002798525488,6.70842344717744));
#79391=CARTESIAN_POINT('Ctrl Pts',(156.922579188606,225.001746898842,7.79157655282252));
#79392=CARTESIAN_POINT('Ctrl Pts',(156.921884783106,225.103951698665,7.78626582759901));
#79393=CARTESIAN_POINT('Ctrl Pts',(156.972873960673,226.223885904837,7.7280358139649));
#79394=CARTESIAN_POINT('Ctrl Pts',(158.344443841372,228.233627929609,7.61688651192019));
#79395=CARTESIAN_POINT('Ctrl Pts',(161.818662966152,228.144786287979,7.4581286466884));
#79396=CARTESIAN_POINT('Ctrl Pts',(163.628441815827,225.177836359257,7.29937078145661));
#79397=CARTESIAN_POINT('Ctrl Pts',(162.117470858342,222.048130601536,7.14061291622482));
#79398=CARTESIAN_POINT('Ctrl Pts',(158.66859065457,221.61997560121,6.98185505099302));
#79399=CARTESIAN_POINT('Ctrl Pts',(157.034064229565,223.573194929989,6.86550959652559));
#79400=CARTESIAN_POINT('Ctrl Pts',(156.923439003533,224.794619706459,6.80208343046876));
#79401=CARTESIAN_POINT('Ctrl Pts',(156.925301112762,224.997290222949,6.79157655282253));
#79402=CARTESIAN_POINT('Origin',(160.,225.,22.2084234471774));
#79403=CARTESIAN_POINT('',(156.930575840473,225.001597660456,8.79157655282252));
#79404=CARTESIAN_POINT('',(156.923755330016,224.997680433942,8.70842344717743));
#79405=CARTESIAN_POINT('',(156.9265,225.,22.2084234471774));
#79406=CARTESIAN_POINT('Ctrl Pts',(156.923755330016,224.997680433942,8.70842344717744));
#79407=CARTESIAN_POINT('Ctrl Pts',(156.931061315003,225.867774151639,8.66325720562389));
#79408=CARTESIAN_POINT('Ctrl Pts',(157.77174400633,227.76966729665,8.56517167565974));
#79409=CARTESIAN_POINT('Ctrl Pts',(160.997212243665,228.493248621389,8.414166857285));
#79410=CARTESIAN_POINT('Ctrl Pts',(163.475637228661,226.056959812147,8.2554089920532));
#79411=CARTESIAN_POINT('Ctrl Pts',(162.773159158663,222.653341424392,8.09665112682142));
#79412=CARTESIAN_POINT('Ctrl Pts',(159.532685935708,221.397384872754,7.93789326158962));
#79413=CARTESIAN_POINT('Ctrl Pts',(157.239882095088,223.061204839663,7.80848403504163));
#79414=CARTESIAN_POINT('Ctrl Pts',(156.929954078905,224.542234016346,7.73199409690423));
#79415=CARTESIAN_POINT('Ctrl Pts',(156.931157428481,224.999096720139,7.70842344717743));
#79416=CARTESIAN_POINT('Ctrl Pts',(156.930575840473,225.001597660456,8.79157655282252));
#79417=CARTESIAN_POINT('Ctrl Pts',(156.928646874646,225.410927488159,8.77044822472926));
#79418=CARTESIAN_POINT('Ctrl Pts',(157.195363353794,226.843078205094,8.6964006082254));
#79419=CARTESIAN_POINT('Ctrl Pts',(159.367387257422,228.57729183873,8.56943370331094));
#79420=CARTESIAN_POINT('Ctrl Pts',(162.662226542055,227.471794008467,8.41067583807916));
#79421=CARTESIAN_POINT('Ctrl Pts',(163.520596200089,224.104110398856,8.25191797284736));
#79422=CARTESIAN_POINT('Ctrl Pts',(161.156916354245,221.556344916982,8.09316010761557));
#79423=CARTESIAN_POINT('Ctrl Pts',(157.848914905693,222.140012018685,7.93971296760729));
#79424=CARTESIAN_POINT('Ctrl Pts',(156.928804260839,224.085521060443,7.83918511600961));
#79425=CARTESIAN_POINT('Ctrl Pts',(156.922579188606,225.001746898842,7.79157655282252));
#79426=CARTESIAN_POINT('Origin',(160.,225.,22.2084234471774));
#79427=CARTESIAN_POINT('',(156.928405453258,224.99738485482,9.79157655282252));
#79428=CARTESIAN_POINT('',(156.923921594218,225.002377969191,9.70842344717744));
#79429=CARTESIAN_POINT('',(156.9265,225.,22.2084234471774));
#79430=CARTESIAN_POINT('Ctrl Pts',(156.923921594218,225.002377969191,9.70842344717744));
#79431=CARTESIAN_POINT('Ctrl Pts',(156.922594939509,225.15775743005,9.70035889116474));
#79432=CARTESIAN_POINT('Ctrl Pts',(157.003932869366,226.331337438034,9.63937504674144));
#79433=CARTESIAN_POINT('Ctrl Pts',(158.514451011063,228.315171547782,9.52547191390754));
#79434=CARTESIAN_POINT('Ctrl Pts',(161.979381312161,228.046189063538,9.36671404867575));
#79435=CARTESIAN_POINT('Ctrl Pts',(163.632781914206,224.989334468133,9.20795618344396));
#79436=CARTESIAN_POINT('Ctrl Pts',(161.961460651225,221.942240967073,9.04919831821217));
#79437=CARTESIAN_POINT('Ctrl Pts',(158.495010677376,221.693608412704,8.89044045298037));
#79438=CARTESIAN_POINT('Ctrl Pts',(157.000266331579,223.680828074275,8.77684882930213));
#79439=CARTESIAN_POINT('Ctrl Pts',(156.922501215394,224.848323809807,8.71617649403449));
#79440=CARTESIAN_POINT('Ctrl Pts',(156.923755330016,224.997680433942,8.70842344717744));
#79441=CARTESIAN_POINT('Ctrl Pts',(156.928405453258,224.99738485482,9.79157655282252));
#79442=CARTESIAN_POINT('Ctrl Pts',(156.934187923251,225.71188530638,9.75463062185951));
#79443=CARTESIAN_POINT('Ctrl Pts',(157.538401080906,227.458614330763,9.6647654024859));
#79444=CARTESIAN_POINT('Ctrl Pts',(160.446152220277,228.605296656013,9.52198089470171));
#79445=CARTESIAN_POINT('Ctrl Pts',(163.270876096285,226.580691413359,9.3632230294699));
#79446=CARTESIAN_POINT('Ctrl Pts',(163.102094297597,223.109437451357,9.20446516423812));
#79447=CARTESIAN_POINT('Ctrl Pts',(160.094275919735,221.36842625953,9.04570729900632));
#79448=CARTESIAN_POINT('Ctrl Pts',(157.411955214648,222.740409857239,8.9080777618678));
#79449=CARTESIAN_POINT('Ctrl Pts',(156.933478279124,224.385695244903,8.82336751313986));
#79450=CARTESIAN_POINT('Ctrl Pts',(156.930575840473,225.001597660456,8.79157655282252));
#79451=CARTESIAN_POINT('Origin',(160.,225.,22.2084234471774));
#79452=CARTESIAN_POINT('',(156.921326205399,224.999944058072,10.7915765528225));
#79453=CARTESIAN_POINT('',(156.931207652796,225.000808750494,10.7084234471774));
#79454=CARTESIAN_POINT('',(156.9265,225.,22.2084234471774));
#79455=CARTESIAN_POINT('Ctrl Pts',(156.931207652796,225.000808750494,10.7084234471774));
#79456=CARTESIAN_POINT('Ctrl Pts',(156.930117006851,225.463728255709,10.684541288295));
#79457=CARTESIAN_POINT('Ctrl Pts',(157.245771271414,226.950995919839,10.6077398410019));
#79458=CARTESIAN_POINT('Ctrl Pts',(159.553847739015,228.605296984961,10.4780191052983));
#79459=CARTESIAN_POINT('Ctrl Pts',(162.786890404461,227.33033475348,10.3192612400665));
#79460=CARTESIAN_POINT('Ctrl Pts',(163.469371081335,223.922650247252,10.1605033748347));
#79461=CARTESIAN_POINT('Ctrl Pts',(160.976683481002,221.500956192374,10.0017455096029));
#79462=CARTESIAN_POINT('Ctrl Pts',(157.762164521819,222.241932542296,9.85105220038383));
#79463=CARTESIAN_POINT('Ctrl Pts',(156.931300393731,224.138163730248,9.75327817957534));
#79464=CARTESIAN_POINT('Ctrl Pts',(156.923921594218,225.002377969191,9.70842344717744));
#79465=CARTESIAN_POINT('Ctrl Pts',(156.921326699174,224.999944063411,10.7915765528225));
#79466=CARTESIAN_POINT('Ctrl Pts',(156.921598761237,226.014279935961,10.7388130189898));
#79467=CARTESIAN_POINT('Ctrl Pts',(158.024018250927,228.046452679611,10.6331301967464));
#79468=CARTESIAN_POINT('Ctrl Pts',(161.485548853394,228.315171245305,10.4745280860925));
#79469=CARTESIAN_POINT('Ctrl Pts',(163.590904586142,225.55010911167,10.3157702208607));
#79470=CARTESIAN_POINT('Ctrl Pts',(162.409864582861,222.281587140667,10.1570123556289));
#79471=CARTESIAN_POINT('Ctrl Pts',(159.023316608111,221.500956511627,9.99825449039707));
#79472=CARTESIAN_POINT('Ctrl Pts',(157.110724309286,223.359076798683,9.87644255612829));
#79473=CARTESIAN_POINT('Ctrl Pts',(156.925905436132,224.688474758045,9.80754991027011));
#79474=CARTESIAN_POINT('Ctrl Pts',(156.928405453258,224.99738485482,9.79157655282252));
#79475=CARTESIAN_POINT('Origin',(160.,225.,22.2084234471774));
#79476=CARTESIAN_POINT('',(156.928242437195,225.002650545767,11.7915765528225));
#79477=CARTESIAN_POINT('',(156.926885812714,224.997194120839,11.7084234471774));
#79478=CARTESIAN_POINT('',(156.9265,225.,22.2084234471774));
#79479=CARTESIAN_POINT('Ctrl Pts',(156.926885812714,224.997194120839,11.7084234471774));
#79480=CARTESIAN_POINT('Ctrl Pts',(156.933817424723,225.763987711147,11.6687236854252));
#79481=CARTESIAN_POINT('Ctrl Pts',(157.612129510202,227.56384737007,11.5761046352624));
#79482=CARTESIAN_POINT('Ctrl Pts',(160.632612800297,228.577292165123,11.4305662966891));
#79483=CARTESIAN_POINT('Ctrl Pts',(163.348485175597,226.408852447405,11.2718084314573));
#79484=CARTESIAN_POINT('Ctrl Pts',(162.999824049866,222.951031025224,11.1130505662255));
#79485=CARTESIAN_POINT('Ctrl Pts',(159.905724071664,221.368425928184,10.9542927009937));
#79486=CARTESIAN_POINT('Ctrl Pts',(157.350375618805,222.847534603159,10.8194169946443));
#79487=CARTESIAN_POINT('Ctrl Pts',(156.932533714971,224.43796794116,10.7374605767056));
#79488=CARTESIAN_POINT('Ctrl Pts',(156.931207652796,225.000808750494,10.7084234471774));
#79489=CARTESIAN_POINT('Ctrl Pts',(156.928242437195,225.002650545767,11.7915765528225));
#79490=CARTESIAN_POINT('Ctrl Pts',(156.925748350471,225.305495671118,11.7759147045306));
#79491=CARTESIAN_POINT('Ctrl Pts',(157.10600206368,226.628710135808,11.7073335678281));
#79492=CARTESIAN_POINT('Ctrl Pts',(159.002787847321,228.493248302664,11.585833142715));
#79493=CARTESIAN_POINT('Ctrl Pts',(162.393861129102,227.732516180389,11.4270752774832));
#79494=CARTESIAN_POINT('Ctrl Pts',(163.594072799666,224.470985357276,11.2683174122514));
#79495=CARTESIAN_POINT('Ctrl Pts',(161.504989185309,221.693608714381,11.1095595470196));
#79496=CARTESIAN_POINT('Ctrl Pts',(158.038539527739,221.942241246064,10.9508016817878));
#79497=CARTESIAN_POINT('Ctrl Pts',(156.922685750034,223.976626178208,10.8448073503888));
#79498=CARTESIAN_POINT('Ctrl Pts',(156.921325896064,224.996949808778,10.7917323074004));
#79499=CARTESIAN_POINT('Ctrl Pts',(156.921326699174,224.999944063411,10.7915765528225));
#79500=CARTESIAN_POINT('Origin',(160.,225.,22.2084234471774));
#79501=CARTESIAN_POINT('',(156.930668018482,224.998485301295,12.7915765528225));
#79502=CARTESIAN_POINT('',(156.921655978846,225.000912860592,12.7084234471774));
#79503=CARTESIAN_POINT('',(156.9265,225.,22.2084234471774));
#79504=CARTESIAN_POINT('Ctrl Pts',(156.921655978846,225.000912860592,12.7084234471774));
#79505=CARTESIAN_POINT('Ctrl Pts',(156.921460221192,225.05087309577,12.7058253709661));
#79506=CARTESIAN_POINT('Ctrl Pts',(156.945200448423,226.118265565256,12.6503080063441));
#79507=CARTESIAN_POINT('Ctrl Pts',(158.181336867912,228.14478657491,12.5418713533116));
#79508=CARTESIAN_POINT('Ctrl Pts',(161.655556309681,228.233628224646,12.3831134880798));
#79509=CARTESIAN_POINT('Ctrl Pts',(163.614610681933,225.363053450345,12.224355622848));
#79510=CARTESIAN_POINT('Ctrl Pts',(162.265573500221,222.160212172565,12.0655977576162));
#79511=CARTESIAN_POINT('Ctrl Pts',(158.843083540198,221.556344602782,11.9068398923844));
#79512=CARTESIAN_POINT('Ctrl Pts',(157.070476778671,223.467003665978,11.7877817889048));
#79513=CARTESIAN_POINT('Ctrl Pts',(156.924577672169,224.741861396884,11.7216429738358));
#79514=CARTESIAN_POINT('Ctrl Pts',(156.926885812714,224.997194120839,11.7084234471774));
#79515=CARTESIAN_POINT('Ctrl Pts',(156.930668018482,224.998485301295,12.7915765528225));
#79516=CARTESIAN_POINT('Ctrl Pts',(156.933387942851,225.60839853352,12.7600971016609));
#79517=CARTESIAN_POINT('Ctrl Pts',(157.404784820172,227.247495698794,12.6756983620886));
#79518=CARTESIAN_POINT('Ctrl Pts',(160.072950508764,228.632064702726,12.5383803341058));
#79519=CARTESIAN_POINT('Ctrl Pts',(163.090939861654,226.908744758514,12.379622468874));
#79520=CARTESIAN_POINT('Ctrl Pts',(163.280101174706,223.438541686369,12.2208646036422));
#79521=CARTESIAN_POINT('Ctrl Pts',(160.467314021654,221.397385201457,12.0621067384104));
#79522=CARTESIAN_POINT('Ctrl Pts',(157.546521604723,222.529438491092,11.9190107214705));
#79523=CARTESIAN_POINT('Ctrl Pts',(156.934175535578,224.282222540545,11.8288339929412));
#79524=CARTESIAN_POINT('Ctrl Pts',(156.928242437195,225.002650545767,11.7915765528225));
#79525=CARTESIAN_POINT('Origin',(160.,225.,22.2084234471774));
#79526=CARTESIAN_POINT('',(156.922714207567,224.998169460982,13.7915765528225));
#79527=CARTESIAN_POINT('',(156.929571798648,225.002226664175,13.7084234471774));
#79528=CARTESIAN_POINT('',(156.9265,225.,22.2084234471774));
#79529=CARTESIAN_POINT('Ctrl Pts',(156.929571798648,225.002226664174,13.7084234471774));
#79530=CARTESIAN_POINT('Ctrl Pts',(156.927180610712,225.358710424651,13.6900077680964));
#79531=CARTESIAN_POINT('Ctrl Pts',(157.1492799851,226.736699514861,13.6186728006047));
#79532=CARTESIAN_POINT('Ctrl Pts',(159.185378775986,228.540283950637,13.4944185447024));
#79533=CARTESIAN_POINT('Ctrl Pts',(162.532414057892,227.604629960118,13.3356606794706));
#79534=CARTESIAN_POINT('Ctrl Pts',(163.561784093599,224.285218732523,13.1769028142388));
#79535=CARTESIAN_POINT('Ctrl Pts',(161.331409466909,221.619975292816,13.018144949007));
#79536=CARTESIAN_POINT('Ctrl Pts',(157.938969959541,222.041123564882,12.8619851599865));
#79537=CARTESIAN_POINT('Ctrl Pts',(156.92544753907,224.03325087096,12.7587446593767));
#79538=CARTESIAN_POINT('Ctrl Pts',(156.921655978846,225.000912860592,12.7084234471774));
#79539=CARTESIAN_POINT('Ctrl Pts',(156.922714207567,224.998169460982,13.7915765528225));
#79540=CARTESIAN_POINT('Ctrl Pts',(156.929131114757,225.908505372441,13.7442794987911));
#79541=CARTESIAN_POINT('Ctrl Pts',(157.838867197776,227.848532288381,13.6440631563491));
#79542=CARTESIAN_POINT('Ctrl Pts',(161.136676040562,228.450388870885,13.4909275254965));
#79543=CARTESIAN_POINT('Ctrl Pts',(163.515275045834,225.916546307426,13.3321696602647));
#79544=CARTESIAN_POINT('Ctrl Pts',(162.676694467393,222.543880599453,13.1734117950329));
#79545=CARTESIAN_POINT('Ctrl Pts',(159.388403217653,221.419055270276,13.0146539298011));
#79546=CARTESIAN_POINT('Ctrl Pts',(157.200879963145,223.14470884355,12.887375515731));
#79547=CARTESIAN_POINT('Ctrl Pts',(156.92881554858,224.583089226957,12.8130163900715));
#79548=CARTESIAN_POINT('Ctrl Pts',(156.930668018482,224.998485301295,12.7915765528225));
#79549=CARTESIAN_POINT('Origin',(160.,225.,22.2084234471774));
#79550=CARTESIAN_POINT('',(156.925120010832,225.002680229931,14.7915765528225));
#79551=CARTESIAN_POINT('',(156.929686910559,224.99782753598,14.7084234471775));
#79552=CARTESIAN_POINT('',(156.9265,225.,22.2084234471774));
#79553=CARTESIAN_POINT('Ctrl Pts',(156.929686910559,224.99782753598,14.7084234471775));
#79554=CARTESIAN_POINT('Ctrl Pts',(156.934013289436,225.660564946541,14.6741901652266));
#79555=CARTESIAN_POINT('Ctrl Pts',(157.470014842063,227.354168864685,14.5870375948652));
#79556=CARTESIAN_POINT('Ctrl Pts',(160.261302601264,228.623387798777,14.4469657360931));
#79557=CARTESIAN_POINT('Ctrl Pts',(163.185812396663,226.745799977952,14.2882078708613));
#79558=CARTESIAN_POINT('Ctrl Pts',(163.194666811915,223.270456085958,14.1294500056295));
#79559=CARTESIAN_POINT('Ctrl Pts',(160.27976228653,221.377990716082,13.9706921403978));
#79560=CARTESIAN_POINT('Ctrl Pts',(157.476644051236,222.635392093966,13.830349954247));
#79561=CARTESIAN_POINT('Ctrl Pts',(156.934051927457,224.334318825988,13.7429270565069));
#79562=CARTESIAN_POINT('Ctrl Pts',(156.929571798648,225.002226664174,13.7084234471774));
#79563=CARTESIAN_POINT('Ctrl Pts',(156.925120010832,225.002680229931,14.7915765528225));
#79564=CARTESIAN_POINT('Ctrl Pts',(156.923321116172,225.199312113646,14.781381184332));
#79565=CARTESIAN_POINT('Ctrl Pts',(157.030083060612,226.414620418541,14.7182665274308));
#79566=CARTESIAN_POINT('Ctrl Pts',(158.648766862283,228.372148393688,14.6022325821191));
#79567=CARTESIAN_POINT('Ctrl Pts',(162.100101640777,227.964251824647,14.4434747168873));
#79568=CARTESIAN_POINT('Ctrl Pts',(163.629423480216,224.843472102255,14.2847168516555));
#79569=CARTESIAN_POINT('Ctrl Pts',(161.837097093285,221.865946705725,14.1259589864237));
#79570=CARTESIAN_POINT('Ctrl Pts',(158.363459518822,221.756706760871,13.9672011211919));
#79571=CARTESIAN_POINT('Ctrl Pts',(156.976235533965,223.763970462451,13.8557403099915));
#79572=CARTESIAN_POINT('Ctrl Pts',(156.921951425256,224.889957185126,13.7971987872017));
#79573=CARTESIAN_POINT('Ctrl Pts',(156.922714207567,224.998169460982,13.7915765528225));
#79574=CARTESIAN_POINT('Origin',(160.,225.,22.2084234471774));
#79575=CARTESIAN_POINT('',(156.931399227217,225.00014204246,15.7915765528225));
#79576=CARTESIAN_POINT('',(156.921724642972,224.998996856206,15.7084234471774));
#79577=CARTESIAN_POINT('',(156.9265,225.,22.2084234471774));
#79578=CARTESIAN_POINT('Ctrl Pts',(156.921724642972,224.998996856206,15.7084234471774));
#79579=CARTESIAN_POINT('Ctrl Pts',(156.925824278053,225.961517777779,15.6583725623568));
#79580=CARTESIAN_POINT('Ctrl Pts',(157.929788518612,227.949094946038,15.5554023891257));
#79581=CARTESIAN_POINT('Ctrl Pts',(161.314169168278,228.386765062254,15.3995129274839));
#79582=CARTESIAN_POINT('Ctrl Pts',(163.558095664808,225.732921162083,15.2407550622521));
#79583=CARTESIAN_POINT('Ctrl Pts',(162.545653148823,222.408307843197,15.0819971970203));
#79584=CARTESIAN_POINT('Ctrl Pts',(159.203428971142,221.4556110843,14.9232393317885));
#79585=CARTESIAN_POINT('Ctrl Pts',(157.15371672642,223.252698357902,14.7987147485075));
#79586=CARTESIAN_POINT('Ctrl Pts',(156.927325385779,224.636076782644,14.7271094536372));
#79587=CARTESIAN_POINT('Ctrl Pts',(156.929686910559,224.99782753598,14.7084234471775));
#79588=CARTESIAN_POINT('Ctrl Pts',(156.931399227217,225.00014204246,15.7915765528225));
#79589=CARTESIAN_POINT('Ctrl Pts',(156.931191312365,225.504442516036,15.7655635814622));
#79590=CARTESIAN_POINT('Ctrl Pts',(157.287359856215,227.03438622062,15.6866313216913));
#79591=CARTESIAN_POINT('Ctrl Pts',(159.698974938352,228.620303812367,15.5547797735098));
#79592=CARTESIAN_POINT('Ctrl Pts',(162.878214941473,227.216550142046,15.396021908278));
#79593=CARTESIAN_POINT('Ctrl Pts',(163.423312743327,223.784209868902,15.2372640430462));
#79594=CARTESIAN_POINT('Ctrl Pts',(160.835394857113,221.464560675923,15.0785061778144));
#79595=CARTESIAN_POINT('Ctrl Pts',(157.69821803158,222.321721228977,14.9299436810732));
#79596=CARTESIAN_POINT('Ctrl Pts',(156.932658319183,224.178689918907,14.8343004727426));
#79597=CARTESIAN_POINT('Ctrl Pts',(156.925120010832,225.002680229931,14.7915765528225));
#79598=CARTESIAN_POINT('Origin',(160.,225.,22.2084234471774));
#79599=CARTESIAN_POINT('',(156.925641295233,224.997245236081,16.7915765528225));
#79600=CARTESIAN_POINT('',(156.926729498164,225.002809226607,16.7084234471774));
#79601=CARTESIAN_POINT('',(156.9265,225.,22.2084234471774));
#79602=CARTESIAN_POINT('Ctrl Pts',(156.926729498164,225.002809226607,16.7084234471774));
#79603=CARTESIAN_POINT('Ctrl Pts',(156.924455817463,225.252888178359,16.6954742478977));
#79604=CARTESIAN_POINT('Ctrl Pts',(157.066706017672,226.522407661068,16.6296057602073));
#79605=CARTESIAN_POINT('Ctrl Pts',(158.825551313761,228.437715589115,16.5108179841064));
#79606=CARTESIAN_POINT('Ctrl Pts',(162.251073866661,227.851295256028,16.3520601188746));
#79607=CARTESIAN_POINT('Ctrl Pts',(163.616413705393,224.655369616393,16.1933022536428));
#79608=CARTESIAN_POINT('Ctrl Pts',(161.672011863123,221.774849690454,16.034544388411));
#79609=CARTESIAN_POINT('Ctrl Pts',(158.197384829492,221.845987200903,15.8757865231793));
#79610=CARTESIAN_POINT('Ctrl Pts',(156.947830929778,223.87121938435,15.767079542768));
#79611=CARTESIAN_POINT('Ctrl Pts',(156.92148969392,224.943835024866,15.7112918507674));
#79612=CARTESIAN_POINT('Ctrl Pts',(156.921724642972,224.998996856206,15.7084234471774));
#79613=CARTESIAN_POINT('Ctrl Pts',(156.925641295233,224.997245236081,16.7915765528225));
#79614=CARTESIAN_POINT('Ctrl Pts',(156.933090102387,225.804358136565,16.7497459785925));
#79615=CARTESIAN_POINT('Ctrl Pts',(157.672221721132,227.644612044043,16.6549961159518));
#79616=CARTESIAN_POINT('Ctrl Pts',(160.775745369292,228.549004776956,16.5073269649006));
#79617=CARTESIAN_POINT('Ctrl Pts',(163.402355473271,226.273260780993,16.3485690996688));
#79618=CARTESIAN_POINT('Ctrl Pts',(162.915129980759,222.832228569406,16.189811234437));
#79619=CARTESIAN_POINT('Ctrl Pts',(159.759977645044,221.375140685337,16.0310533692052));
#79620=CARTESIAN_POINT('Ctrl Pts',(157.305481948964,222.930694311157,15.8983084753337));
#79621=CARTESIAN_POINT('Ctrl Pts',(156.931614282347,224.478522722518,15.8184828698728));
#79622=CARTESIAN_POINT('Ctrl Pts',(156.931399227217,225.00014204246,15.7915765528225));
#79623=CARTESIAN_POINT('Origin',(160.,225.,22.2084234471774));
#79624=CARTESIAN_POINT('',(156.922341197581,225.001583255068,17.7915765528225));
#79625=CARTESIAN_POINT('',(156.931246696043,224.999274061703,17.7084234471774));
#79626=CARTESIAN_POINT('',(156.9265,225.,22.2084234471774));
#79627=CARTESIAN_POINT('Ctrl Pts',(156.931246696043,224.999274061703,17.7084234471774));
#79628=CARTESIAN_POINT('Ctrl Pts',(156.932425020426,225.556892698229,17.679656645028));
#79629=CARTESIAN_POINT('Ctrl Pts',(157.344548498198,227.141926833519,17.5979705544679));
#79630=CARTESIAN_POINT('Ctrl Pts',(159.887220508192,228.631046523769,17.4633651754972));
#79631=CARTESIAN_POINT('Ctrl Pts',(162.98934452274,227.064228072664,17.3046073102654));
#79632=CARTESIAN_POINT('Ctrl Pts',(163.355620553903,223.60822814226,17.1458494450336));
#79633=CARTESIAN_POINT('Ctrl Pts',(160.650832783067,221.425977775001,16.9870915798018));
#79634=CARTESIAN_POINT('Ctrl Pts',(157.61960481157,222.425872241985,16.8412829138498));
#79635=CARTESIAN_POINT('Ctrl Pts',(156.933747632514,224.230894471467,16.7483935363083));
#79636=CARTESIAN_POINT('Ctrl Pts',(156.926729498164,225.002809226607,16.7084234471774));
#79637=CARTESIAN_POINT('Ctrl Pts',(156.922341197581,225.001583255068,17.7915765528225));
#79638=CARTESIAN_POINT('Ctrl Pts',(156.921769984656,225.092572081796,17.7868476641333));
#79639=CARTESIAN_POINT('Ctrl Pts',(156.966697348799,226.201212063418,17.7291994870335));
#79640=CARTESIAN_POINT('Ctrl Pts',(158.309079864678,228.215276638311,17.6186320215231));
#79641=CARTESIAN_POINT('Ctrl Pts',(161.78406422512,228.164542738612,17.4598741562913));
#79642=CARTESIAN_POINT('Ctrl Pts',(163.62627326692,225.217619271453,17.3011162910595));
#79643=CARTESIAN_POINT('Ctrl Pts',(162.14971706585,222.071530741175,17.1423584258277));
#79644=CARTESIAN_POINT('Ctrl Pts',(158.705739934788,221.605577120181,16.9836005605959));
#79645=CARTESIAN_POINT('Ctrl Pts',(157.041609772818,223.55043060198,16.8666732695942));
#79646=CARTESIAN_POINT('Ctrl Pts',(156.923666718143,224.783290624422,16.8026652670031));
#79647=CARTESIAN_POINT('Ctrl Pts',(156.925641295233,224.997245236081,16.7915765528225));
#79648=CARTESIAN_POINT('Origin',(160.,225.,22.2084234471774));
#79649=CARTESIAN_POINT('',(156.930395245889,225.001742688239,18.7915765528225));
#79650=CARTESIAN_POINT('',(156.924068523622,224.997572468126,18.7084234471774));
#79651=CARTESIAN_POINT('',(156.9265,225.,22.2084234471774));
#79652=CARTESIAN_POINT('Ctrl Pts',(156.924068523622,224.997572468126,18.7084234471774));
#79653=CARTESIAN_POINT('Ctrl Pts',(156.931499697293,225.856684407074,18.6638390421582));
#79654=CARTESIAN_POINT('Ctrl Pts',(157.753898863975,227.747989763203,18.5663353487284));
#79655=CARTESIAN_POINT('Ctrl Pts',(160.958841607661,228.503973810221,18.4159123668879));
#79656=CARTESIAN_POINT('Ctrl Pts',(163.46383623651,226.095014669232,18.2571545016561));
#79657=CARTESIAN_POINT('Ctrl Pts',(162.798728578809,222.6838958807,18.0983966364243));
#79658=CARTESIAN_POINT('Ctrl Pts',(159.57222439446,221.39247658273,17.9396387711925));
#79659=CARTESIAN_POINT('Ctrl Pts',(157.250921044534,223.038417999758,17.8096477081103));
#79660=CARTESIAN_POINT('Ctrl Pts',(156.93025737984,224.531099796532,17.7325759334386));
#79661=CARTESIAN_POINT('Ctrl Pts',(156.931246696043,224.999274061703,17.7084234471774));
#79662=CARTESIAN_POINT('Ctrl Pts',(156.930395245889,225.001742688239,18.7915765528225));
#79663=CARTESIAN_POINT('Ctrl Pts',(156.928332768056,225.399743321893,18.7710300612636));
#79664=CARTESIAN_POINT('Ctrl Pts',(157.185171945213,226.820276067233,18.697564281294));
#79665=CARTESIAN_POINT('Ctrl Pts',(159.328201281756,228.570130672657,18.5711792129139));
#79666=CARTESIAN_POINT('Ctrl Pts',(162.634953757174,227.500846255061,18.4124213476821));
#79667=CARTESIAN_POINT('Ctrl Pts',(163.530211822273,224.142773276525,18.2536634824503));
#79668=CARTESIAN_POINT('Ctrl Pts',(161.194612857913,221.569240989169,18.0949056172185));
#79669=CARTESIAN_POINT('Ctrl Pts',(157.867843883242,222.118667809481,17.9408766406759));
#79670=CARTESIAN_POINT('Ctrl Pts',(156.928162222561,224.074348926167,17.8397669525439));
#79671=CARTESIAN_POINT('Ctrl Pts',(156.922341197581,225.001583255068,17.7915765528225));
#79672=CARTESIAN_POINT('Origin',(160.,225.,22.2084234471774));
#79673=CARTESIAN_POINT('',(156.929637674279,224.99697422706,19.7915765528225));
#79674=CARTESIAN_POINT('',(156.923621908153,225.002226325067,19.7084234471775));
#79675=CARTESIAN_POINT('',(156.9265,225.,22.2084234471774));
#79676=CARTESIAN_POINT('',(159.206200717467,222.030777046254,20.));
#79677=CARTESIAN_POINT('Ctrl Pts',(159.206200717467,222.030777046254,20.));
#79678=CARTESIAN_POINT('Ctrl Pts',(158.218929051303,222.29471665351,19.9470807115894));
#79679=CARTESIAN_POINT('Ctrl Pts',(157.120586599505,223.3366576531,19.8776062291969));
#79680=CARTESIAN_POINT('Ctrl Pts',(156.927233150508,224.676771814036,19.8081317468044));
#79681=CARTESIAN_POINT('Ctrl Pts',(156.929637674279,224.99697422706,19.7915765528225));
#79682=CARTESIAN_POINT('',(160.795594451476,222.025442790985,20.));
#79683=CARTESIAN_POINT('Origin',(160.,225.,20.));
#79684=CARTESIAN_POINT('Ctrl Pts',(160.795596253159,222.025437437374,20.));
#79685=CARTESIAN_POINT('Ctrl Pts',(159.833965310981,221.769854476539,19.948244384658));
#79686=CARTESIAN_POINT('Ctrl Pts',(157.769883232907,222.243618109764,19.8510522003838));
#79687=CARTESIAN_POINT('Ctrl Pts',(156.930816787522,224.127195112091,19.7538600161097));
#79688=CARTESIAN_POINT('Ctrl Pts',(156.923621908153,225.002226325067,19.7084234471775));
#79689=CARTESIAN_POINT('Origin',(-160.,225.,22.2084234471774));
#79690=CARTESIAN_POINT('',(-163.078662397867,225.00016520217,0.791576552822534));
#79691=CARTESIAN_POINT('',(-163.068635962885,225.000702088854,0.708423447177441));
#79692=CARTESIAN_POINT('',(-163.0735,225.,22.2084234471774));
#79693=CARTESIAN_POINT('',(-159.206200717467,222.030777046254,0.));
#79694=CARTESIAN_POINT('Ctrl Pts',(-163.068635962885,225.000702088854,0.708423447177441));
#79695=CARTESIAN_POINT('Ctrl Pts',(-163.069474402958,225.474958141244,0.683959451760685));
#79696=CARTESIAN_POINT('Ctrl Pts',(-162.742950137614,226.973918053232,0.60657616793333));
#79697=CARTESIAN_POINT('Ctrl Pts',(-160.407275482247,228.609330107362,0.476273595695376));
#79698=CARTESIAN_POINT('Ctrl Pts',(-157.186291303474,227.300991486183,0.317515730463588));
#79699=CARTESIAN_POINT('Ctrl Pts',(-156.545696053065,223.882027393836,0.158757865231792));
#79700=CARTESIAN_POINT('Ctrl Pts',(-158.218929051303,222.29471665351,0.0529192884105984));
#79701=CARTESIAN_POINT('Ctrl Pts',(-159.206200717467,222.030777046254,0.));
#79702=CARTESIAN_POINT('',(-160.793799282533,222.030777046254,0.));
#79703=CARTESIAN_POINT('Origin',(-160.,225.,0.));
#79704=CARTESIAN_POINT('Ctrl Pts',(-163.078662397867,225.00016520217,0.791576552822534));
#79705=CARTESIAN_POINT('Ctrl Pts',(-163.078668346653,225.008356238375,0.791150470866062));
#79706=CARTESIAN_POINT('Ctrl Pts',(-163.074932205839,226.033866360525,0.737805100498993));
#79707=CARTESIAN_POINT('Ctrl Pts',(-161.945876935419,228.067610699799,0.631540441721325));
#79708=CARTESIAN_POINT('Ctrl Pts',(-158.478135238796,228.298893703494,0.472782576489533));
#79709=CARTESIAN_POINT('Ctrl Pts',(-156.403376103572,225.51024998876,0.314024711257742));
#79710=CARTESIAN_POINT('Ctrl Pts',(-157.610972173068,222.280093121964,0.156430519094562));
#79711=CARTESIAN_POINT('Ctrl Pts',(-159.833965155725,221.769854515183,0.0517556153419857));
#79712=CARTESIAN_POINT('Ctrl Pts',(-160.795596246196,222.025437627191,5.28345271179342E-15));
#79713=CARTESIAN_POINT('Origin',(-160.,225.,22.2084234471774));
#79714=CARTESIAN_POINT('',(-163.071455427707,225.00258189293,1.79157655282252));
#79715=CARTESIAN_POINT('',(-163.073451224303,224.99719052414,1.70842344717743));
#79716=CARTESIAN_POINT('',(-163.0735,225.,22.2084234471774));
#79717=CARTESIAN_POINT('Ctrl Pts',(-163.073451224303,224.99719052414,1.70842344717743));
#79718=CARTESIAN_POINT('Ctrl Pts',(-163.066339609044,225.775004891986,1.66814184889093));
#79719=CARTESIAN_POINT('Ctrl Pts',(-162.371724554443,227.585965139188,1.57494096219383));
#79720=CARTESIAN_POINT('Ctrl Pts',(-159.328201268715,228.570130738719,1.42882078708613));
#79721=CARTESIAN_POINT('Ctrl Pts',(-156.636247443033,226.37206105408,1.27006292185434));
#79722=CARTESIAN_POINT('Ctrl Pts',(-157.022865107512,222.918220169874,1.11130505662255));
#79723=CARTESIAN_POINT('Ctrl Pts',(-160.134021050498,221.369750629735,0.952547191390755));
#79724=CARTESIAN_POINT('Ctrl Pts',(-162.66224199813,222.870106397301,0.81825332157572));
#79725=CARTESIAN_POINT('Ctrl Pts',(-163.067660731426,224.449071225008,0.736878740171281));
#79726=CARTESIAN_POINT('Ctrl Pts',(-163.068635962885,225.000702088854,0.708423447177441));
#79727=CARTESIAN_POINT('Ctrl Pts',(-163.071455427707,225.00258189293,1.79157655282252));
#79728=CARTESIAN_POINT('Ctrl Pts',(-163.07395708261,225.316755887693,1.77533286799631));
#79729=CARTESIAN_POINT('Ctrl Pts',(-162.885142267915,226.65152261772,1.70616989475949));
#79730=CARTESIAN_POINT('Ctrl Pts',(-160.958841546672,228.50397358649,1.58408763311208));
#79731=CARTESIAN_POINT('Ctrl Pts',(-157.576314291936,227.706100789163,1.42532976788028));
#79732=CARTESIAN_POINT('Ctrl Pts',(-156.411946257884,224.431594893095,1.2665719026485));
#79733=CARTESIAN_POINT('Ctrl Pts',(-158.531360393914,221.677313586384,1.1078140374167));
#79734=CARTESIAN_POINT('Ctrl Pts',(-161.985587155348,221.963143531564,0.949482254141382));
#79735=CARTESIAN_POINT('Ctrl Pts',(-163.077929508605,223.991031283085,0.84406975927666));
#79736=CARTESIAN_POINT('Ctrl Pts',(-163.078662397867,225.00016520217,0.791576552822534));
#79737=CARTESIAN_POINT('Origin',(-160.,225.,22.2084234471774));
#79738=CARTESIAN_POINT('',(-163.069508305251,224.998331926558,2.79157655282253));
#79739=CARTESIAN_POINT('',(-163.07818897851,225.001105518255,2.70842344717743));
#79740=CARTESIAN_POINT('',(-163.0735,225.,22.2084234471774));
#79741=CARTESIAN_POINT('Ctrl Pts',(-163.07818897851,225.001105518255,2.70842344717743));
#79742=CARTESIAN_POINT('Ctrl Pts',(-163.078472562891,225.062262487795,2.70524353443178));
#79743=CARTESIAN_POINT('Ctrl Pts',(-163.049103003345,226.140900372622,2.64914433327553));
#79744=CARTESIAN_POINT('Ctrl Pts',(-161.784064257062,228.164542795226,2.54012584370868));
#79745=CARTESIAN_POINT('Ctrl Pts',(-158.309079834391,228.215276695892,2.38136797847689));
#79746=CARTESIAN_POINT('Ctrl Pts',(-156.381625086582,225.323389859127,2.22261011324509));
#79747=CARTESIAN_POINT('Ctrl Pts',(-157.765707735213,222.135535871982,2.0638522480133));
#79748=CARTESIAN_POINT('Ctrl Pts',(-161.194612879462,221.569240927476,1.90509438278151));
#79749=CARTESIAN_POINT('Ctrl Pts',(-162.937600862259,223.489791467657,1.78661811583622));
#79750=CARTESIAN_POINT('Ctrl Pts',(-163.075682376832,224.753164036289,1.72106113730153));
#79751=CARTESIAN_POINT('Ctrl Pts',(-163.073451224303,224.99719052414,1.70842344717743));
#79752=CARTESIAN_POINT('Ctrl Pts',(-163.069508305251,224.998331926558,2.79157655282253));
#79753=CARTESIAN_POINT('Ctrl Pts',(-163.066447188156,225.619428959942,2.75951526512656));
#79754=CARTESIAN_POINT('Ctrl Pts',(-162.581779638644,227.270080409104,2.67453468902));
#79755=CARTESIAN_POINT('Ctrl Pts',(-159.887220515355,228.631046293149,2.53663482450283));
#79756=CARTESIAN_POINT('Ctrl Pts',(-156.88831246471,226.874731278963,2.37787695927104));
#79757=CARTESIAN_POINT('Ctrl Pts',(-156.73722075101,223.402662149674,2.21911909403925));
#79758=CARTESIAN_POINT('Ctrl Pts',(-159.572224421631,221.392476811998,2.06036122880746));
#79759=CARTESIAN_POINT('Ctrl Pts',(-162.468601048588,222.551761429388,1.91784704840188));
#79760=CARTESIAN_POINT('Ctrl Pts',(-163.065807097017,224.293228010995,1.8282521564069));
#79761=CARTESIAN_POINT('Ctrl Pts',(-163.071455427707,225.00258189293,1.79157655282252));
#79762=CARTESIAN_POINT('Origin',(-160.,225.,22.2084234471774));
#79763=CARTESIAN_POINT('',(-163.07753383765,224.998327969244,3.79157655282253));
#79764=CARTESIAN_POINT('',(-163.07018410239,225.002107482812,3.70842344717744));
#79765=CARTESIAN_POINT('',(-163.0735,225.,22.2084234471774));
#79766=CARTESIAN_POINT('Ctrl Pts',(-163.07018410239,225.002107482812,3.70842344717744));
#79767=CARTESIAN_POINT('Ctrl Pts',(-163.072506971742,225.36992761417,3.68942593156203));
#79768=CARTESIAN_POINT('Ctrl Pts',(-162.841128078544,226.759518741551,3.61750912753603));
#79769=CARTESIAN_POINT('Ctrl Pts',(-160.775745383176,228.54900484047,3.49267303509943));
#79770=CARTESIAN_POINT('Ctrl Pts',(-157.439173090395,227.576699784501,3.33391516986764));
#79771=CARTESIAN_POINT('Ctrl Pts',(-156.446269479642,224.246199191696,3.17515730463585));
#79772=CARTESIAN_POINT('Ctrl Pts',(-158.705739911624,221.605577059435,3.01639943940406));
#79773=CARTESIAN_POINT('Ctrl Pts',(-162.080734399406,222.062197658976,2.86082148691792));
#79774=CARTESIAN_POINT('Ctrl Pts',(-163.073753224711,224.044503961607,2.75816282284238));
#79775=CARTESIAN_POINT('Ctrl Pts',(-163.07818897851,225.001105518255,2.70842344717743));
#79776=CARTESIAN_POINT('Ctrl Pts',(-163.077533837651,224.998327969245,3.79157655282253));
#79777=CARTESIAN_POINT('Ctrl Pts',(-163.071488992078,225.919667205275,3.74369766225681));
#79778=CARTESIAN_POINT('Ctrl Pts',(-162.142316936304,227.869913312169,3.6428994832805));
#79779=CARTESIAN_POINT('Ctrl Pts',(-158.825551388348,228.437715370794,3.48918201589359));
#79780=CARTESIAN_POINT('Ctrl Pts',(-156.474884376031,225.877938695212,3.3304241506618));
#79781=CARTESIAN_POINT('Ctrl Pts',(-157.350403044487,222.514672558763,3.17166628543001));
#79782=CARTESIAN_POINT('Ctrl Pts',(-160.650832741734,221.425978001981,3.01290842019821));
#79783=CARTESIAN_POINT('Ctrl Pts',(-162.809386154267,223.167520916372,2.88621184266239));
#79784=CARTESIAN_POINT('Ctrl Pts',(-163.071499765581,224.594266984157,2.81243455353716));
#79785=CARTESIAN_POINT('Ctrl Pts',(-163.069508305251,224.998331926558,2.79157655282253));
#79786=CARTESIAN_POINT('Origin',(-160.,225.,22.2084234471774));
#79787=CARTESIAN_POINT('',(-163.074541166319,225.002732334593,4.79157655282253));
#79788=CARTESIAN_POINT('',(-163.07056439307,224.997713479429,4.70842344717743));
#79789=CARTESIAN_POINT('',(-163.0735,225.,22.2084234471774));
#79790=CARTESIAN_POINT('Ctrl Pts',(-163.07056439307,224.997713479429,4.70842344717743));
#79791=CARTESIAN_POINT('Ctrl Pts',(-163.065908852707,225.671576023543,4.67360832869228));
#79792=CARTESIAN_POINT('Ctrl Pts',(-162.51566601189,227.376629151021,4.58587392179654));
#79793=CARTESIAN_POINT('Ctrl Pts',(-159.698974932965,228.620303877157,4.44522022649019));
#79794=CARTESIAN_POINT('Ctrl Pts',(-156.79523300249,226.710755606563,4.28646236125839));
#79795=CARTESIAN_POINT('Ctrl Pts',(-156.82449370205,223.235523872175,4.1277044960266));
#79796=CARTESIAN_POINT('Ctrl Pts',(-159.759977640748,221.375140620465,3.96894663079481));
#79797=CARTESIAN_POINT('Ctrl Pts',(-162.537573577682,222.657868348294,3.82918628117842));
#79798=CARTESIAN_POINT('Ctrl Pts',(-163.066036410239,224.345331556,3.74234521997263));
#79799=CARTESIAN_POINT('Ctrl Pts',(-163.07018410239,225.002107482812,3.70842344717744));
#79800=CARTESIAN_POINT('Ctrl Pts',(-163.074541166319,225.002732334593,4.79157655282253));
#79801=CARTESIAN_POINT('Ctrl Pts',(-163.076456484954,225.210644742118,4.78079934779766));
#79802=CARTESIAN_POINT('Ctrl Pts',(-162.962447901099,226.437380725571,4.71710285436219));
#79803=CARTESIAN_POINT('Ctrl Pts',(-161.314169084819,228.386764847169,4.60048707251614));
#79804=CARTESIAN_POINT('Ctrl Pts',(-157.867515236049,227.941041523849,4.44172920728434));
#79805=CARTESIAN_POINT('Ctrl Pts',(-156.372511359387,224.803677113565,4.28297134205255));
#79806=CARTESIAN_POINT('Ctrl Pts',(-158.197384943971,221.845987401207,4.12421347682076));
#79807=CARTESIAN_POINT('Ctrl Pts',(-161.672011756938,221.774849895275,3.96545561158897));
#79808=CARTESIAN_POINT('Ctrl Pts',(-163.03001231082,223.786649909991,3.85457663692289));
#79809=CARTESIAN_POINT('Ctrl Pts',(-163.078170202158,224.90133498873,3.79661695066741));
#79810=CARTESIAN_POINT('Ctrl Pts',(-163.077533837651,224.998327969245,3.79157655282253));
#79811=CARTESIAN_POINT('Origin',(-160.,225.,22.2084234471774));
#79812=CARTESIAN_POINT('',(-163.068595449041,224.999957001683,5.79157655282253));
#79813=CARTESIAN_POINT('',(-163.078415614449,224.999192687023,5.70842344717743));
#79814=CARTESIAN_POINT('',(-163.0735,225.,22.2084234471774));
#79815=CARTESIAN_POINT('Ctrl Pts',(-163.078415614449,224.999192687023,5.70842344717743));
#79816=CARTESIAN_POINT('Ctrl Pts',(-163.074998316644,225.972784173914,5.65779072582253));
#79817=CARTESIAN_POINT('Ctrl Pts',(-162.050392591303,227.970126754334,5.55423871605704));
#79818=CARTESIAN_POINT('Ctrl Pts',(-158.648766838101,228.372148454037,5.39776741788094));
#79819=CARTESIAN_POINT('Ctrl Pts',(-156.434080534475,225.69385489785,5.23900955264915));
#79820=CARTESIAN_POINT('Ctrl Pts',(-157.48292358547,222.380545366436,5.08025168741736));
#79821=CARTESIAN_POINT('Ctrl Pts',(-160.835394872063,221.464560612651,4.92149382218557));
#79822=CARTESIAN_POINT('Ctrl Pts',(-162.855790248658,223.275517803288,4.79755107543892));
#79823=CARTESIAN_POINT('Ctrl Pts',(-163.072985315288,224.647298988948,4.72652761710288));
#79824=CARTESIAN_POINT('Ctrl Pts',(-163.07056439307,224.997713479429,4.70842344717743));
#79825=CARTESIAN_POINT('Ctrl Pts',(-163.068595449041,224.999957001683,5.79157655282253));
#79826=CARTESIAN_POINT('Ctrl Pts',(-163.068531108738,225.515539530394,5.76498174492791));
#79827=CARTESIAN_POINT('Ctrl Pts',(-162.700883802754,227.057132605117,5.6854676486227));
#79828=CARTESIAN_POINT('Ctrl Pts',(-160.26130258467,228.623387568664,5.5530342639069));
#79829=CARTESIAN_POINT('Ctrl Pts',(-157.097648859785,227.184851109893,5.39427639867509));
#79830=CARTESIAN_POINT('Ctrl Pts',(-156.590226784293,223.746739001265,5.23551853344331));
#79831=CARTESIAN_POINT('Ctrl Pts',(-159.203429021729,221.455611309395,5.07676066821151));
#79832=CARTESIAN_POINT('Ctrl Pts',(-162.318767642849,222.343634628425,4.92878000800459));
#79833=CARTESIAN_POINT('Ctrl Pts',(-163.067051699669,224.189732860741,4.83371863620826));
#79834=CARTESIAN_POINT('Ctrl Pts',(-163.074541166319,225.002732334593,4.79157655282253));
#79835=CARTESIAN_POINT('Origin',(-160.,225.,22.2084234471774));
#79836=CARTESIAN_POINT('',(-163.074698972508,224.997290222874,6.79157655282254));
#79837=CARTESIAN_POINT('',(-163.072934938036,225.002798525283,6.70842344717744));
#79838=CARTESIAN_POINT('',(-163.0735,225.,22.2084234471774));
#79839=CARTESIAN_POINT('Ctrl Pts',(-163.072934938036,225.002798525283,6.70842344717744));
#79840=CARTESIAN_POINT('Ctrl Pts',(-163.075279612769,225.264186775707,6.69489241136339));
#79841=CARTESIAN_POINT('Ctrl Pts',(-162.925138298921,226.545199477924,6.62844208713874));
#79842=CARTESIAN_POINT('Ctrl Pts',(-161.136676060905,228.450388932634,6.50907247450349));
#79843=CARTESIAN_POINT('Ctrl Pts',(-157.717791126824,227.826435725977,6.3503146092717));
#79844=CARTESIAN_POINT('Ctrl Pts',(-156.387583663728,224.615728654052,6.1915567440399));
#79845=CARTESIAN_POINT('Ctrl Pts',(-158.363459489534,221.756706702828,6.03279887880811));
#79846=CARTESIAN_POINT('Ctrl Pts',(-161.837097126162,221.865946649636,5.87404101357632));
#79847=CARTESIAN_POINT('Ctrl Pts',(-163.057796029152,223.893848493671,5.76591586969943));
#79848=CARTESIAN_POINT('Ctrl Pts',(-163.078569939169,224.955225423166,5.71071001423313));
#79849=CARTESIAN_POINT('Ctrl Pts',(-163.078415614449,224.999192687023,5.70842344717743));
#79850=CARTESIAN_POINT('Ctrl Pts',(-163.074698972508,224.997290222874,6.79157655282254));
#79851=CARTESIAN_POINT('Ctrl Pts',(-163.067182320426,225.815396773934,6.74916414205817));
#79852=CARTESIAN_POINT('Ctrl Pts',(-162.310901168231,227.666553034595,6.65383244288321));
#79853=CARTESIAN_POINT('Ctrl Pts',(-159.185378827721,228.540283725802,6.50558145529764));
#79854=CARTESIAN_POINT('Ctrl Pts',(-156.583885023213,226.235870130265,6.34682359006585));
#79855=CARTESIAN_POINT('Ctrl Pts',(-157.108819511125,222.800388240108,6.18806572483406));
#79856=CARTESIAN_POINT('Ctrl Pts',(-160.279762268762,221.377990946107,6.02930785960227));
#79857=CARTESIAN_POINT('Ctrl Pts',(-162.706367520053,222.953434108801,5.89714480226509));
#79858=CARTESIAN_POINT('Ctrl Pts',(-163.068659135346,224.489615197929,5.81790103333851));
#79859=CARTESIAN_POINT('Ctrl Pts',(-163.068595449041,224.999957001683,5.79157655282253));
#79860=CARTESIAN_POINT('Origin',(-160.,225.,22.2084234471774));
#79861=CARTESIAN_POINT('',(-163.077420896739,225.00174689889,7.79157655282253));
#79862=CARTESIAN_POINT('',(-163.068842346438,224.999096720205,7.70842344717744));
#79863=CARTESIAN_POINT('',(-163.0735,225.,22.2084234471774));
#79864=CARTESIAN_POINT('Ctrl Pts',(-163.068842346438,224.999096720205,7.70842344717744));
#79865=CARTESIAN_POINT('Ctrl Pts',(-163.06734401399,225.567952377292,7.67907480849364));
#79866=CARTESIAN_POINT('Ctrl Pts',(-162.642861510995,227.164604692527,7.59680688139924));
#79867=CARTESIAN_POINT('Ctrl Pts',(-160.07295051007,228.632064767727,7.46161966589424));
#79868=CARTESIAN_POINT('Ctrl Pts',(-156.988196799222,227.031319210184,7.30286180066245));
#79869=CARTESIAN_POINT('Ctrl Pts',(-156.65984525929,223.571510391361,7.14410393543066));
#79870=CARTESIAN_POINT('Ctrl Pts',(-159.388403206707,221.41905520619,6.98534607019887));
#79871=CARTESIAN_POINT('Ctrl Pts',(-162.396431314486,222.448010961485,6.84011924078112));
#79872=CARTESIAN_POINT('Ctrl Pts',(-163.066109692584,224.241908777081,6.74781169977398));
#79873=CARTESIAN_POINT('Ctrl Pts',(-163.072934938036,225.002798525283,6.70842344717744));
#79874=CARTESIAN_POINT('Ctrl Pts',(-163.077420896739,225.00174689889,7.79157655282253));
#79875=CARTESIAN_POINT('Ctrl Pts',(-163.078115302259,225.103951701548,7.78626582759902));
#79876=CARTESIAN_POINT('Ctrl Pts',(-163.027126123278,226.223885938778,7.7280358139649));
#79877=CARTESIAN_POINT('Ctrl Pts',(-161.655556204541,228.233628019286,7.61688651192019));
#79878=CARTESIAN_POINT('Ctrl Pts',(-158.181336983412,228.144786375193,7.45812864668841));
#79879=CARTESIAN_POINT('Ctrl Pts',(-156.371558083546,225.177836364189,7.2993707814566));
#79880=CARTESIAN_POINT('Ctrl Pts',(-157.882529082935,222.048130519673,7.14061291622482));
#79881=CARTESIAN_POINT('Ctrl Pts',(-161.331409382354,221.619975507472,6.98185505099302));
#79882=CARTESIAN_POINT('Ctrl Pts',(-162.965935852688,223.57319489042,6.8655095965256));
#79883=CARTESIAN_POINT('Ctrl Pts',(-163.076561081789,224.794619700763,6.80208343046877));
#79884=CARTESIAN_POINT('Ctrl Pts',(-163.074698972508,224.997290222874,6.79157655282254));
#79885=CARTESIAN_POINT('Origin',(-160.,225.,22.2084234471774));
#79886=CARTESIAN_POINT('',(-163.06942424465,225.0015976605,8.79157655282253));
#79887=CARTESIAN_POINT('',(-163.07624444436,224.997680434113,8.70842344717744));
#79888=CARTESIAN_POINT('',(-163.0735,225.,22.2084234471774));
#79889=CARTESIAN_POINT('Ctrl Pts',(-163.07624444436,224.997680434113,8.70842344717744));
#79890=CARTESIAN_POINT('Ctrl Pts',(-163.068938459909,225.867774087993,8.66325720562389));
#79891=CARTESIAN_POINT('Ctrl Pts',(-162.228255830241,227.769667093511,8.56517167565974));
#79892=CARTESIAN_POINT('Ctrl Pts',(-159.002787829475,228.493248365181,8.414166857285));
#79893=CARTESIAN_POINT('Ctrl Pts',(-156.524363026255,226.056959734625,8.2554089920532));
#79894=CARTESIAN_POINT('Ctrl Pts',(-157.226841044731,222.653341596505,8.09665112682142));
#79895=CARTESIAN_POINT('Ctrl Pts',(-160.467314030017,221.397385136983,7.93789326158962));
#79896=CARTESIAN_POINT('Ctrl Pts',(-162.760117702474,223.061204981861,7.80848403504163));
#79897=CARTESIAN_POINT('Ctrl Pts',(-163.070045695926,224.54223404992,7.73199409690424));
#79898=CARTESIAN_POINT('Ctrl Pts',(-163.068842346438,224.999096720205,7.70842344717744));
#79899=CARTESIAN_POINT('Ctrl Pts',(-163.06942424465,225.0015976605,8.79157655282253));
#79900=CARTESIAN_POINT('Ctrl Pts',(-163.071353210531,225.410927499555,8.77044822472927));
#79901=CARTESIAN_POINT('Ctrl Pts',(-162.804636723986,226.843078256208,8.69640060822541));
#79902=CARTESIAN_POINT('Ctrl Pts',(-160.632612760122,228.577291937938,8.56943370331094));
#79903=CARTESIAN_POINT('Ctrl Pts',(-157.337773384114,227.471794077016,8.41067583807916));
#79904=CARTESIAN_POINT('Ctrl Pts',(-156.479403702276,224.10411037401,8.25191797284736));
#79905=CARTESIAN_POINT('Ctrl Pts',(-158.843083613671,221.55634482148,8.09316010761557));
#79906=CARTESIAN_POINT('Ctrl Pts',(-162.151085153962,222.14001193937,7.93971296760729));
#79907=CARTESIAN_POINT('Ctrl Pts',(-163.071195824334,224.085521035082,7.83918511600961));
#79908=CARTESIAN_POINT('Ctrl Pts',(-163.077420896739,225.00174689889,7.79157655282253));
#79909=CARTESIAN_POINT('Origin',(-160.,225.,22.2084234471774));
#79910=CARTESIAN_POINT('',(-163.071594631926,224.997384854747,9.79157655282253));
#79911=CARTESIAN_POINT('',(-163.07607818017,225.002377969017,9.70842344717744));
#79912=CARTESIAN_POINT('',(-163.0735,225.,22.2084234471774));
#79913=CARTESIAN_POINT('Ctrl Pts',(-163.07607818017,225.002377969017,9.70842344717744));
#79914=CARTESIAN_POINT('Ctrl Pts',(-163.077404834783,225.157757418479,9.70035889116474));
#79915=CARTESIAN_POINT('Ctrl Pts',(-162.99606691089,226.331337340389,9.63937504674144));
#79916=CARTESIAN_POINT('Ctrl Pts',(-161.485548879981,228.315171304634,9.52547191390754));
#79917=CARTESIAN_POINT('Ctrl Pts',(-158.020618833015,228.046188840119,9.36671404867576));
#79918=CARTESIAN_POINT('Ctrl Pts',(-156.367218352237,224.989334468915,9.20795618344395));
#79919=CARTESIAN_POINT('Ctrl Pts',(-158.038539492636,221.942241191341,9.04919831821217));
#79920=CARTESIAN_POINT('Ctrl Pts',(-161.504989212242,221.693608655208,8.89044045298038));
#79921=CARTESIAN_POINT('Ctrl Pts',(-162.999733448409,223.680828171028,8.77684882930214));
#79922=CARTESIAN_POINT('Ctrl Pts',(-163.07749855889,224.848323820932,8.71617649403449));
#79923=CARTESIAN_POINT('Ctrl Pts',(-163.07624444436,224.997680434113,8.70842344717744));
#79924=CARTESIAN_POINT('Ctrl Pts',(-163.071594631926,224.997384854747,9.79157655282253));
#79925=CARTESIAN_POINT('Ctrl Pts',(-163.065812161773,225.711885326123,9.75463062185952));
#79926=CARTESIAN_POINT('Ctrl Pts',(-162.461598987361,227.458614398947,9.66476540248591));
#79927=CARTESIAN_POINT('Ctrl Pts',(-159.55384776735,228.605296755998,9.52198089470171));
#79928=CARTESIAN_POINT('Ctrl Pts',(-156.729123813004,226.580691457195,9.36322302946991));
#79929=CARTESIAN_POINT('Ctrl Pts',(-156.897905616373,223.109437398927,9.20446516423812));
#79930=CARTESIAN_POINT('Ctrl Pts',(-159.90572407765,221.368426158816,9.04570729900633));
#79931=CARTESIAN_POINT('Ctrl Pts',(-162.588044857126,222.740409794574,8.90807776186779));
#79932=CARTESIAN_POINT('Ctrl Pts',(-163.066521805919,224.385695227867,8.82336751313987));
#79933=CARTESIAN_POINT('Ctrl Pts',(-163.06942424465,225.0015976605,8.79157655282253));
#79934=CARTESIAN_POINT('Origin',(-160.,225.,22.2084234471774));
#79935=CARTESIAN_POINT('',(-163.078673879984,224.99994405807,10.7915765528225));
#79936=CARTESIAN_POINT('',(-163.068792122127,225.000808750435,10.7084234471774));
#79937=CARTESIAN_POINT('',(-163.0735,225.,22.2084234471774));
#79938=CARTESIAN_POINT('Ctrl Pts',(-163.068792122127,225.000808750435,10.7084234471774));
#79939=CARTESIAN_POINT('Ctrl Pts',(-163.069882767991,225.463728221697,10.684541288295));
#79940=CARTESIAN_POINT('Ctrl Pts',(-162.75422852658,226.950995776746,10.6077398410019));
#79941=CARTESIAN_POINT('Ctrl Pts',(-160.446152228262,228.605296720535,10.4780191052983));
#79942=CARTESIAN_POINT('Ctrl Pts',(-157.213109799941,227.330334582564,10.3192612400665));
#79943=CARTESIAN_POINT('Ctrl Pts',(-156.530629173122,223.922650326269,10.1605033748347));
#79944=CARTESIAN_POINT('Ctrl Pts',(-159.023316590632,221.500956449007,10.0017455096029));
#79945=CARTESIAN_POINT('Ctrl Pts',(-162.237835314049,222.241932744583,9.85105220038383));
#79946=CARTESIAN_POINT('Ctrl Pts',(-163.068699381198,224.138163793459,9.75327817957534));
#79947=CARTESIAN_POINT('Ctrl Pts',(-163.07607818017,225.002377969017,9.70842344717744));
#79948=CARTESIAN_POINT('Ctrl Pts',(-163.078673386206,224.999944063409,10.7915765528225));
#79949=CARTESIAN_POINT('Ctrl Pts',(-163.078401324136,226.01427996409,10.7388130189898));
#79950=CARTESIAN_POINT('Ctrl Pts',(-161.975981803872,228.046452764098,10.6331301967464));
#79951=CARTESIAN_POINT('Ctrl Pts',(-158.514451105407,228.315171337243,10.4745280860925));
#79952=CARTESIAN_POINT('Ctrl Pts',(-156.409095314272,225.550109126926,10.3157702208607));
#79953=CARTESIAN_POINT('Ctrl Pts',(-157.590135350307,222.281587065278,10.1570123556289));
#79954=CARTESIAN_POINT('Ctrl Pts',(-160.976683418975,221.500956414589,9.99825449039708));
#79955=CARTESIAN_POINT('Ctrl Pts',(-162.889275770842,223.359076753176,9.8764425561283));
#79956=CARTESIAN_POINT('Ctrl Pts',(-163.074094649121,224.688474749405,9.80754991027012));
#79957=CARTESIAN_POINT('Ctrl Pts',(-163.071594631926,224.997384854747,9.79157655282253));
#79958=CARTESIAN_POINT('Origin',(-160.,225.,22.2084234471774));
#79959=CARTESIAN_POINT('',(-163.071757647993,225.00265054584,11.7915765528225));
#79960=CARTESIAN_POINT('',(-163.073113961892,224.997194121045,11.7084234471774));
#79961=CARTESIAN_POINT('',(-163.0735,225.,22.2084234471774));
#79962=CARTESIAN_POINT('Ctrl Pts',(-163.073113961892,224.997194121045,11.7084234471774));
#79963=CARTESIAN_POINT('Ctrl Pts',(-163.066182350392,225.763987655113,11.6687236854252));
#79964=CARTESIAN_POINT('Ctrl Pts',(-162.387870314662,227.563847182028,11.5761046352624));
#79965=CARTESIAN_POINT('Ctrl Pts',(-159.367387246101,228.577291902751,11.4305662966891));
#79966=CARTESIAN_POINT('Ctrl Pts',(-156.651515069994,226.408852344075,11.2718084314573));
#79967=CARTESIAN_POINT('Ctrl Pts',(-157.000176170152,222.951031175503,11.1130505662255));
#79968=CARTESIAN_POINT('Ctrl Pts',(-160.094275921422,221.368426194538,10.9542927009937));
#79969=CARTESIAN_POINT('Ctrl Pts',(-162.649624186861,222.847534761029,10.8194169946443));
#79970=CARTESIAN_POINT('Ctrl Pts',(-163.067466060049,224.437967982382,10.7374605767056));
#79971=CARTESIAN_POINT('Ctrl Pts',(-163.068792122127,225.000808750435,10.7084234471774));
#79972=CARTESIAN_POINT('Ctrl Pts',(-163.071757647993,225.00265054584,11.7915765528225));
#79973=CARTESIAN_POINT('Ctrl Pts',(-163.074251734786,225.30549567959,11.7759147045306));
#79974=CARTESIAN_POINT('Ctrl Pts',(-162.893998016579,226.628710180977,11.7073335678281));
#79975=CARTESIAN_POINT('Ctrl Pts',(-160.997212180335,228.493248399541,11.585833142715));
#79976=CARTESIAN_POINT('Ctrl Pts',(-157.606138804509,227.732516256169,11.4270752774832));
#79977=CARTESIAN_POINT('Ctrl Pts',(-156.40592710066,224.470985342605,11.2683174122514));
#79978=CARTESIAN_POINT('Ctrl Pts',(-158.495010772954,221.693608622685,11.1095595470196));
#79979=CARTESIAN_POINT('Ctrl Pts',(-161.961460526658,221.942241161264,10.9508016817878));
#79980=CARTESIAN_POINT('Ctrl Pts',(-163.077314335309,223.976626149827,10.8448073503888));
#79981=CARTESIAN_POINT('Ctrl Pts',(-163.078674189316,224.996949808694,10.7917323074004));
#79982=CARTESIAN_POINT('Ctrl Pts',(-163.078673386206,224.999944063409,10.7915765528225));
#79983=CARTESIAN_POINT('Origin',(-160.,225.,22.2084234471774));
#79984=CARTESIAN_POINT('',(-163.069332066639,224.998485301253,12.7915765528225));
#79985=CARTESIAN_POINT('',(-163.078343795376,225.000912860525,12.7084234471774));
#79986=CARTESIAN_POINT('',(-163.0735,225.,22.2084234471774));
#79987=CARTESIAN_POINT('Ctrl Pts',(-163.078343795376,225.000912860525,12.7084234471774));
#79988=CARTESIAN_POINT('Ctrl Pts',(-163.078539553016,225.050873092039,12.7058253709661));
#79989=CARTESIAN_POINT('Ctrl Pts',(-163.054799327526,226.118265483238,12.6503080063441));
#79990=CARTESIAN_POINT('Ctrl Pts',(-161.8186629987,228.14478634426,12.5418713533116));
#79991=CARTESIAN_POINT('Ctrl Pts',(-158.344443811744,228.233627987479,12.3831134880798));
#79992=CARTESIAN_POINT('Ctrl Pts',(-156.385389583177,225.363053423717,12.224355622848));
#79993=CARTESIAN_POINT('Ctrl Pts',(-157.734426665945,222.160212380846,12.0655977576162));
#79994=CARTESIAN_POINT('Ctrl Pts',(-161.156916374949,221.556344855353,11.9068398923844));
#79995=CARTESIAN_POINT('Ctrl Pts',(-162.929523006467,223.467003778414,11.7877817889048));
#79996=CARTESIAN_POINT('Ctrl Pts',(-163.075422102268,224.741861415817,11.7216429738358));
#79997=CARTESIAN_POINT('Ctrl Pts',(-163.073113961892,224.997194121045,11.7084234471774));
#79998=CARTESIAN_POINT('Ctrl Pts',(-163.069332066639,224.998485301253,12.7915765528225));
#79999=CARTESIAN_POINT('Ctrl Pts',(-163.066612142194,225.608398550393,12.7600971016609));
#80000=CARTESIAN_POINT('Ctrl Pts',(-162.595215251801,227.247495761124,12.6756983620886));
#80001=CARTESIAN_POINT('Ctrl Pts',(-159.927049489213,228.632064803453,12.5383803341058));
#80002=CARTESIAN_POINT('Ctrl Pts',(-156.909060052626,226.908744811449,12.379622468874));
#80003=CARTESIAN_POINT('Ctrl Pts',(-156.719898734327,223.438541643066,12.2208646036422));
#80004=CARTESIAN_POINT('Ctrl Pts',(-159.532685965386,221.397385101546,12.0621067384104));
#80005=CARTESIAN_POINT('Ctrl Pts',(-162.453478463319,222.529438422577,11.9190107214705));
#80006=CARTESIAN_POINT('Ctrl Pts',(-163.065824549446,224.282222520639,11.8288339929412));
#80007=CARTESIAN_POINT('Ctrl Pts',(-163.071757647993,225.00265054584,11.7915765528225));
#80008=CARTESIAN_POINT('Origin',(-160.,225.,22.2084234471774));
#80009=CARTESIAN_POINT('',(-163.077285877774,224.998169460932,13.7915765528225));
#80010=CARTESIAN_POINT('',(-163.070427976155,225.002226664011,13.7084234471774));
#80011=CARTESIAN_POINT('',(-163.0735,225.,22.2084234471774));
#80012=CARTESIAN_POINT('Ctrl Pts',(-163.070427976155,225.002226664011,13.7084234471774));
#80013=CARTESIAN_POINT('Ctrl Pts',(-163.072819163915,225.358710398342,13.6900077680963));
#80014=CARTESIAN_POINT('Ctrl Pts',(-162.850719805817,226.736699387485,13.6186728006046));
#80015=CARTESIAN_POINT('Ctrl Pts',(-160.814621164266,228.540283690979,13.4944185447024));
#80016=CARTESIAN_POINT('Ctrl Pts',(-157.467586127845,227.604629769084,13.3356606794706));
#80017=CARTESIAN_POINT('Ctrl Pts',(-156.438216167636,224.285218784948,13.1769028142388));
#80018=CARTESIAN_POINT('Ctrl Pts',(-158.668590630742,221.61997554072,13.018144949007));
#80019=CARTESIAN_POINT('Ctrl Pts',(-162.061029889295,222.041123781898,12.8619851599865));
#80020=CARTESIAN_POINT('Ctrl Pts',(-163.07455223543,224.033250941865,12.7587446593767));
#80021=CARTESIAN_POINT('Ctrl Pts',(-163.078343795376,225.000912860525,12.7084234471774));
#80022=CARTESIAN_POINT('Ctrl Pts',(-163.077285877774,224.998169460932,13.7915765528225));
#80023=CARTESIAN_POINT('Ctrl Pts',(-163.070868970407,225.908505397637,13.7442794987911));
#80024=CARTESIAN_POINT('Ctrl Pts',(-162.161132862158,227.848532367378,13.6440631563491));
#80025=CARTESIAN_POINT('Ctrl Pts',(-158.863323927915,228.450388966574,13.4909275254965));
#80026=CARTESIAN_POINT('Ctrl Pts',(-156.484724856678,225.916546332844,13.3321696602647));
#80027=CARTESIAN_POINT('Ctrl Pts',(-157.323305458375,222.543880531338,13.1734117950329));
#80028=CARTESIAN_POINT('Ctrl Pts',(-160.611596799308,221.419055170966,13.0146539298011));
#80029=CARTESIAN_POINT('Ctrl Pts',(-162.799120114483,223.144708792098,12.887375515731));
#80030=CARTESIAN_POINT('Ctrl Pts',(-163.071184536592,224.583089215395,12.8130163900715));
#80031=CARTESIAN_POINT('Ctrl Pts',(-163.069332066639,224.998485301253,12.7915765528225));
#80032=CARTESIAN_POINT('Origin',(-160.,225.,22.2084234471774));
#80033=CARTESIAN_POINT('',(-163.074880074443,225.002680230006,14.7915765528225));
#80034=CARTESIAN_POINT('',(-163.070312864252,224.997827536139,14.7084234471775));
#80035=CARTESIAN_POINT('',(-163.0735,225.,22.2084234471774));
#80036=CARTESIAN_POINT('Ctrl Pts',(-163.070312864252,224.997827536139,14.7084234471775));
#80037=CARTESIAN_POINT('Ctrl Pts',(-163.065986485692,225.660564898092,14.6741901652266));
#80038=CARTESIAN_POINT('Ctrl Pts',(-162.529984972378,227.354168692021,14.5870375948652));
#80039=CARTESIAN_POINT('Ctrl Pts',(-159.738697417901,228.623387533023,14.4469657360931));
#80040=CARTESIAN_POINT('Ctrl Pts',(-156.814187836997,226.745799849908,14.2882078708613));
#80041=CARTESIAN_POINT('Ctrl Pts',(-156.805333422394,223.270456212809,14.1294500056295));
#80042=CARTESIAN_POINT('Ctrl Pts',(-159.720237733989,221.377990981734,13.9706921403977));
#80043=CARTESIAN_POINT('Ctrl Pts',(-162.523355763691,222.635392267396,13.830349954247));
#80044=CARTESIAN_POINT('Ctrl Pts',(-163.065947847675,224.334318874811,13.7429270565069));
#80045=CARTESIAN_POINT('Ctrl Pts',(-163.070427976155,225.002226664011,13.7084234471774));
#80046=CARTESIAN_POINT('Ctrl Pts',(-163.074880074443,225.002680230006,14.7915765528225));
#80047=CARTESIAN_POINT('Ctrl Pts',(-163.076678969153,225.199312119173,14.781381184332));
#80048=CARTESIAN_POINT('Ctrl Pts',(-162.969917021752,226.414620457773,14.7182665274308));
#80049=CARTESIAN_POINT('Ctrl Pts',(-161.35123317519,228.372148487207,14.602232582119));
#80050=CARTESIAN_POINT('Ctrl Pts',(-157.899898300982,227.964251906854,14.4434747168873));
#80051=CARTESIAN_POINT('Ctrl Pts',(-156.37057641913,224.843472097915,14.2847168516555));
#80052=CARTESIAN_POINT('Ctrl Pts',(-158.162902855767,221.865946618808,14.1259589864237));
#80053=CARTESIAN_POINT('Ctrl Pts',(-161.636540526564,221.756706670925,13.9672011211919));
#80054=CARTESIAN_POINT('Ctrl Pts',(-163.023764549892,223.763970428172,13.8557403099915));
#80055=CARTESIAN_POINT('Ctrl Pts',(-163.078048660107,224.889957182075,13.7971987872017));
#80056=CARTESIAN_POINT('Ctrl Pts',(-163.077285877774,224.998169460932,13.7915765528225));
#80057=CARTESIAN_POINT('Origin',(-160.,225.,22.2084234471774));
#80058=CARTESIAN_POINT('',(-163.068600857884,225.000142042464,15.7915765528225));
#80059=CARTESIAN_POINT('',(-163.078275131255,224.99899685628,15.7084234471774));
#80060=CARTESIAN_POINT('',(-163.0735,225.,22.2084234471774));
#80061=CARTESIAN_POINT('Ctrl Pts',(-163.078275131255,224.99899685628,15.7084234471774));
#80062=CARTESIAN_POINT('Ctrl Pts',(-163.074175496475,225.961517707257,15.6583725623568));
#80063=CARTESIAN_POINT('Ctrl Pts',(-162.07021132955,227.949094729739,15.5554023891257));
#80064=CARTESIAN_POINT('Ctrl Pts',(-158.685830928108,228.386764813856,15.3995129274839));
#80065=CARTESIAN_POINT('Ctrl Pts',(-156.441904596157,225.732921108328,15.2407550622521));
#80066=CARTESIAN_POINT('Ctrl Pts',(-157.454347037885,222.408308033282,15.0819971970203));
#80067=CARTESIAN_POINT('Ctrl Pts',(-160.796570970435,221.455611344259,14.9232393317885));
#80068=CARTESIAN_POINT('Ctrl Pts',(-162.846283064823,223.252698486056,14.7987147485075));
#80069=CARTESIAN_POINT('Ctrl Pts',(-163.072674388859,224.636076809336,14.7271094536372));
#80070=CARTESIAN_POINT('Ctrl Pts',(-163.070312864252,224.997827536139,14.7084234471775));
#80071=CARTESIAN_POINT('Ctrl Pts',(-163.068600857884,225.000142042464,15.7915765528225));
#80072=CARTESIAN_POINT('Ctrl Pts',(-163.068808772742,225.504442530025,15.7655635814622));
#80073=CARTESIAN_POINT('Ctrl Pts',(-162.712640219014,227.034386277039,15.6866313216913));
#80074=CARTESIAN_POINT('Ctrl Pts',(-160.301025069996,228.620303912768,15.5547797735098));
#80075=CARTESIAN_POINT('Ctrl Pts',(-157.121784978706,227.216550203517,15.396021908278));
#80076=CARTESIAN_POINT('Ctrl Pts',(-156.576687161735,223.784209835184,15.2372640430462));
#80077=CARTESIAN_POINT('Ctrl Pts',(-159.164605119719,221.464560577875,15.0785061778144));
#80078=CARTESIAN_POINT('Ctrl Pts',(-162.301782032254,222.321721154701,14.9299436810732));
#80079=CARTESIAN_POINT('Ctrl Pts',(-163.067341765883,224.17868989613,14.8343004727426));
#80080=CARTESIAN_POINT('Ctrl Pts',(-163.074880074443,225.002680230006,14.7915765528225));
#80081=CARTESIAN_POINT('Origin',(-160.,225.,22.2084234471774));
#80082=CARTESIAN_POINT('',(-163.074358790027,224.997245236004,16.7915765528225));
#80083=CARTESIAN_POINT('',(-163.073270276431,225.002809226401,16.7084234471774));
#80084=CARTESIAN_POINT('',(-163.0735,225.,22.2084234471774));
#80085=CARTESIAN_POINT('Ctrl Pts',(-163.073270276431,225.002809226401,16.7084234471774));
#80086=CARTESIAN_POINT('Ctrl Pts',(-163.075543956965,225.252888159811,16.6954742478977));
#80087=CARTESIAN_POINT('Ctrl Pts',(-162.933293767189,226.522407549409,16.6296057602074));
#80088=CARTESIAN_POINT('Ctrl Pts',(-161.1744486001,228.437715336979,16.5108179841064));
#80089=CARTESIAN_POINT('Ctrl Pts',(-157.748926298441,227.851295046903,16.3520601188746));
#80090=CARTESIAN_POINT('Ctrl Pts',(-156.383586559849,224.655369641669,16.1933022536428));
#80091=CARTESIAN_POINT('Ctrl Pts',(-158.327988259509,221.774849926999,16.034544388411));
#80092=CARTESIAN_POINT('Ctrl Pts',(-161.802615038297,221.845987432231,15.8757865231792));
#80093=CARTESIAN_POINT('Ctrl Pts',(-163.052168846365,223.87121946714,15.767079542768));
#80094=CARTESIAN_POINT('Ctrl Pts',(-163.078510080291,224.943835028985,15.7112918507674));
#80095=CARTESIAN_POINT('Ctrl Pts',(-163.078275131255,224.99899685628,15.7084234471774));
#80096=CARTESIAN_POINT('Ctrl Pts',(-163.074358790027,224.997245236004,16.7915765528225));
#80097=CARTESIAN_POINT('Ctrl Pts',(-163.066909982667,225.804358158871,16.7497459785925));
#80098=CARTESIAN_POINT('Ctrl Pts',(-162.327778343425,227.644612117386,16.6549961159518));
#80099=CARTESIAN_POINT('Ctrl Pts',(-159.224254609194,228.54900487538,16.5073269649006));
#80100=CARTESIAN_POINT('Ctrl Pts',(-156.597644432372,226.273260816304,16.3485690996688));
#80101=CARTESIAN_POINT('Ctrl Pts',(-157.084869938397,222.832228509288,16.189811234437));
#80102=CARTESIAN_POINT('Ctrl Pts',(-160.240022361613,221.37514058481,16.0310533692052));
#80103=CARTESIAN_POINT('Ctrl Pts',(-162.694518125763,222.93069425377,15.8983084753337));
#80104=CARTESIAN_POINT('Ctrl Pts',(-163.068385802748,224.478522708056,15.8184828698728));
#80105=CARTESIAN_POINT('Ctrl Pts',(-163.068600857884,225.000142042464,15.7915765528225));
#80106=CARTESIAN_POINT('Origin',(-160.,225.,22.2084234471774));
#80107=CARTESIAN_POINT('',(-163.077658887757,225.001583255091,17.7915765528225));
#80108=CARTESIAN_POINT('',(-163.068753078883,224.999274061734,17.7084234471774));
#80109=CARTESIAN_POINT('',(-163.0735,225.,22.2084234471774));
#80110=CARTESIAN_POINT('Ctrl Pts',(-163.068753078883,224.999274061734,17.7084234471775));
#80111=CARTESIAN_POINT('Ctrl Pts',(-163.067574754586,225.556892657374,17.679656645028));
#80112=CARTESIAN_POINT('Ctrl Pts',(-162.655451307041,227.14192667646,17.5979705544679));
#80113=CARTESIAN_POINT('Ctrl Pts',(-160.112779483536,228.631046257429,17.4633651754972));
#80114=CARTESIAN_POINT('Ctrl Pts',(-157.01065569651,227.064227921279,17.3046073102654));
#80115=CARTESIAN_POINT('Ctrl Pts',(-156.644379692211,223.608228244332,17.1458494450336));
#80116=CARTESIAN_POINT('Ctrl Pts',(-159.349167264668,221.425978037138,16.9870915798018));
#80117=CARTESIAN_POINT('Ctrl Pts',(-162.380395013843,222.425872430781,16.8412829138497));
#80118=CARTESIAN_POINT('Ctrl Pts',(-163.066252142595,224.230894527875,16.7483935363083));
#80119=CARTESIAN_POINT('Ctrl Pts',(-163.073270276431,225.002809226401,16.7084234471774));
#80120=CARTESIAN_POINT('Ctrl Pts',(-163.077658887757,225.001583255091,17.7915765528225));
#80121=CARTESIAN_POINT('Ctrl Pts',(-163.078230100695,225.092572084339,17.7868476641333));
#80122=CARTESIAN_POINT('Ctrl Pts',(-163.033302735283,226.201212096667,17.7291994870335));
#80123=CARTESIAN_POINT('Ctrl Pts',(-161.690920182255,228.21527672754,17.6186320215231));
#80124=CARTESIAN_POINT('Ctrl Pts',(-158.215935725382,228.164542826343,17.4598741562913));
#80125=CARTESIAN_POINT('Ctrl Pts',(-156.373726632524,225.217619277503,17.3011162910595));
#80126=CARTESIAN_POINT('Ctrl Pts',(-157.850282874527,222.071530659953,17.1423584258277));
#80127=CARTESIAN_POINT('Ctrl Pts',(-161.294260101108,221.605577026048,16.9836005605959));
#80128=CARTESIAN_POINT('Ctrl Pts',(-162.958390309227,223.55043056178,16.8666732695942));
#80129=CARTESIAN_POINT('Ctrl Pts',(-163.076333367171,224.783290618411,16.8026652670031));
#80130=CARTESIAN_POINT('Ctrl Pts',(-163.074358790027,224.997245236004,16.7915765528225));
#80131=CARTESIAN_POINT('Origin',(-160.,225.,22.2084234471774));
#80132=CARTESIAN_POINT('',(-163.069604839599,225.001742689702,18.7915765528225));
#80133=CARTESIAN_POINT('',(-163.07593125098,224.997572466666,18.7084234471774));
#80134=CARTESIAN_POINT('',(-163.0735,225.,22.2084234471774));
#80135=CARTESIAN_POINT('Ctrl Pts',(-163.07593125098,224.997572466666,18.7084234471774));
#80136=CARTESIAN_POINT('Ctrl Pts',(-163.068500077913,225.856684342497,18.6638390421582));
#80137=CARTESIAN_POINT('Ctrl Pts',(-162.24610097103,227.747989564111,18.5663353487284));
#80138=CARTESIAN_POINT('Ctrl Pts',(-159.041158462775,228.503973551838,18.4159123668879));
#80139=CARTESIAN_POINT('Ctrl Pts',(-156.536164017499,226.095014589637,18.2571545016561));
#80140=CARTESIAN_POINT('Ctrl Pts',(-157.201271626476,222.683896050202,18.0983966364243));
#80141=CARTESIAN_POINT('Ctrl Pts',(-160.427775574161,221.392476847509,17.9396387711926));
#80142=CARTESIAN_POINT('Ctrl Pts',(-162.749078753838,223.038418143583,17.8096477081103));
#80143=CARTESIAN_POINT('Ctrl Pts',(-163.069742395014,224.531099830892,17.7325759334386));
#80144=CARTESIAN_POINT('Ctrl Pts',(-163.068753078883,224.999274061734,17.7084234471775));
#80145=CARTESIAN_POINT('Ctrl Pts',(-163.069604839599,225.001742689702,18.7915765528225));
#80146=CARTESIAN_POINT('Ctrl Pts',(-163.071667317009,225.399743333181,18.7710300612636));
#80147=CARTESIAN_POINT('Ctrl Pts',(-162.814828130989,226.820276113243,18.697564281294));
#80148=CARTESIAN_POINT('Ctrl Pts',(-160.671798738453,228.570130775029,18.5711792129139));
#80149=CARTESIAN_POINT('Ctrl Pts',(-157.365046168866,227.50084632268,18.4124213476821));
#80150=CARTESIAN_POINT('Ctrl Pts',(-156.469788080311,224.142773253644,18.2536634824503));
#80151=CARTESIAN_POINT('Ctrl Pts',(-158.805387108694,221.569240893567,18.0949056172185));
#80152=CARTESIAN_POINT('Ctrl Pts',(-162.132156176017,222.118667729787,17.9408766406759));
#80153=CARTESIAN_POINT('Ctrl Pts',(-163.071837862639,224.074348900514,17.8397669525439));
#80154=CARTESIAN_POINT('Ctrl Pts',(-163.077658887757,225.001583255091,17.7915765528225));
#80155=CARTESIAN_POINT('Origin',(-160.,225.,22.2084234471774));
#80156=CARTESIAN_POINT('',(-163.070362295124,224.996974657089,19.7915765528225));
#80157=CARTESIAN_POINT('',(-163.076377868511,225.002226294578,19.7084234471774));
#80158=CARTESIAN_POINT('',(-163.0735,225.,22.2084234471774));
#80159=CARTESIAN_POINT('',(-160.793799282533,222.030777046254,20.));
#80160=CARTESIAN_POINT('Ctrl Pts',(-160.793799282533,222.030777046254,20.));
#80161=CARTESIAN_POINT('Ctrl Pts',(-161.781070948697,222.29471665351,19.9470807115894));
#80162=CARTESIAN_POINT('Ctrl Pts',(-162.879413320178,223.336658232169,19.8776062291969));
#80163=CARTESIAN_POINT('Ctrl Pts',(-163.072766807016,224.67677228815,19.8081317468044));
#80164=CARTESIAN_POINT('Ctrl Pts',(-163.070362295124,224.996974657089,19.7915765528225));
#80165=CARTESIAN_POINT('',(-159.204405557221,222.025443011815,20.));
#80166=CARTESIAN_POINT('Origin',(-160.,225.,20.));
#80167=CARTESIAN_POINT('Ctrl Pts',(-159.204403754918,222.025437656558,20.));
#80168=CARTESIAN_POINT('Ctrl Pts',(-160.166034868365,221.76985452113,19.948244384658));
#80169=CARTESIAN_POINT('Ctrl Pts',(-162.230116403007,222.243618617642,19.8510522003838));
#80170=CARTESIAN_POINT('Ctrl Pts',(-163.069182947608,224.12719520771,19.7538600161096));
#80171=CARTESIAN_POINT('Ctrl Pts',(-163.076377868511,225.002226294578,19.7084234471774));
#80172=CARTESIAN_POINT('Origin',(-160.,-225.,22.2084234471774));
#80173=CARTESIAN_POINT('',(-163.078662475314,-224.999834801063,0.791576552822534));
#80174=CARTESIAN_POINT('',(-163.068636046267,-224.999297928038,0.708423447177441));
#80175=CARTESIAN_POINT('',(-163.0735,-225.,22.2084234471774));
#80176=CARTESIAN_POINT('',(-159.206200717467,-227.969222953746,0.));
#80177=CARTESIAN_POINT('Ctrl Pts',(-163.068636046267,-224.999297928038,
0.708423447177441));
#80178=CARTESIAN_POINT('Ctrl Pts',(-163.069474488198,-224.52504187083,0.683959451760682));
#80179=CARTESIAN_POINT('Ctrl Pts',(-162.742950219825,-223.0260819319,0.606576167933325));
#80180=CARTESIAN_POINT('Ctrl Pts',(-160.407275491335,-221.390669642609,
0.47627359569537));
#80181=CARTESIAN_POINT('Ctrl Pts',(-157.18629120154,-222.69900868369,0.317515730463582));
#80182=CARTESIAN_POINT('Ctrl Pts',(-156.545696171353,-226.117971753255,
0.158757865231786));
#80183=CARTESIAN_POINT('Ctrl Pts',(-158.218929051303,-227.70528334649,0.0529192884105924));
#80184=CARTESIAN_POINT('Ctrl Pts',(-159.206200717467,-227.969222953746,
-4.44089209850063E-15));
#80185=CARTESIAN_POINT('',(-160.793799282533,-227.969222953746,0.));
#80186=CARTESIAN_POINT('Origin',(-160.,-225.,0.));
#80187=CARTESIAN_POINT('Ctrl Pts',(-163.078662475314,-224.999834801063,
0.791576552822534));
#80188=CARTESIAN_POINT('Ctrl Pts',(-163.078668424108,-224.991643764631,
0.791150470866062));
#80189=CARTESIAN_POINT('Ctrl Pts',(-163.074932284103,-223.966133613979,
0.737805100498994));
#80190=CARTESIAN_POINT('Ctrl Pts',(-161.945876991572,-221.932389200875,
0.631540441721325));
#80191=CARTESIAN_POINT('Ctrl Pts',(-158.478135184779,-221.701106251642,
0.472782576489533));
#80192=CARTESIAN_POINT('Ctrl Pts',(-156.403376046572,-224.489749930199,
0.314024711257741));
#80193=CARTESIAN_POINT('Ctrl Pts',(-157.610972032634,-227.719907066083,
0.156430519094562));
#80194=CARTESIAN_POINT('Ctrl Pts',(-159.833965217804,-228.230145500202,
0.0517556153419857));
#80195=CARTESIAN_POINT('Ctrl Pts',(-160.795596249024,-227.974562448592,
5.26163314307215E-15));
#80196=CARTESIAN_POINT('Origin',(-160.,-225.,22.2084234471774));
#80197=CARTESIAN_POINT('',(-163.071455505625,-224.997418107078,1.79157655282252));
#80198=CARTESIAN_POINT('',(-163.073451306714,-225.002809475945,1.70842344717744));
#80199=CARTESIAN_POINT('',(-163.0735,-225.,22.2084234471774));
#80200=CARTESIAN_POINT('Ctrl Pts',(-163.073451306714,-225.002809475945,
1.70842344717744));
#80201=CARTESIAN_POINT('Ctrl Pts',(-163.066339691424,-224.224995087548,
1.66814184889093));
#80202=CARTESIAN_POINT('Ctrl Pts',(-162.371724618713,-222.414034792748,
1.57494096219383));
#80203=CARTESIAN_POINT('Ctrl Pts',(-159.328201249173,-221.429869162289,
1.42882078708612));
#80204=CARTESIAN_POINT('Ctrl Pts',(-156.636247355474,-223.627938915385,
1.27006292185434));
#80205=CARTESIAN_POINT('Ctrl Pts',(-157.022865023245,-227.081779873964,
1.11130505662254));
#80206=CARTESIAN_POINT('Ctrl Pts',(-160.134021061057,-228.63024949042,0.952547191390747));
#80207=CARTESIAN_POINT('Ctrl Pts',(-162.662242062284,-227.129893626905,
0.818253321575716));
#80208=CARTESIAN_POINT('Ctrl Pts',(-163.067660812648,-225.550928797488,
0.73687874017128));
#80209=CARTESIAN_POINT('Ctrl Pts',(-163.068636046267,-224.999297928038,
0.708423447177441));
#80210=CARTESIAN_POINT('Ctrl Pts',(-163.071455505625,-224.997418107078,
1.79157655282252));
#80211=CARTESIAN_POINT('Ctrl Pts',(-163.073957160591,-224.683244104354,
1.77533286799631));
#80212=CARTESIAN_POINT('Ctrl Pts',(-162.885142341109,-223.348477340461,
1.70616989475949));
#80213=CARTESIAN_POINT('Ctrl Pts',(-160.958841571036,-221.496026324134,
1.58408763311208));
#80214=CARTESIAN_POINT('Ctrl Pts',(-157.576314230351,-222.293899143107,
1.42532976788029));
#80215=CARTESIAN_POINT('Ctrl Pts',(-156.411946167088,-225.568405119559,
1.2665719026485));
#80216=CARTESIAN_POINT('Ctrl Pts',(-158.531360356103,-228.322686501262,
1.1078140374167));
#80217=CARTESIAN_POINT('Ctrl Pts',(-161.985587207006,-228.036856539208,
0.949482254141382));
#80218=CARTESIAN_POINT('Ctrl Pts',(-163.077929585162,-226.008968748127,
0.844069759276661));
#80219=CARTESIAN_POINT('Ctrl Pts',(-163.078662475314,-224.999834801063,
0.791576552822534));
#80220=CARTESIAN_POINT('Origin',(-160.,-225.,22.2084234471774));
#80221=CARTESIAN_POINT('',(-163.069508383124,-225.001668073485,2.79157655282253));
#80222=CARTESIAN_POINT('',(-163.078189061057,-224.998894481712,2.70842344717744));
#80223=CARTESIAN_POINT('',(-163.0735,-225.,22.2084234471774));
#80224=CARTESIAN_POINT('Ctrl Pts',(-163.078189061057,-224.998894481711,
2.70842344717744));
#80225=CARTESIAN_POINT('Ctrl Pts',(-163.078472645446,-224.937737510531,
2.70524353443178));
#80226=CARTESIAN_POINT('Ctrl Pts',(-163.049103085114,-223.859099596781,
2.64914433327553));
#80227=CARTESIAN_POINT('Ctrl Pts',(-161.784064304926,-221.835457119938,
2.54012584370867));
#80228=CARTESIAN_POINT('Ctrl Pts',(-158.309079789007,-221.784723217824,
2.38136797847688));
#80229=CARTESIAN_POINT('Ctrl Pts',(-156.381624989618,-224.676610132315,
2.22261011324509));
#80230=CARTESIAN_POINT('Ctrl Pts',(-157.765707675159,-227.864464204611,
2.0638522480133));
#80231=CARTESIAN_POINT('Ctrl Pts',(-161.194612911753,-228.430759164971,
1.90509438278151));
#80232=CARTESIAN_POINT('Ctrl Pts',(-162.937600940753,-226.510208572312,
1.78661811583622));
#80233=CARTESIAN_POINT('Ctrl Pts',(-163.075682459254,-225.246835970244,
1.72106113730153));
#80234=CARTESIAN_POINT('Ctrl Pts',(-163.073451306714,-225.002809475945,
1.70842344717744));
#80235=CARTESIAN_POINT('Ctrl Pts',(-163.069508383124,-225.001668073485,
2.79157655282253));
#80236=CARTESIAN_POINT('Ctrl Pts',(-163.066447265951,-224.380571024344,
2.75951526512656));
#80237=CARTESIAN_POINT('Ctrl Pts',(-162.581779704143,-222.729919533307,
2.67453468902));
#80238=CARTESIAN_POINT('Ctrl Pts',(-159.887220512494,-221.368953614723,
2.53663482450283));
#80239=CARTESIAN_POINT('Ctrl Pts',(-156.888312385766,-223.125268673492,
2.37787695927104));
#80240=CARTESIAN_POINT('Ctrl Pts',(-156.737220668234,-226.597337890817,
2.21911909403925));
#80241=CARTESIAN_POINT('Ctrl Pts',(-159.572224410776,-228.60752327959,2.06036122880746));
#80242=CARTESIAN_POINT('Ctrl Pts',(-162.468601111221,-227.448238632615,
1.91784704840188));
#80243=CARTESIAN_POINT('Ctrl Pts',(-163.065807174792,-225.706772006991,
1.8282521564069));
#80244=CARTESIAN_POINT('Ctrl Pts',(-163.071455505625,-224.997418107078,
1.79157655282252));
#80245=CARTESIAN_POINT('Origin',(-160.,-225.,22.2084234471774));
#80246=CARTESIAN_POINT('',(-163.077533915727,-225.001672030798,3.79157655282253));
#80247=CARTESIAN_POINT('',(-163.070184184725,-224.997892517132,3.70842344717744));
#80248=CARTESIAN_POINT('',(-163.0735,-225.,22.2084234471774));
#80249=CARTESIAN_POINT('Ctrl Pts',(-163.070184184725,-224.997892517132,
3.70842344717744));
#80250=CARTESIAN_POINT('Ctrl Pts',(-163.072507054139,-224.630072375909,
3.68942593156203));
#80251=CARTESIAN_POINT('Ctrl Pts',(-162.841128154736,-223.240481211263,
3.61750912753603));
#80252=CARTESIAN_POINT('Ctrl Pts',(-160.77574540398,-221.450995064354,3.49267303509943));
#80253=CARTESIAN_POINT('Ctrl Pts',(-157.439173021718,-222.423300146398,
3.33391516986764));
#80254=CARTESIAN_POINT('Ctrl Pts',(-156.446269384341,-225.753800828521,
3.17515730463584));
#80255=CARTESIAN_POINT('Ctrl Pts',(-158.705739876912,-228.394423031591,
3.01639943940405));
#80256=CARTESIAN_POINT('Ctrl Pts',(-162.080734455212,-227.937802419816,
2.86082148691792));
#80257=CARTESIAN_POINT('Ctrl Pts',(-163.073753307137,-225.95549606401,2.75816282284238));
#80258=CARTESIAN_POINT('Ctrl Pts',(-163.078189061057,-224.998894481711,
2.70842344717744));
#80259=CARTESIAN_POINT('Ctrl Pts',(-163.077533915727,-225.001672030798,
3.79157655282253));
#80260=CARTESIAN_POINT('Ctrl Pts',(-163.071489070002,-224.080332771393,
3.74369766225681));
#80261=CARTESIAN_POINT('Ctrl Pts',(-162.142316990654,-222.130086615022,
3.6428994832805));
#80262=CARTESIAN_POINT('Ctrl Pts',(-158.825551358552,-221.562284541991,
3.48918201589359));
#80263=CARTESIAN_POINT('Ctrl Pts',(-156.474884286599,-224.122061282515,
3.3304241506618));
#80264=CARTESIAN_POINT('Ctrl Pts',(-157.350402977267,-227.485327504289,
3.17166628543));
#80265=CARTESIAN_POINT('Ctrl Pts',(-160.650832758246,-228.574022088692,
3.01290842019821));
#80266=CARTESIAN_POINT('Ctrl Pts',(-162.80938622554,-226.832479130116,2.88621184266238));
#80267=CARTESIAN_POINT('Ctrl Pts',(-163.071499843504,-225.405733026137,
2.81243455353716));
#80268=CARTESIAN_POINT('Ctrl Pts',(-163.069508383124,-225.001668073485,
2.79157655282253));
#80269=CARTESIAN_POINT('Origin',(-160.,-225.,22.2084234471774));
#80270=CARTESIAN_POINT('',(-163.07454124432,-224.997267665337,4.79157655282253));
#80271=CARTESIAN_POINT('',(-163.070564475416,-225.002286520632,4.70842344717744));
#80272=CARTESIAN_POINT('',(-163.0735,-225.,22.2084234471774));
#80273=CARTESIAN_POINT('Ctrl Pts',(-163.070564475416,-225.002286520632,
4.70842344717744));
#80274=CARTESIAN_POINT('Ctrl Pts',(-163.065908934927,-224.328423958447,
4.67360832869229));
#80275=CARTESIAN_POINT('Ctrl Pts',(-162.515666079354,-222.623370785243,
4.58587392179653));
#80276=CARTESIAN_POINT('Ctrl Pts',(-159.698974924892,-221.379696025755,
4.44522022649019));
#80277=CARTESIAN_POINT('Ctrl Pts',(-156.795232916545,-223.289244347558,
4.28646236125839));
#80278=CARTESIAN_POINT('Ctrl Pts',(-156.82449361689,-226.764476175145,4.1277044960266));
#80279=CARTESIAN_POINT('Ctrl Pts',(-159.759977634311,-228.624859476745,
3.96894663079481));
#80280=CARTESIAN_POINT('Ctrl Pts',(-162.537573645734,-227.342131714516,
3.82918628117842));
#80281=CARTESIAN_POINT('Ctrl Pts',(-163.066036492463,-225.654668461557,
3.74234521997263));
#80282=CARTESIAN_POINT('Ctrl Pts',(-163.070184184725,-224.997892517132,
3.70842344717744));
#80283=CARTESIAN_POINT('Ctrl Pts',(-163.07454124432,-224.997267665337,4.79157655282253));
#80284=CARTESIAN_POINT('Ctrl Pts',(-163.076456563004,-224.789355252538,
4.78079934779766));
#80285=CARTESIAN_POINT('Ctrl Pts',(-162.962447976256,-223.562619237962,
4.71710285436219));
#80286=CARTESIAN_POINT('Ctrl Pts',(-161.314169118159,-221.613235066909,
4.60048707251614));
#80287=CARTESIAN_POINT('Ctrl Pts',(-157.867515181948,-222.058958401537,
4.44172920728434));
#80288=CARTESIAN_POINT('Ctrl Pts',(-156.372511267358,-225.196322891415,
4.28297134205255));
#80289=CARTESIAN_POINT('Ctrl Pts',(-158.197384898239,-228.15401267881,4.12421347682076));
#80290=CARTESIAN_POINT('Ctrl Pts',(-161.672011799357,-228.225150186546,
3.96545561158896));
#80291=CARTESIAN_POINT('Ctrl Pts',(-163.030012387691,-226.213350120791,
3.85457663692289));
#80292=CARTESIAN_POINT('Ctrl Pts',(-163.07817028025,-225.098665013773,3.79661695066741));
#80293=CARTESIAN_POINT('Ctrl Pts',(-163.077533915727,-225.001672030798,
3.79157655282253));
#80294=CARTESIAN_POINT('Origin',(-160.,-225.,22.2084234471774));
#80295=CARTESIAN_POINT('',(-163.068595526891,-225.000042998318,5.79157655282253));
#80296=CARTESIAN_POINT('',(-163.078415697005,-225.000807312998,5.70842344717744));
#80297=CARTESIAN_POINT('',(-163.0735,-225.,22.2084234471774));
#80298=CARTESIAN_POINT('Ctrl Pts',(-163.078415697005,-225.000807312998,
5.70842344717744));
#80299=CARTESIAN_POINT('Ctrl Pts',(-163.074998399108,-224.027215799998,
5.65779072582254));
#80300=CARTESIAN_POINT('Ctrl Pts',(-162.05039264629,-222.029873166014,5.55423871605704));
#80301=CARTESIAN_POINT('Ctrl Pts',(-158.648766801864,-221.627851455529,
5.39776741788094));
#80302=CARTESIAN_POINT('Ctrl Pts',(-156.434080438846,-224.306145083543,
5.23900955264915));
#80303=CARTESIAN_POINT('Ctrl Pts',(-157.482923517968,-227.619454703812,
5.08025168741736));
#80304=CARTESIAN_POINT('Ctrl Pts',(-160.835394894467,-228.535439482161,
4.92149382218556));
#80305=CARTESIAN_POINT('Ctrl Pts',(-162.855790325244,-226.724482242959,
4.79755107543892));
#80306=CARTESIAN_POINT('Ctrl Pts',(-163.072985397698,-225.352701020511,
4.72652761710288));
#80307=CARTESIAN_POINT('Ctrl Pts',(-163.070564475416,-225.002286520632,
4.70842344717744));
#80308=CARTESIAN_POINT('Ctrl Pts',(-163.068595526891,-225.000042998318,
5.79157655282253));
#80309=CARTESIAN_POINT('Ctrl Pts',(-163.068531186586,-224.484460456527,
5.76498174492791));
#80310=CARTESIAN_POINT('Ctrl Pts',(-162.700883871275,-222.942867342694,
5.6854676486227));
#80311=CARTESIAN_POINT('Ctrl Pts',(-160.261302591299,-221.376612339411,
5.55303426390689));
#80312=CARTESIAN_POINT('Ctrl Pts',(-157.097648786153,-222.815148834678,
5.3942763986751));
#80313=CARTESIAN_POINT('Ctrl Pts',(-156.590226697787,-226.253261030531,
5.2355185334433));
#80314=CARTESIAN_POINT('Ctrl Pts',(-159.203429001521,-228.544388780525,
5.07676066821151));
#80315=CARTESIAN_POINT('Ctrl Pts',(-162.318767701676,-227.656365438967,
4.92878000800459));
#80316=CARTESIAN_POINT('Ctrl Pts',(-163.067051777479,-225.810267159815,
4.83371863620826));
#80317=CARTESIAN_POINT('Ctrl Pts',(-163.07454124432,-224.997267665337,4.79157655282253));
#80318=CARTESIAN_POINT('Origin',(-160.,-225.,22.2084234471774));
#80319=CARTESIAN_POINT('',(-163.074699050512,-225.002709777195,6.79157655282254));
#80320=CARTESIAN_POINT('',(-163.072935020445,-224.997201474642,6.70842344717745));
#80321=CARTESIAN_POINT('',(-163.0735,-225.,22.2084234471774));
#80322=CARTESIAN_POINT('Ctrl Pts',(-163.072935020445,-224.997201474642,
6.70842344717745));
#80323=CARTESIAN_POINT('Ctrl Pts',(-163.075279695241,-224.735813217208,
6.69489241136339));
#80324=CARTESIAN_POINT('Ctrl Pts',(-162.925138377367,-223.454800480637,
6.62844208713874));
#80325=CARTESIAN_POINT('Ctrl Pts',(-161.136676091388,-221.549610974834,
6.50907247450348));
#80326=CARTESIAN_POINT('Ctrl Pts',(-157.71779106562,-222.173564198225,6.3503146092717));
#80327=CARTESIAN_POINT('Ctrl Pts',(-156.387583566852,-225.384271356254,
6.1915567440399));
#80328=CARTESIAN_POINT('Ctrl Pts',(-158.363459445645,-228.24329338415,6.03279887880811));
#80329=CARTESIAN_POINT('Ctrl Pts',(-161.837097175429,-228.134053434412,
5.87404101357632));
#80330=CARTESIAN_POINT('Ctrl Pts',(-163.057796111155,-226.106151535993,
5.76591586969943));
#80331=CARTESIAN_POINT('Ctrl Pts',(-163.07857002173,-225.044774578035,5.71071001423314));
#80332=CARTESIAN_POINT('Ctrl Pts',(-163.078415697005,-225.000807312998,
5.70842344717744));
#80333=CARTESIAN_POINT('Ctrl Pts',(-163.074699050512,-225.002709777195,
6.79157655282254));
#80334=CARTESIAN_POINT('Ctrl Pts',(-163.067182398241,-224.18460320538,6.74916414205817));
#80335=CARTESIAN_POINT('Ctrl Pts',(-162.310901226859,-222.333446897755,
6.65383244288321));
#80336=CARTESIAN_POINT('Ctrl Pts',(-159.185378807054,-221.459716184381,
6.50558145529764));
#80337=CARTESIAN_POINT('Ctrl Pts',(-156.583884936547,-223.764129838381,
6.34682359006585));
#80338=CARTESIAN_POINT('Ctrl Pts',(-157.108819437776,-227.199611815696,
6.18806572483406));
#80339=CARTESIAN_POINT('Ctrl Pts',(-160.27976227586,-228.622009145783,6.02930785960227));
#80340=CARTESIAN_POINT('Ctrl Pts',(-162.706367588713,-227.04656594312,5.89714480226509));
#80341=CARTESIAN_POINT('Ctrl Pts',(-163.068659213197,-225.510384815019,
5.81790103333851));
#80342=CARTESIAN_POINT('Ctrl Pts',(-163.068595526891,-225.000042998318,
5.79157655282253));
#80343=CARTESIAN_POINT('Origin',(-160.,-225.,22.2084234471774));
#80344=CARTESIAN_POINT('',(-163.077420974813,-224.998253101066,7.79157655282253));
#80345=CARTESIAN_POINT('',(-163.068842428738,-225.000903279819,7.70842344717744));
#80346=CARTESIAN_POINT('',(-163.0735,-225.,22.2084234471774));
#80347=CARTESIAN_POINT('Ctrl Pts',(-163.068842428738,-225.000903279819,
7.70842344717744));
#80348=CARTESIAN_POINT('Ctrl Pts',(-163.067344096249,-224.432047607476,
7.67907480849364));
#80349=CARTESIAN_POINT('Ctrl Pts',(-162.64286158187,-222.835395249423,7.59680688139924));
#80350=CARTESIAN_POINT('Ctrl Pts',(-160.072950512026,-221.36793513487,7.46161966589424));
#80351=CARTESIAN_POINT('Ctrl Pts',(-156.988196718452,-222.968680735341,
7.30286180066245));
#80352=CARTESIAN_POINT('Ctrl Pts',(-156.659845169714,-226.428489646948,
7.14410393543065));
#80353=CARTESIAN_POINT('Ctrl Pts',(-159.388403190305,-228.580944889843,
6.98534607019887));
#80354=CARTESIAN_POINT('Ctrl Pts',(-162.396431378753,-227.551989106954,
6.84011924078113));
#80355=CARTESIAN_POINT('Ctrl Pts',(-163.06610977481,-225.75809124325,6.74781169977399));
#80356=CARTESIAN_POINT('Ctrl Pts',(-163.072935020445,-224.997201474642,
6.70842344717745));
#80357=CARTESIAN_POINT('Ctrl Pts',(-163.077420974813,-224.998253101066,
7.79157655282253));
#80358=CARTESIAN_POINT('Ctrl Pts',(-163.07811538035,-224.896048295815,7.78626582759902));
#80359=CARTESIAN_POINT('Ctrl Pts',(-163.027126200076,-223.776114030172,
7.7280358139649));
#80360=CARTESIAN_POINT('Ctrl Pts',(-161.655556246542,-221.766371898677,
7.61688651192019));
#80361=CARTESIAN_POINT('Ctrl Pts',(-158.181336937272,-221.855213545024,
7.4581286466884));
#80362=CARTESIAN_POINT('Ctrl Pts',(-156.371557991493,-224.822163631299,
7.29937078145661));
#80363=CARTESIAN_POINT('Ctrl Pts',(-157.882529029215,-227.951869555216,
7.14061291622481));
#80364=CARTESIAN_POINT('Ctrl Pts',(-161.331409416131,-228.380024578279,
6.98185505099302));
#80365=CARTESIAN_POINT('Ctrl Pts',(-162.965935927934,-226.426805145778,
6.8655095965256));
#80366=CARTESIAN_POINT('Ctrl Pts',(-163.076561159841,-225.205380304447,
6.80208343046877));
#80367=CARTESIAN_POINT('Ctrl Pts',(-163.074699050512,-225.002709777195,
6.79157655282254));
#80368=CARTESIAN_POINT('Origin',(-160.,-225.,22.2084234471774));
#80369=CARTESIAN_POINT('',(-163.069424322521,-224.99840233946,8.79157655282254));
#80370=CARTESIAN_POINT('',(-163.076244526858,-225.00231956595,8.70842344717745));
#80371=CARTESIAN_POINT('',(-163.0735,-225.,22.2084234471774));
#80372=CARTESIAN_POINT('Ctrl Pts',(-163.076244526858,-225.00231956595,8.70842344717745));
#80373=CARTESIAN_POINT('Ctrl Pts',(-163.068938542211,-224.132225888735,
8.66325720562389));
#80374=CARTESIAN_POINT('Ctrl Pts',(-162.228255889997,-222.230332832212,
8.56517167565975));
#80375=CARTESIAN_POINT('Ctrl Pts',(-159.002787802732,-221.506751541139,
8.41416685728499));
#80376=CARTESIAN_POINT('Ctrl Pts',(-156.524362933047,-223.943040237029,
8.25540899205321));
#80377=CARTESIAN_POINT('Ctrl Pts',(-157.226840970362,-227.346658466427,
8.09665112682141));
#80378=CARTESIAN_POINT('Ctrl Pts',(-160.46731404255,-228.602614959631,7.93789326158962));
#80379=CARTESIAN_POINT('Ctrl Pts',(-162.760117776494,-226.938795070132,
7.80848403504163));
#80380=CARTESIAN_POINT('Ctrl Pts',(-163.070045778257,-225.457765962356,
7.73199409690424));
#80381=CARTESIAN_POINT('Ctrl Pts',(-163.068842428738,-225.000903279819,
7.70842344717744));
#80382=CARTESIAN_POINT('Ctrl Pts',(-163.069424322521,-224.99840233946,8.79157655282254));
#80383=CARTESIAN_POINT('Ctrl Pts',(-163.071353288451,-224.58907249002,8.77044822472927));
#80384=CARTESIAN_POINT('Ctrl Pts',(-162.804636795139,-223.156921697034,
8.6964006082254));
#80385=CARTESIAN_POINT('Ctrl Pts',(-160.632612776171,-221.422707971306,
8.56943370331094));
#80386=CARTESIAN_POINT('Ctrl Pts',(-157.337773316573,-222.528205860274,
8.41067583807916));
#80387=CARTESIAN_POINT('Ctrl Pts',(-156.479403612958,-225.895889648718,
8.25191797284736));
#80388=CARTESIAN_POINT('Ctrl Pts',(-158.84308358432,-228.443655265885,8.09316010761556));
#80389=CARTESIAN_POINT('Ctrl Pts',(-162.151085208535,-227.859988133188,
7.93971296760729));
#80390=CARTESIAN_POINT('Ctrl Pts',(-163.07119590225,-225.914478988118,7.83918511600961));
#80391=CARTESIAN_POINT('Ctrl Pts',(-163.077420974813,-224.998253101066,
7.79157655282253));
#80392=CARTESIAN_POINT('Origin',(-160.,-225.,22.2084234471774));
#80393=CARTESIAN_POINT('',(-163.071594709852,-225.002615145319,9.79157655282253));
#80394=CARTESIAN_POINT('',(-163.076078262664,-224.997622030919,9.70842344717745));
#80395=CARTESIAN_POINT('',(-163.0735,-225.,22.2084234471774));
#80396=CARTESIAN_POINT('Ctrl Pts',(-163.076078262664,-224.997622030919,
9.70842344717745));
#80397=CARTESIAN_POINT('Ctrl Pts',(-163.077404917311,-224.84224257729,9.70035889116474));
#80398=CARTESIAN_POINT('Ctrl Pts',(-162.996066991238,-223.668662623908,
9.63937504674145));
#80399=CARTESIAN_POINT('Ctrl Pts',(-161.48554891982,-221.684828606461,9.52547191390754));
#80400=CARTESIAN_POINT('Ctrl Pts',(-158.020618779932,-221.953811078189,
9.36671404867575));
#80401=CARTESIAN_POINT('Ctrl Pts',(-156.367218254814,-225.010665531371,
9.20795618344397));
#80402=CARTESIAN_POINT('Ctrl Pts',(-158.038539440034,-228.057758890661,
9.04919831821217));
#80403=CARTESIAN_POINT('Ctrl Pts',(-161.504989252603,-228.306391433462,
8.89044045298037));
#80404=CARTESIAN_POINT('Ctrl Pts',(-162.999733528855,-226.319171864349,
8.77684882930213));
#80405=CARTESIAN_POINT('Ctrl Pts',(-163.077498641421,-225.151676183136,
8.71617649403449));
#80406=CARTESIAN_POINT('Ctrl Pts',(-163.076244526858,-225.00231956595,8.70842344717745));
#80407=CARTESIAN_POINT('Ctrl Pts',(-163.071594709852,-225.002615145319,
9.79157655282253));
#80408=CARTESIAN_POINT('Ctrl Pts',(-163.065812239552,-224.288114655817,
9.75463062185952));
#80409=CARTESIAN_POINT('Ctrl Pts',(-162.461599049811,-222.541385538678,
9.66476540248591));
#80410=CARTESIAN_POINT('Ctrl Pts',(-159.553847756031,-221.394703152536,
9.5219808947017));
#80411=CARTESIAN_POINT('Ctrl Pts',(-156.729123730022,-223.419308502703,
9.3632230294699));
#80412=CARTESIAN_POINT('Ctrl Pts',(-156.897905537673,-226.890562649037,
9.20446516423812));
#80413=CARTESIAN_POINT('Ctrl Pts',(-159.905724075259,-228.631573933316,
9.04570729900632));
#80414=CARTESIAN_POINT('Ctrl Pts',(-162.588044922784,-227.259590262751,
8.9080777618678));
#80415=CARTESIAN_POINT('Ctrl Pts',(-163.066521883717,-225.614304787718,
8.82336751313987));
#80416=CARTESIAN_POINT('Ctrl Pts',(-163.069424322521,-224.99840233946,8.79157655282254));
#80417=CARTESIAN_POINT('Origin',(-160.,-225.,22.2084234471774));
#80418=CARTESIAN_POINT('',(-163.078673958092,-225.000055941931,10.7915765528225));
#80419=CARTESIAN_POINT('',(-163.068792204425,-224.999191249543,10.7084234471774));
#80420=CARTESIAN_POINT('',(-163.0735,-225.,22.2084234471774));
#80421=CARTESIAN_POINT('Ctrl Pts',(-163.068792204425,-224.999191249543,
10.7084234471774));
#80422=CARTESIAN_POINT('Ctrl Pts',(-163.069882850319,-224.536271765866,
10.684541288295));
#80423=CARTESIAN_POINT('Ctrl Pts',(-162.754228600442,-223.049004170933,
10.6077398410019));
#80424=CARTESIAN_POINT('Ctrl Pts',(-160.446152240227,-221.39470318278,10.4780191052983));
#80425=CARTESIAN_POINT('Ctrl Pts',(-157.213109725203,-222.669665354942,
10.3192612400665));
#80426=CARTESIAN_POINT('Ctrl Pts',(-156.530629080082,-226.077349702623,
10.1605033748347));
#80427=CARTESIAN_POINT('Ctrl Pts',(-159.02331656444,-228.499043644829,10.0017455096029));
#80428=CARTESIAN_POINT('Ctrl Pts',(-162.237835374063,-227.758067329382,
9.85105220038383));
#80429=CARTESIAN_POINT('Ctrl Pts',(-163.068699463494,-225.861836229654,
9.75327817957534));
#80430=CARTESIAN_POINT('Ctrl Pts',(-163.076078262664,-224.997622030919,
9.70842344717745));
#80431=CARTESIAN_POINT('Ctrl Pts',(-163.078673464311,-225.000055936592,
10.7915765528225));
#80432=CARTESIAN_POINT('Ctrl Pts',(-163.078401402235,-223.985720010178,
10.7388130189898));
#80433=CARTESIAN_POINT('Ctrl Pts',(-161.975981854003,-221.953547158614,
10.6331301967464));
#80434=CARTESIAN_POINT('Ctrl Pts',(-158.514451067719,-221.684828578651,
10.4745280860924));
#80435=CARTESIAN_POINT('Ctrl Pts',(-156.409095223172,-224.449890859119,
10.3157702208607));
#80436=CARTESIAN_POINT('Ctrl Pts',(-157.590135289169,-227.718413003688,
10.1570123556289));
#80437=CARTESIAN_POINT('Ctrl Pts',(-160.976683443753,-228.499043674182,
9.99825449039708));
#80438=CARTESIAN_POINT('Ctrl Pts',(-162.889275844143,-226.640923288454,
9.87644255612829));
#80439=CARTESIAN_POINT('Ctrl Pts',(-163.074094727111,-225.311525258498,
9.80754991027011));
#80440=CARTESIAN_POINT('Ctrl Pts',(-163.071594709852,-225.002615145319,
9.79157655282253));
#80441=CARTESIAN_POINT('Origin',(-160.,-225.,22.2084234471774));
#80442=CARTESIAN_POINT('',(-163.071757725923,-224.997349454093,11.7915765528225));
#80443=CARTESIAN_POINT('',(-163.073114044306,-225.00280587903,11.7084234471775));
#80444=CARTESIAN_POINT('',(-163.0735,-225.,22.2084234471774));
#80445=CARTESIAN_POINT('Ctrl Pts',(-163.073114044306,-225.00280587903,11.7084234471775));
#80446=CARTESIAN_POINT('Ctrl Pts',(-163.06618243262,-224.236012324399,11.6687236854253));
#80447=CARTESIAN_POINT('Ctrl Pts',(-162.3878703787,-222.436152749216,11.5761046352624));
#80448=CARTESIAN_POINT('Ctrl Pts',(-159.367387229136,-221.422708001315,
11.4305662966891));
#80449=CARTESIAN_POINT('Ctrl Pts',(-156.651514980196,-223.591147618143,
11.2718084314573));
#80450=CARTESIAN_POINT('Ctrl Pts',(-157.000176089704,-227.048968879445,
11.1130505662255));
#80451=CARTESIAN_POINT('Ctrl Pts',(-160.09427592395,-228.631573902853,10.9542927009937));
#80452=CARTESIAN_POINT('Ctrl Pts',(-162.649624257918,-227.152465296695,
10.8194169946443));
#80453=CARTESIAN_POINT('Ctrl Pts',(-163.067466142311,-225.56203203269,10.7374605767056));
#80454=CARTESIAN_POINT('Ctrl Pts',(-163.068792204425,-224.999191249543,
10.7084234471774));
#80455=CARTESIAN_POINT('Ctrl Pts',(-163.071757725923,-224.997349454093,
11.7915765528225));
#80456=CARTESIAN_POINT('Ctrl Pts',(-163.07425181278,-224.694504312659,11.7759147045306));
#80457=CARTESIAN_POINT('Ctrl Pts',(-162.893998089999,-223.371289777703,
11.7073335678281));
#80458=CARTESIAN_POINT('Ctrl Pts',(-160.997212205634,-221.506751511835,
11.585833142715));
#80459=CARTESIAN_POINT('Ctrl Pts',(-157.606138743777,-222.267483674507,
11.4270752774832));
#80460=CARTESIAN_POINT('Ctrl Pts',(-156.405927009479,-225.529014670817,
11.2683174122514));
#80461=CARTESIAN_POINT('Ctrl Pts',(-158.495010734773,-228.306391461198,
11.1095595470196));
#80462=CARTESIAN_POINT('Ctrl Pts',(-161.96146057642,-228.057758916311,10.9508016817878));
#80463=CARTESIAN_POINT('Ctrl Pts',(-163.07731441338,-226.023373876136,10.8448073503888));
#80464=CARTESIAN_POINT('Ctrl Pts',(-163.078674267421,-225.003050191384,
10.7917323074004));
#80465=CARTESIAN_POINT('Ctrl Pts',(-163.078673464311,-225.000055936592,
10.7915765528225));
#80466=CARTESIAN_POINT('Origin',(-160.,-225.,22.2084234471774));
#80467=CARTESIAN_POINT('',(-163.069332144507,-225.001514698785,12.7915765528225));
#80468=CARTESIAN_POINT('',(-163.07834387793,-224.99908713945,12.7084234471775));
#80469=CARTESIAN_POINT('',(-163.0735,-225.,22.2084234471774));
#80470=CARTESIAN_POINT('Ctrl Pts',(-163.07834387793,-224.99908713945,12.7084234471775));
#80471=CARTESIAN_POINT('Ctrl Pts',(-163.078539635575,-224.949126906597,
12.7058253709661));
#80472=CARTESIAN_POINT('Ctrl Pts',(-163.054799409449,-223.881734486773,
12.6503080063442));
#80473=CARTESIAN_POINT('Ctrl Pts',(-161.818663047472,-221.855213571405,
12.5418713533116));
#80474=CARTESIAN_POINT('Ctrl Pts',(-158.344443767345,-221.766371925803,
12.3831134880798));
#80475=CARTESIAN_POINT('Ctrl Pts',(-156.385389486241,-224.636946566547,
12.224355622848));
#80476=CARTESIAN_POINT('Ctrl Pts',(-157.734426605188,-227.839787695311,
12.0655977576162));
#80477=CARTESIAN_POINT('Ctrl Pts',(-161.156916405975,-228.443655236998,
11.9068398923844));
#80478=CARTESIAN_POINT('Ctrl Pts',(-162.92952308503,-226.532996262698,11.7877817889048));
#80479=CARTESIAN_POINT('Ctrl Pts',(-163.075422184743,-225.258138591106,
11.7216429738358));
#80480=CARTESIAN_POINT('Ctrl Pts',(-163.073114044306,-225.00280587903,11.7084234471775));
#80481=CARTESIAN_POINT('Ctrl Pts',(-163.069332144507,-225.001514698785,
12.7915765528225));
#80482=CARTESIAN_POINT('Ctrl Pts',(-163.066612219994,-224.391601434172,
12.7600971016609));
#80483=CARTESIAN_POINT('Ctrl Pts',(-162.595215317641,-222.752504181858,
12.6756983620886));
#80484=CARTESIAN_POINT('Ctrl Pts',(-159.927049487362,-221.367935104402,
12.5383803341058));
#80485=CARTESIAN_POINT('Ctrl Pts',(-156.909059974209,-223.091255140127,
12.379622468874));
#80486=CARTESIAN_POINT('Ctrl Pts',(-156.719898651112,-226.561458396548,
12.2208646036422));
#80487=CARTESIAN_POINT('Ctrl Pts',(-159.53268595353,-228.602614989851,12.0621067384104));
#80488=CARTESIAN_POINT('Ctrl Pts',(-162.453478525563,-227.470561640101,
11.9190107214705));
#80489=CARTESIAN_POINT('Ctrl Pts',(-163.065824627226,-225.717777497571,
11.8288339929412));
#80490=CARTESIAN_POINT('Ctrl Pts',(-163.071757725923,-224.997349454093,
11.7915765528225));
#80491=CARTESIAN_POINT('Origin',(-160.,-225.,22.2084234471774));
#80492=CARTESIAN_POINT('',(-163.077285955845,-225.001830539115,13.7915765528225));
#80493=CARTESIAN_POINT('',(-163.070428058496,-224.997773335929,13.7084234471775));
#80494=CARTESIAN_POINT('',(-163.0735,-225.,22.2084234471774));
#80495=CARTESIAN_POINT('Ctrl Pts',(-163.070428058496,-224.997773335929,
13.7084234471775));
#80496=CARTESIAN_POINT('Ctrl Pts',(-163.072819246321,-224.641289592038,
13.6900077680964));
#80497=CARTESIAN_POINT('Ctrl Pts',(-162.850719882267,-223.26330056594,13.6186728006047));
#80498=CARTESIAN_POINT('Ctrl Pts',(-160.814621186112,-221.459716214079,
13.4944185447024));
#80499=CARTESIAN_POINT('Ctrl Pts',(-157.467586059932,-222.395370161066,
13.3356606794706));
#80500=CARTESIAN_POINT('Ctrl Pts',(-156.438216072117,-225.714781234221,
13.1769028142388));
#80501=CARTESIAN_POINT('Ctrl Pts',(-158.668590595037,-228.380024549925,
13.018144949007));
#80502=CARTESIAN_POINT('Ctrl Pts',(-162.061029944568,-227.958876297453,
12.8619851599865));
#80503=CARTESIAN_POINT('Ctrl Pts',(-163.074552317882,-225.966749084061,
12.7587446593767));
#80504=CARTESIAN_POINT('Ctrl Pts',(-163.07834387793,-224.99908713945,12.7084234471775));
#80505=CARTESIAN_POINT('Ctrl Pts',(-163.077285955845,-225.001830539115,
13.7915765528225));
#80506=CARTESIAN_POINT('Ctrl Pts',(-163.070869048314,-224.091494579315,
13.7442794987911));
#80507=CARTESIAN_POINT('Ctrl Pts',(-162.161132916986,-222.151467560355,
13.6440631563491));
#80508=CARTESIAN_POINT('Ctrl Pts',(-158.863323899077,-221.54961094589,13.4909275254965));
#80509=CARTESIAN_POINT('Ctrl Pts',(-156.484724767496,-224.083453643903,
13.3321696602647));
#80510=CARTESIAN_POINT('Ctrl Pts',(-157.323305390468,-227.456119530974,
13.1734117950329));
#80511=CARTESIAN_POINT('Ctrl Pts',(-160.611596814825,-228.580944919882,
13.0146539298011));
#80512=CARTESIAN_POINT('Ctrl Pts',(-162.799120185496,-226.855291254971,
12.887375515731));
#80513=CARTESIAN_POINT('Ctrl Pts',(-163.071184614508,-225.416910795182,
12.8130163900715));
#80514=CARTESIAN_POINT('Ctrl Pts',(-163.069332144507,-225.001514698785,
12.7915765528225));
#80515=CARTESIAN_POINT('Origin',(-160.,-225.,22.2084234471774));
#80516=CARTESIAN_POINT('',(-163.074880152452,-224.997319769926,14.7915765528225));
#80517=CARTESIAN_POINT('',(-163.070312946591,-225.002172463919,14.7084234471775));
#80518=CARTESIAN_POINT('',(-163.0735,-225.,22.2084234471774));
#80519=CARTESIAN_POINT('Ctrl Pts',(-163.070312946591,-225.002172463919,
14.7084234471775));
#80520=CARTESIAN_POINT('Ctrl Pts',(-163.065986567915,-224.339435084193,
14.6741901652266));
#80521=CARTESIAN_POINT('Ctrl Pts',(-162.529985040226,-222.645831244846,
14.5870375948652));
#80522=CARTESIAN_POINT('Ctrl Pts',(-159.738697410893,-221.376612369806,
14.4469657360931));
#80523=CARTESIAN_POINT('Ctrl Pts',(-156.814187751561,-223.254200103273,
14.2882078708613));
#80524=CARTESIAN_POINT('Ctrl Pts',(-156.805333336721,-226.729543833573,
14.1294500056295));
#80525=CARTESIAN_POINT('Ctrl Pts',(-159.720237726487,-228.622009115399,
13.9706921403977));
#80526=CARTESIAN_POINT('Ctrl Pts',(-162.523355831361,-227.364607796017,
13.830349954247));
#80527=CARTESIAN_POINT('Ctrl Pts',(-163.065947929897,-225.665681143041,
13.7429270565069));
#80528=CARTESIAN_POINT('Ctrl Pts',(-163.070428058496,-224.997773335929,
13.7084234471775));
#80529=CARTESIAN_POINT('Ctrl Pts',(-163.074880152452,-224.997319769926,
14.7915765528225));
#80530=CARTESIAN_POINT('Ctrl Pts',(-163.076679047208,-224.80068787577,14.781381184332));
#80531=CARTESIAN_POINT('Ctrl Pts',(-162.969917097099,-223.585379506338,
14.7182665274308));
#80532=CARTESIAN_POINT('Ctrl Pts',(-161.351233209471,-221.627851427242,
14.6022325821191));
#80533=CARTESIAN_POINT('Ctrl Pts',(-157.899898247702,-222.035748017944,
14.4434747168873));
#80534=CARTESIAN_POINT('Ctrl Pts',(-156.370576327052,-225.156527906056,
14.2847168516555));
#80535=CARTESIAN_POINT('Ctrl Pts',(-158.16290280916,-228.134053460702,14.1259589864237));
#80536=CARTESIAN_POINT('Ctrl Pts',(-161.636540568083,-228.243293411356,
13.9672011211919));
#80537=CARTESIAN_POINT('Ctrl Pts',(-163.023764626605,-226.236029603186,
13.8557403099915));
#80538=CARTESIAN_POINT('Ctrl Pts',(-163.078048738197,-225.110042820717,
13.7971987872017));
#80539=CARTESIAN_POINT('Ctrl Pts',(-163.077285955845,-225.001830539115,
13.7915765528225));
#80540=CARTESIAN_POINT('Origin',(-160.,-225.,22.2084234471774));
#80541=CARTESIAN_POINT('',(-163.068600935734,-224.999857957532,15.7915765528225));
#80542=CARTESIAN_POINT('',(-163.078275213807,-225.001003143747,15.7084234471775));
#80543=CARTESIAN_POINT('',(-163.0735,-225.,22.2084234471774));
#80544=CARTESIAN_POINT('Ctrl Pts',(-163.078275213807,-225.001003143747,
15.7084234471775));
#80545=CARTESIAN_POINT('Ctrl Pts',(-163.074175578918,-224.038482266957,
15.6583725623569));
#80546=CARTESIAN_POINT('Ctrl Pts',(-162.070211385068,-222.050905191173,
15.5554023891257));
#80547=CARTESIAN_POINT('Ctrl Pts',(-158.685830892865,-221.613235095319,
15.3995129274839));
#80548=CARTESIAN_POINT('Ctrl Pts',(-156.441904500737,-224.267078872017,
15.2407550622521));
#80549=CARTESIAN_POINT('Ctrl Pts',(-157.454346969616,-227.591692036222,
15.0819971970203));
#80550=CARTESIAN_POINT('Ctrl Pts',(-160.796570991797,-228.544388750793,
14.9232393317885));
#80551=CARTESIAN_POINT('Ctrl Pts',(-162.846283141153,-226.747301560803,
14.7987147485075));
#80552=CARTESIAN_POINT('Ctrl Pts',(-163.072674471261,-225.363923200424,
14.7271094536372));
#80553=CARTESIAN_POINT('Ctrl Pts',(-163.070312946591,-225.002172463919,
14.7084234471775));
#80554=CARTESIAN_POINT('Ctrl Pts',(-163.068600935734,-224.999857957532,
15.7915765528225));
#80555=CARTESIAN_POINT('Ctrl Pts',(-163.068808850597,-224.495557457177,
15.7655635814622));
#80556=CARTESIAN_POINT('Ctrl Pts',(-162.712640287833,-222.965613671348,
15.6866313216913));
#80557=CARTESIAN_POINT('Ctrl Pts',(-160.301025077633,-221.379695995386,
15.5547797735098));
#80558=CARTESIAN_POINT('Ctrl Pts',(-157.121784905686,-222.78344974025,15.396021908278));
#80559=CARTESIAN_POINT('Ctrl Pts',(-156.576687074886,-226.21579019566,15.2372640430462));
#80560=CARTESIAN_POINT('Ctrl Pts',(-159.164605098526,-228.535439511819,
15.0785061778144));
#80561=CARTESIAN_POINT('Ctrl Pts',(-162.30178209065,-227.678278913247,14.9299436810732));
#80562=CARTESIAN_POINT('Ctrl Pts',(-163.067341843701,-225.821310124706,
14.8343004727426));
#80563=CARTESIAN_POINT('Ctrl Pts',(-163.074880152452,-224.997319769926,
14.7915765528225));
#80564=CARTESIAN_POINT('Origin',(-160.,-225.,22.2084234471774));
#80565=CARTESIAN_POINT('',(-163.074358868023,-225.002754764066,16.7915765528225));
#80566=CARTESIAN_POINT('',(-163.073270358849,-224.997190773524,16.7084234471775));
#80567=CARTESIAN_POINT('',(-163.0735,-225.,22.2084234471774));
#80568=CARTESIAN_POINT('Ctrl Pts',(-163.073270358849,-224.997190773524,
16.7084234471774));
#80569=CARTESIAN_POINT('Ctrl Pts',(-163.075544039444,-224.747111833407,
16.6954742478977));
#80570=CARTESIAN_POINT('Ctrl Pts',(-162.933293845853,-223.477592409764,
16.6296057602074));
#80571=CARTESIAN_POINT('Ctrl Pts',(-161.174448631596,-221.562284570829,
16.5108179841064));
#80572=CARTESIAN_POINT('Ctrl Pts',(-157.748926238073,-222.148704876632,
16.3520601188746));
#80573=CARTESIAN_POINT('Ctrl Pts',(-156.383586462865,-225.344630367573,
16.1933022536428));
#80574=CARTESIAN_POINT('Ctrl Pts',(-158.327988214669,-228.225150159492,
16.034544388411));
#80575=CARTESIAN_POINT('Ctrl Pts',(-161.80261508664,-228.154012652352,15.8757865231792));
#80576=CARTESIAN_POINT('Ctrl Pts',(-163.052168928217,-226.128780563132,
15.767079542768));
#80577=CARTESIAN_POINT('Ctrl Pts',(-163.078510162849,-225.056164972521,
15.7112918507675));
#80578=CARTESIAN_POINT('Ctrl Pts',(-163.078275213807,-225.001003143747,
15.7084234471775));
#80579=CARTESIAN_POINT('Ctrl Pts',(-163.074358868023,-225.002754764066,
16.7915765528225));
#80580=CARTESIAN_POINT('Ctrl Pts',(-163.066910060473,-224.195641820723,
16.7497459785925));
#80581=CARTESIAN_POINT('Ctrl Pts',(-162.327778402481,-222.35538781552,16.6549961159518));
#80582=CARTESIAN_POINT('Ctrl Pts',(-159.224254589513,-221.450995034583,
16.5073269649006));
#80583=CARTESIAN_POINT('Ctrl Pts',(-156.597644346055,-223.726739151393,
16.3485690996688));
#80584=CARTESIAN_POINT('Ctrl Pts',(-157.08486986444,-227.167771545708,16.189811234437));
#80585=CARTESIAN_POINT('Ctrl Pts',(-160.240022367702,-228.624859507152,
16.0310533692052));
#80586=CARTESIAN_POINT('Ctrl Pts',(-162.694518194122,-227.069305798728,
15.8983084753337));
#80587=CARTESIAN_POINT('Ctrl Pts',(-163.068385880592,-225.521477305173,
15.8184828698728));
#80588=CARTESIAN_POINT('Ctrl Pts',(-163.068600935734,-224.999857957532,
15.7915765528225));
#80589=CARTESIAN_POINT('Origin',(-160.,-225.,22.2084234471774));
#80590=CARTESIAN_POINT('',(-163.077658965824,-224.998416744887,17.7915765528225));
#80591=CARTESIAN_POINT('',(-163.06875316118,-225.000725938278,17.7084234471775));
#80592=CARTESIAN_POINT('',(-163.0735,-225.,22.2084234471774));
#80593=CARTESIAN_POINT('Ctrl Pts',(-163.06875316118,-225.000725938278,17.7084234471775));
#80594=CARTESIAN_POINT('Ctrl Pts',(-163.067574836851,-224.443107327688,
17.679656645028));
#80595=CARTESIAN_POINT('Ctrl Pts',(-162.655451378254,-222.858073266113,
17.5979705544679));
#80596=CARTESIAN_POINT('Ctrl Pts',(-160.11277948656,-221.368953645186,17.4633651754972));
#80597=CARTESIAN_POINT('Ctrl Pts',(-157.010655616342,-222.935772023368,
17.3046073102654));
#80598=CARTESIAN_POINT('Ctrl Pts',(-156.644379602221,-226.39177179299,17.1458494450336));
#80599=CARTESIAN_POINT('Ctrl Pts',(-159.349167247214,-228.574022058711,
16.9870915798018));
#80600=CARTESIAN_POINT('Ctrl Pts',(-162.38039507768,-227.574127638251,16.8412829138497));
#80601=CARTESIAN_POINT('Ctrl Pts',(-163.066252224825,-225.76910549275,16.7483935363083));
#80602=CARTESIAN_POINT('Ctrl Pts',(-163.073270358849,-224.997190773524,
16.7084234471774));
#80603=CARTESIAN_POINT('Ctrl Pts',(-163.077658965824,-224.998416744887,
17.7915765528225));
#80604=CARTESIAN_POINT('Ctrl Pts',(-163.078230178775,-224.907427913335,
17.7868476641333));
#80605=CARTESIAN_POINT('Ctrl Pts',(-163.033302812201,-223.798787872917,
17.7291994870335));
#80606=CARTESIAN_POINT('Ctrl Pts',(-161.690920225189,-221.784723190834,
17.6186320215231));
#80607=CARTESIAN_POINT('Ctrl Pts',(-158.215935680102,-221.835457093401,
17.4598741562913));
#80608=CARTESIAN_POINT('Ctrl Pts',(-156.373726540536,-224.782380716962,
17.3011162910595));
#80609=CARTESIAN_POINT('Ctrl Pts',(-157.850282819984,-227.928469414349,
17.1423584258277));
#80610=CARTESIAN_POINT('Ctrl Pts',(-161.294260133946,-228.394423060065,
16.9836005605959));
#80611=CARTESIAN_POINT('Ctrl Pts',(-162.95839038428,-226.449569474996,16.8666732695942));
#80612=CARTESIAN_POINT('Ctrl Pts',(-163.076333445217,-225.216709387087,
16.8026652670031));
#80613=CARTESIAN_POINT('Ctrl Pts',(-163.074358868023,-225.002754764066,
16.7915765528225));
#80614=CARTESIAN_POINT('Origin',(-160.,-225.,22.2084234471774));
#80615=CARTESIAN_POINT('',(-163.069604917803,-224.99825730896,18.7915765528225));
#80616=CARTESIAN_POINT('',(-163.075931333395,-225.0024275328,18.7084234471774));
#80617=CARTESIAN_POINT('',(-163.0735,-225.,22.2084234471774));
#80618=CARTESIAN_POINT('Ctrl Pts',(-163.075931333395,-225.0024275328,18.7084234471774));
#80619=CARTESIAN_POINT('Ctrl Pts',(-163.068500160107,-224.143315633891,
18.6638390421582));
#80620=CARTESIAN_POINT('Ctrl Pts',(-162.246101031359,-222.252010363093,
18.5663353487284));
#80621=CARTESIAN_POINT('Ctrl Pts',(-159.04115843702,-221.496026353686,18.4159123668879));
#80622=CARTESIAN_POINT('Ctrl Pts',(-156.536163924622,-223.90498538126,18.2571545016561));
#80623=CARTESIAN_POINT('Ctrl Pts',(-157.201271551415,-227.316104011775,
18.0983966364243));
#80624=CARTESIAN_POINT('Ctrl Pts',(-160.427775585634,-228.607523249306,
17.9396387711926));
#80625=CARTESIAN_POINT('Ctrl Pts',(-162.749078827562,-226.961581909006,
17.8096477081103));
#80626=CARTESIAN_POINT('Ctrl Pts',(-163.069742477337,-225.468900181672,
17.7325759334386));
#80627=CARTESIAN_POINT('Ctrl Pts',(-163.06875316118,-225.000725938278,17.7084234471775));
#80628=CARTESIAN_POINT('Ctrl Pts',(-163.069604917803,-224.99825730896,18.7915765528225));
#80629=CARTESIAN_POINT('Ctrl Pts',(-163.071667394827,-224.600256656493,
18.7710300612636));
#80630=CARTESIAN_POINT('Ctrl Pts',(-162.8148282007,-223.179723844664,18.697564281294));
#80631=CARTESIAN_POINT('Ctrl Pts',(-160.671798756939,-221.429869131324,
18.5711792129139));
#80632=CARTESIAN_POINT('Ctrl Pts',(-157.365046101209,-222.499153615461,
18.4124213476821));
#80633=CARTESIAN_POINT('Ctrl Pts',(-156.469787991194,-225.857226767288,
18.2536634824503));
#80634=CARTESIAN_POINT('Ctrl Pts',(-158.805387078146,-228.430759193889,
18.0949056172185));
#80635=CARTESIAN_POINT('Ctrl Pts',(-162.132156230227,-227.881332343118,
17.9408766406759));
#80636=CARTESIAN_POINT('Ctrl Pts',(-163.071837940579,-225.925651122953,
17.8397669525439));
#80637=CARTESIAN_POINT('Ctrl Pts',(-163.077658965824,-224.998416744887,
17.7915765528225));
#80638=CARTESIAN_POINT('Origin',(-160.,-225.,22.2084234471774));
#80639=CARTESIAN_POINT('',(-163.070362267144,-225.003024949566,19.7915765528225));
#80640=CARTESIAN_POINT('',(-163.076377950168,-224.997773694264,19.7084234471775));
#80641=CARTESIAN_POINT('',(-163.0735,-225.,22.2084234471774));
#80642=CARTESIAN_POINT('',(-160.793799282533,-227.969222953746,20.));
#80643=CARTESIAN_POINT('Ctrl Pts',(-160.793799282533,-227.969222953746,
20.));
#80644=CARTESIAN_POINT('Ctrl Pts',(-161.781070948697,-227.70528334649,19.9470807115894));
#80645=CARTESIAN_POINT('Ctrl Pts',(-162.879413246734,-226.663341238238,
19.8776062291969));
#80646=CARTESIAN_POINT('Ctrl Pts',(-163.072766768174,-225.323227278198,
19.8081317468044));
#80647=CARTESIAN_POINT('Ctrl Pts',(-163.070362267144,-225.003024949566,
19.7915765528225));
#80648=CARTESIAN_POINT('',(-159.204405553981,-227.97455706887,20.));
#80649=CARTESIAN_POINT('Origin',(-160.,-225.,20.));
#80650=CARTESIAN_POINT('Ctrl Pts',(-159.204403751904,-227.974562423527,
20.));
#80651=CARTESIAN_POINT('Ctrl Pts',(-160.166034802714,-228.230145495107,
19.948244384658));
#80652=CARTESIAN_POINT('Ctrl Pts',(-162.230116536165,-227.756381568108,
19.8510522003838));
#80653=CARTESIAN_POINT('Ctrl Pts',(-163.069183044459,-225.872804827253,
19.7538600161097));
#80654=CARTESIAN_POINT('Ctrl Pts',(-163.076377950168,-224.997773694264,
19.7084234471775));
#80655=CARTESIAN_POINT('Origin',(160.,-225.,22.2084234471774));
#80656=CARTESIAN_POINT('',(156.921337778595,-224.999834790454,0.791576552822529));
#80657=CARTESIAN_POINT('',(156.931363877713,-224.999297943428,0.708423447177436));
#80658=CARTESIAN_POINT('',(156.9265,-225.,22.2084234471774));
#80659=CARTESIAN_POINT('',(160.793799282533,-227.969222953746,0.));
#80660=CARTESIAN_POINT('Ctrl Pts',(156.931363877713,-224.999297943428,0.708423447177436));
#80661=CARTESIAN_POINT('Ctrl Pts',(156.93052543409,-224.525041881822,0.683959451760682));
#80662=CARTESIAN_POINT('Ctrl Pts',(157.257049705227,-223.026081918318,0.606576167933329));
#80663=CARTESIAN_POINT('Ctrl Pts',(159.592724500381,-221.390669414731,0.476273595695376));
#80664=CARTESIAN_POINT('Ctrl Pts',(162.813708891355,-222.699008838373,0.317515730463588));
#80665=CARTESIAN_POINT('Ctrl Pts',(163.454303720846,-226.117970975858,0.158757865231792));
#80666=CARTESIAN_POINT('Ctrl Pts',(161.781070948697,-227.70528334649,0.0529192884105984));
#80667=CARTESIAN_POINT('Ctrl Pts',(160.793799282533,-227.969222953746,0.));
#80668=CARTESIAN_POINT('',(159.206200717467,-227.969222953746,0.));
#80669=CARTESIAN_POINT('Origin',(160.,-225.,0.));
#80670=CARTESIAN_POINT('Ctrl Pts',(156.921337778595,-224.999834790454,0.791576552822529));
#80671=CARTESIAN_POINT('Ctrl Pts',(156.921331829825,-224.991643754766,0.791150470866057));
#80672=CARTESIAN_POINT('Ctrl Pts',(156.925067972487,-223.966133697564,0.737805100498987));
#80673=CARTESIAN_POINT('Ctrl Pts',(158.054123192547,-221.932389526572,0.631540441721319));
#80674=CARTESIAN_POINT('Ctrl Pts',(161.52186463808,-221.701106398635,0.472782576489526));
#80675=CARTESIAN_POINT('Ctrl Pts',(163.596623766652,-224.489750196051,0.314024711257736));
#80676=CARTESIAN_POINT('Ctrl Pts',(162.389027506789,-227.719906449348,0.156430519094557));
#80677=CARTESIAN_POINT('Ctrl Pts',(160.16603498601,-228.230145450022,0.0517556153419843));
#80678=CARTESIAN_POINT('Ctrl Pts',(159.204403760484,-227.974562200359,5.38238616003273E-15));
#80679=CARTESIAN_POINT('Origin',(160.,-225.,22.2084234471774));
#80680=CARTESIAN_POINT('',(156.92854474983,-224.997418107049,1.79157655282252));
#80681=CARTESIAN_POINT('',(156.926548618152,-225.002809476022,1.70842344717743));
#80682=CARTESIAN_POINT('',(156.9265,-225.,22.2084234471774));
#80683=CARTESIAN_POINT('Ctrl Pts',(156.926548618152,-225.002809476022,1.70842344717743));
#80684=CARTESIAN_POINT('Ctrl Pts',(156.933660233471,-224.224995068889,1.66814184889093));
#80685=CARTESIAN_POINT('Ctrl Pts',(157.628275322693,-222.414034730693,1.57494096219383));
#80686=CARTESIAN_POINT('Ctrl Pts',(160.671798768642,-221.429869072041,1.42882078708613));
#80687=CARTESIAN_POINT('Ctrl Pts',(163.363752724354,-223.627938887541,1.27006292185434));
#80688=CARTESIAN_POINT('Ctrl Pts',(162.977135053578,-227.081779913939,1.11130505662255));
#80689=CARTESIAN_POINT('Ctrl Pts',(159.865978929321,-228.630249599949,0.952547191390754));
#80690=CARTESIAN_POINT('Ctrl Pts',(157.337757879225,-227.129893648995,0.818253321575718));
#80691=CARTESIAN_POINT('Ctrl Pts',(156.932339113301,-225.550928817993,0.736878740171278));
#80692=CARTESIAN_POINT('Ctrl Pts',(156.931363877713,-224.999297943428,0.708423447177436));
#80693=CARTESIAN_POINT('Ctrl Pts',(156.92854474983,-224.997418107049,1.79157655282252));
#80694=CARTESIAN_POINT('Ctrl Pts',(156.926043095071,-224.683244130428,1.7753328679963));
#80695=CARTESIAN_POINT('Ctrl Pts',(157.114857898856,-223.348477477565,1.70616989475949));
#80696=CARTESIAN_POINT('Ctrl Pts',(159.041158508843,-221.496026617155,1.58408763311207));
#80697=CARTESIAN_POINT('Ctrl Pts',(162.423685567743,-222.293899365156,1.42532976788028));
#80698=CARTESIAN_POINT('Ctrl Pts',(163.588053535237,-225.568405078077,1.26657190264849));
#80699=CARTESIAN_POINT('Ctrl Pts',(161.468639519931,-228.322686213904,1.1078140374167));
#80700=CARTESIAN_POINT('Ctrl Pts',(158.01441296236,-228.036856307199,0.949482254141376));
#80701=CARTESIAN_POINT('Ctrl Pts',(156.922070665826,-226.008968645781,0.844069759276654));
#80702=CARTESIAN_POINT('Ctrl Pts',(156.921337778595,-224.999834790454,0.791576552822529));
#80703=CARTESIAN_POINT('Origin',(160.,-225.,22.2084234471774));
#80704=CARTESIAN_POINT('',(156.930491872184,-225.001668073344,2.79157655282252));
#80705=CARTESIAN_POINT('',(156.921810863685,-224.99889448168,2.70842344717744));
#80706=CARTESIAN_POINT('',(156.9265,-225.,22.2084234471774));
#80707=CARTESIAN_POINT('Ctrl Pts',(156.921810863685,-224.998894481681,2.70842344717744));
#80708=CARTESIAN_POINT('Ctrl Pts',(156.92152727929,-224.937737509005,2.70524353443178));
#80709=CARTESIAN_POINT('Ctrl Pts',(156.950896840338,-223.859099568886,2.64914433327553));
#80710=CARTESIAN_POINT('Ctrl Pts',(158.215935651436,-221.835457042593,2.54012584370868));
#80711=CARTESIAN_POINT('Ctrl Pts',(161.69092025237,-221.784723139159,2.38136797847689));
#80712=CARTESIAN_POINT('Ctrl Pts',(163.618375098784,-224.676610124513,2.22261011324509));
#80713=CARTESIAN_POINT('Ctrl Pts',(162.234292379592,-227.864464274441,2.0638522480133));
#80714=CARTESIAN_POINT('Ctrl Pts',(158.805387058807,-228.430759249254,1.90509438278151));
#80715=CARTESIAN_POINT('Ctrl Pts',(157.062398987685,-226.510208608751,1.78661811583622));
#80716=CARTESIAN_POINT('Ctrl Pts',(156.924317465603,-225.2468359762,1.72106113730153));
#80717=CARTESIAN_POINT('Ctrl Pts',(156.926548618152,-225.002809476022,1.70842344717743));
#80718=CARTESIAN_POINT('Ctrl Pts',(156.930491872184,-225.001668073344,2.79157655282252));
#80719=CARTESIAN_POINT('Ctrl Pts',(156.933552989102,-224.380571075862,2.75951526512656));
#80720=CARTESIAN_POINT('Ctrl Pts',(157.418220510598,-222.729919722113,2.67453468901999));
#80721=CARTESIAN_POINT('Ctrl Pts',(160.112779478126,-221.368953916766,2.53663482450283));
#80722=CARTESIAN_POINT('Ctrl Pts',(163.111687355417,-223.125268829368,2.37787695927104));
#80723=CARTESIAN_POINT('Ctrl Pts',(163.262779060384,-226.597337758068,2.21911909403925));
#80724=CARTESIAN_POINT('Ctrl Pts',(160.427775553637,-228.607522979317,2.06036122880745));
#80725=CARTESIAN_POINT('Ctrl Pts',(157.531399094122,-227.448238429336,1.91784704840188));
#80726=CARTESIAN_POINT('Ctrl Pts',(156.934193080194,-225.706771948024,1.8282521564069));
#80727=CARTESIAN_POINT('Ctrl Pts',(156.92854474983,-224.997418107049,1.79157655282252));
#80728=CARTESIAN_POINT('Origin',(160.,-225.,22.2084234471774));
#80729=CARTESIAN_POINT('',(156.922466340248,-225.001672030659,3.79157655282253));
#80730=CARTESIAN_POINT('',(156.929815740211,-224.99789251708,3.70842344717744));
#80731=CARTESIAN_POINT('',(156.9265,-225.,22.2084234471774));
#80732=CARTESIAN_POINT('Ctrl Pts',(156.929815740211,-224.99789251708,3.70842344717744));
#80733=CARTESIAN_POINT('Ctrl Pts',(156.92749287074,-224.630072366865,3.68942593156203));
#80734=CARTESIAN_POINT('Ctrl Pts',(157.1588717758,-223.240481168243,3.61750912753603));
#80735=CARTESIAN_POINT('Ctrl Pts',(159.224254577053,-221.450994977583,3.49267303509943));
#80736=CARTESIAN_POINT('Ctrl Pts',(162.560827040894,-222.423300083398,3.33391516986764));
#80737=CARTESIAN_POINT('Ctrl Pts',(163.553730702545,-225.753800846953,3.17515730463585));
#80738=CARTESIAN_POINT('Ctrl Pts',(161.294260154735,-228.39442311458,3.01639943940406));
#80739=CARTESIAN_POINT('Ctrl Pts',(157.91926549391,-227.937802491651,2.86082148691792));
#80740=CARTESIAN_POINT('Ctrl Pts',(156.926246617715,-225.955496087366,2.75816282284238));
#80741=CARTESIAN_POINT('Ctrl Pts',(156.921810863685,-224.998894481681,2.70842344717744));
#80742=CARTESIAN_POINT('Ctrl Pts',(156.922466340248,-225.001672030659,3.79157655282253));
#80743=CARTESIAN_POINT('Ctrl Pts',(156.928511185471,-224.080332847886,3.74369766225681));
#80744=CARTESIAN_POINT('Ctrl Pts',(157.857683187534,-222.130086853728,3.6428994832805));
#80745=CARTESIAN_POINT('Ctrl Pts',(161.174448543763,-221.562284827925,3.48918201589358));
#80746=CARTESIAN_POINT('Ctrl Pts',(163.525115420198,-224.122061355537,3.33042415066179));
#80747=CARTESIAN_POINT('Ctrl Pts',(162.649596802351,-227.485327297572,3.17166628543));
#80748=CARTESIAN_POINT('Ctrl Pts',(159.349167295888,-228.574021791418,3.01290842019821));
#80749=CARTESIAN_POINT('Ctrl Pts',(157.190614008131,-226.832478977704,2.88621184266238));
#80750=CARTESIAN_POINT('Ctrl Pts',(156.928500411969,-225.405732992389,2.81243455353715));
#80751=CARTESIAN_POINT('Ctrl Pts',(156.930491872184,-225.001668073344,2.79157655282252));
#80752=CARTESIAN_POINT('Origin',(160.,-225.,22.2084234471774));
#80753=CARTESIAN_POINT('',(156.925459011406,-224.997267665565,4.79157655282252));
#80754=CARTESIAN_POINT('',(156.92943544951,-225.002286520688,4.70842344717744));
#80755=CARTESIAN_POINT('',(156.9265,-225.,22.2084234471774));
#80756=CARTESIAN_POINT('Ctrl Pts',(156.92943544951,-225.002286520688,4.70842344717743));
#80757=CARTESIAN_POINT('Ctrl Pts',(156.934090990113,-224.328423942027,4.67360832869228));
#80758=CARTESIAN_POINT('Ctrl Pts',(157.484333859139,-222.623370727135,4.58587392179654));
#80759=CARTESIAN_POINT('Ctrl Pts',(160.301025082467,-221.37969593724,4.44522022649019));
#80760=CARTESIAN_POINT('Ctrl Pts',(163.20476716181,-223.289244305731,4.2864623612584));
#80761=CARTESIAN_POINT('Ctrl Pts',(163.17550646075,-226.764476218285,4.1277044960266));
#80762=CARTESIAN_POINT('Ctrl Pts',(160.240022371557,-228.624859565371,3.96894663079482));
#80763=CARTESIAN_POINT('Ctrl Pts',(157.462426292223,-227.34213177178,3.82918628117842));
#80764=CARTESIAN_POINT('Ctrl Pts',(156.933963432573,-225.654668477563,3.74234521997263));
#80765=CARTESIAN_POINT('Ctrl Pts',(156.929815740211,-224.99789251708,3.70842344717744));
#80766=CARTESIAN_POINT('Ctrl Pts',(156.925459011406,-224.997267665564,4.79157655282252));
#80767=CARTESIAN_POINT('Ctrl Pts',(156.923543692882,-224.789355270059,4.78079934779766));
#80768=CARTESIAN_POINT('Ctrl Pts',(157.037552270148,-223.562619357517,4.71710285436219));
#80769=CARTESIAN_POINT('Ctrl Pts',(158.685830991148,-221.613235348605,4.60048707251613));
#80770=CARTESIAN_POINT('Ctrl Pts',(162.132484640682,-222.05895864616,4.44172920728435));
#80771=CARTESIAN_POINT('Ctrl Pts',(163.627488430923,-225.196322875086,4.28297134205254));
#80772=CARTESIAN_POINT('Ctrl Pts',(161.802614951828,-228.154012416474,4.12421347682076));
#80773=CARTESIAN_POINT('Ctrl Pts',(158.327988339714,-228.225149918293,3.96545561158896));
#80774=CARTESIAN_POINT('Ctrl Pts',(156.969987864332,-226.21335001987,3.85457663692289));
#80775=CARTESIAN_POINT('Ctrl Pts',(156.921829975778,-225.098665005566,3.79661695066741));
#80776=CARTESIAN_POINT('Ctrl Pts',(156.922466340248,-225.001672030659,3.79157655282253));
#80777=CARTESIAN_POINT('Origin',(160.,-225.,22.2084234471774));
#80778=CARTESIAN_POINT('',(156.931404728341,-225.000042998315,5.79157655282252));
#80779=CARTESIAN_POINT('',(156.921584227729,-225.000807313018,5.70842344717744));
#80780=CARTESIAN_POINT('',(156.9265,-225.,22.2084234471774));
#80781=CARTESIAN_POINT('Ctrl Pts',(156.921584227729,-225.000807313018,5.70842344717744));
#80782=CARTESIAN_POINT('Ctrl Pts',(156.925001525709,-224.027215776214,5.65779072582254));
#80783=CARTESIAN_POINT('Ctrl Pts',(157.949607303578,-222.029873093395,5.55423871605704));
#80784=CARTESIAN_POINT('Ctrl Pts',(161.351233231173,-221.627851373082,5.39776741788094));
#80785=CARTESIAN_POINT('Ctrl Pts',(163.56591964834,-224.306145066578,5.23900955264915));
#80786=CARTESIAN_POINT('Ctrl Pts',(162.517076543573,-227.619454767856,5.08025168741736));
#80787=CARTESIAN_POINT('Ctrl Pts',(159.164605085109,-228.535439568601,4.92149382218557));
#80788=CARTESIAN_POINT('Ctrl Pts',(157.144209604933,-226.724482285122,4.79755107543892));
#80789=CARTESIAN_POINT('Ctrl Pts',(156.927014527169,-225.352701029134,4.72652761710288));
#80790=CARTESIAN_POINT('Ctrl Pts',(156.92943544951,-225.002286520688,4.70842344717743));
#80791=CARTESIAN_POINT('Ctrl Pts',(156.931404728341,-225.000042998315,5.79157655282252));
#80792=CARTESIAN_POINT('Ctrl Pts',(156.93146906864,-224.484460499407,5.76498174492791));
#80793=CARTESIAN_POINT('Ctrl Pts',(157.299116353373,-222.942867513797,5.6854676486227));
#80794=CARTESIAN_POINT('Ctrl Pts',(159.738697430435,-221.376612640788,5.55303426390689));
#80795=CARTESIAN_POINT('Ctrl Pts',(162.902350972443,-222.815149016404,5.39427639867509));
#80796=CARTESIAN_POINT('Ctrl Pts',(163.409773018603,-226.25326092629,5.23551853344331));
#80797=CARTESIAN_POINT('Ctrl Pts',(160.796570932224,-228.544388485719,5.07676066821151));
#80798=CARTESIAN_POINT('Ctrl Pts',(157.681232491188,-227.656365218022,4.92878000800459));
#80799=CARTESIAN_POINT('Ctrl Pts',(156.932948477624,-225.810267092421,4.83371863620826));
#80800=CARTESIAN_POINT('Ctrl Pts',(156.925459011406,-224.997267665564,4.79157655282252));
#80801=CARTESIAN_POINT('Origin',(160.,-225.,22.2084234471774));
#80802=CARTESIAN_POINT('',(156.925301205227,-225.00270977697,6.79157655282253));
#80803=CARTESIAN_POINT('',(156.927064904423,-224.997201474574,6.70842344717744));
#80804=CARTESIAN_POINT('',(156.9265,-225.,22.2084234471774));
#80805=CARTESIAN_POINT('Ctrl Pts',(156.927064904423,-224.997201474574,6.70842344717744));
#80806=CARTESIAN_POINT('Ctrl Pts',(156.92472022957,-224.735813210749,6.69489241136339));
#80807=CARTESIAN_POINT('Ctrl Pts',(157.074861551115,-223.454800442857,6.62844208713874));
#80808=CARTESIAN_POINT('Ctrl Pts',(158.863323880821,-221.549610890473,6.50907247450349));
#80809=CARTESIAN_POINT('Ctrl Pts',(162.282208990179,-222.17356412912,6.3503146092717));
#80810=CARTESIAN_POINT('Ctrl Pts',(163.61241652147,-225.384271365649,6.19155674403991));
#80811=CARTESIAN_POINT('Ctrl Pts',(161.636540594368,-228.243293463447,6.03279887880811));
#80812=CARTESIAN_POINT('Ctrl Pts',(158.162902779655,-228.134053511038,5.87404101357632));
#80813=CARTESIAN_POINT('Ctrl Pts',(156.942203814083,-226.106151563038,5.76591586969943));
#80814=CARTESIAN_POINT('Ctrl Pts',(156.921429903001,-225.04477457913,5.71071001423314));
#80815=CARTESIAN_POINT('Ctrl Pts',(156.921584227729,-225.000807313018,5.70842344717744));
#80816=CARTESIAN_POINT('Ctrl Pts',(156.925301205227,-225.00270977697,6.79157655282253));
#80817=CARTESIAN_POINT('Ctrl Pts',(156.932817856874,-224.184603273201,6.74916414205816));
#80818=CARTESIAN_POINT('Ctrl Pts',(157.689098965352,-222.333447119547,6.6538324428832));
#80819=CARTESIAN_POINT('Ctrl Pts',(160.814621125189,-221.459716478846,6.50558145529765));
#80820=CARTESIAN_POINT('Ctrl Pts',(163.416114779316,-223.764129941176,6.34682359006585));
#80821=CARTESIAN_POINT('Ctrl Pts',(162.891180321749,-227.199611632742,6.18806572483406));
#80822=CARTESIAN_POINT('Ctrl Pts',(159.72023774741,-228.622008844521,6.02930785960227));
#80823=CARTESIAN_POINT('Ctrl Pts',(157.29363263639,-227.046565772896,5.89714480226509));
#80824=CARTESIAN_POINT('Ctrl Pts',(156.93134104204,-225.510384772568,5.81790103333851));
#80825=CARTESIAN_POINT('Ctrl Pts',(156.931404728341,-225.000042998315,5.79157655282252));
#80826=CARTESIAN_POINT('Origin',(160.,-225.,22.2084234471774));
#80827=CARTESIAN_POINT('',(156.922579281153,-224.998253101211,7.79157655282253));
#80828=CARTESIAN_POINT('',(156.93115749623,-225.000903279841,7.70842344717744));
#80829=CARTESIAN_POINT('',(156.9265,-225.,22.2084234471774));
#80830=CARTESIAN_POINT('Ctrl Pts',(156.93115749623,-225.000903279841,7.70842344717744));
#80831=CARTESIAN_POINT('Ctrl Pts',(156.932655828756,-224.43204759359,7.67907480849364));
#80832=CARTESIAN_POINT('Ctrl Pts',(157.357138353513,-222.8353951965,7.59680688139925));
#80833=CARTESIAN_POINT('Ctrl Pts',(159.92704948619,-221.367935046067,7.46161966589424));
#80834=CARTESIAN_POINT('Ctrl Pts',(163.011803355185,-222.968680685676,7.30286180066245));
#80835=CARTESIAN_POINT('Ctrl Pts',(163.340154911951,-226.428489681874,7.14410393543066));
#80836=CARTESIAN_POINT('Ctrl Pts',(160.611596824648,-228.580944977395,6.98534607019887));
#80837=CARTESIAN_POINT('Ctrl Pts',(157.603568562655,-227.551989169349,6.84011924078113));
#80838=CARTESIAN_POINT('Ctrl Pts',(156.933890150225,-225.758091261785,6.74781169977399));
#80839=CARTESIAN_POINT('Ctrl Pts',(156.927064904423,-224.997201474574,6.70842344717744));
#80840=CARTESIAN_POINT('Ctrl Pts',(156.922579281153,-224.998253101211,7.79157655282253));
#80841=CARTESIAN_POINT('Ctrl Pts',(156.921884875674,-224.896048304461,7.78626582759901));
#80842=CARTESIAN_POINT('Ctrl Pts',(156.972874051707,-223.776114131969,7.7280358139649));
#80843=CARTESIAN_POINT('Ctrl Pts',(158.344443891159,-221.766372167636,7.6168865119202));
#80844=CARTESIAN_POINT('Ctrl Pts',(161.81866291146,-221.855213806593,7.45812864668839));
#80845=CARTESIAN_POINT('Ctrl Pts',(163.628441706709,-224.822163646091,7.29937078145661));
#80846=CARTESIAN_POINT('Ctrl Pts',(162.117470794664,-227.951869309693,7.14061291622481));
#80847=CARTESIAN_POINT('Ctrl Pts',(158.668590694609,-228.380024297143,6.98185505099302));
#80848=CARTESIAN_POINT('Ctrl Pts',(157.03406431876,-226.426805027102,6.86550959652559));
#80849=CARTESIAN_POINT('Ctrl Pts',(156.923439096054,-225.205380287364,6.80208343046876));
#80850=CARTESIAN_POINT('Ctrl Pts',(156.925301205227,-225.00270977697,6.79157655282253));
#80851=CARTESIAN_POINT('Origin',(160.,-225.,22.2084234471774));
#80852=CARTESIAN_POINT('',(156.93057593278,-224.998402339592,8.79157655282253));
#80853=CARTESIAN_POINT('',(156.923755397929,-225.002319566006,8.70842344717744));
#80854=CARTESIAN_POINT('',(156.9265,-225.,22.2084234471774));
#80855=CARTESIAN_POINT('Ctrl Pts',(156.923755397929,-225.002319566006,8.70842344717744));
#80856=CARTESIAN_POINT('Ctrl Pts',(156.931061382755,-224.132225867519,8.66325720562389));
#80857=CARTESIAN_POINT('Ctrl Pts',(157.771744055523,-222.230332764495,8.56517167565975));
#80858=CARTESIAN_POINT('Ctrl Pts',(160.99721222165,-221.50675145573,8.41416685728499));
#80859=CARTESIAN_POINT('Ctrl Pts',(163.475637151931,-223.943040211187,8.25540899205321));
#80860=CARTESIAN_POINT('Ctrl Pts',(162.773159097441,-227.346658523802,8.09665112682141));
#80861=CARTESIAN_POINT('Ctrl Pts',(159.532685946025,-228.602615047713,7.93789326158963));
#80862=CARTESIAN_POINT('Ctrl Pts',(157.239882156022,-226.938795117535,7.80848403504162));
#80863=CARTESIAN_POINT('Ctrl Pts',(156.929954146681,-225.457765973548,7.73199409690423));
#80864=CARTESIAN_POINT('Ctrl Pts',(156.93115749623,-225.000903279841,7.70842344717744));
#80865=CARTESIAN_POINT('Ctrl Pts',(156.93057593278,-224.998402339592,8.79157655282253));
#80866=CARTESIAN_POINT('Ctrl Pts',(156.92864696701,-224.589072524199,8.77044822472927));
#80867=CARTESIAN_POINT('Ctrl Pts',(157.195363438138,-223.156921850333,8.69640060822541));
#80868=CARTESIAN_POINT('Ctrl Pts',(159.367387276447,-221.422708268849,8.56943370331094));
#80869=CARTESIAN_POINT('Ctrl Pts',(162.662226461995,-222.528206065867,8.41067583807915));
#80870=CARTESIAN_POINT('Ctrl Pts',(163.520596094214,-225.895889574202,8.25191797284736));
#80871=CARTESIAN_POINT('Ctrl Pts',(161.156916319453,-228.443654979458,8.09316010761556));
#80872=CARTESIAN_POINT('Ctrl Pts',(157.848914970382,-227.859987895307,7.93971296760729));
#80873=CARTESIAN_POINT('Ctrl Pts',(156.928804353199,-225.914478912056,7.83918511600961));
#80874=CARTESIAN_POINT('Ctrl Pts',(156.922579281153,-224.998253101211,7.79157655282253));
#80875=CARTESIAN_POINT('Origin',(160.,-225.,22.2084234471774));
#80876=CARTESIAN_POINT('',(156.928405545629,-225.002615145101,9.79157655282253));
#80877=CARTESIAN_POINT('',(156.923921662128,-224.997622030861,9.70842344717744));
#80878=CARTESIAN_POINT('',(156.9265,-225.,22.2084234471774));
#80879=CARTESIAN_POINT('Ctrl Pts',(156.923921662128,-224.997622030861,9.70842344717744));
#80880=CARTESIAN_POINT('Ctrl Pts',(156.922595007447,-224.842242573433,9.70035889116474));
#80881=CARTESIAN_POINT('Ctrl Pts',(157.003932935509,-223.668662591357,9.63937504674144));
#80882=CARTESIAN_POINT('Ctrl Pts',(158.514451043859,-221.684828525406,9.52547191390756));
#80883=CARTESIAN_POINT('Ctrl Pts',(161.979381268463,-221.953811003712,9.36671404867575));
#80884=CARTESIAN_POINT('Ctrl Pts',(163.632781834006,-225.010665531631,9.20795618344396));
#80885=CARTESIAN_POINT('Ctrl Pts',(161.961460607923,-228.057758965422,9.04919831821217));
#80886=CARTESIAN_POINT('Ctrl Pts',(158.495010710601,-228.306391514302,8.89044045298037));
#80887=CARTESIAN_POINT('Ctrl Pts',(157.000266397803,-226.319171896602,8.77684882930213));
#80888=CARTESIAN_POINT('Ctrl Pts',(156.922501283335,-225.151676186844,8.71617649403449));
#80889=CARTESIAN_POINT('Ctrl Pts',(156.923755397929,-225.002319566006,8.70842344717744));
#80890=CARTESIAN_POINT('Ctrl Pts',(156.928405545629,-225.002615145101,9.79157655282253));
#80891=CARTESIAN_POINT('Ctrl Pts',(156.934188015448,-224.288114715028,9.75463062185952));
#80892=CARTESIAN_POINT('Ctrl Pts',(157.538401154934,-222.541385743175,9.66476540248591));
#80893=CARTESIAN_POINT('Ctrl Pts',(160.44615220686,-221.394703452409,9.52198089470169));
#80894=CARTESIAN_POINT('Ctrl Pts',(163.270875997921,-223.419308634178,9.36322302946991));
#80895=CARTESIAN_POINT('Ctrl Pts',(163.102094204308,-226.890562491788,9.20446516423811));
#80896=CARTESIAN_POINT('Ctrl Pts',(160.0942759169,-228.631573631259,9.04570729900633));
#80897=CARTESIAN_POINT('Ctrl Pts',(157.411955292478,-227.259590074809,8.90807776186779));
#80898=CARTESIAN_POINT('Ctrl Pts',(156.933478371343,-225.614304736623,8.82336751313986));
#80899=CARTESIAN_POINT('Ctrl Pts',(156.93057593278,-224.998402339592,8.79157655282253));
#80900=CARTESIAN_POINT('Origin',(160.,-225.,22.2084234471774));
#80901=CARTESIAN_POINT('',(156.921326297986,-225.000055941926,10.7915765528225));
#80902=CARTESIAN_POINT('',(156.931207720544,-224.999191249524,10.7084234471774));
#80903=CARTESIAN_POINT('',(156.9265,-225.,22.2084234471774));
#80904=CARTESIAN_POINT('Ctrl Pts',(156.931207720544,-224.999191249524,10.7084234471774));
#80905=CARTESIAN_POINT('Ctrl Pts',(156.930117074624,-224.536271754528,10.684541288295));
#80906=CARTESIAN_POINT('Ctrl Pts',(157.245771332218,-223.049004123232,10.6077398410019));
#80907=CARTESIAN_POINT('Ctrl Pts',(159.553847748865,-221.394703094632,10.4780191052983));
#80908=CARTESIAN_POINT('Ctrl Pts',(162.786890342936,-222.669665297966,10.3192612400665));
#80909=CARTESIAN_POINT('Ctrl Pts',(163.469371004743,-226.077349728964,10.1605033748347));
#80910=CARTESIAN_POINT('Ctrl Pts',(160.97668345944,-228.499043730379,10.0017455096029));
#80911=CARTESIAN_POINT('Ctrl Pts',(157.762164571223,-227.758067396816,9.85105220038384));
#80912=CARTESIAN_POINT('Ctrl Pts',(156.931300461478,-225.861836250725,9.75327817957534));
#80913=CARTESIAN_POINT('Ctrl Pts',(156.923921662128,-224.997622030861,9.70842344717744));
#80914=CARTESIAN_POINT('Ctrl Pts',(156.921326791759,-225.000055936587,10.7915765528225));
#80915=CARTESIAN_POINT('Ctrl Pts',(156.921598853813,-223.985720094541,10.7388130189898));
#80916=CARTESIAN_POINT('Ctrl Pts',(158.024018310351,-221.953547412004,10.6331301967464));
#80917=CARTESIAN_POINT('Ctrl Pts',(161.48554880872,-221.684828854392,10.4745280860924));
#80918=CARTESIAN_POINT('Ctrl Pts',(163.590904478153,-224.449890904874,10.3157702208607));
#80919=CARTESIAN_POINT('Ctrl Pts',(162.40986451039,-227.718412777583,10.1570123556289));
#80920=CARTESIAN_POINT('Ctrl Pts',(159.023316637483,-228.499043383147,9.99825449039708));
#80921=CARTESIAN_POINT('Ctrl Pts',(157.110724396174,-226.64092315197,9.87644255612829));
#80922=CARTESIAN_POINT('Ctrl Pts',(156.925905528579,-225.311525232587,9.80754991027011));
#80923=CARTESIAN_POINT('Ctrl Pts',(156.928405545629,-225.002615145101,9.79157655282253));
#80924=CARTESIAN_POINT('Origin',(160.,-225.,22.2084234471774));
#80925=CARTESIAN_POINT('',(156.928242529572,-224.997349454313,11.7915765528225));
#80926=CARTESIAN_POINT('',(156.926885880558,-225.002805879099,11.7084234471774));
#80927=CARTESIAN_POINT('',(156.9265,-225.,22.2084234471774));
#80928=CARTESIAN_POINT('Ctrl Pts',(156.926885880558,-225.002805879099,11.7084234471774));
#80929=CARTESIAN_POINT('Ctrl Pts',(156.933817492414,-224.236012305719,11.6687236854252));
#80930=CARTESIAN_POINT('Ctrl Pts',(157.612129562918,-222.436152686531,11.5761046352624));
#80931=CARTESIAN_POINT('Ctrl Pts',(160.632612786331,-221.422707913851,11.4305662966891));
#80932=CARTESIAN_POINT('Ctrl Pts',(163.348485101673,-223.591147583697,11.2718084314573));
#80933=CARTESIAN_POINT('Ctrl Pts',(162.99982398364,-227.048968929542,11.1130505662255));
#80934=CARTESIAN_POINT('Ctrl Pts',(159.905724073745,-228.631573991643,10.9542927009937));
#80935=CARTESIAN_POINT('Ctrl Pts',(157.350375677299,-227.152465349322,10.8194169946443));
#80936=CARTESIAN_POINT('Ctrl Pts',(156.93253378269,-225.562032046432,10.7374605767056));
#80937=CARTESIAN_POINT('Ctrl Pts',(156.931207720544,-224.999191249524,10.7084234471774));
#80938=CARTESIAN_POINT('Ctrl Pts',(156.928242529572,-224.997349454313,11.7915765528225));
#80939=CARTESIAN_POINT('Ctrl Pts',(156.925748442923,-224.694504338069,11.7759147045306));
#80940=CARTESIAN_POINT('Ctrl Pts',(157.106002150711,-223.371289913171,11.7073335678281));
#80941=CARTESIAN_POINT('Ctrl Pts',(159.00278787731,-221.506751802388,11.585833142715));
#80942=CARTESIAN_POINT('Ctrl Pts',(162.393861057113,-222.267483901785,11.4270752774832));
#80943=CARTESIAN_POINT('Ctrl Pts',(163.594072691582,-225.529014626816,11.2683174122514));
#80944=CARTESIAN_POINT('Ctrl Pts',(161.504989140049,-228.306391186187,11.1095595470196));
#80945=CARTESIAN_POINT('Ctrl Pts',(158.038539586726,-228.057758661981,10.9508016817878));
#80946=CARTESIAN_POINT('Ctrl Pts',(156.922685842577,-226.023373791017,10.8448073503888));
#80947=CARTESIAN_POINT('Ctrl Pts',(156.921325988649,-225.00305019113,10.7917323074004));
#80948=CARTESIAN_POINT('Ctrl Pts',(156.921326791759,-225.000055936587,10.7915765528225));
#80949=CARTESIAN_POINT('Origin',(160.,-225.,22.2084234471774));
#80950=CARTESIAN_POINT('',(156.930668110786,-225.001514698659,12.7915765528225));
#80951=CARTESIAN_POINT('',(156.921656046805,-224.999087139428,12.7084234471775));
#80952=CARTESIAN_POINT('',(156.9265,-225.,22.2084234471774));
#80953=CARTESIAN_POINT('Ctrl Pts',(156.921656046805,-224.999087139428,12.7084234471775));
#80954=CARTESIAN_POINT('Ctrl Pts',(156.921460289156,-224.949126905353,12.7058253709661));
#80955=CARTESIAN_POINT('Ctrl Pts',(156.945200515863,-223.881734459432,12.6503080063441));
#80956=CARTESIAN_POINT('Ctrl Pts',(158.181336908062,-221.855213494516,12.5418713533116));
#80957=CARTESIAN_POINT('Ctrl Pts',(161.655556273132,-221.766371846742,12.3831134880798));
#80958=CARTESIAN_POINT('Ctrl Pts',(163.614610602134,-224.63694655767,12.224355622848));
#80959=CARTESIAN_POINT('Ctrl Pts',(162.265573450205,-227.839787764742,12.0655977576162));
#80960=CARTESIAN_POINT('Ctrl Pts',(158.843083565739,-228.443655321194,11.9068398923844));
#80961=CARTESIAN_POINT('Ctrl Pts',(157.070476843345,-226.532996300179,11.7877817889048));
#80962=CARTESIAN_POINT('Ctrl Pts',(156.924577740064,-225.258138597417,11.7216429738358));
#80963=CARTESIAN_POINT('Ctrl Pts',(156.926885880558,-225.002805879099,11.7084234471774));
#80964=CARTESIAN_POINT('Ctrl Pts',(156.930668110786,-225.001514698659,12.7915765528225));
#80965=CARTESIAN_POINT('Ctrl Pts',(156.933388035073,-224.391601484776,12.7600971016609));
#80966=CARTESIAN_POINT('Ctrl Pts',(157.404784898217,-222.752504368794,12.6756983620886));
#80967=CARTESIAN_POINT('Ctrl Pts',(160.072950506571,-221.367935406501,12.5383803341058));
#80968=CARTESIAN_POINT('Ctrl Pts',(163.090939768701,-223.091255298888,12.379622468874));
#80969=CARTESIAN_POINT('Ctrl Pts',(163.280101076064,-226.561458266673,12.2208646036422));
#80970=CARTESIAN_POINT('Ctrl Pts',(160.467314007601,-228.602614690202,12.0621067384104));
#80971=CARTESIAN_POINT('Ctrl Pts',(157.546521678506,-227.470561434611,11.9190107214705));
#80972=CARTESIAN_POINT('Ctrl Pts',(156.934175627776,-225.717777437869,11.8288339929412));
#80973=CARTESIAN_POINT('Ctrl Pts',(156.928242529572,-224.997349454313,11.7915765528225));
#80974=CARTESIAN_POINT('Origin',(160.,-225.,22.2084234471774));
#80975=CARTESIAN_POINT('',(156.92271430011,-225.001830538963,13.7915765528225));
#80976=CARTESIAN_POINT('',(156.929571866433,-224.997773335875,13.7084234471774));
#80977=CARTESIAN_POINT('',(156.9265,-225.,22.2084234471774));
#80978=CARTESIAN_POINT('Ctrl Pts',(156.929571866433,-224.997773335875,13.7084234471774));
#80979=CARTESIAN_POINT('Ctrl Pts',(156.92718067855,-224.641289583268,13.6900077680964));
#80980=CARTESIAN_POINT('Ctrl Pts',(157.149280048035,-223.263300523479,13.6186728006047));
#80981=CARTESIAN_POINT('Ctrl Pts',(159.185378793971,-221.459716127521,13.4944185447024));
#80982=CARTESIAN_POINT('Ctrl Pts',(162.532414001985,-222.395370097384,13.3356606794706));
#80983=CARTESIAN_POINT('Ctrl Pts',(163.561784014967,-225.714781251697,13.1769028142388));
#80984=CARTESIAN_POINT('Ctrl Pts',(161.331409437515,-228.380024632565,13.018144949007));
#80985=CARTESIAN_POINT('Ctrl Pts',(157.938970005041,-227.958876369796,12.8619851599865));
#80986=CARTESIAN_POINT('Ctrl Pts',(156.925447606946,-225.966749107697,12.7587446593767));
#80987=CARTESIAN_POINT('Ctrl Pts',(156.921656046805,-224.999087139428,12.7084234471775));
#80988=CARTESIAN_POINT('Ctrl Pts',(156.92271430011,-225.001830538963,13.7915765528225));
#80989=CARTESIAN_POINT('Ctrl Pts',(156.929131207107,-224.09149465488,13.7442794987911));
#80990=CARTESIAN_POINT('Ctrl Pts',(157.838867262768,-222.151467797283,13.6440631563491));
#80991=CARTESIAN_POINT('Ctrl Pts',(161.136676006379,-221.549611232878,13.4909275254965));
#80992=CARTESIAN_POINT('Ctrl Pts',(163.515274940119,-224.083453720138,13.3321696602647));
#80993=CARTESIAN_POINT('Ctrl Pts',(162.676694386897,-227.456119326685,13.1734117950329));
#80994=CARTESIAN_POINT('Ctrl Pts',(159.388403236045,-228.580944622035,13.0146539298011));
#80995=CARTESIAN_POINT('Ctrl Pts',(157.200880047322,-226.855291100656,12.887375515731));
#80996=CARTESIAN_POINT('Ctrl Pts',(156.92881564094,-225.416910760505,12.8130163900715));
#80997=CARTESIAN_POINT('Ctrl Pts',(156.930668110786,-225.001514698659,12.7915765528225));
#80998=CARTESIAN_POINT('Origin',(160.,-225.,22.2084234471774));
#80999=CARTESIAN_POINT('',(156.925120103303,-224.997319770149,14.7915765528225));
#81000=CARTESIAN_POINT('',(156.929686978342,-225.002172463972,14.7084234471774));
#81001=CARTESIAN_POINT('',(156.9265,-225.,22.2084234471774));
#81002=CARTESIAN_POINT('Ctrl Pts',(156.929686978341,-225.002172463972,14.7084234471774));
#81003=CARTESIAN_POINT('Ctrl Pts',(156.934013357123,-224.339435068042,14.6741901652266));
#81004=CARTESIAN_POINT('Ctrl Pts',(157.470014897917,-222.645831187287,14.5870375948652));
#81005=CARTESIAN_POINT('Ctrl Pts',(160.261302595496,-221.376612281216,14.4469657360931));
#81006=CARTESIAN_POINT('Ctrl Pts',(163.185812326331,-223.254200060589,14.2882078708613));
#81007=CARTESIAN_POINT('Ctrl Pts',(163.194666741387,-226.72954387586,14.1294500056295));
#81008=CARTESIAN_POINT('Ctrl Pts',(160.279762280353,-228.622009203956,13.9706921403977));
#81009=CARTESIAN_POINT('Ctrl Pts',(157.476644106943,-227.364607853831,13.830349954247));
#81010=CARTESIAN_POINT('Ctrl Pts',(156.934051995142,-225.665681159316,13.7429270565069));
#81011=CARTESIAN_POINT('Ctrl Pts',(156.929571866433,-224.997773335875,13.7084234471774));
#81012=CARTESIAN_POINT('Ctrl Pts',(156.925120103303,-224.997319770149,14.7915765528225));
#81013=CARTESIAN_POINT('Ctrl Pts',(156.923321208696,-224.800687892348,14.781381184332));
#81014=CARTESIAN_POINT('Ctrl Pts',(157.030083149926,-223.585379624,14.7182665274308));
#81015=CARTESIAN_POINT('Ctrl Pts',(158.648766902918,-221.627851707722,14.6022325821191));
#81016=CARTESIAN_POINT('Ctrl Pts',(162.100101577621,-222.035748264497,14.4434747168873));
#81017=CARTESIAN_POINT('Ctrl Pts',(163.629423371069,-225.156527893037,14.2847168516555));
#81018=CARTESIAN_POINT('Ctrl Pts',(161.837097038039,-228.134053200026,14.1259589864237));
#81019=CARTESIAN_POINT('Ctrl Pts',(158.363459568037,-228.243293141594,13.9672011211919));
#81020=CARTESIAN_POINT('Ctrl Pts',(156.976235624899,-226.236029500378,13.8557403099915));
#81021=CARTESIAN_POINT('Ctrl Pts',(156.921951517821,-225.110042811564,13.7971987872017));
#81022=CARTESIAN_POINT('Ctrl Pts',(156.92271430011,-225.001830538963,13.7915765528225));
#81023=CARTESIAN_POINT('Origin',(160.,-225.,22.2084234471774));
#81024=CARTESIAN_POINT('',(156.931399319499,-224.999857957544,15.7915765528225));
#81025=CARTESIAN_POINT('',(156.92172471093,-225.001003143772,15.7084234471775));
#81026=CARTESIAN_POINT('',(156.9265,-225.,22.2084234471774));
#81027=CARTESIAN_POINT('Ctrl Pts',(156.92172471093,-225.001003143772,15.7084234471775));
#81028=CARTESIAN_POINT('Ctrl Pts',(156.92582434592,-224.038482243449,15.6583725623569));
#81029=CARTESIAN_POINT('Ctrl Pts',(157.929788564316,-222.050905119068,15.5554023891257));
#81030=CARTESIAN_POINT('Ctrl Pts',(161.314169139266,-221.613235012514,15.3995129274839));
#81031=CARTESIAN_POINT('Ctrl Pts',(163.558095586257,-224.267078854098,15.2407550622521));
#81032=CARTESIAN_POINT('Ctrl Pts',(162.545653092624,-227.591692099587,15.0819971970203));
#81033=CARTESIAN_POINT('Ctrl Pts',(159.203428988727,-228.544388837452,14.9232393317885));
#81034=CARTESIAN_POINT('Ctrl Pts',(157.153716789256,-226.747301603524,14.7987147485075));
#81035=CARTESIAN_POINT('Ctrl Pts',(156.927325453613,-225.363923209321,14.7271094536372));
#81036=CARTESIAN_POINT('Ctrl Pts',(156.929686978341,-225.002172463972,14.7084234471774));
#81037=CARTESIAN_POINT('Ctrl Pts',(156.931399319499,-224.999857957544,15.7915765528225));
#81038=CARTESIAN_POINT('Ctrl Pts',(156.931191404653,-224.495557499134,15.7655635814622));
#81039=CARTESIAN_POINT('Ctrl Pts',(157.287359937792,-222.96561384056,15.6866313216913));
#81040=CARTESIAN_POINT('Ctrl Pts',(159.698974947405,-221.379696296506,15.5547797735098));
#81041=CARTESIAN_POINT('Ctrl Pts',(162.878214854917,-222.783449924613,15.396021908278));
#81042=CARTESIAN_POINT('Ctrl Pts',(163.423312640378,-226.215790094536,15.2372640430462));
#81043=CARTESIAN_POINT('Ctrl Pts',(160.83539483199,-228.535439217757,15.0785061778144));
#81044=CARTESIAN_POINT('Ctrl Pts',(157.698218100801,-227.67827869048,14.9299436810732));
#81045=CARTESIAN_POINT('Ctrl Pts',(156.932658411426,-225.821310056393,14.8343004727426));
#81046=CARTESIAN_POINT('Ctrl Pts',(156.925120103303,-224.997319770149,14.7915765528225));
#81047=CARTESIAN_POINT('Origin',(160.,-225.,22.2084234471774));
#81048=CARTESIAN_POINT('',(156.925641387687,-225.002754763835,16.7915765528225));
#81049=CARTESIAN_POINT('',(156.926729566011,-224.997190773455,16.7084234471774));
#81050=CARTESIAN_POINT('',(156.9265,-225.,22.2084234471774));
#81051=CARTESIAN_POINT('Ctrl Pts',(156.926729566011,-224.997190773455,16.7084234471775));
#81052=CARTESIAN_POINT('Ctrl Pts',(156.92445588536,-224.747111827224,16.6954742478977));
#81053=CARTESIAN_POINT('Ctrl Pts',(157.066706082429,-223.477592372542,16.6296057602074));
#81054=CARTESIAN_POINT('Ctrl Pts',(158.825551339689,-221.562284486778,16.5108179841064));
#81055=CARTESIAN_POINT('Ctrl Pts',(162.251073816965,-222.14870480692,16.3520601188746));
#81056=CARTESIAN_POINT('Ctrl Pts',(163.616413625555,-225.344630375999,16.1933022536428));
#81057=CARTESIAN_POINT('Ctrl Pts',(161.672011826211,-228.225150238345,16.034544388411));
#81058=CARTESIAN_POINT('Ctrl Pts',(158.197384869287,-228.154012729466,15.8757865231792));
#81059=CARTESIAN_POINT('Ctrl Pts',(156.947830997159,-226.12878059073,15.767079542768));
#81060=CARTESIAN_POINT('Ctrl Pts',(156.921489761883,-225.056164973894,15.7112918507675));
#81061=CARTESIAN_POINT('Ctrl Pts',(156.92172471093,-225.001003143772,15.7084234471775));
#81062=CARTESIAN_POINT('Ctrl Pts',(156.925641387687,-225.002754763835,16.7915765528225));
#81063=CARTESIAN_POINT('Ctrl Pts',(156.933090194617,-224.195641887624,16.7497459785925));
#81064=CARTESIAN_POINT('Ctrl Pts',(157.672221791135,-222.355388035489,16.6549961159518));
#81065=CARTESIAN_POINT('Ctrl Pts',(160.775745345963,-221.450995329772,16.5073269649006));
#81066=CARTESIAN_POINT('Ctrl Pts',(163.402355370953,-223.726739257298,16.3485690996688));
#81067=CARTESIAN_POINT('Ctrl Pts',(162.915129893092,-227.167771365402,16.189811234437));
#81068=CARTESIAN_POINT('Ctrl Pts',(159.759977652262,-228.624859205653,16.0310533692052));
#81069=CARTESIAN_POINT('Ctrl Pts',(157.305482029995,-227.069305626613,15.8983084753337));
#81070=CARTESIAN_POINT('Ctrl Pts',(156.931614374622,-225.521477261799,15.8184828698728));
#81071=CARTESIAN_POINT('Ctrl Pts',(156.931399319499,-224.999857957544,15.7915765528225));
#81072=CARTESIAN_POINT('Origin',(160.,-225.,22.2084234471774));
#81073=CARTESIAN_POINT('',(156.92234129012,-224.998416744957,17.7915765528225));
#81074=CARTESIAN_POINT('',(156.93124676379,-225.000725938288,17.7084234471774));
#81075=CARTESIAN_POINT('',(156.9265,-225.,22.2084234471774));
#81076=CARTESIAN_POINT('Ctrl Pts',(156.93124676379,-225.000725938288,17.7084234471775));
#81077=CARTESIAN_POINT('Ctrl Pts',(156.932425088148,-224.443107314068,17.679656645028));
#81078=CARTESIAN_POINT('Ctrl Pts',(157.344548556821,-222.858073213756,17.5979705544679));
#81079=CARTESIAN_POINT('Ctrl Pts',(159.887220510682,-221.3689535564,17.4633651754972));
#81080=CARTESIAN_POINT('Ctrl Pts',(162.989344456746,-222.935771972903,17.3046073102654));
#81081=CARTESIAN_POINT('Ctrl Pts',(163.355620479822,-226.391771827016,17.1458494450336));
#81082=CARTESIAN_POINT('Ctrl Pts',(160.650832768699,-228.574022146095,16.9870915798018));
#81083=CARTESIAN_POINT('Ctrl Pts',(157.619604864121,-227.574127701187,16.8412829138497));
#81084=CARTESIAN_POINT('Ctrl Pts',(156.933747700207,-225.769105511554,16.7483935363083));
#81085=CARTESIAN_POINT('Ctrl Pts',(156.926729566011,-224.997190773455,16.7084234471775));
#81086=CARTESIAN_POINT('Ctrl Pts',(156.92234129012,-224.998416744957,17.7915765528225));
#81087=CARTESIAN_POINT('Ctrl Pts',(156.92177007721,-224.907427920962,17.7868476641333));
#81088=CARTESIAN_POINT('Ctrl Pts',(156.966697439976,-223.798787972635,17.7291994870335));
#81089=CARTESIAN_POINT('Ctrl Pts',(158.309079915571,-221.784723458447,17.6186320215231));
#81090=CARTESIAN_POINT('Ctrl Pts',(161.784064171446,-221.835457356522,17.4598741562913));
#81091=CARTESIAN_POINT('Ctrl Pts',(163.626273157879,-224.782380735109,17.3011162910595));
#81092=CARTESIAN_POINT('Ctrl Pts',(162.149717001196,-227.928469170749,17.1423584258277));
#81093=CARTESIAN_POINT('Ctrl Pts',(158.705739973713,-228.394422777744,16.983600560596));
#81094=CARTESIAN_POINT('Ctrl Pts',(157.041609861784,-226.449569354426,16.8666732695942));
#81095=CARTESIAN_POINT('Ctrl Pts',(156.923666810657,-225.21670936906,16.8026652670031));
#81096=CARTESIAN_POINT('Ctrl Pts',(156.925641387687,-225.002754763835,16.7915765528225));
#81097=CARTESIAN_POINT('Origin',(160.,-225.,22.2084234471774));
#81098=CARTESIAN_POINT('',(156.93039533859,-224.998257313349,18.7915765528225));
#81099=CARTESIAN_POINT('',(156.924068591467,-225.002427532313,18.7084234471774));
#81100=CARTESIAN_POINT('',(156.9265,-225.,22.2084234471774));
#81101=CARTESIAN_POINT('Ctrl Pts',(156.924068591467,-225.002427532313,18.7084234471774));
#81102=CARTESIAN_POINT('Ctrl Pts',(156.931499764956,-224.143315612363,18.6638390421582));
#81103=CARTESIAN_POINT('Ctrl Pts',(157.753898913639,-222.252010296725,18.5663353487284));
#81104=CARTESIAN_POINT('Ctrl Pts',(160.95884158646,-221.496026267553,18.4159123668879));
#81105=CARTESIAN_POINT('Ctrl Pts',(163.463836160053,-223.904985354727,18.2571545016561));
#81106=CARTESIAN_POINT('Ctrl Pts',(162.798728517017,-227.31610406828,18.0983966364243));
#81107=CARTESIAN_POINT('Ctrl Pts',(159.572224403905,-228.607523337571,17.9396387711925));
#81108=CARTESIAN_POINT('Ctrl Pts',(157.250921105224,-226.961581956951,17.8096477081102));
#81109=CARTESIAN_POINT('Ctrl Pts',(156.930257447609,-225.468900193126,17.7325759334386));
#81110=CARTESIAN_POINT('Ctrl Pts',(156.93124676379,-225.000725938288,17.7084234471775));
#81111=CARTESIAN_POINT('Ctrl Pts',(156.93039533859,-224.998257313349,18.7915765528225));
#81112=CARTESIAN_POINT('Ctrl Pts',(156.9283328603,-224.600256690347,18.7710300612636));
#81113=CARTESIAN_POINT('Ctrl Pts',(157.185172027845,-223.179723982655,18.697564281294));
#81114=CARTESIAN_POINT('Ctrl Pts',(159.328201303672,-221.429869438357,18.5711792129139));
#81115=CARTESIAN_POINT('Ctrl Pts',(162.634953676974,-222.499153818262,18.4124213476821));
#81116=CARTESIAN_POINT('Ctrl Pts',(163.530211716637,-225.857226698665,18.2536634824503));
#81117=CARTESIAN_POINT('Ctrl Pts',(161.194612821702,-228.430758907163,18.0949056172185));
#81118=CARTESIAN_POINT('Ctrl Pts',(157.867843947502,-227.8813321041,17.9408766406759));
#81119=CARTESIAN_POINT('Ctrl Pts',(156.92816231495,-225.925651046016,17.8397669525439));
#81120=CARTESIAN_POINT('Ctrl Pts',(156.92234129012,-224.998416744957,17.7915765528225));
#81121=CARTESIAN_POINT('Origin',(160.,-225.,22.2084234471774));
#81122=CARTESIAN_POINT('',(156.929637641087,-225.003026239314,19.7915765528225));
#81123=CARTESIAN_POINT('',(156.923621975382,-224.997773684101,19.7084234471775));
#81124=CARTESIAN_POINT('',(156.9265,-225.,22.2084234471774));
#81125=CARTESIAN_POINT('',(159.206200717467,-227.969222953746,20.));
#81126=CARTESIAN_POINT('Ctrl Pts',(159.206200717467,-227.969222953746,20.));
#81127=CARTESIAN_POINT('Ctrl Pts',(158.218929051303,-227.70528334649,19.9470807115894));
#81128=CARTESIAN_POINT('Ctrl Pts',(157.120586512374,-226.663342975009,19.8776062291969));
#81129=CARTESIAN_POINT('Ctrl Pts',(156.927233104428,-225.32322870017,19.8081317468044));
#81130=CARTESIAN_POINT('Ctrl Pts',(156.929637641087,-225.003026239314,19.7915765528225));
#81131=CARTESIAN_POINT('',(160.795594448913,-227.974557142491,20.));
#81132=CARTESIAN_POINT('Origin',(160.,-225.,20.));
#81133=CARTESIAN_POINT('Ctrl Pts',(160.795596250783,-227.974562496599,20.));
#81134=CARTESIAN_POINT('Ctrl Pts',(159.833965257065,-228.230145509978,19.948244384658));
#81135=CARTESIAN_POINT('Ctrl Pts',(157.769883342468,-227.756381737407,19.8510522003838));
#81136=CARTESIAN_POINT('Ctrl Pts',(156.930816867245,-225.872804859128,19.7538600161097));
#81137=CARTESIAN_POINT('Ctrl Pts',(156.923621975382,-224.997773684101,19.7084234471775));
#81138=CARTESIAN_POINT('Origin',(0.,-225.,22.2084234471774));
#81139=CARTESIAN_POINT('',(-3.07861202077411,-224.999832022693,0.791576552822534));
#81140=CARTESIAN_POINT('',(-3.0685846317264,-224.999284761019,0.708423447177441));
#81141=CARTESIAN_POINT('',(-3.0735,-225.,22.2084234471774));
#81142=CARTESIAN_POINT('',(0.793799282532883,-227.969222953746,0.));
#81143=CARTESIAN_POINT('Ctrl Pts',(-3.0685846317264,-224.999284761019,0.708423447177441));
#81144=CARTESIAN_POINT('Ctrl Pts',(-3.06942175779765,-224.525030255484,
0.683959451760685));
#81145=CARTESIAN_POINT('Ctrl Pts',(-2.74289872526648,-223.026084056979,
0.606576167933331));
#81146=CARTESIAN_POINT('Ctrl Pts',(-0.407268923958301,-221.390844620734,
0.476273595695375));
#81147=CARTESIAN_POINT('Ctrl Pts',(2.81363672347351,-222.698855636535,0.317515730463589));
#81148=CARTESIAN_POINT('Ctrl Pts',(3.45438722685837,-226.118548219769,0.158757865231791));
#81149=CARTESIAN_POINT('Ctrl Pts',(1.7810709486973,-227.70528334649,0.0529192884105984));
#81150=CARTESIAN_POINT('Ctrl Pts',(0.793799282532894,-227.969222953746,
0.));
#81151=CARTESIAN_POINT('',(-0.79379928253288,-227.969222953746,0.));
#81152=CARTESIAN_POINT('Origin',(0.,-225.,0.));
#81153=CARTESIAN_POINT('Ctrl Pts',(-3.07861202077411,-224.999832022693,
0.791576552822534));
#81154=CARTESIAN_POINT('Ctrl Pts',(-3.07861796321176,-224.991641138211,
0.791150470866062));
#81155=CARTESIAN_POINT('Ctrl Pts',(-3.0748810844841,-223.966150069617,0.737805100498994));
#81156=CARTESIAN_POINT('Ctrl Pts',(-1.94583857424385,-221.93245816329,0.631540441721324));
#81157=CARTESIAN_POINT('Ctrl Pts',(1.52182610974532,-221.701128880727,0.472782576489534));
#81158=CARTESIAN_POINT('Ctrl Pts',(3.59659356700835,-224.489814123823,0.314024711257741));
#81159=CARTESIAN_POINT('Ctrl Pts',(2.38892380770087,-227.719767850893,0.156430519094562));
#81160=CARTESIAN_POINT('Ctrl Pts',(0.166093791691783,-228.230152288131,
0.0517556153419859));
#81161=CARTESIAN_POINT('Ctrl Pts',(-0.795579109021638,-227.974527535833,
5.47833805229769E-15));
#81162=CARTESIAN_POINT('Origin',(0.,-225.,22.2084234471774));
#81163=CARTESIAN_POINT('',(-3.07140453603582,-224.997418081988,1.79157655282252));
#81164=CARTESIAN_POINT('',(-3.0734003899706,-225.00280942625,1.70842344717744));
#81165=CARTESIAN_POINT('',(-3.0735,-225.,22.2084234471774));
#81166=CARTESIAN_POINT('Ctrl Pts',(-3.0734003899706,-225.00280942625,1.70842344717744));
#81167=CARTESIAN_POINT('Ctrl Pts',(-3.0662887666649,-224.225007664595,1.66814184889093));
#81168=CARTESIAN_POINT('Ctrl Pts',(-2.37168479031072,-222.414076548772,
1.57494096219383));
#81169=CARTESIAN_POINT('Ctrl Pts',(0.671786427681058,-221.42993104244,1.42882078708613));
#81170=CARTESIAN_POINT('Ctrl Pts',(3.36369894488889,-223.627956478202,1.27006292185434));
#81171=CARTESIAN_POINT('Ctrl Pts',(2.97708229266655,-227.081755146954,1.11130505662255));
#81172=CARTESIAN_POINT('Ctrl Pts',(-0.134013670091176,-228.630171025583,
0.952547191390754));
#81173=CARTESIAN_POINT('Ctrl Pts',(-2.66220315787947,-227.129884296831,
0.818253321575719));
#81174=CARTESIAN_POINT('Ctrl Pts',(-3.0676109286487,-225.55091382564,0.736878740171282));
#81175=CARTESIAN_POINT('Ctrl Pts',(-3.0685846317264,-224.999284761019,0.708423447177441));
#81176=CARTESIAN_POINT('Ctrl Pts',(-3.07140453603582,-224.997418081988,
1.79157655282252));
#81177=CARTESIAN_POINT('Ctrl Pts',(-3.07390614987845,-224.683249285408,
1.77533286799631));
#81178=CARTESIAN_POINT('Ctrl Pts',(-2.88509446209608,-223.348504675664,
1.70616989475949));
#81179=CARTESIAN_POINT('Ctrl Pts',(-0.958825609453758,-221.496084913414,
1.58408763311208));
#81180=CARTESIAN_POINT('Ctrl Pts',(2.42364543444732,-222.293943229063,1.42532976788028));
#81181=CARTESIAN_POINT('Ctrl Pts',(3.58799453273333,-225.568397245971,1.2665719026485));
#81182=CARTESIAN_POINT('Ctrl Pts',(1.46861470818642,-228.322628432602,1.1078140374167));
#81183=CARTESIAN_POINT('Ctrl Pts',(-1.98555300558023,-228.036811542638,
0.949482254141381));
#81184=CARTESIAN_POINT('Ctrl Pts',(-3.07787991371872,-226.008947249495,
0.844069759276661));
#81185=CARTESIAN_POINT('Ctrl Pts',(-3.07861202077411,-224.999832022693,
0.791576552822534));
#81186=CARTESIAN_POINT('Origin',(0.,-225.,22.2084234471774));
#81187=CARTESIAN_POINT('',(-3.0694574394746,-225.001668045267,2.79157655282253));
#81188=CARTESIAN_POINT('',(-3.07813805695758,-224.998894504048,2.70842344717744));
#81189=CARTESIAN_POINT('',(-3.0735,-225.,22.2084234471774));
#81190=CARTESIAN_POINT('Ctrl Pts',(-3.07813805695758,-224.998894504048,
2.70842344717744));
#81191=CARTESIAN_POINT('Ctrl Pts',(-3.07842163656956,-224.937738546132,
2.70524353443178));
#81192=CARTESIAN_POINT('Ctrl Pts',(-3.04905256116106,-223.859118502933,
2.64914433327553));
#81193=CARTESIAN_POINT('Ctrl Pts',(-1.78403472552871,-221.835509530578,
2.54012584370868));
#81194=CARTESIAN_POINT('Ctrl Pts',(1.69089215999812,-221.784776548785,2.38136797847689));
#81195=CARTESIAN_POINT('Ctrl Pts',(3.61831511248521,-224.676615388503,2.2226101132451));
#81196=CARTESIAN_POINT('Ctrl Pts',(2.23425519005939,-227.864416938342,2.0638522480133));
#81197=CARTESIAN_POINT('Ctrl Pts',(-1.19459291014185,-228.430701931157,
1.90509438278151));
#81198=CARTESIAN_POINT('Ctrl Pts',(-2.93755249238743,-226.510184003648,
1.78661811583622));
#81199=CARTESIAN_POINT('Ctrl Pts',(-3.07563154502501,-225.246831959117,
1.72106113730153));
#81200=CARTESIAN_POINT('Ctrl Pts',(-3.0734003899706,-225.00280942625,1.70842344717744));
#81201=CARTESIAN_POINT('Ctrl Pts',(-3.0694574394746,-225.001668045267,2.79157655282253));
#81202=CARTESIAN_POINT('Ctrl Pts',(-3.06639637311186,-224.380581303629,
2.75951526512656));
#81203=CARTESIAN_POINT('Ctrl Pts',(-2.58173685518177,-222.729957206475,
2.67453468902));
#81204=CARTESIAN_POINT('Ctrl Pts',(0.112777615932726,-221.369013886482,
2.53663482450283));
#81205=CARTESIAN_POINT('Ctrl Pts',(3.11163596998505,-223.125299771423,2.37787695927105));
#81206=CARTESIAN_POINT('Ctrl Pts',(3.26272518188304,-226.597311412118,2.21911909403925));
#81207=CARTESIAN_POINT('Ctrl Pts',(0.427768485964111,-228.607463345116,
2.06036122880746));
#81208=CARTESIAN_POINT('Ctrl Pts',(-2.46856013316054,-227.448198100151,
1.91784704840188));
#81209=CARTESIAN_POINT('Ctrl Pts',(-3.06575629805317,-225.706760227272,
1.8282521564069));
#81210=CARTESIAN_POINT('Ctrl Pts',(-3.07140453603582,-224.997418081988,
1.79157655282252));
#81211=CARTESIAN_POINT('Origin',(0.,-225.,22.2084234471774));
#81212=CARTESIAN_POINT('',(-3.07748283886488,-225.001672003054,3.79157655282253));
#81213=CARTESIAN_POINT('',(-3.07013331070642,-224.99789255212,3.70842344717744));
#81214=CARTESIAN_POINT('',(-3.0735,-225.,22.2084234471774));
#81215=CARTESIAN_POINT('Ctrl Pts',(-3.07013331070642,-224.99789255212,3.70842344717744));
#81216=CARTESIAN_POINT('Ctrl Pts',(-3.07245614163896,-224.630078505823,
3.68942593156204));
#81217=CARTESIAN_POINT('Ctrl Pts',(-2.84108107627447,-223.240510367213,
3.61750912753603));
#81218=CARTESIAN_POINT('Ctrl Pts',(-0.775732549268024,-221.451053872185,
3.49267303509943));
#81219=CARTESIAN_POINT('Ctrl Pts',(2.56078454381028,-222.423342844173,3.33391516986764));
#81220=CARTESIAN_POINT('Ctrl Pts',(3.55367173029338,-225.753788335947,3.17515730463585));
#81221=CARTESIAN_POINT('Ctrl Pts',(1.29423867433457,-228.394366788354,3.01639943940406));
#81222=CARTESIAN_POINT('Ctrl Pts',(-2.08069997222285,-227.93775373254,2.86082148691792));
#81223=CARTESIAN_POINT('Ctrl Pts',(-3.07370237774903,-225.955480237129,
2.75816282284238));
#81224=CARTESIAN_POINT('Ctrl Pts',(-3.07813805695758,-224.998894504048,
2.70842344717744));
#81225=CARTESIAN_POINT('Ctrl Pts',(-3.07748283886488,-225.001672003054,
3.79157655282253));
#81226=CARTESIAN_POINT('Ctrl Pts',(-3.07143809346347,-224.080348034814,
3.74369766225681));
#81227=CARTESIAN_POINT('Ctrl Pts',(-2.1422814352906,-222.130134246004,3.6428994832805));
#81228=CARTESIAN_POINT('Ctrl Pts',(1.17442914948988,-221.562341596822,3.48918201589359));
#81229=CARTESIAN_POINT('Ctrl Pts',(3.52505720816877,-224.122075853096,3.3304241506618));
#81230=CARTESIAN_POINT('Ctrl Pts',(2.64955304819789,-227.485286256663,3.17166628543001));
#81231=CARTESIAN_POINT('Ctrl Pts',(-0.650821956575191,-228.573962770645,
3.01290842019821));
#81232=CARTESIAN_POINT('Ctrl Pts',(-2.80933959903191,-226.832448718571,
2.88621184266239));
#81233=CARTESIAN_POINT('Ctrl Pts',(-3.07144886679926,-225.405726292203,
2.81243455353716));
#81234=CARTESIAN_POINT('Ctrl Pts',(-3.0694574394746,-225.001668045267,2.79157655282253));
#81235=CARTESIAN_POINT('Origin',(0.,-225.,22.2084234471774));
#81236=CARTESIAN_POINT('',(-3.07449021712595,-224.997267710685,4.79157655282253));
#81237=CARTESIAN_POINT('',(-3.07051359504914,-225.002286482744,4.70842344717744));
#81238=CARTESIAN_POINT('',(-3.0735,-225.,22.2084234471774));
#81239=CARTESIAN_POINT('Ctrl Pts',(-3.07051359504914,-225.002286482744,
4.70842344717744));
#81240=CARTESIAN_POINT('Ctrl Pts',(-3.0658581317049,-224.328435086706,4.67360832869229));
#81241=CARTESIAN_POINT('Ctrl Pts',(-2.51562439385663,-222.623410166854,
4.58587392179654));
#81242=CARTESIAN_POINT('Ctrl Pts',(0.301020087018748,-221.379756015497,
4.44522022649019));
#81243=CARTESIAN_POINT('Ctrl Pts',(3.20471397929018,-223.289272695415,4.2864623612584));
#81244=CARTESIAN_POINT('Ctrl Pts',(3.17545376384016,-226.764446937104,4.1277044960266));
#81245=CARTESIAN_POINT('Ctrl Pts',(0.240018388386984,-228.624799411569,
3.96894663079481));
#81246=CARTESIAN_POINT('Ctrl Pts',(-2.53753159714771,-227.342092904446,
3.82918628117842));
#81247=CARTESIAN_POINT('Ctrl Pts',(-3.0659856871576,-225.654657613507,3.74234521997263));
#81248=CARTESIAN_POINT('Ctrl Pts',(-3.07013331070642,-224.99789255212,3.70842344717744));
#81249=CARTESIAN_POINT('Ctrl Pts',(-3.07449021712595,-224.997267710685,
4.79157655282253));
#81250=CARTESIAN_POINT('Ctrl Pts',(-3.07640550402147,-224.789358748543,
4.78079934779766));
#81251=CARTESIAN_POINT('Ctrl Pts',(-2.96239880943811,-223.562643093719,
4.7171028543622));
#81252=CARTESIAN_POINT('Ctrl Pts',(-1.31414730730727,-221.61329127598,4.60048707251613));
#81253=CARTESIAN_POINT('Ctrl Pts',(2.13244942587199,-222.059007213082,4.44172920728434));
#81254=CARTESIAN_POINT('Ctrl Pts',(3.62742852835224,-225.196319633101,4.28297134205255));
#81255=CARTESIAN_POINT('Ctrl Pts',(1.80258518432463,-228.153960332663,4.12421347682076));
#81256=CARTESIAN_POINT('Ctrl Pts',(-1.67198404950171,-228.225096659724,
3.96545561158897));
#81257=CARTESIAN_POINT('Ctrl Pts',(-3.02996209952885,-226.213329983221,
3.85457663692289));
#81258=CARTESIAN_POINT('Ctrl Pts',(-3.0781191928266,-225.098663376268,3.79661695066741));
#81259=CARTESIAN_POINT('Ctrl Pts',(-3.07748283886488,-225.001672003054,
3.79157655282253));
#81260=CARTESIAN_POINT('Origin',(0.,-225.,22.2084234471774));
#81261=CARTESIAN_POINT('',(-3.06854459837578,-225.000042997605,5.79157655282253));
#81262=CARTESIAN_POINT('',(-3.0783646865402,-225.000807299621,5.70842344717745));
#81263=CARTESIAN_POINT('',(-3.0735,-225.,22.2084234471774));
#81264=CARTESIAN_POINT('Ctrl Pts',(-3.0783646865402,-225.000807299621,5.70842344717745));
#81265=CARTESIAN_POINT('Ctrl Pts',(-3.07494744526968,-224.027231919385,
5.65779072582254));
#81266=CARTESIAN_POINT('Ctrl Pts',(-2.0503586705405,-222.029922382093,5.55423871605704));
#81267=CARTESIAN_POINT('Ctrl Pts',(1.35121080771192,-221.627907333254,5.39776741788095));
#81268=CARTESIAN_POINT('Ctrl Pts',(3.56586047257395,-224.306156580971,5.23900955264915));
#81269=CARTESIAN_POINT('Ctrl Pts',(2.51703477316183,-227.619411298497,5.08025168741736));
#81270=CARTESIAN_POINT('Ctrl Pts',(-0.835381051670971,-228.535380898648,
4.92149382218557));
#81271=CARTESIAN_POINT('Ctrl Pts',(-2.85574300376166,-226.724453667661,
4.79755107543892));
#81272=CARTESIAN_POINT('Ctrl Pts',(-3.07293447721565,-225.352695176127,
4.72652761710288));
#81273=CARTESIAN_POINT('Ctrl Pts',(-3.07051359504914,-225.002286482744,
4.70842344717744));
#81274=CARTESIAN_POINT('Ctrl Pts',(-3.06854459837578,-225.000042997605,
5.79157655282253));
#81275=CARTESIAN_POINT('Ctrl Pts',(-3.06848025913913,-224.484469012775,
5.76498174492791));
#81276=CARTESIAN_POINT('Ctrl Pts',(-2.70083904555456,-222.942901484278,
5.6854676486227));
#81277=CARTESIAN_POINT('Ctrl Pts',(-0.261298254542071,-221.376672475636,
5.5530342639069));
#81278=CARTESIAN_POINT('Ctrl Pts',(2.90230304443695,-222.815185095966,5.3942763986751));
#81279=CARTESIAN_POINT('Ctrl Pts',(3.40971671127761,-226.253240230551,5.23551853344331));
#81280=CARTESIAN_POINT('Ctrl Pts',(0.796557778040768,-228.54432995542,5.07676066821151));
#81281=CARTESIAN_POINT('Ctrl Pts',(-2.31872921781764,-227.656321352104,
4.92878000800459));
#81282=CARTESIAN_POINT('Ctrl Pts',(-3.06700087458563,-225.810253712066,
4.83371863620826));
#81283=CARTESIAN_POINT('Ctrl Pts',(-3.07449021712595,-224.997267710685,
4.79157655282253));
#81284=CARTESIAN_POINT('Origin',(0.,-225.,22.2084234471774));
#81285=CARTESIAN_POINT('',(-3.07464802069915,-225.002709732222,6.79157655282253));
#81286=CARTESIAN_POINT('',(-3.07288410079718,-224.997201521015,6.70842344717745));
#81287=CARTESIAN_POINT('',(-3.0735,-225.,22.2084234471774));
#81288=CARTESIAN_POINT('Ctrl Pts',(-3.07288410079718,-224.997201521015,
6.70842344717745));
#81289=CARTESIAN_POINT('Ctrl Pts',(-3.07522873674104,-224.735817594879,
6.69489241136339));
#81290=CARTESIAN_POINT('Ctrl Pts',(-2.92508990676295,-223.454826085153,
6.62844208713874));
#81291=CARTESIAN_POINT('Ctrl Pts',(-1.13665725625273,-221.549668149031,
6.50907247450349));
#81292=CARTESIAN_POINT('Ctrl Pts',(2.2821711173499,-222.173611033291,6.35031460927169));
#81293=CARTESIAN_POINT('Ctrl Pts',(3.61235657409808,-225.384264988738,6.19155674403991));
#81294=CARTESIAN_POINT('Ctrl Pts',(1.63651343628419,-228.243239641602,6.03279887880811));
#81295=CARTESIAN_POINT('Ctrl Pts',(-1.83706673406269,-228.13400150201,5.87404101357632));
#81296=CARTESIAN_POINT('Ctrl Pts',(-3.05774544236497,-226.106133206661,
5.76591586969943));
#81297=CARTESIAN_POINT('Ctrl Pts',(-3.0785190087078,-225.044773836104,5.71071001423314));
#81298=CARTESIAN_POINT('Ctrl Pts',(-3.0783646865402,-225.000807299621,5.70842344717745));
#81299=CARTESIAN_POINT('Ctrl Pts',(-3.07464802069915,-225.002709732222,
6.79157655282254));
#81300=CARTESIAN_POINT('Ctrl Pts',(-3.06713149317871,-224.184616738264,
6.74916414205817));
#81301=CARTESIAN_POINT('Ctrl Pts',(-2.31086287355762,-222.333491153698,
6.65383244288321));
#81302=CARTESIAN_POINT('Ctrl Pts',(0.814607672933798,-221.459774941358,
6.50558145529765));
#81303=CARTESIAN_POINT('Ctrl Pts',(3.41605836726569,-223.76415034973,6.34682359006585));
#81304=CARTESIAN_POINT('Ctrl Pts',(2.89113257820927,-227.19957530943,6.18806572483406));
#81305=CARTESIAN_POINT('Ctrl Pts',(-0.279757632733263,-228.621949032436,
6.02930785960227));
#81306=CARTESIAN_POINT('Ctrl Pts',(-2.70632267198121,-227.046531976909,
5.89714480226509));
#81307=CARTESIAN_POINT('Ctrl Pts',(-3.06860828362547,-225.510376344323,
5.81790103333851));
#81308=CARTESIAN_POINT('Ctrl Pts',(-3.06854459837578,-225.000042997605,
5.79157655282253));
#81309=CARTESIAN_POINT('Origin',(0.,-225.,22.2084234471774));
#81310=CARTESIAN_POINT('',(-3.07736989982489,-224.998253130058,7.79157655282253));
#81311=CARTESIAN_POINT('',(-3.06879157690567,-225.000903264851,7.70842344717744));
#81312=CARTESIAN_POINT('',(-3.0735,-225.,22.2084234471774));
#81313=CARTESIAN_POINT('Ctrl Pts',(-3.06879157690567,-225.000903264851,
7.70842344717744));
#81314=CARTESIAN_POINT('Ctrl Pts',(-3.06729326924488,-224.432057018653,
7.67907480849364));
#81315=CARTESIAN_POINT('Ctrl Pts',(-2.64281778869516,-222.835431117709,
7.59680688139924));
#81316=CARTESIAN_POINT('Ctrl Pts',(-0.0729493032098818,-221.367995319502,
7.46161966589424));
#81317=CARTESIAN_POINT('Ctrl Pts',(3.01175337487511,-222.968714395038,7.30286180066245));
#81318=CARTESIAN_POINT('Ctrl Pts',(3.34009948270872,-226.428465976356,7.14410393543066));
#81319=CARTESIAN_POINT('Ctrl Pts',(0.611586675313532,-228.580885552287,
6.98534607019887));
#81320=CARTESIAN_POINT('Ctrl Pts',(-2.39639166901593,-227.551946819569,
6.84011924078113));
#81321=CARTESIAN_POINT('Ctrl Pts',(-3.06605896825943,-225.758078681403,
6.74781169977399));
#81322=CARTESIAN_POINT('Ctrl Pts',(-3.07288410079718,-224.997201521015,
6.70842344717745));
#81323=CARTESIAN_POINT('Ctrl Pts',(-3.07736989982489,-224.998253130058,
7.79157655282253));
#81324=CARTESIAN_POINT('Ctrl Pts',(-3.07806429383697,-224.896050021069,
7.78626582759902));
#81325=CARTESIAN_POINT('Ctrl Pts',(-3.02707595981422,-223.776134342622,
7.7280358139649));
#81326=CARTESIAN_POINT('Ctrl Pts',(-1.655528769796,-221.766425566186,7.6168865119202));
#81327=CARTESIAN_POINT('Ctrl Pts',(1.81863287894903,-221.855265738056,7.4581286466884));
#81328=CARTESIAN_POINT('Ctrl Pts',(3.62838178839593,-224.822166582794,7.29937078145661));
#81329=CARTESIAN_POINT('Ctrl Pts',(2.11743582778552,-227.951820563965,7.14061291622481));
#81330=CARTESIAN_POINT('Ctrl Pts',(-1.33138731914806,-228.379968481073,
6.98185505099303));
#81331=CARTESIAN_POINT('Ctrl Pts',(-2.96588670322775,-226.426781465541,
6.8655095965256));
#81332=CARTESIAN_POINT('Ctrl Pts',(-3.07651009912286,-225.205376895815,
6.80208343046877));
#81333=CARTESIAN_POINT('Ctrl Pts',(-3.07464802069915,-225.002709732222,
6.79157655282254));
#81334=CARTESIAN_POINT('Origin',(0.,-225.,22.2084234471774));
#81335=CARTESIAN_POINT('',(-3.06937338025089,-224.998402365976,8.79157655282253));
#81336=CARTESIAN_POINT('',(-3.07619355237033,-225.002319527513,8.70842344717744));
#81337=CARTESIAN_POINT('',(-3.0735,-225.,22.2084234471774));
#81338=CARTESIAN_POINT('Ctrl Pts',(-3.07619355237033,-225.002319527513,
8.70842344717744));
#81339=CARTESIAN_POINT('Ctrl Pts',(-3.06888768878592,-224.132240268067,
8.66325720562389));
#81340=CARTESIAN_POINT('Ctrl Pts',(-2.22821896698895,-222.230378726602,
8.56517167565974));
#81341=CARTESIAN_POINT('Ctrl Pts',(0.997195673100731,-221.506809425532,
8.414166857285));
#81342=CARTESIAN_POINT('Ctrl Pts',(3.47557947438652,-223.943057751236,8.2554089920532));
#81343=CARTESIAN_POINT('Ctrl Pts',(2.7731130773876,-227.346619581445,8.09665112682141));
#81344=CARTESIAN_POINT('Ctrl Pts',(-0.467306298986418,-228.602555262994,
7.93789326158962));
#81345=CARTESIAN_POINT('Ctrl Pts',(-2.76007204034179,-226.938762943595,
7.80848403504163));
#81346=CARTESIAN_POINT('Ctrl Pts',(-3.06999490648549,-225.457758377008,
7.73199409690424));
#81347=CARTESIAN_POINT('Ctrl Pts',(-3.06879157690567,-225.000903264851,
7.70842344717744));
#81348=CARTESIAN_POINT('Ctrl Pts',(-3.06937338025089,-224.998402365975,
8.79157655282253));
#81349=CARTESIAN_POINT('Ctrl Pts',(-3.07130231416634,-224.589079310054,
8.77044822472927));
#81350=CARTESIAN_POINT('Ctrl Pts',(-2.8045902474645,-223.156952286025,8.6964006082254));
#81351=CARTESIAN_POINT('Ctrl Pts',(-0.632602276895449,-221.422767342497,
8.56943370331095));
#81352=CARTESIAN_POINT('Ctrl Pts',(2.6621824992875,-222.528246883865,8.41067583807915));
#81353=CARTESIAN_POINT('Ctrl Pts',(3.52053795681035,-225.89587477992,8.25191797284737));
#81354=CARTESIAN_POINT('Ctrl Pts',(1.15689721470216,-228.443598112622,8.09316010761557));
#81355=CARTESIAN_POINT('Ctrl Pts',(-2.15104950765063,-227.859940666864,
7.93971296760729));
#81356=CARTESIAN_POINT('Ctrl Pts',(-3.07114493057695,-225.914463810798,
7.83918511600961));
#81357=CARTESIAN_POINT('Ctrl Pts',(-3.07736989982489,-224.998253130058,
7.79157655282253));
#81358=CARTESIAN_POINT('Origin',(0.,-225.,22.2084234471774));
#81359=CARTESIAN_POINT('',(-3.0715437315608,-225.002615101916,9.79157655282254));
#81360=CARTESIAN_POINT('',(-3.07602729093121,-224.997622070323,9.70842344717745));
#81361=CARTESIAN_POINT('',(-3.0735,-225.,22.2084234471774));
#81362=CARTESIAN_POINT('Ctrl Pts',(-3.07602729093122,-224.997622070323,
9.70842344717744));
#81363=CARTESIAN_POINT('Ctrl Pts',(-3.0773539235959,-224.842245191388,9.70035889116474));
#81364=CARTESIAN_POINT('Ctrl Pts',(-2.99601734532136,-223.668684684651,
9.63937504674144));
#81365=CARTESIAN_POINT('Ctrl Pts',(-1.48552430373511,-221.684883540053,
9.52547191390755));
#81366=CARTESIAN_POINT('Ctrl Pts',(1.97934842100312,-221.953861554645,9.36671404867575));
#81367=CARTESIAN_POINT('Ctrl Pts',(3.63272154867527,-225.010665354639,9.20795618344396));
#81368=CARTESIAN_POINT('Ctrl Pts',(1.96142805785311,-228.057708222487,9.04919831821216));
#81369=CARTESIAN_POINT('Ctrl Pts',(-1.50496431438492,-228.306336645357,
8.89044045298038));
#81370=CARTESIAN_POINT('Ctrl Pts',(-2.99968382218232,-226.319150005193,
8.77684882930213));
#81371=CARTESIAN_POINT('Ctrl Pts',(-3.07744764615261,-225.151673669807,
8.71617649403449));
#81372=CARTESIAN_POINT('Ctrl Pts',(-3.07619355237033,-225.002319527513,
8.70842344717744));
#81373=CARTESIAN_POINT('Ctrl Pts',(-3.0715437315608,-225.002615101916,9.79157655282254));
#81374=CARTESIAN_POINT('Ctrl Pts',(-3.0657613572303,-224.288126470754,9.75463062185952));
#81375=CARTESIAN_POINT('Ctrl Pts',(-2.4615581954256,-222.541426343529,9.66476540248591));
#81376=CARTESIAN_POINT('Ctrl Pts',(0.446144839320715,-221.394762988514,
9.5219808947017));
#81377=CARTESIAN_POINT('Ctrl Pts',(3.27082198427282,-223.419334736943,9.36322302946992));
#81378=CARTESIAN_POINT('Ctrl Pts',(3.1020429778404,-226.890531271963,9.20446516423812));
#81379=CARTESIAN_POINT('Ctrl Pts',(0.0942743600733127,-228.631513661226,
9.04570729900632));
#81380=CARTESIAN_POINT('Ctrl Pts',(-2.58800196981665,-227.259552761042,
8.9080777618678));
#81381=CARTESIAN_POINT('Ctrl Pts',(-3.06647098961733,-225.614294592295,
8.82336751313987));
#81382=CARTESIAN_POINT('Ctrl Pts',(-3.06937338025089,-224.998402365975,
8.79157655282253));
#81383=CARTESIAN_POINT('Origin',(0.,-225.,22.2084234471774));
#81384=CARTESIAN_POINT('',(-3.0786228608021,-225.000055941039,10.7915765528225));
#81385=CARTESIAN_POINT('',(-3.06874135342515,-224.999191262945,10.7084234471775));
#81386=CARTESIAN_POINT('',(-3.0735,-225.,22.2084234471774));
#81387=CARTESIAN_POINT('Ctrl Pts',(-3.06874135342515,-224.999191262945,
10.7084234471774));
#81388=CARTESIAN_POINT('Ctrl Pts',(-3.06983198124641,-224.536279450012,
10.684541288295));
#81389=CARTESIAN_POINT('Ctrl Pts',(-2.75418296187546,-223.049036499641,
10.607739841002));
#81390=CARTESIAN_POINT('Ctrl Pts',(-0.446144847322243,-221.394762923856,
10.4780191052983));
#81391=CARTESIAN_POINT('Ctrl Pts',(2.78684409501469,-222.669703969432,10.3192612400665));
#81392=CARTESIAN_POINT('Ctrl Pts',(3.46931343118415,-226.077331850548,10.1605033748347));
#81393=CARTESIAN_POINT('Ctrl Pts',(0.976667251561304,-228.498985664407,
10.0017455096029));
#81394=CARTESIAN_POINT('Ctrl Pts',(-2.23779829231897,-227.758021627206,
9.85105220038384));
#81395=CARTESIAN_POINT('Ctrl Pts',(-3.06864861403061,-225.861821948715,
9.75327817957534));
#81396=CARTESIAN_POINT('Ctrl Pts',(-3.07602729093122,-224.997622070323,
9.70842344717744));
#81397=CARTESIAN_POINT('Ctrl Pts',(-3.07862236853609,-225.000055935664,
10.7915765528225));
#81398=CARTESIAN_POINT('Ctrl Pts',(-3.07835031097462,-223.985736843864,
10.7388130189898));
#81399=CARTESIAN_POINT('Ctrl Pts',(-1.97594905925326,-221.953597719633,
10.6331301967464));
#81400=CARTESIAN_POINT('Ctrl Pts',(1.48552427709262,-221.684883599509,10.4745280860925));
#81401=CARTESIAN_POINT('Ctrl Pts',(3.59084517971103,-224.449899989107,10.3157702208607));
#81402=CARTESIAN_POINT('Ctrl Pts',(2.40982471506444,-227.718367887042,10.1570123556289));
#81403=CARTESIAN_POINT('Ctrl Pts',(-0.97666723404505,-228.498985601654,
9.99825449039707));
#81404=CARTESIAN_POINT('Ctrl Pts',(-2.88922789173994,-226.640896054566,
9.8764425561283));
#81405=CARTESIAN_POINT('Ctrl Pts',(-3.07404370732726,-225.311520088211,
9.80754991027012));
#81406=CARTESIAN_POINT('Ctrl Pts',(-3.0715437315608,-225.002615101916,9.79157655282254));
#81407=CARTESIAN_POINT('Origin',(0.,-225.,22.2084234471774));
#81408=CARTESIAN_POINT('',(-3.07170674492633,-224.997349498083,11.7915765528225));
#81409=CARTESIAN_POINT('',(-3.07306312169136,-225.002805832536,11.7084234471775));
#81410=CARTESIAN_POINT('',(-3.0735,-225.,22.2084234471774));
#81411=CARTESIAN_POINT('Ctrl Pts',(-3.07306312169136,-225.002805832536,
11.7084234471775));
#81412=CARTESIAN_POINT('Ctrl Pts',(-3.06613162486477,-224.236024983951,
11.6687236854253));
#81413=CARTESIAN_POINT('Ctrl Pts',(-2.38783081082145,-222.436195233095,
11.5761046352625));
#81414=CARTESIAN_POINT('Ctrl Pts',(0.632602288240958,-221.42276727834,11.430566296689));
#81415=CARTESIAN_POINT('Ctrl Pts',(3.34842953419328,-223.591170963338,11.2718084314573));
#81416=CARTESIAN_POINT('Ctrl Pts',(2.99977420212569,-227.048934927288,11.1130505662255));
#81417=CARTESIAN_POINT('Ctrl Pts',(-0.0942743617640601,-228.631513726356,
10.9542927009937));
#81418=CARTESIAN_POINT('Ctrl Pts',(-2.64958035268347,-227.152429629564,
10.8194169946443));
#81419=CARTESIAN_POINT('Ctrl Pts',(-3.06741531328495,-225.562022719616,
10.7374605767056));
#81420=CARTESIAN_POINT('Ctrl Pts',(-3.06874135342515,-224.999191262945,
10.7084234471774));
#81421=CARTESIAN_POINT('Ctrl Pts',(-3.07170674492633,-224.997349498083,
11.7915765528225));
#81422=CARTESIAN_POINT('Ctrl Pts',(-3.07420079038922,-224.694509382875,
11.7759147045306));
#81423=CARTESIAN_POINT('Ctrl Pts',(-2.89395005922289,-223.371316808894,
11.7073335678281));
#81424=CARTESIAN_POINT('Ctrl Pts',(-0.997195655216347,-221.506809488182,
11.585833142715));
#81425=CARTESIAN_POINT('Ctrl Pts',(2.39382152606057,-222.267529025221,11.4270752774832));
#81426=CARTESIAN_POINT('Ctrl Pts',(3.5940133408216,-225.529005890927,11.2683174122514));
#81427=CARTESIAN_POINT('Ctrl Pts',(1.50496428739385,-228.306336586058,11.1095595470196));
#81428=CARTESIAN_POINT('Ctrl Pts',(-1.96142802267546,-228.057708167648,
10.9508016817878));
#81429=CARTESIAN_POINT('Ctrl Pts',(-3.07726334016045,-226.023356891522,
10.8448073503888));
#81430=CARTESIAN_POINT('Ctrl Pts',(-3.07862317163262,-225.003050140761,
10.7917323074004));
#81431=CARTESIAN_POINT('Ctrl Pts',(-3.07862236853609,-225.000055935664,
10.7915765528225));
#81432=CARTESIAN_POINT('Origin',(0.,-225.,22.2084234471774));
#81433=CARTESIAN_POINT('',(-3.06928120376705,-225.001514673646,12.7915765528225));
#81434=CARTESIAN_POINT('',(-3.07829286865601,-224.999087154577,12.7084234471774));
#81435=CARTESIAN_POINT('',(-3.0735,-225.,22.2084234471774));
#81436=CARTESIAN_POINT('Ctrl Pts',(-3.07829286865601,-224.999087154577,
12.7084234471774));
#81437=CARTESIAN_POINT('Ctrl Pts',(-3.07848862305667,-224.949127749583,
12.7058253709661));
#81438=CARTESIAN_POINT('Ctrl Pts',(-3.05474879031452,-223.881753016838,
12.6503080063441));
#81439=CARTESIAN_POINT('Ctrl Pts',(-1.81863291156572,-221.855265681656,
12.5418713533116));
#81440=CARTESIAN_POINT('Ctrl Pts',(1.65552879948739,-221.766425508193,12.3831134880798));
#81441=CARTESIAN_POINT('Ctrl Pts',(3.61455061835174,-224.636952582474,12.224355622848));
#81442=CARTESIAN_POINT('Ctrl Pts',(2.26553585343932,-227.839740638999,12.0655977576162));
#81443=CARTESIAN_POINT('Ctrl Pts',(-1.15689723545072,-228.443598174382,
11.9068398923844));
#81444=CARTESIAN_POINT('Ctrl Pts',(-2.92947454176964,-226.532970860394,
11.7877817889048));
#81445=CARTESIAN_POINT('Ctrl Pts',(-3.07537122388234,-225.258134313656,
11.7216429738359));
#81446=CARTESIAN_POINT('Ctrl Pts',(-3.07306312169136,-225.002805832536,
11.7084234471775));
#81447=CARTESIAN_POINT('Ctrl Pts',(-3.06928120376705,-225.001514673646,
12.7915765528225));
#81448=CARTESIAN_POINT('Ctrl Pts',(-3.06656132439523,-224.391611531572,
12.7600971016609));
#81449=CARTESIAN_POINT('Ctrl Pts',(-2.59517224566867,-222.752541482839,
12.6756983620886));
#81450=CARTESIAN_POINT('Ctrl Pts',(0.0729493019015324,-221.367995384641,
12.5383803341057));
#81451=CARTESIAN_POINT('Ctrl Pts',(3.09088872643165,-223.091286818965,12.379622468874));
#81452=CARTESIAN_POINT('Ctrl Pts',(3.28004691007777,-226.561432481514,12.2208646036422));
#81453=CARTESIAN_POINT('Ctrl Pts',(0.467306290605433,-228.602555198383,
12.0621067384104));
#81454=CARTESIAN_POINT('Ctrl Pts',(-2.45343780595167,-227.470520636967,
11.9190107214705));
#81455=CARTESIAN_POINT('Ctrl Pts',(-3.06577374469831,-225.717765584843,
11.8288339929412));
#81456=CARTESIAN_POINT('Ctrl Pts',(-3.07170674492633,-224.997349498083,
11.7915765528225));
#81457=CARTESIAN_POINT('Origin',(0.,-225.,22.2084234471774));
#81458=CARTESIAN_POINT('',(-3.07723488309734,-225.001830508734,13.7915765528225));
#81459=CARTESIAN_POINT('',(-3.07037718038997,-224.997773372826,13.7084234471775));
#81460=CARTESIAN_POINT('',(-3.0735,-225.,22.2084234471774));
#81461=CARTESIAN_POINT('Ctrl Pts',(-3.07037718038997,-224.997773372826,
13.7084234471775));
#81462=CARTESIAN_POINT('Ctrl Pts',(-3.07276832859184,-224.641295536,13.6900077680964));
#81463=CARTESIAN_POINT('Ctrl Pts',(-2.8506726448042,-223.26332934368,13.6186728006047));
#81464=CARTESIAN_POINT('Ctrl Pts',(-0.814607687543583,-221.459774877865,
13.4944185447024));
#81465=CARTESIAN_POINT('Ctrl Pts',(2.53237197705076,-222.395413320727,13.3356606794706));
#81466=CARTESIAN_POINT('Ctrl Pts',(3.56172490783136,-225.714769390036,13.1769028142388));
#81467=CARTESIAN_POINT('Ctrl Pts',(1.33138734302612,-228.379968541692,13.018144949007));
#81468=CARTESIAN_POINT('Ctrl Pts',(-2.06099579255385,-227.958827267799,
12.8619851599865));
#81469=CARTESIAN_POINT('Ctrl Pts',(-3.07450137143537,-225.966733064678,
12.7587446593767));
#81470=CARTESIAN_POINT('Ctrl Pts',(-3.07829286865601,-224.999087154577,
12.7084234471774));
#81471=CARTESIAN_POINT('Ctrl Pts',(-3.07723488309734,-225.001830508734,
13.7915765528225));
#81472=CARTESIAN_POINT('Ctrl Pts',(-3.07081808206618,-224.091509657493,
13.7442794987911));
#81473=CARTESIAN_POINT('Ctrl Pts',(-2.16109704934214,-222.151514836552,
13.6440631563491));
#81474=CARTESIAN_POINT('Ctrl Pts',(1.13665723586709,-221.549668210912,13.4909275254965));
#81475=CARTESIAN_POINT('Ctrl Pts',(3.51521689058642,-224.083468855535,13.3321696602647));
#81476=CARTESIAN_POINT('Ctrl Pts',(2.67665018527361,-227.45607876753,13.1734117950329));
#81477=CARTESIAN_POINT('Ctrl Pts',(-0.611586664344894,-228.580885488065,
13.0146539298011));
#81478=CARTESIAN_POINT('Ctrl Pts',(-2.79907372937866,-226.855260463285,
12.887375515731));
#81479=CARTESIAN_POINT('Ctrl Pts',(-3.07113364302239,-225.416903875844,
12.8130163900715));
#81480=CARTESIAN_POINT('Ctrl Pts',(-3.06928120376705,-225.001514673646,
12.7915765528225));
#81481=CARTESIAN_POINT('Origin',(0.,-225.,22.2084234471774));
#81482=CARTESIAN_POINT('',(-3.07482911963311,-224.997319814409,14.7915765528225));
#81483=CARTESIAN_POINT('',(-3.07026207039166,-225.002172427921,14.7084234471775));
#81484=CARTESIAN_POINT('',(-3.0735,-225.,22.2084234471774));
#81485=CARTESIAN_POINT('Ctrl Pts',(-3.07026207039166,-225.002172427921,
14.7084234471775));
#81486=CARTESIAN_POINT('Ctrl Pts',(-3.06593576340553,-224.339446029993,
14.6741901652266));
#81487=CARTESIAN_POINT('Ctrl Pts',(-2.52994311745615,-222.645870254276,
14.5870375948652));
#81488=CARTESIAN_POINT('Ctrl Pts',(0.261298259228322,-221.376672410653,
14.4469657360931));
#81489=CARTESIAN_POINT('Ctrl Pts',(3.18575945837514,-223.254229031811,14.2882078708613));
#81490=CARTESIAN_POINT('Ctrl Pts',(3.19461372649398,-226.729515174404,14.1294500056295));
#81491=CARTESIAN_POINT('Ctrl Pts',(0.279757637750653,-228.621949097395,
13.9706921403977));
#81492=CARTESIAN_POINT('Ctrl Pts',(-2.52331401844028,-227.364568613608,
13.830349954247));
#81493=CARTESIAN_POINT('Ctrl Pts',(-3.06589712602745,-225.665670112463,
13.7429270565069));
#81494=CARTESIAN_POINT('Ctrl Pts',(-3.07037718038997,-224.997773372826,
13.7084234471775));
#81495=CARTESIAN_POINT('Ctrl Pts',(-3.07482911963311,-224.997319814409,
14.7915765528225));
#81496=CARTESIAN_POINT('Ctrl Pts',(-3.07662798453365,-224.800691183691,
14.781381184332));
#81497=CARTESIAN_POINT('Ctrl Pts',(-2.96986780631845,-223.58540298435,14.7182665274308));
#81498=CARTESIAN_POINT('Ctrl Pts',(-1.35121078347837,-221.627907393731,
14.6022325821191));
#81499=CARTESIAN_POINT('Ctrl Pts',(2.10006689756961,-222.035797214701,14.4434747168873));
#81500=CARTESIAN_POINT('Ctrl Pts',(3.62936343654465,-225.156525308212,14.2847168516555));
#81501=CARTESIAN_POINT('Ctrl Pts',(1.83706670111546,-228.134001445802,14.1259589864237));
#81502=CARTESIAN_POINT('Ctrl Pts',(-1.6365134069338,-228.243239583436,13.9672011211919));
#81503=CARTESIAN_POINT('Ctrl Pts',(-3.02371444213389,-226.236009089191,
13.8557403099915));
#81504=CARTESIAN_POINT('Ctrl Pts',(-3.07799765278989,-225.110040994371,
13.7971987872017));
#81505=CARTESIAN_POINT('Ctrl Pts',(-3.07723488309734,-225.001830508734,
13.7915765528225));
#81506=CARTESIAN_POINT('Origin',(0.,-225.,22.2084234471774));
#81507=CARTESIAN_POINT('',(-3.06855000713338,-224.999857959883,15.7915765528225));
#81508=CARTESIAN_POINT('',(-3.07822420567057,-225.001003127123,15.7084234471775));
#81509=CARTESIAN_POINT('',(-3.0735,-225.,22.2084234471774));
#81510=CARTESIAN_POINT('Ctrl Pts',(-3.07822420567056,-225.001003127123,
15.7084234471775));
#81511=CARTESIAN_POINT('Ctrl Pts',(-3.07412463871347,-224.038498199653,
15.6583725623569));
#81512=CARTESIAN_POINT('Ctrl Pts',(-2.07017708091493,-222.050954058745,
15.5554023891257));
#81513=CARTESIAN_POINT('Ctrl Pts',(1.31414733087609,-221.613291215241,15.3995129274839));
#81514=CARTESIAN_POINT('Ctrl Pts',(3.55803654033007,-224.267091016787,15.2407550622521));
#81515=CARTESIAN_POINT('Ctrl Pts',(2.54561084798977,-227.591649090945,15.0819971970203));
#81516=CARTESIAN_POINT('Ctrl Pts',(-0.796557792326769,-228.544330018986,
14.9232393317885));
#81517=CARTESIAN_POINT('Ctrl Pts',(-2.8462359772097,-226.747272607382,14.7987147485075));
#81518=CARTESIAN_POINT('Ctrl Pts',(-3.07262355593096,-225.363917170084,
14.7271094536372));
#81519=CARTESIAN_POINT('Ctrl Pts',(-3.07026207039166,-225.002172427921,
14.7084234471775));
#81520=CARTESIAN_POINT('Ctrl Pts',(-3.06855000713338,-224.999857959883,
15.7915765528225));
#81521=CARTESIAN_POINT('Ctrl Pts',(-3.06875791854356,-224.495565829248,
15.7655635814622));
#81522=CARTESIAN_POINT('Ctrl Pts',(-2.71259526698658,-222.96564743543,15.6866313216913));
#81523=CARTESIAN_POINT('Ctrl Pts',(-0.301020081620057,-221.379756080425,
15.5547797735098));
#81524=CARTESIAN_POINT('Ctrl Pts',(2.87816732548634,-222.783486527642,15.396021908278));
#81525=CARTESIAN_POINT('Ctrl Pts',(3.42325610946395,-226.21577001757,15.2372640430462));
#81526=CARTESIAN_POINT('Ctrl Pts',(0.835381036688694,-228.535380835242,
15.0785061778144));
#81527=CARTESIAN_POINT('Ctrl Pts',(-2.30174388869721,-227.678234462693,
14.9299436810732));
#81528=CARTESIAN_POINT('Ctrl Pts',(-3.0672909359933,-225.82129649368,14.8343004727426));
#81529=CARTESIAN_POINT('Ctrl Pts',(-3.07482911963311,-224.997319814409,
14.7915765528225));
#81530=CARTESIAN_POINT('Origin',(0.,-225.,22.2084234471774));
#81531=CARTESIAN_POINT('',(-3.07430784425243,-225.002754717764,16.7915765528225));
#81532=CARTESIAN_POINT('',(-3.07321943364514,-224.997190820081,16.7084234471775));
#81533=CARTESIAN_POINT('',(-3.0735,-225.,22.2084234471774));
#81534=CARTESIAN_POINT('Ctrl Pts',(-3.07321943364514,-224.997190820081,
16.7084234471775));
#81535=CARTESIAN_POINT('Ctrl Pts',(-3.07549307656515,-224.747116023829,
16.6954742478977));
#81536=CARTESIAN_POINT('Ctrl Pts',(-2.93324524011334,-223.477617636429,
16.6296057602074));
#81537=CARTESIAN_POINT('Ctrl Pts',(-1.17442917055295,-221.562341535168,
16.5108179841064));
#81538=CARTESIAN_POINT('Ctrl Pts',(2.25103646081656,-222.148752123552,16.3520601188746));
#81539=CARTESIAN_POINT('Ctrl Pts',(3.61635361185226,-225.344624656961,16.1933022536428));
#81540=CARTESIAN_POINT('Ctrl Pts',(1.67198407948828,-228.225096717565,16.034544388411));
#81541=CARTESIAN_POINT('Ctrl Pts',(-1.80258521665346,-228.153960389228,
15.8757865231792));
#81542=CARTESIAN_POINT('Ctrl Pts',(-3.05211835267063,-226.128761858828,
15.767079542768));
#81543=CARTESIAN_POINT('Ctrl Pts',(-3.07845915081927,-225.056164041845,
15.7112918507675));
#81544=CARTESIAN_POINT('Ctrl Pts',(-3.07822420567056,-225.001003127123,
15.7084234471775));
#81545=CARTESIAN_POINT('Ctrl Pts',(-3.07430784425243,-225.002754717764,
16.7915765528225));
#81546=CARTESIAN_POINT('Ctrl Pts',(-3.06685916030357,-224.195655169849,
16.7497459785925));
#81547=CARTESIAN_POINT('Ctrl Pts',(-2.32773976850131,-222.355431708145,
16.6549961159518));
#81548=CARTESIAN_POINT('Ctrl Pts',(0.775732535354965,-221.451053935833,
16.5073269649006));
#81549=CARTESIAN_POINT('Ctrl Pts',(3.40229918628707,-223.726760283541,16.3485690996688));
#81550=CARTESIAN_POINT('Ctrl Pts',(2.91508175397509,-227.167735567766,16.189811234437));
#81551=CARTESIAN_POINT('Ctrl Pts',(-0.240018384082209,-228.62479934656,
16.0310533692052));
#81552=CARTESIAN_POINT('Ctrl Pts',(-2.69447347406282,-227.069271455095,
15.8983084753337));
#81553=CARTESIAN_POINT('Ctrl Pts',(-3.06833495556379,-225.521468650369,
15.8184828698728));
#81554=CARTESIAN_POINT('Ctrl Pts',(-3.06855000713338,-224.999857959883,
15.7915765528225));
#81555=CARTESIAN_POINT('Origin',(0.,-225.,22.2084234471774));
#81556=CARTESIAN_POINT('',(-3.07760789837034,-224.998416752929,17.7915765528225));
#81557=CARTESIAN_POINT('',(-3.06870231121375,-225.000725933415,17.7084234471775));
#81558=CARTESIAN_POINT('',(-3.0735,-225.,22.2084234471774));
#81559=CARTESIAN_POINT('Ctrl Pts',(-3.06870231121375,-225.000725933415,
17.7084234471775));
#81560=CARTESIAN_POINT('Ctrl Pts',(-3.06752400629039,-224.443116559207,
17.679656645028));
#81561=CARTESIAN_POINT('Ctrl Pts',(-2.65540737602782,-222.858108746021,
17.5979705544679));
#81562=CARTESIAN_POINT('Ctrl Pts',(-0.112777617954695,-221.369013821348,
17.4633651754972));
#81563=CARTESIAN_POINT('Ctrl Pts',(2.98929484919384,-222.935806224066,17.3046073102654));
#81564=CARTESIAN_POINT('Ctrl Pts',(3.35556479392172,-226.39174873303,17.1458494450336));
#81565=CARTESIAN_POINT('Ctrl Pts',(0.650821968247489,-228.573962834745,
16.9870915798018));
#81566=CARTESIAN_POINT('Ctrl Pts',(-2.3803556336648,-227.574084984456,16.8412829138497));
#81567=CARTESIAN_POINT('Ctrl Pts',(-3.0662014159128,-225.769092748505,16.7483935363083));
#81568=CARTESIAN_POINT('Ctrl Pts',(-3.07321943364514,-224.997190820081,
16.7084234471775));
#81569=CARTESIAN_POINT('Ctrl Pts',(-3.07760789837034,-224.998416752929,
17.7915765528225));
#81570=CARTESIAN_POINT('Ctrl Pts',(-3.07817910364606,-224.907429428249,
17.7868476641333));
#81571=CARTESIAN_POINT('Ctrl Pts',(-3.03325250153319,-223.79880775355,17.7291994870335));
#81572=CARTESIAN_POINT('Ctrl Pts',(-1.69089212962583,-221.784776606531,
17.6186320215231));
#81573=CARTESIAN_POINT('Ctrl Pts',(1.78403469350766,-221.835509587289,17.4598741562913));
#81574=CARTESIAN_POINT('Ctrl Pts',(3.6262132841795,-224.782384342542,17.3011162910595));
#81575=CARTESIAN_POINT('Ctrl Pts',(2.14968149722227,-227.928420804412,17.1423584258278));
#81576=CARTESIAN_POINT('Ctrl Pts',(-1.29423865111908,-228.394366727483,
16.9836005605959));
#81577=CARTESIAN_POINT('Ctrl Pts',(-2.9583412850881,-226.44954541655,16.8666732695942));
#81578=CARTESIAN_POINT('Ctrl Pts',(-3.07628238868196,-225.216705789839,
16.8026652670031));
#81579=CARTESIAN_POINT('Ctrl Pts',(-3.07430784425243,-225.002754717764,
16.7915765528225));
#81580=CARTESIAN_POINT('Origin',(0.,-225.,22.2084234471774));
#81581=CARTESIAN_POINT('',(-3.06955372481635,-224.998258419941,18.7915765528225));
#81582=CARTESIAN_POINT('',(-3.07588044059715,-225.00242799355,18.7084234471775));
#81583=CARTESIAN_POINT('',(-3.0735,-225.,22.2084234471774));
#81584=CARTESIAN_POINT('Ctrl Pts',(-3.07588044059715,-225.00242799355,18.7084234471775));
#81585=CARTESIAN_POINT('Ctrl Pts',(-3.06844940786727,-224.143330357591,
18.6638390421582));
#81586=CARTESIAN_POINT('Ctrl Pts',(-2.24606371110549,-222.252055139543,
18.5663353487284));
#81587=CARTESIAN_POINT('Ctrl Pts',(0.958825626738842,-221.496084849927,
18.4159123668879));
#81588=CARTESIAN_POINT('Ctrl Pts',(3.4637786989553,-223.905003298803,18.2571545016562));
#81589=CARTESIAN_POINT('Ctrl Pts',(2.79868206393424,-227.316065751486,18.0983966364243));
#81590=CARTESIAN_POINT('Ctrl Pts',(-0.427768493644222,-228.607463409909,
17.9396387711926));
#81591=CARTESIAN_POINT('Ctrl Pts',(-2.74903327485336,-226.961549419753,
17.8096477081102));
#81592=CARTESIAN_POINT('Ctrl Pts',(-3.06969161107839,-225.468892421981,
17.7325759334385));
#81593=CARTESIAN_POINT('Ctrl Pts',(-3.06870231121375,-225.000725933415,
17.7084234471775));
#81594=CARTESIAN_POINT('Ctrl Pts',(-3.06955372481635,-224.998258419941,
18.7915765528225));
#81595=CARTESIAN_POINT('Ctrl Pts',(-3.07161652142556,-224.600263410142,
18.7710300612636));
#81596=CARTESIAN_POINT('Ctrl Pts',(-2.81478286658869,-223.1797504858,18.697564281294));
#81597=CARTESIAN_POINT('Ctrl Pts',(-0.671786414007324,-221.429931110442,
18.5711792129139));
#81598=CARTESIAN_POINT('Ctrl Pts',(2.63490948932574,-222.499193694183,18.4124213476821));
#81599=CARTESIAN_POINT('Ctrl Pts',(3.53015379637291,-225.857213283498,18.2536634824503));
#81600=CARTESIAN_POINT('Ctrl Pts',(1.19459288842475,-228.430701869046,18.0949056172185));
#81601=CARTESIAN_POINT('Ctrl Pts',(-2.13212074104536,-227.881284704446,
17.9408766406759));
#81602=CARTESIAN_POINT('Ctrl Pts',(-3.07178695134263,-225.925635775,17.8397669525439));
#81603=CARTESIAN_POINT('Ctrl Pts',(-3.07760789837034,-224.998416752929,
17.7915765528225));
#81604=CARTESIAN_POINT('Origin',(0.,-225.,22.2084234471774));
#81605=CARTESIAN_POINT('',(-3.07038308399263,-225.003292812227,19.7915765528225));
#81606=CARTESIAN_POINT('',(-3.0763285686357,-224.997783098605,19.7084234471775));
#81607=CARTESIAN_POINT('',(-3.0735,-225.,22.2084234471774));
#81608=CARTESIAN_POINT('',(-0.793799282532889,-227.969222953746,20.));
#81609=CARTESIAN_POINT('Ctrl Pts',(-0.793799282532874,-227.969222953746,
20.));
#81610=CARTESIAN_POINT('Ctrl Pts',(-1.78107094869727,-227.70528334649,19.9470807115894));
#81611=CARTESIAN_POINT('Ctrl Pts',(-2.87946808286553,-226.663720267333,
19.8776062291969));
#81612=CARTESIAN_POINT('Ctrl Pts',(-3.07279570905048,-225.323526622123,
19.8081317468044));
#81613=CARTESIAN_POINT('Ctrl Pts',(-3.07038308399263,-225.003292812227,
19.7915765528225));
#81614=CARTESIAN_POINT('',(0.795577412305969,-227.974522386933,20.));
#81615=CARTESIAN_POINT('Origin',(0.,-225.,20.));
#81616=CARTESIAN_POINT('Ctrl Pts',(0.795579146452471,-227.974527555281,
20.));
#81617=CARTESIAN_POINT('Ctrl Pts',(-0.166093705500148,-228.23015226012,
19.948244384658));
#81618=CARTESIAN_POINT('Ctrl Pts',(-2.23002419682037,-227.756253006398,
19.8510522003838));
#81619=CARTESIAN_POINT('Ctrl Pts',(-3.06912206206202,-225.872782873122,
19.7538600161097));
#81620=CARTESIAN_POINT('Ctrl Pts',(-3.0763285686357,-224.997783098605,19.7084234471775));
#81621=CARTESIAN_POINT('Origin',(0.,-225.,22.2084234471774));
#81622=CARTESIAN_POINT('Ctrl Pts',(-3.0763285686357,-224.997783098605,19.7084234471775));
#81623=CARTESIAN_POINT('Ctrl Pts',(-3.07751537187321,-224.85368379687,19.7009407276991));
#81624=CARTESIAN_POINT('Ctrl Pts',(-3.00279426336461,-223.69169114993,19.6405387198101));
#81625=CARTESIAN_POINT('Ctrl Pts',(-1.52182615633225,-221.701128865433,
19.5272174235105));
#81626=CARTESIAN_POINT('Ctrl Pts',(1.94583861817437,-221.932458083289,19.3684595582787));
#81627=CARTESIAN_POINT('Ctrl Pts',(3.63261183657197,-224.970764508319,19.2097016930469));
#81628=CARTESIAN_POINT('Ctrl Pts',(1.99484845140044,-228.036042436051,19.0509438278151));
#81629=CARTESIAN_POINT('Ctrl Pts',(-1.46861473543692,-228.322628496388,
18.8921859625833));
#81630=CARTESIAN_POINT('Ctrl Pts',(-2.9928033600919,-226.341875538283,18.7780125023707));
#81631=CARTESIAN_POINT('Ctrl Pts',(-3.07726964364369,-225.163032999144,
18.7167583305688));
#81632=CARTESIAN_POINT('Ctrl Pts',(-3.07588044059715,-225.00242799355,18.7084234471775));
#81633=CARTESIAN_POINT('Ctrl Pts',(-3.07038308399263,-225.003292812227,
19.7915765528225));
#81634=CARTESIAN_POINT('Ctrl Pts',(-3.06508366403289,-224.299887432922,
19.7552124583938));
#81635=CARTESIAN_POINT('Ctrl Pts',(-2.47776214952136,-222.562456695511,
19.6659290755545));
#81636=CARTESIAN_POINT('Ctrl Pts',(0.40726891511089,-221.390844838622,19.5237264043046));
#81637=CARTESIAN_POINT('Ctrl Pts',(3.25295021883841,-223.383185295634,19.3649685390728));
#81638=CARTESIAN_POINT('Ctrl Pts',(3.12275738725604,-226.856580639298,19.206210673841));
#81639=CARTESIAN_POINT('Ctrl Pts',(0.1340136609786,-228.63017093477,19.0474528086092));
#81640=CARTESIAN_POINT('Ctrl Pts',(-2.57444325081393,-227.28215157222,18.9092414349364));
#81641=CARTESIAN_POINT('Ctrl Pts',(-3.06630360810496,-225.625334413095,
18.8239493496742));
#81642=CARTESIAN_POINT('Ctrl Pts',(-3.06955372481635,-224.998258419941,
18.7915765528225));
#81643=CARTESIAN_POINT('Ctrl Pts',(1.91346599666507,-223.364012796625,20.));
#81644=CARTESIAN_POINT('Ctrl Pts',(2.45743451545281,-224.000243484622,19.9470807115894));
#81645=CARTESIAN_POINT('Ctrl Pts',(2.85075800802285,-225.847693925911,19.8412421347682));
#81646=CARTESIAN_POINT('Ctrl Pts',(0.831598049327248,-227.85876780774,19.6824842695364));
#81647=CARTESIAN_POINT('Ctrl Pts',(-1.94946036222679,-227.24729402904,19.5237264043046));
#81648=CARTESIAN_POINT('Ctrl Pts',(-2.94596530464746,-224.582107318842,
19.3649685390728));
#81649=CARTESIAN_POINT('Ctrl Pts',(-1.24652589834599,-222.297898785986,
19.206210673841));
#81650=CARTESIAN_POINT('Ctrl Pts',(1.59383397470441,-222.487380258559,19.0474528086093));
#81651=CARTESIAN_POINT('Ctrl Pts',(2.97546780496825,-224.976053245386,18.8886949433774));
#81652=CARTESIAN_POINT('Ctrl Pts',(1.63397786770802,-227.48681855629,18.7299370781457));
#81653=CARTESIAN_POINT('Ctrl Pts',(-1.20294049014559,-227.721560839322,
18.5711792129139));
#81654=CARTESIAN_POINT('Ctrl Pts',(-2.93892187964717,-225.46557347867,18.4124213476821));
#81655=CARTESIAN_POINT('Ctrl Pts',(-1.9852049751549,-222.783472249891,18.2536634824503));
#81656=CARTESIAN_POINT('Ctrl Pts',(0.785372869795044,-222.129947489732,
18.0949056172185));
#81657=CARTESIAN_POINT('Ctrl Pts',(2.83717679343419,-224.10308957369,17.9361477519867));
#81658=CARTESIAN_POINT('Ctrl Pts',(2.29239697281744,-226.897086555837,17.7773898867549));
#81659=CARTESIAN_POINT('Ctrl Pts',(-0.350384637302541,-227.954868760191,
17.6186320215231));
#81660=CARTESIAN_POINT('Ctrl Pts',(-2.67249415737608,-226.308355800229,
17.4598741562913));
#81661=CARTESIAN_POINT('Ctrl Pts',(-2.54873717095616,-223.464435363585,
17.3011162910595));
#81662=CARTESIAN_POINT('Ctrl Pts',(-0.0923760055965229,-222.025863769398,
17.1423584258277));
#81663=CARTESIAN_POINT('Ctrl Pts',(2.44852766645372,-223.309221463831,16.9836005605959));
#81664=CARTESIAN_POINT('Ctrl Pts',(2.74853891937463,-226.13997964386,16.8248426953642));
#81665=CARTESIAN_POINT('Ctrl Pts',(0.533087458943556,-227.927428481038,
16.6660848301323));
#81666=CARTESIAN_POINT('Ctrl Pts',(-2.170245621756,-227.035694896164,16.5073269649006));
#81667=CARTESIAN_POINT('Ctrl Pts',(-2.88736999535495,-224.280893418101,
16.3485690996688));
#81668=CARTESIAN_POINT('Ctrl Pts',(-0.961973462458767,-222.184218257617,
16.189811234437));
#81669=CARTESIAN_POINT('Ctrl Pts',(1.84382114530851,-222.664546435999,16.0310533692052));
#81670=CARTESIAN_POINT('Ctrl Pts',(2.96215071346611,-225.282281624825,15.8722955039734));
#81671=CARTESIAN_POINT('Ctrl Pts',(1.36952006510874,-227.641672681461,15.7135376387416));
#81672=CARTESIAN_POINT('Ctrl Pts',(-1.47649529296408,-227.583405004029,
15.5547797735098));
#81673=CARTESIAN_POINT('Ctrl Pts',(-2.9712222169863,-225.160805168439,15.396021908278));
#81674=CARTESIAN_POINT('Ctrl Pts',(-1.74668668485902,-222.591036449047,
15.2372640430462));
#81675=CARTESIAN_POINT('Ctrl Pts',(1.07641643256242,-222.225951076743,15.0785061778144));
#81676=CARTESIAN_POINT('Ctrl Pts',(2.91438327323278,-224.399675169924,14.9197483125827));
#81677=CARTESIAN_POINT('Ctrl Pts',(2.08510665684536,-227.12281652398,14.7609904473508));
#81678=CARTESIAN_POINT('Ctrl Pts',(-0.652459489891874,-227.903156278769,
14.6022325821191));
#81679=CARTESIAN_POINT('Ctrl Pts',(-2.79289473713753,-226.026527521392,
14.4434747168873));
#81680=CARTESIAN_POINT('Ctrl Pts',(-2.37727283078277,-223.210420816804,
14.2847168516555));
#81681=CARTESIAN_POINT('Ctrl Pts',(0.214029076820345,-222.032136910304,
14.1259589864237));
#81682=CARTESIAN_POINT('Ctrl Pts',(2.60945158173399,-223.570041186785,13.9672011211919));
#81683=CARTESIAN_POINT('Ctrl Pts',(2.61670410165888,-226.416643712889,13.8084432559601));
#81684=CARTESIAN_POINT('Ctrl Pts',(0.229149130644944,-227.966733968665,
13.6496853907283));
#81685=CARTESIAN_POINT('Ctrl Pts',(-2.36812311572418,-226.801669412983,
13.4909275254965));
#81686=CARTESIAN_POINT('Ctrl Pts',(-2.7980891797067,-223.987717081388,13.3321696602647));
#81687=CARTESIAN_POINT('Ctrl Pts',(-0.66724413645386,-222.1002060371,13.1734117950329));
#81688=CARTESIAN_POINT('Ctrl Pts',(2.07426271424282,-222.866586313626,13.0146539298011));
#81689=CARTESIAN_POINT('Ctrl Pts',(2.91740441043288,-225.585466712028,12.8558960645693));
#81690=CARTESIAN_POINT('Ctrl Pts',(1.0905377049189,-227.768527998604,12.6971381993376));
#81691=CARTESIAN_POINT('Ctrl Pts',(-1.7343890652525,-227.417832569728,12.5383803341058));
#81692=CARTESIAN_POINT('Ctrl Pts',(-2.972003031108,-224.854336868116,12.379622468874));
#81693=CARTESIAN_POINT('Ctrl Pts',(-1.48963993976465,-222.424152059076,
12.2208646036422));
#81694=CARTESIAN_POINT('Ctrl Pts',(1.35604156587263,-222.351383184277,12.0621067384104));
#81695=CARTESIAN_POINT('Ctrl Pts',(2.96067388374833,-224.702628315074,11.9033488731786));
#81696=CARTESIAN_POINT('Ctrl Pts',(1.85569757964323,-227.326028000221,11.7445910079468));
#81697=CARTESIAN_POINT('Ctrl Pts',(-0.947613076377819,-227.820646951035,
11.585833142715));
#81698=CARTESIAN_POINT('Ctrl Pts',(-2.88366828216186,-225.733809923181,
11.4270752774832));
#81699=CARTESIAN_POINT('Ctrl Pts',(-2.18059038950889,-222.975390082488,
11.2683174122514));
#81700=CARTESIAN_POINT('Ctrl Pts',(0.518163741872992,-222.069893158686,
11.1095595470196));
#81701=CARTESIAN_POINT('Ctrl Pts',(2.74269443706901,-223.846029900831,10.9508016817878));
#81702=CARTESIAN_POINT('Ctrl Pts',(2.4571112913133,-226.678280032356,10.792043816556));
#81703=CARTESIAN_POINT('Ctrl Pts',(-0.0772200116287812,-227.974568344266,
10.6332859513242));
#81704=CARTESIAN_POINT('Ctrl Pts',(-2.54087956296479,-226.548531824475,
10.4745280860925));
#81705=CARTESIAN_POINT('Ctrl Pts',(-2.67912623819311,-223.70527903982,10.3157702208607));
#81706=CARTESIAN_POINT('Ctrl Pts',(-0.365436685581164,-222.046954827007,
10.1570123556289));
#81707=CARTESIAN_POINT('Ctrl Pts',(2.28270050730421,-223.091257440392,9.99825449039708));
#81708=CARTESIAN_POINT('Ctrl Pts',(2.84171028566979,-225.882441169271,9.83949662516528));
#81709=CARTESIAN_POINT('Ctrl Pts',(0.799986922337905,-227.866014774734,
9.6807387599335));
#81710=CARTESIAN_POINT('Ctrl Pts',(-1.97388444085889,-227.226611771064,
9.5219808947017));
#81711=CARTESIAN_POINT('Ctrl Pts',(-2.94125684140276,-224.549413762076,
9.36322302946991));
#81712=CARTESIAN_POINT('Ctrl Pts',(-1.21679109635696,-222.284592260317,
9.20446516423812));
#81713=CARTESIAN_POINT('Ctrl Pts',(1.6212818122256,-222.504911815135,9.04570729900632));
#81714=CARTESIAN_POINT('Ctrl Pts',(2.97555767001464,-225.008735978625,8.88694943377453));
#81715=CARTESIAN_POINT('Ctrl Pts',(1.60660326521724,-227.504564974821,8.72819156854273));
#81716=CARTESIAN_POINT('Ctrl Pts',(-1.23271438472883,-227.70821620455,8.56943370331095));
#81717=CARTESIAN_POINT('Ctrl Pts',(-2.94385187824639,-225.433308070373,
8.41067583807916));
#81718=CARTESIAN_POINT('Ctrl Pts',(-1.96077624855704,-222.76183640723,8.25191797284736));
#81719=CARTESIAN_POINT('Ctrl Pts',(0.816801726706074,-222.138731976176,
8.09316010761557));
#81720=CARTESIAN_POINT('Ctrl Pts',(2.84684279380774,-224.134259928009,7.93440224238378));
#81721=CARTESIAN_POINT('Ctrl Pts',(2.27145344796592,-226.922113159684,7.77564437715198));
#81722=CARTESIAN_POINT('Ctrl Pts',(-0.382770004131556,-227.950848503201,
7.61688651192019));
#81723=CARTESIAN_POINT('Ctrl Pts',(-2.6866823634999,-226.278967412628,7.4581286466884));
#81724=CARTESIAN_POINT('Ctrl Pts',(-2.53174312944437,-223.436575396312,
7.29937078145661));
#81725=CARTESIAN_POINT('Ctrl Pts',(-0.0597526828797273,-222.025029515811,
7.14061291622481));
#81726=CARTESIAN_POINT('Ctrl Pts',(2.46692341670672,-223.336176505452,6.98185505099303));
#81727=CARTESIAN_POINT('Ctrl Pts',(2.73587130233258,-226.170054691875,6.82309718576122));
#81728=CARTESIAN_POINT('Ctrl Pts',(0.500949879649189,-227.933098870305,
6.66433932052944));
#81729=CARTESIAN_POINT('Ctrl Pts',(-2.19244085318975,-227.011771077973,
6.50558145529764));
#81730=CARTESIAN_POINT('Ctrl Pts',(-2.8793098034051,-224.249270474191,6.34682359006586));
#81731=CARTESIAN_POINT('Ctrl Pts',(-0.9310345347702,-222.173837502908,6.18806572483406));
#81732=CARTESIAN_POINT('Ctrl Pts',(1.86932350347434,-222.684908337827,6.02930785960227));
#81733=CARTESIAN_POINT('Ctrl Pts',(2.95887674484852,-225.314750970928,5.87054999437047));
#81734=CARTESIAN_POINT('Ctrl Pts',(1.34046610569235,-227.656533527813,5.71179212913868));
#81735=CARTESIAN_POINT('Ctrl Pts',(-1.50473906068093,-227.56705670451,5.55303426390689));
#81736=CARTESIAN_POINT('Ctrl Pts',(-2.97280709789139,-225.128209686185,
5.3942763986751));
#81737=CARTESIAN_POINT('Ctrl Pts',(-1.72016219601459,-222.572025168107,
5.2355185334433));
#81738=CARTESIAN_POINT('Ctrl Pts',(1.10677508001132,-222.237923120698,5.07676066821152));
#81739=CARTESIAN_POINT('Ctrl Pts',(2.92079184633315,-224.431673724612,4.91800280297971));
#81740=CARTESIAN_POINT('Ctrl Pts',(2.06170002974943,-227.14555651341,4.75924493774793));
#81741=CARTESIAN_POINT('Ctrl Pts',(-0.684259572989003,-227.89582606551,
4.60048707251613));
#81742=CARTESIAN_POINT('Ctrl Pts',(-2.80398484143082,-225.995835716326,
4.44172920728434));
#81743=CARTESIAN_POINT('Ctrl Pts',(-2.35750329326922,-223.184456558731,
4.28297134205255));
#81744=CARTESIAN_POINT('Ctrl Pts',(0.246565176206193,-222.034662687169,
4.12421347682075));
#81745=CARTESIAN_POINT('Ctrl Pts',(2.62497720607225,-223.598745407746,3.96545561158896));
#81746=CARTESIAN_POINT('Ctrl Pts',(2.60101020024974,-226.445256275959,3.80669774635717));
#81747=CARTESIAN_POINT('Ctrl Pts',(0.196598761270279,-227.969068657434,
3.64793988112538));
#81748=CARTESIAN_POINT('Ctrl Pts',(-2.38773985594611,-226.775589520002,
3.48918201589359));
#81749=CARTESIAN_POINT('Ctrl Pts',(-2.78681905160012,-223.957090924459,
3.33042415066179));
#81750=CARTESIAN_POINT('Ctrl Pts',(-0.635401559389043,-222.093062672271,
3.17166628543));
#81751=CARTESIAN_POINT('Ctrl Pts',(2.09753541208473,-222.889463351295,3.01290842019821));
#81752=CARTESIAN_POINT('Ctrl Pts',(2.91080806279928,-225.617427081746,2.85415055496642));
#81753=CARTESIAN_POINT('Ctrl Pts',(1.06010927692769,-227.780321584409,2.69539268973463));
#81754=CARTESIAN_POINT('Ctrl Pts',(-1.76080145317522,-227.398665855655,
2.53663482450284));
#81755=CARTESIAN_POINT('Ctrl Pts',(-2.97022681197801,-224.821751284356,
2.37787695927104));
#81756=CARTESIAN_POINT('Ctrl Pts',(-1.46130060892094,-222.407969820474,
2.21911909403925));
#81757=CARTESIAN_POINT('Ctrl Pts',(1.38500765016929,-222.366414498639,2.06036122880746));
#81758=CARTESIAN_POINT('Ctrl Pts',(2.96375737617749,-224.735116069809,1.90160336357566));
#81759=CARTESIAN_POINT('Ctrl Pts',(1.83007562745225,-227.346240326103,1.74284549834387));
#81760=CARTESIAN_POINT('Ctrl Pts',(-0.978489556298073,-227.810083654364,
1.58408763311208));
#81761=CARTESIAN_POINT('Ctrl Pts',(-2.89154460401165,-225.702142338414,
1.42532976788028));
#81762=CARTESIAN_POINT('Ctrl Pts',(-2.15825110157835,-222.951592652511,
1.2665719026485));
#81763=CARTESIAN_POINT('Ctrl Pts',(0.550259421404619,-222.075760988886,
1.1078140374167));
#81764=CARTESIAN_POINT('Ctrl Pts',(2.75520159224266,-223.876160869976,0.94905617218491));
#81765=CARTESIAN_POINT('Ctrl Pts',(2.43852437670019,-226.705163033173,0.790298306953122));
#81766=CARTESIAN_POINT('Ctrl Pts',(-0.109770429300331,-227.973468539745,
0.631540441721324));
#81767=CARTESIAN_POINT('Ctrl Pts',(-2.55784670274268,-226.520722864724,
0.472782576489534));
#81768=CARTESIAN_POINT('Ctrl Pts',(-2.66448750437358,-223.675669147007,
0.314024711257742));
#81769=CARTESIAN_POINT('Ctrl Pts',(-0.333593465451435,-222.043745349829,
0.155266846025945));
#81770=CARTESIAN_POINT('Ctrl Pts',(2.30464631571321,-223.1151355344,-0.0034910192058416));
#81771=CARTESIAN_POINT('Ctrl Pts',(2.82948425040376,-225.916201445671,-0.162248884437639));
#81772=CARTESIAN_POINT('Ctrl Pts',(1.45887298303089,-227.215894200354,-0.268087461258832));
#81773=CARTESIAN_POINT('Ctrl Pts',(0.65019999797512,-227.432086802035,-0.32100674966943));
#81774=CARTESIAN_POINT('Ctrl Pts',(2.0543315503421,-223.243574678773,20.1070022498898));
#81775=CARTESIAN_POINT('Ctrl Pts',(2.63834594750733,-223.926643402192,20.0540829614792));
#81776=CARTESIAN_POINT('Ctrl Pts',(3.06062513181772,-225.910099463522,19.948244384658));
#81777=CARTESIAN_POINT('Ctrl Pts',(0.892818640578617,-228.069224597028,
19.7894865194262));
#81778=CARTESIAN_POINT('Ctrl Pts',(-2.09297574936987,-227.412735337235,
19.6307286541944));
#81779=CARTESIAN_POINT('Ctrl Pts',(-3.16284139989857,-224.551342892398,
19.4719707889626));
#81780=CARTESIAN_POINT('Ctrl Pts',(-1.33829265100808,-222.098975479135,
19.3132129237308));
#81781=CARTESIAN_POINT('Ctrl Pts',(1.71116885586107,-222.302406200136,19.1544550584991));
#81782=CARTESIAN_POINT('Ctrl Pts',(3.19451581550283,-224.97429033303,18.9956971932673));
#81783=CARTESIAN_POINT('Ctrl Pts',(1.75426806227216,-227.669893182877,18.8369393280355));
#81784=CARTESIAN_POINT('Ctrl Pts',(-1.29149857190937,-227.921916725011,
18.6781814628037));
#81785=CARTESIAN_POINT('Ctrl Pts',(-3.15527945198531,-225.499848070413,
18.5194235975719));
#81786=CARTESIAN_POINT('Ctrl Pts',(-2.13135180947283,-222.620295893842,
18.3606657323401));
#81787=CARTESIAN_POINT('Ctrl Pts',(0.843190455442978,-221.91865994313,18.2019078671083));
#81788=CARTESIAN_POINT('Ctrl Pts',(3.04604409527456,-224.037060815394,18.0431500018765));
#81789=CARTESIAN_POINT('Ctrl Pts',(2.46115866985638,-227.03674628772,17.8843921366447));
#81790=CARTESIAN_POINT('Ctrl Pts',(-0.376179256083103,-228.172400310097,
17.7256342714129));
#81791=CARTESIAN_POINT('Ctrl Pts',(-2.86923785171585,-226.404674347058,
17.5668764061811));
#81792=CARTESIAN_POINT('Ctrl Pts',(-2.73637012256843,-223.351390154999,
17.4081185409494));
#81793=CARTESIAN_POINT('Ctrl Pts',(-0.0991765430492469,-221.806913786715,
17.2493606757175));
#81794=CARTESIAN_POINT('Ctrl Pts',(2.62878339403376,-223.184749717243,17.0906028104857));
#81795=CARTESIAN_POINT('Ctrl Pts',(2.95088087755699,-226.223902673583,16.931844945254));
#81796=CARTESIAN_POINT('Ctrl Pts',(0.5723322953782,-228.142939932274,16.7730870800222));
#81797=CARTESIAN_POINT('Ctrl Pts',(-2.33001477974293,-227.185558697854,
16.6143292147904));
#81798=CARTESIAN_POINT('Ctrl Pts',(-3.09993242069985,-224.227954224518,
16.4555713495586));
#81799=CARTESIAN_POINT('Ctrl Pts',(-1.0327920318235,-221.9769260168,16.2968134843268));
#81800=CARTESIAN_POINT('Ctrl Pts',(1.97955958381119,-222.492614998516,16.138055619095));
#81801=CARTESIAN_POINT('Ctrl Pts',(3.18021834626149,-225.303062635537,15.9792977538632));
#81802=CARTESIAN_POINT('Ctrl Pts',(1.47034140323525,-227.836147360162,15.8205398886314));
#81803=CARTESIAN_POINT('Ctrl Pts',(-1.58519193419387,-227.773590132429,
15.6617820233996));
#81804=CARTESIAN_POINT('Ctrl Pts',(-3.1899576757939,-225.1726433245,15.5030241581678));
#81805=CARTESIAN_POINT('Ctrl Pts',(-1.87527427794497,-222.41369335281,15.344266292936));
#81806=CARTESIAN_POINT('Ctrl Pts',(1.15566006533364,-222.021731122909,15.1855084277043));
#81807=CARTESIAN_POINT('Ctrl Pts',(3.12893436226521,-224.355480452212,15.0267505624724));
#81808=CARTESIAN_POINT('Ctrl Pts',(2.23860805389349,-227.279094046301,14.8679926972407));
#81809=CARTESIAN_POINT('Ctrl Pts',(-0.700492257370171,-228.116880858842,
14.7092348320089));
#81810=CARTESIAN_POINT('Ctrl Pts',(-2.99850208223497,-226.102098431937,
14.5504769667771));
#81811=CARTESIAN_POINT('Ctrl Pts',(-2.55228291935149,-223.078675563464,
14.3917191015453));
#81812=CARTESIAN_POINT('Ctrl Pts',(0.229785470956337,-221.813648743753,
14.2329612363135));
#81813=CARTESIAN_POINT('Ctrl Pts',(2.80155420728104,-223.46477046846,14.0742033710817));
#81814=CARTESIAN_POINT('Ctrl Pts',(2.80934064327058,-226.520934200061,13.9154455058499));
#81815=CARTESIAN_POINT('Ctrl Pts',(0.246018633013514,-228.185139011575,
13.7566876406181));
#81816=CARTESIAN_POINT('Ctrl Pts',(-2.54245962050307,-226.934304724948,
13.5979297753863));
#81817=CARTESIAN_POINT('Ctrl Pts',(-3.00407892931503,-223.913194830113,
13.4391719101545));
#81818=CARTESIAN_POINT('Ctrl Pts',(-0.716365320150435,-221.886728984022,
13.2804140449227));
#81819=CARTESIAN_POINT('Ctrl Pts',(2.22696580184547,-222.709528649326,13.1216561796909));
#81820=CARTESIAN_POINT('Ctrl Pts',(3.1321779095657,-225.628567604697,12.9628983144592));
#81821=CARTESIAN_POINT('Ctrl Pts',(1.17082091762131,-227.972341512967,12.8041404492274));
#81822=CARTESIAN_POINT('Ctrl Pts',(-1.8620713320887,-227.595828585454,12.6453825839956));
#81823=CARTESIAN_POINT('Ctrl Pts',(-3.19079597189529,-224.843613438612,
12.4866247187638));
#81824=CARTESIAN_POINT('Ctrl Pts',(-1.59930426369834,-222.234523266603,
12.327866853532));
#81825=CARTESIAN_POINT('Ctrl Pts',(1.45587064374422,-222.156397292249,12.1691089883002));
#81826=CARTESIAN_POINT('Ctrl Pts',(3.1786327952828,-224.680736404207,12.0103511230684));
#81827=CARTESIAN_POINT('Ctrl Pts',(1.99231033757526,-227.49726554648,11.8515932578366));
#81828=CARTESIAN_POINT('Ctrl Pts',(-1.01737446273545,-228.028297358817,
11.6928353926048));
#81829=CARTESIAN_POINT('Ctrl Pts',(-3.09595819475795,-225.78783154745,11.534077527373));
#81830=CARTESIAN_POINT('Ctrl Pts',(-2.3411211086836,-222.826342334837,11.3753196621412));
#81831=CARTESIAN_POINT('Ctrl Pts',(0.556309923995647,-221.854184531904,
11.2165617969094));
#81832=CARTESIAN_POINT('Ctrl Pts',(2.94460613611043,-223.761076921667,11.0578039316776));
#81833=CARTESIAN_POINT('Ctrl Pts',(2.63799892825076,-226.801831664,10.8990460664458));
#81834=CARTESIAN_POINT('Ctrl Pts',(-0.0829047950072066,-228.193550138296,
10.7402882012141));
#81835=CARTESIAN_POINT('Ctrl Pts',(-2.72793405313473,-226.662531651607,
10.5815303359823));
#81836=CARTESIAN_POINT('Ctrl Pts',(-2.87635817310677,-223.609964262744,
10.4227724707505));
#81837=CARTESIAN_POINT('Ctrl Pts',(-0.392339406161525,-221.829557525957,
10.2640146055187));
#81838=CARTESIAN_POINT('Ctrl Pts',(2.45074836987437,-222.950739616739,10.1052567402869));
#81839=CARTESIAN_POINT('Ctrl Pts',(3.05091133417458,-225.947404729696,9.9464988750551));
#81840=CARTESIAN_POINT('Ctrl Pts',(0.858880365412371,-228.077005071292,
9.7877410098233));
#81841=CARTESIAN_POINT('Ctrl Pts',(-2.11919788000057,-227.390530492641,
9.62898314459151));
#81842=CARTESIAN_POINT('Ctrl Pts',(-3.15778630897244,-224.516242501131,
9.47022527935972));
#81843=CARTESIAN_POINT('Ctrl Pts',(-1.30636883214967,-222.084689353562,
9.31146741412793));
#81844=CARTESIAN_POINT('Ctrl Pts',(1.74063734848477,-222.321228394972,9.15270954889614));
#81845=CARTESIAN_POINT('Ctrl Pts',(3.19461229623485,-225.009379103963,8.99395168366434));
#81846=CARTESIAN_POINT('Ctrl Pts',(1.72487819609586,-227.688946057376,8.83519381843254));
#81847=CARTESIAN_POINT('Ctrl Pts',(-1.32346436128086,-227.907589684819,
8.67643595320076));
#81848=CARTESIAN_POINT('Ctrl Pts',(-3.16057238725731,-225.465207347053,
8.51767808796896));
#81849=CARTESIAN_POINT('Ctrl Pts',(-2.10512468870239,-222.597067263559,
8.35892022273717));
#81850=CARTESIAN_POINT('Ctrl Pts',(0.87693304217096,-221.928091125962,8.20016235750538));
#81851=CARTESIAN_POINT('Ctrl Pts',(3.05642168733399,-224.070525869085,8.04140449227358));
#81852=CARTESIAN_POINT('Ctrl Pts',(2.43867332443981,-227.063615300271,7.88264662704179));
#81853=CARTESIAN_POINT('Ctrl Pts',(-0.410948769083177,-228.168084089798,
7.72388876181));
#81854=CARTESIAN_POINT('Ctrl Pts',(-2.88447056530141,-226.373122444925,
7.56513089657821));
#81855=CARTESIAN_POINT('Ctrl Pts',(-2.71812501358486,-223.321479192452,
7.40637303134642));
#81856=CARTESIAN_POINT('Ctrl Pts',(-0.0641515563231119,-221.806018117041,
7.24761516611463));
#81857=CARTESIAN_POINT('Ctrl Pts',(2.64853340276285,-223.213689135314,7.08885730088283));
#81858=CARTESIAN_POINT('Ctrl Pts',(2.93728069579129,-226.256191786702,6.93009943565104));
#81859=CARTESIAN_POINT('Ctrl Pts',(0.537828811537304,-228.149027764299,
6.77134157041925));
#81860=CARTESIAN_POINT('Ctrl Pts',(-2.35384397988601,-227.159873655842,
6.61258370518746));
#81861=CARTESIAN_POINT('Ctrl Pts',(-3.09127885348033,-224.194003262493,
6.45382583995566));
#81862=CARTESIAN_POINT('Ctrl Pts',(-0.999575441931042,-221.965781051616,
6.29506797472387));
#81863=CARTESIAN_POINT('Ctrl Pts',(2.0069393747662,-222.514475902981,6.13631010949208));
#81864=CARTESIAN_POINT('Ctrl Pts',(3.17670335459837,-225.337922310198,5.97755224426028));
#81865=CARTESIAN_POINT('Ctrl Pts',(1.43914854922296,-227.85210223241,5.81879437902849));
#81866=CARTESIAN_POINT('Ctrl Pts',(-1.61551495180818,-227.756038303676,
5.6600365137967));
#81867=CARTESIAN_POINT('Ctrl Pts',(-3.191659232473,-225.137648227797,5.50127864856491));
#81868=CARTESIAN_POINT('Ctrl Pts',(-1.84679710908763,-222.393282499251,
5.34252078333311));
#81869=CARTESIAN_POINT('Ctrl Pts',(1.18825365591152,-222.034584524883,5.18376291810132));
#81870=CARTESIAN_POINT('Ctrl Pts',(3.13581472174675,-224.389834676731,5.02500505286953));
#81871=CARTESIAN_POINT('Ctrl Pts',(2.21347827755356,-227.303508108439,4.86624718763774));
#81872=CARTESIAN_POINT('Ctrl Pts',(-0.734633399216325,-228.109011009889,
4.70748932240595));
#81873=CARTESIAN_POINT('Ctrl Pts',(-3.0104086179069,-226.069147157342,4.54873145717415));
#81874=CARTESIAN_POINT('Ctrl Pts',(-2.53105798788129,-223.05079986845,4.38997359194236));
#81875=CARTESIAN_POINT('Ctrl Pts',(0.264716813143711,-221.816360463278,
4.23121572671057));
#81876=CARTESIAN_POINT('Ctrl Pts',(2.81822279714489,-223.495587836969,4.07245786147878));
#81877=CARTESIAN_POINT('Ctrl Pts',(2.79249138811321,-226.551653163007,3.91369999624698));
#81878=CARTESIAN_POINT('Ctrl Pts',(0.21107197030918,-228.18764557548,3.75494213101519));
#81879=CARTESIAN_POINT('Ctrl Pts',(-2.56352050604952,-226.906304882216,
3.5961842657834));
#81880=CARTESIAN_POINT('Ctrl Pts',(-2.99197911683543,-223.880314036541,
3.43742640055161));
#81881=CARTESIAN_POINT('Ctrl Pts',(-0.682178556015369,-221.879059738909,
3.27866853531981));
#81882=CARTESIAN_POINT('Ctrl Pts',(2.25195178932658,-222.734089848921,3.11991067008802));
#81883=CARTESIAN_POINT('Ctrl Pts',(3.12509595196398,-225.662880833146,2.96115280485623));
#81884=CARTESIAN_POINT('Ctrl Pts',(1.13815240939665,-227.985003319058,2.80239493962443));
#81885=CARTESIAN_POINT('Ctrl Pts',(-1.89042814737785,-227.575250856085,
2.64363707439265));
#81886=CARTESIAN_POINT('Ctrl Pts',(-3.18888899105247,-224.80862896911,2.48487920916085));
#81887=CARTESIAN_POINT('Ctrl Pts',(-1.5688786477902,-222.217149723842,2.32612134392906));
#81888=CARTESIAN_POINT('Ctrl Pts',(1.48696915344557,-222.172535182021,2.16736347869727));
#81889=CARTESIAN_POINT('Ctrl Pts',(3.18194328828006,-224.715615842707,2.00860561346548));
#81890=CARTESIAN_POINT('Ctrl Pts',(1.96480214832129,-227.518965863516,1.84984774823368));
#81891=CARTESIAN_POINT('Ctrl Pts',(-1.05052400757933,-228.016956413295,
1.69108988300189));
#81892=CARTESIAN_POINT('Ctrl Pts',(-3.10441435572704,-225.753832658197,
1.53233201777009));
#81893=CARTESIAN_POINT('Ctrl Pts',(-2.3171372468915,-222.800792985486,1.37357415253831));
#81894=CARTESIAN_POINT('Ctrl Pts',(0.590768423496762,-221.860484340071,
1.21481628730651));
#81895=CARTESIAN_POINT('Ctrl Pts',(2.95803404312474,-223.793426072718,1.05605842207472));
#81896=CARTESIAN_POINT('Ctrl Pts',(2.61804368202231,-226.830693737766,0.897300556842932));
#81897=CARTESIAN_POINT('Ctrl Pts',(-0.117851509563945,-228.192369368358,
0.738542691611135));
#81898=CARTESIAN_POINT('Ctrl Pts',(-2.74615027993235,-226.632675451654,
0.579784826379343));
#81899=CARTESIAN_POINT('Ctrl Pts',(-2.86064176487431,-223.578174548627,
0.421026961147553));
#81900=CARTESIAN_POINT('Ctrl Pts',(-0.35815195162039,-221.826111773464,
0.262269095915755));
#81901=CARTESIAN_POINT('Ctrl Pts',(2.47430978496665,-222.976375568444,0.103511230683969));
#81902=CARTESIAN_POINT('Ctrl Pts',(3.0377852425553,-225.98365037037,-0.0552466345478286));
#81903=CARTESIAN_POINT('Ctrl Pts',(1.56627230491969,-227.379023915733,-0.161085211369022));
#81904=CARTESIAN_POINT('Ctrl Pts',(0.698066426161045,-227.611132185939,
-0.21400449977962));
#81905=CARTESIAN_POINT('Ctrl Pts',(2.19519710401913,-223.123136560921,20.2140044997796));
#81906=CARTESIAN_POINT('Ctrl Pts',(2.81925737956185,-223.853043319762,20.161085211369));
#81907=CARTESIAN_POINT('Ctrl Pts',(3.27049225561258,-225.972505001132,20.0552466345478));
#81908=CARTESIAN_POINT('Ctrl Pts',(0.95403923182999,-228.279681386317,19.896488769316));
#81909=CARTESIAN_POINT('Ctrl Pts',(-2.23649113651294,-227.57817664543,19.7377309040842));
#81910=CARTESIAN_POINT('Ctrl Pts',(-3.37971749514968,-224.520578465953,
19.5789730388524));
#81911=CARTESIAN_POINT('Ctrl Pts',(-1.43005940367016,-221.900052172284,
19.4202151736207));
#81912=CARTESIAN_POINT('Ctrl Pts',(1.82850373701772,-222.117432141712,19.2614573083889));
#81913=CARTESIAN_POINT('Ctrl Pts',(3.4135638260374,-224.972527420675,19.1026994431571));
#81914=CARTESIAN_POINT('Ctrl Pts',(1.8745582568363,-227.852967809464,18.9439415779253));
#81915=CARTESIAN_POINT('Ctrl Pts',(-1.38005665367314,-228.122272610699,
18.7851837126935));
#81916=CARTESIAN_POINT('Ctrl Pts',(-3.37163702432346,-225.534122662157,
18.6264258474617));
#81917=CARTESIAN_POINT('Ctrl Pts',(-2.27749864379076,-222.457119537793,
18.4676679822299));
#81918=CARTESIAN_POINT('Ctrl Pts',(0.901008041090908,-221.707372396528,
18.3089101169981));
#81919=CARTESIAN_POINT('Ctrl Pts',(3.25491139711493,-223.971032057098,18.1501522517663));
#81920=CARTESIAN_POINT('Ctrl Pts',(2.62992036689531,-227.176406019603,17.9913943865345));
#81921=CARTESIAN_POINT('Ctrl Pts',(-0.401973874863661,-228.389931860003,
17.8326365213027));
#81922=CARTESIAN_POINT('Ctrl Pts',(-3.06598154605562,-226.500992893887,
17.6738786560709));
#81923=CARTESIAN_POINT('Ctrl Pts',(-2.92400307418069,-223.238344946413,
17.5151207908392));
#81924=CARTESIAN_POINT('Ctrl Pts',(-0.105977080501971,-221.587963804031,
17.3563629256074));
#81925=CARTESIAN_POINT('Ctrl Pts',(2.8090391216138,-223.060277970654,17.1976050603756));
#81926=CARTESIAN_POINT('Ctrl Pts',(3.15322283573935,-226.307825703306,17.0388471951438));
#81927=CARTESIAN_POINT('Ctrl Pts',(0.611577131812846,-228.358451383509,
16.880089329912));
#81928=CARTESIAN_POINT('Ctrl Pts',(-2.48978393772987,-227.335422499545,
16.7213314646802));
#81929=CARTESIAN_POINT('Ctrl Pts',(-3.31249484604475,-224.175015030935,
16.5625735994484));
#81930=CARTESIAN_POINT('Ctrl Pts',(-1.10361060118822,-221.769633775984,
16.4038157342166));
#81931=CARTESIAN_POINT('Ctrl Pts',(2.11529802231388,-222.320683561034,16.2450578689848));
#81932=CARTESIAN_POINT('Ctrl Pts',(3.39828597905688,-225.323843646249,16.086300003753));
#81933=CARTESIAN_POINT('Ctrl Pts',(1.57116274136176,-228.030622038864,15.9275421385212));
#81934=CARTESIAN_POINT('Ctrl Pts',(-1.69388857542366,-227.963775260828,
15.7687842732894));
#81935=CARTESIAN_POINT('Ctrl Pts',(-3.4086931346015,-225.184481480561,15.6100264080576));
#81936=CARTESIAN_POINT('Ctrl Pts',(-2.00386187103092,-222.236350256573,
15.4512685428259));
#81937=CARTESIAN_POINT('Ctrl Pts',(1.23490369810486,-221.817511169074,15.2925106775941));
#81938=CARTESIAN_POINT('Ctrl Pts',(3.34348545129764,-224.311285734499,15.1337528123623));
#81939=CARTESIAN_POINT('Ctrl Pts',(2.39210945094163,-227.435371568623,14.9749949471305));
#81940=CARTESIAN_POINT('Ctrl Pts',(-0.748525024848471,-228.330605438914,
14.8162370818987));
#81941=CARTESIAN_POINT('Ctrl Pts',(-3.20410942733242,-226.177669342483,
14.6574792166669));
#81942=CARTESIAN_POINT('Ctrl Pts',(-2.7272930079202,-222.946930310123,14.4987213514351));
#81943=CARTESIAN_POINT('Ctrl Pts',(0.245541865092328,-221.595160577203,
14.3399634862033));
#81944=CARTESIAN_POINT('Ctrl Pts',(2.99365683282809,-223.359499750136,14.1812056209715));
#81945=CARTESIAN_POINT('Ctrl Pts',(3.00197718488228,-226.625224687232,14.0224477557397));
#81946=CARTESIAN_POINT('Ctrl Pts',(0.262888135382085,-228.403544054485,
13.8636898905079));
#81947=CARTESIAN_POINT('Ctrl Pts',(-2.71679612528197,-227.066940036914,
13.7049320252761));
#81948=CARTESIAN_POINT('Ctrl Pts',(-3.21006867892337,-223.83867257884,13.5461741600443));
#81949=CARTESIAN_POINT('Ctrl Pts',(-0.765486503847009,-221.673251930943,
13.3874162948126));
#81950=CARTESIAN_POINT('Ctrl Pts',(2.37966888944811,-222.552470985027,13.2286584295807));
#81951=CARTESIAN_POINT('Ctrl Pts',(3.34695140869854,-225.671668497367,13.069900564349));
#81952=CARTESIAN_POINT('Ctrl Pts',(1.25110413032372,-228.17615502733,12.9111426991172));
#81953=CARTESIAN_POINT('Ctrl Pts',(-1.9897535989249,-227.773824601179,12.7523848338854));
#81954=CARTESIAN_POINT('Ctrl Pts',(-3.40958891268259,-224.832890009108,
12.5936269686536));
#81955=CARTESIAN_POINT('Ctrl Pts',(-1.70896858763203,-222.044894474129,
12.4348691034218));
#81956=CARTESIAN_POINT('Ctrl Pts',(1.5556997216158,-221.961411400221,12.27611123819));
#81957=CARTESIAN_POINT('Ctrl Pts',(3.39659170681727,-224.658844493341,12.1173533729582));
#81958=CARTESIAN_POINT('Ctrl Pts',(2.12892309550729,-227.668503092739,11.9585955077264));
#81959=CARTESIAN_POINT('Ctrl Pts',(-1.08713584909309,-228.2359477666,11.7998376424946));
#81960=CARTESIAN_POINT('Ctrl Pts',(-3.30824810735405,-225.841853171718,
11.6410797772628));
#81961=CARTESIAN_POINT('Ctrl Pts',(-2.5016518278583,-222.677294587186,11.482321912031));
#81962=CARTESIAN_POINT('Ctrl Pts',(0.594456106118301,-221.638475905122,
11.3235640467992));
#81963=CARTESIAN_POINT('Ctrl Pts',(3.14651783515185,-223.676123942502,11.1648061815675));
#81964=CARTESIAN_POINT('Ctrl Pts',(2.81888656518823,-226.925383295644,11.0060483163357));
#81965=CARTESIAN_POINT('Ctrl Pts',(-0.088589578385632,-228.412531932326,
10.8472904511039));
#81966=CARTESIAN_POINT('Ctrl Pts',(-2.91498854330466,-226.776531478738,
10.6885325858721));
#81967=CARTESIAN_POINT('Ctrl Pts',(-3.07359010802042,-223.514649485669,
10.5297747206403));
#81968=CARTESIAN_POINT('Ctrl Pts',(-0.419242126741886,-221.612160224906,
10.3710168554085));
#81969=CARTESIAN_POINT('Ctrl Pts',(2.61879623244453,-222.810221793085,10.2122589901767));
#81970=CARTESIAN_POINT('Ctrl Pts',(3.26011238267936,-226.012368290122,10.0535011249449));
#81971=CARTESIAN_POINT('Ctrl Pts',(0.917773808486839,-228.287995367849,
9.89474325971311));
#81972=CARTESIAN_POINT('Ctrl Pts',(-2.26451131914225,-227.554449214218,
9.73598539448132));
#81973=CARTESIAN_POINT('Ctrl Pts',(-3.37431577654211,-224.483071240186,
9.57722752924952));
#81974=CARTESIAN_POINT('Ctrl Pts',(-1.39594656794239,-221.884786446808,
9.41846966401774));
#81975=CARTESIAN_POINT('Ctrl Pts',(1.85999288474394,-222.137544974808,9.25971179878594));
#81976=CARTESIAN_POINT('Ctrl Pts',(3.41366692245506,-225.010022229301,9.10095393355416));
#81977=CARTESIAN_POINT('Ctrl Pts',(1.84315312697449,-227.873327139932,8.94219606832235));
#81978=CARTESIAN_POINT('Ctrl Pts',(-1.41421433783289,-228.106963165088,
8.78343820309057));
#81979=CARTESIAN_POINT('Ctrl Pts',(-3.37729289626824,-225.497106623734,
8.62468033785877));
#81980=CARTESIAN_POINT('Ctrl Pts',(-2.24947312884774,-222.432298119887,
8.46592247262698));
#81981=CARTESIAN_POINT('Ctrl Pts',(0.937064357635844,-221.717450275747,
8.30716460739519));
#81982=CARTESIAN_POINT('Ctrl Pts',(3.26600058086026,-224.00679181016,8.1484067421634));
#81983=CARTESIAN_POINT('Ctrl Pts',(2.6058932009137,-227.205117440858,7.9896488769316));
#81984=CARTESIAN_POINT('Ctrl Pts',(-0.439127534034797,-228.385319676397,
7.83089101169981));
#81985=CARTESIAN_POINT('Ctrl Pts',(-3.08225876710292,-226.467277477221,
7.67213314646802));
#81986=CARTESIAN_POINT('Ctrl Pts',(-2.90450689772536,-223.206382988593,
7.51337528123622));
#81987=CARTESIAN_POINT('Ctrl Pts',(-0.0685504297664977,-221.587006718271,
7.35461741600443));
#81988=CARTESIAN_POINT('Ctrl Pts',(2.83014338881898,-223.091201765176,7.19585955077264));
#81989=CARTESIAN_POINT('Ctrl Pts',(3.13869008925,-226.342328881529,7.03710168554085));
#81990=CARTESIAN_POINT('Ctrl Pts',(0.574707743425419,-228.364956658293,
6.87834382030906));
#81991=CARTESIAN_POINT('Ctrl Pts',(-2.51524710658227,-227.307976233711,
6.71958595507726));
#81992=CARTESIAN_POINT('Ctrl Pts',(-3.30324790355557,-224.138736050795,
6.56082808984547));
#81993=CARTESIAN_POINT('Ctrl Pts',(-1.06811634909188,-221.757724600324,
6.40207022461368));
#81994=CARTESIAN_POINT('Ctrl Pts',(2.14455524605805,-222.344043468136,6.24331235938189));
#81995=CARTESIAN_POINT('Ctrl Pts',(3.39452996434822,-225.361093649468,6.08455449415009));
#81996=CARTESIAN_POINT('Ctrl Pts',(1.53783099275358,-228.047670937006,5.9257966289183));
#81997=CARTESIAN_POINT('Ctrl Pts',(-1.72629084293543,-227.945019902843,
5.76703876368651));
#81998=CARTESIAN_POINT('Ctrl Pts',(-3.41051136705461,-225.147086769408,
5.60828089845472));
#81999=CARTESIAN_POINT('Ctrl Pts',(-1.97343202216067,-222.214539830395,
5.44952303322292));
#82000=CARTESIAN_POINT('Ctrl Pts',(1.26973223181172,-221.831245929069,5.29076516799113));
#82001=CARTESIAN_POINT('Ctrl Pts',(3.35083759716036,-224.347995628851,5.13200730275934));
#82002=CARTESIAN_POINT('Ctrl Pts',(2.36525652535769,-227.461459703468,4.97324943752755));
#82003=CARTESIAN_POINT('Ctrl Pts',(-0.785007225443646,-228.322195954269,
4.81449157229575));
#82004=CARTESIAN_POINT('Ctrl Pts',(-3.21683239438297,-226.142458598359,
4.65573370706396));
#82005=CARTESIAN_POINT('Ctrl Pts',(-2.70461268249337,-222.91714317817,4.49697584183217));
#82006=CARTESIAN_POINT('Ctrl Pts',(0.282868450081229,-221.598058239388,
4.33821797660038));
#82007=CARTESIAN_POINT('Ctrl Pts',(3.01146838821754,-223.392430266192,4.17946011136859));
#82008=CARTESIAN_POINT('Ctrl Pts',(2.98397257597669,-226.658050050056,4.02070224613679));
#82009=CARTESIAN_POINT('Ctrl Pts',(0.225545179348082,-228.406222493524,
3.861944380905));
#82010=CARTESIAN_POINT('Ctrl Pts',(-2.73930115615294,-227.03702024443,3.70318651567321));
#82011=CARTESIAN_POINT('Ctrl Pts',(-3.19713918207074,-223.803537148623,
3.54442865044141));
#82012=CARTESIAN_POINT('Ctrl Pts',(-0.728955552641697,-221.665056805547,
3.38567078520962));
#82013=CARTESIAN_POINT('Ctrl Pts',(2.40636816656843,-222.578716346547,3.22691291997783));
#82014=CARTESIAN_POINT('Ctrl Pts',(3.33938384112868,-225.708334584547,3.06815505474604));
#82015=CARTESIAN_POINT('Ctrl Pts',(1.21619554186561,-228.189685053706,2.90939718951424));
#82016=CARTESIAN_POINT('Ctrl Pts',(-2.02005484158048,-227.751835856514,
2.75063932428246));
#82017=CARTESIAN_POINT('Ctrl Pts',(-3.40755117012691,-224.795506653864,
2.59188145905066));
#82018=CARTESIAN_POINT('Ctrl Pts',(-1.67645668665946,-222.02632962721,2.43312359381887));
#82019=CARTESIAN_POINT('Ctrl Pts',(1.58893065672184,-221.978655865403,2.27436572858708));
#82020=CARTESIAN_POINT('Ctrl Pts',(3.40012920038263,-224.696115615605,2.11560786335529));
#82021=CARTESIAN_POINT('Ctrl Pts',(2.09952866919034,-227.691691400929,1.95684999812349));
#82022=CARTESIAN_POINT('Ctrl Pts',(-1.12255845886059,-228.223829172226,
1.7980921328917));
#82023=CARTESIAN_POINT('Ctrl Pts',(-3.31728410744242,-225.80552297798,1.6393342676599));
#82024=CARTESIAN_POINT('Ctrl Pts',(-2.47602339220465,-222.649993318462,
1.48057640242812));
#82025=CARTESIAN_POINT('Ctrl Pts',(0.631277425588911,-221.645207691255,
1.32181853719632));
#82026=CARTESIAN_POINT('Ctrl Pts',(3.16086649400682,-223.71069127546,1.16306067196453));
#82027=CARTESIAN_POINT('Ctrl Pts',(2.79756298734443,-226.95622444236,1.00430280673274));
#82028=CARTESIAN_POINT('Ctrl Pts',(-0.12593258982756,-228.41127019697,0.845544941500945));
#82029=CARTESIAN_POINT('Ctrl Pts',(-2.93445385712201,-226.744628038583,
0.686787076269153));
#82030=CARTESIAN_POINT('Ctrl Pts',(-3.05679602537503,-223.480679950247,
0.528029211037362));
#82031=CARTESIAN_POINT('Ctrl Pts',(-0.382710437789346,-221.608478197099,
0.369271345805565));
#82032=CARTESIAN_POINT('Ctrl Pts',(2.64397325422008,-222.83761560249,0.210513480573779));
#82033=CARTESIAN_POINT('Ctrl Pts',(3.24608623470683,-226.05109929507,0.0517556153419814));
#82034=CARTESIAN_POINT('Ctrl Pts',(1.6736716268085,-227.542153631111,-0.0540829614792118));
#82035=CARTESIAN_POINT('Ctrl Pts',(0.745932854346969,-227.790177569842,
-0.10700224988981));
#82036=CARTESIAN_POINT('Ctrl Pts',(2.33606265769616,-223.002698443069,20.3210067496694));
#82037=CARTESIAN_POINT('Ctrl Pts',(3.00016881161637,-223.779443237332,20.2680874612588));
#82038=CARTESIAN_POINT('Ctrl Pts',(3.48035937940744,-226.034910538743,20.1622488844376));
#82039=CARTESIAN_POINT('Ctrl Pts',(1.01525982308136,-228.490138175606,20.0034910192058));
#82040=CARTESIAN_POINT('Ctrl Pts',(-2.38000652365602,-227.743617953626,
19.8447331539741));
#82041=CARTESIAN_POINT('Ctrl Pts',(-3.59659359040079,-224.489814039508,
19.6859752887423));
#82042=CARTESIAN_POINT('Ctrl Pts',(-1.52182615633225,-221.701128865433,
19.5272174235105));
#82043=CARTESIAN_POINT('Ctrl Pts',(1.94583861817437,-221.932458083289,19.3684595582787));
#82044=CARTESIAN_POINT('Ctrl Pts',(3.63261183657197,-224.970764508319,19.2097016930469));
#82045=CARTESIAN_POINT('Ctrl Pts',(1.99484845140044,-228.036042436051,19.0509438278151));
#82046=CARTESIAN_POINT('Ctrl Pts',(-1.46861473543692,-228.322628496388,
18.8921859625833));
#82047=CARTESIAN_POINT('Ctrl Pts',(-3.5879945966616,-225.5683972539,18.7334280973515));
#82048=CARTESIAN_POINT('Ctrl Pts',(-2.42364547810869,-222.293943181744,
18.5746702321197));
#82049=CARTESIAN_POINT('Ctrl Pts',(0.958825626738842,-221.496084849927,
18.4159123668879));
#82050=CARTESIAN_POINT('Ctrl Pts',(3.4637786989553,-223.905003298803,18.2571545016562));
#82051=CARTESIAN_POINT('Ctrl Pts',(2.79868206393424,-227.316065751486,18.0983966364243));
#82052=CARTESIAN_POINT('Ctrl Pts',(-0.427768493644222,-228.607463409909,
17.9396387711926));
#82053=CARTESIAN_POINT('Ctrl Pts',(-3.26272524039538,-226.597311440717,
17.7808809059607));
#82054=CARTESIAN_POINT('Ctrl Pts',(-3.11163602579296,-223.125299737827,
17.622123040729));
#82055=CARTESIAN_POINT('Ctrl Pts',(-0.112777617954695,-221.369013821348,
17.4633651754972));
#82056=CARTESIAN_POINT('Ctrl Pts',(2.98929484919384,-222.935806224066,17.3046073102654));
#82057=CARTESIAN_POINT('Ctrl Pts',(3.35556479392172,-226.39174873303,17.1458494450336));
#82058=CARTESIAN_POINT('Ctrl Pts',(0.650821968247489,-228.573962834745,
16.9870915798018));
#82059=CARTESIAN_POINT('Ctrl Pts',(-2.6495530957168,-227.485286301235,16.82833371457));
#82060=CARTESIAN_POINT('Ctrl Pts',(-3.52505727138965,-224.122075837352,
16.6695758493382));
#82061=CARTESIAN_POINT('Ctrl Pts',(-1.17442917055295,-221.562341535168,
16.5108179841064));
#82062=CARTESIAN_POINT('Ctrl Pts',(2.25103646081656,-222.148752123552,16.3520601188746));
#82063=CARTESIAN_POINT('Ctrl Pts',(3.61635361185226,-225.344624656961,16.1933022536428));
#82064=CARTESIAN_POINT('Ctrl Pts',(1.67198407948828,-228.225096717565,16.034544388411));
#82065=CARTESIAN_POINT('Ctrl Pts',(-1.80258521665346,-228.153960389228,
15.8757865231792));
#82066=CARTESIAN_POINT('Ctrl Pts',(-3.6274285934091,-225.196319636622,15.7170286579474));
#82067=CARTESIAN_POINT('Ctrl Pts',(-2.13244946411687,-222.059007160336,
15.5582707927157));
#82068=CARTESIAN_POINT('Ctrl Pts',(1.31414733087609,-221.613291215241,15.3995129274839));
#82069=CARTESIAN_POINT('Ctrl Pts',(3.55803654033007,-224.267091016787,15.2407550622521));
#82070=CARTESIAN_POINT('Ctrl Pts',(2.54561084798977,-227.591649090945,15.0819971970203));
#82071=CARTESIAN_POINT('Ctrl Pts',(-0.796557792326769,-228.544330018986,
14.9232393317885));
#82072=CARTESIAN_POINT('Ctrl Pts',(-3.40971677242986,-226.253240253028,
14.7644814665567));
#82073=CARTESIAN_POINT('Ctrl Pts',(-2.90230309648892,-222.815185056782,
14.6057236013249));
#82074=CARTESIAN_POINT('Ctrl Pts',(0.261298259228322,-221.376672410653,
14.4469657360931));
#82075=CARTESIAN_POINT('Ctrl Pts',(3.18575945837514,-223.254229031811,14.2882078708613));
#82076=CARTESIAN_POINT('Ctrl Pts',(3.19461372649398,-226.729515174404,14.1294500056295));
#82077=CARTESIAN_POINT('Ctrl Pts',(0.279757637750653,-228.621949097395,
13.9706921403977));
#82078=CARTESIAN_POINT('Ctrl Pts',(-2.89113263006087,-227.199575348879,
13.8119342751659));
#82079=CARTESIAN_POINT('Ctrl Pts',(-3.4160584285317,-223.764150327565,13.6531764099342));
#82080=CARTESIAN_POINT('Ctrl Pts',(-0.814607687543583,-221.459774877865,
13.4944185447024));
#82081=CARTESIAN_POINT('Ctrl Pts',(2.53237197705076,-222.395413320727,13.3356606794706));
#82082=CARTESIAN_POINT('Ctrl Pts',(3.56172490783136,-225.714769390036,13.1769028142388));
#82083=CARTESIAN_POINT('Ctrl Pts',(1.33138734302612,-228.379968541692,13.018144949007));
#82084=CARTESIAN_POINT('Ctrl Pts',(-2.11743586576109,-227.951820616905,
12.8593870837752));
#82085=CARTESIAN_POINT('Ctrl Pts',(-3.62838185346989,-224.822166579605,
12.7006292185434));
#82086=CARTESIAN_POINT('Ctrl Pts',(-1.81863291156572,-221.855265681656,
12.5418713533116));
#82087=CARTESIAN_POINT('Ctrl Pts',(1.65552879948739,-221.766425508193,12.3831134880798));
#82088=CARTESIAN_POINT('Ctrl Pts',(3.61455061835174,-224.636952582474,12.224355622848));
#82089=CARTESIAN_POINT('Ctrl Pts',(2.26553585343932,-227.839740638999,12.0655977576162));
#82090=CARTESIAN_POINT('Ctrl Pts',(-1.15689723545072,-228.443598174382,
11.9068398923844));
#82091=CARTESIAN_POINT('Ctrl Pts',(-3.52053801995014,-225.895874795987,
11.7480820271526));
#82092=CARTESIAN_POINT('Ctrl Pts',(-2.66218254703301,-222.528246839534,
11.5893241619209));
#82093=CARTESIAN_POINT('Ctrl Pts',(0.632602288240958,-221.42276727834,11.430566296689));
#82094=CARTESIAN_POINT('Ctrl Pts',(3.34842953419328,-223.591170963338,11.2718084314573));
#82095=CARTESIAN_POINT('Ctrl Pts',(2.99977420212569,-227.048934927288,11.1130505662255));
#82096=CARTESIAN_POINT('Ctrl Pts',(-0.0942743617640601,-228.631513726356,
10.9542927009937));
#82097=CARTESIAN_POINT('Ctrl Pts',(-3.10204303347459,-226.890531305869,
10.7955348357619));
#82098=CARTESIAN_POINT('Ctrl Pts',(-3.27082204293408,-223.419334708594,
10.6367769705301));
#82099=CARTESIAN_POINT('Ctrl Pts',(-0.446144847322243,-221.394762923856,
10.4780191052983));
#82100=CARTESIAN_POINT('Ctrl Pts',(2.78684409501469,-222.669703969432,10.3192612400665));
#82101=CARTESIAN_POINT('Ctrl Pts',(3.46931343118415,-226.077331850548,10.1605033748347));
#82102=CARTESIAN_POINT('Ctrl Pts',(0.976667251561304,-228.498985664407,
10.0017455096029));
#82103=CARTESIAN_POINT('Ctrl Pts',(-2.40982475828392,-227.718367935795,
9.84298764437113));
#82104=CARTESIAN_POINT('Ctrl Pts',(-3.59084524411178,-224.449899979241,
9.68422977913933));
#82105=CARTESIAN_POINT('Ctrl Pts',(-1.48552430373511,-221.684883540053,
9.52547191390755));
#82106=CARTESIAN_POINT('Ctrl Pts',(1.97934842100312,-221.953861554645,9.36671404867575));
#82107=CARTESIAN_POINT('Ctrl Pts',(3.63272154867527,-225.010665354639,9.20795618344396));
#82108=CARTESIAN_POINT('Ctrl Pts',(1.96142805785311,-228.057708222487,9.04919831821216));
#82109=CARTESIAN_POINT('Ctrl Pts',(-1.50496431438492,-228.306336645357,
8.89044045298038));
#82110=CARTESIAN_POINT('Ctrl Pts',(-3.59401340527916,-225.529005900414,
8.73168258774858));
#82111=CARTESIAN_POINT('Ctrl Pts',(-2.39382156899309,-222.267528976215,
8.57292472251679));
#82112=CARTESIAN_POINT('Ctrl Pts',(0.997195673100731,-221.506809425532,
8.414166857285));
#82113=CARTESIAN_POINT('Ctrl Pts',(3.47557947438652,-223.943057751236,8.2554089920532));
#82114=CARTESIAN_POINT('Ctrl Pts',(2.7731130773876,-227.346619581445,8.09665112682141));
#82115=CARTESIAN_POINT('Ctrl Pts',(-0.467306298986418,-228.602555262994,
7.93789326158962));
#82116=CARTESIAN_POINT('Ctrl Pts',(-3.28004696890443,-226.561432509518,
7.77913539635783));
#82117=CARTESIAN_POINT('Ctrl Pts',(-3.09088878186585,-223.091286784733,
7.62037753112604));
#82118=CARTESIAN_POINT('Ctrl Pts',(-0.0729493032098818,-221.367995319502,
7.46161966589424));
#82119=CARTESIAN_POINT('Ctrl Pts',(3.01175337487511,-222.968714395038,7.30286180066245));
#82120=CARTESIAN_POINT('Ctrl Pts',(3.34009948270872,-226.428465976356,7.14410393543066));
#82121=CARTESIAN_POINT('Ctrl Pts',(0.611586675313532,-228.580885552287,
6.98534607019887));
#82122=CARTESIAN_POINT('Ctrl Pts',(-2.67665023327852,-227.456078811579,
6.82658820496708));
#82123=CARTESIAN_POINT('Ctrl Pts',(-3.51521695363081,-224.083468839097,
6.66783033973528));
#82124=CARTESIAN_POINT('Ctrl Pts',(-1.13665725625273,-221.549668149031,
6.50907247450349));
#82125=CARTESIAN_POINT('Ctrl Pts',(2.2821711173499,-222.173611033291,6.35031460927169));
#82126=CARTESIAN_POINT('Ctrl Pts',(3.61235657409808,-225.384264988738,6.19155674403991));
#82127=CARTESIAN_POINT('Ctrl Pts',(1.63651343628419,-228.243239641602,6.03279887880811));
#82128=CARTESIAN_POINT('Ctrl Pts',(-1.83706673406269,-228.13400150201,5.87404101357632));
#82129=CARTESIAN_POINT('Ctrl Pts',(-3.62936350163622,-225.156525311019,
5.71528314834453));
#82130=CARTESIAN_POINT('Ctrl Pts',(-2.10006693523372,-222.03579716154,5.55652528311273));
#82131=CARTESIAN_POINT('Ctrl Pts',(1.35121080771192,-221.627907333254,5.39776741788095));
#82132=CARTESIAN_POINT('Ctrl Pts',(3.56586047257395,-224.306156580971,5.23900955264915));
#82133=CARTESIAN_POINT('Ctrl Pts',(2.51703477316183,-227.619411298497,5.08025168741736));
#82134=CARTESIAN_POINT('Ctrl Pts',(-0.835381051670971,-228.535380898648,
4.92149382218557));
#82135=CARTESIAN_POINT('Ctrl Pts',(-3.42325617085904,-226.215770039375,
4.76273595695377));
#82136=CARTESIAN_POINT('Ctrl Pts',(-2.87816737710544,-222.783486487889,
4.60397809172198));
#82137=CARTESIAN_POINT('Ctrl Pts',(0.301020087018748,-221.379756015497,
4.44522022649019));
#82138=CARTESIAN_POINT('Ctrl Pts',(3.20471397929018,-223.289272695415,4.2864623612584));
#82139=CARTESIAN_POINT('Ctrl Pts',(3.17545376384016,-226.764446937104,4.1277044960266));
#82140=CARTESIAN_POINT('Ctrl Pts',(0.240018388386984,-228.624799411569,
3.96894663079481));
#82141=CARTESIAN_POINT('Ctrl Pts',(-2.91508180625635,-227.167735606644,
3.81018876556302));
#82142=CARTESIAN_POINT('Ctrl Pts',(-3.40229924730605,-223.726760260705,
3.65143090033123));
#82143=CARTESIAN_POINT('Ctrl Pts',(-0.775732549268024,-221.451053872185,
3.49267303509943));
#82144=CARTESIAN_POINT('Ctrl Pts',(2.56078454381028,-222.423342844173,3.33391516986764));
#82145=CARTESIAN_POINT('Ctrl Pts',(3.55367173029338,-225.753788335947,3.17515730463585));
#82146=CARTESIAN_POINT('Ctrl Pts',(1.29423867433457,-228.394366788354,3.01639943940406));
#82147=CARTESIAN_POINT('Ctrl Pts',(-2.14968153578312,-227.928420856944,
2.85764157417227));
#82148=CARTESIAN_POINT('Ctrl Pts',(-3.62621334920136,-224.782384338617,
2.69888370894047));
#82149=CARTESIAN_POINT('Ctrl Pts',(-1.78403472552871,-221.835509530578,
2.54012584370868));
#82150=CARTESIAN_POINT('Ctrl Pts',(1.69089215999812,-221.784776548785,2.38136797847689));
#82151=CARTESIAN_POINT('Ctrl Pts',(3.61831511248521,-224.676615388503,2.2226101132451));
#82152=CARTESIAN_POINT('Ctrl Pts',(2.23425519005939,-227.864416938342,2.0638522480133));
#82153=CARTESIAN_POINT('Ctrl Pts',(-1.19459291014185,-228.430701931157,
1.90509438278151));
#82154=CARTESIAN_POINT('Ctrl Pts',(-3.53015385915781,-225.857213297762,
1.74633651754971));
#82155=CARTESIAN_POINT('Ctrl Pts',(-2.63490953751781,-222.499193651437,
1.58757865231793));
#82156=CARTESIAN_POINT('Ctrl Pts',(0.671786427681058,-221.42993104244,1.42882078708613));
#82157=CARTESIAN_POINT('Ctrl Pts',(3.36369894488889,-223.627956478202,1.27006292185434));
#82158=CARTESIAN_POINT('Ctrl Pts',(2.97708229266655,-227.081755146954,1.11130505662255));
#82159=CARTESIAN_POINT('Ctrl Pts',(-0.134013670091176,-228.630171025583,
0.952547191390754));
#82160=CARTESIAN_POINT('Ctrl Pts',(-3.12275743431167,-226.856580625513,
0.793789326158964));
#82161=CARTESIAN_POINT('Ctrl Pts',(-3.25295028587576,-223.383185351868,
0.635031460927172));
#82162=CARTESIAN_POINT('Ctrl Pts',(-0.407268923958301,-221.390844620734,
0.476273595695375));
#82163=CARTESIAN_POINT('Ctrl Pts',(2.81363672347351,-222.698855636535,0.317515730463589));
#82164=CARTESIAN_POINT('Ctrl Pts',(3.45438722685837,-226.118548219769,0.158757865231791));
#82165=CARTESIAN_POINT('Ctrl Pts',(1.7810709486973,-227.70528334649,0.0529192884105984));
#82166=CARTESIAN_POINT('Ctrl Pts',(0.793799282532894,-227.969222953746,
0.));
#82167=CARTESIAN_POINT('Ctrl Pts',(0.793799282532894,-227.969222953746,
0.));
#82168=CARTESIAN_POINT('Ctrl Pts',(0.886846209318506,-227.93518597229,-1.38596896950808E-16));
#82169=CARTESIAN_POINT('Ctrl Pts',(0.977826029880219,-227.896378586582,
-3.02210246537631E-15));
#82170=CARTESIAN_POINT('Ctrl Pts',(1.06653104448955,-227.853129778678,-2.55351295663786E-15));
#82171=CARTESIAN_POINT('Ctrl Pts',(1.15720914088208,-227.808918979669,-2.07450052617888E-15));
#82172=CARTESIAN_POINT('Ctrl Pts',(1.24551077493275,-227.760066361007,6.89322567199222E-15));
#82173=CARTESIAN_POINT('Ctrl Pts',(1.33118514398854,-227.706877789535,9.71445146547012E-15));
#82174=CARTESIAN_POINT('Ctrl Pts',(1.41411883983993,-227.65539068951,1.24454278877419E-14));
#82175=CARTESIAN_POINT('Ctrl Pts',(1.49459099567019,-227.59983974531,7.56147219830355E-15));
#82176=CARTESIAN_POINT('Ctrl Pts',(1.57234042917301,-227.540471725161,8.60422844084496E-15));
#82177=CARTESIAN_POINT('Ctrl Pts',(1.64037118348797,-227.488524707531,9.5166401530687E-15));
#82178=CARTESIAN_POINT('Ctrl Pts',(1.70631705692185,-227.433654524465,-2.93526588135532E-15));
#82179=CARTESIAN_POINT('Ctrl Pts',(1.76997783386621,-227.376013525802,-4.27435864480685E-15));
#82180=CARTESIAN_POINT('Ctrl Pts',(1.78334877283042,-227.363906946022,-4.55561389280964E-15));
#82181=CARTESIAN_POINT('Ctrl Pts',(1.79662071187958,-227.351676197238,9.63133291544271E-15));
#82182=CARTESIAN_POINT('Ctrl Pts',(1.80977452688484,-227.339339080185,9.2148511043888E-15));
#82183=CARTESIAN_POINT('Ctrl Pts',(1.88220124459658,-227.271409213922,6.92164487112471E-15));
#82184=CARTESIAN_POINT('Ctrl Pts',(1.95116222786656,-227.200157774703,-1.31419746077129E-15));
#82185=CARTESIAN_POINT('Ctrl Pts',(2.01641817244364,-227.125876259157,-1.55431223447522E-15));
#82186=CARTESIAN_POINT('Ctrl Pts',(2.08131428700746,-227.052004341832,-1.79310298317626E-15));
#82187=CARTESIAN_POINT('Ctrl Pts',(2.14254659564994,-226.97513487391,-3.97077426484381E-15));
#82188=CARTESIAN_POINT('Ctrl Pts',(2.19983611488132,-226.895527810078,-6.80011602582908E-15));
#82189=CARTESIAN_POINT('Ctrl Pts',(2.25566846428196,-226.817945567073,-9.55749294035897E-15));
#82190=CARTESIAN_POINT('Ctrl Pts',(2.30775631089947,-226.737762479143,2.11375777811272E-16));
#82191=CARTESIAN_POINT('Ctrl Pts',(2.35579462634617,-226.655205071499,7.49400541621981E-16));
#82192=CARTESIAN_POINT('Ctrl Pts',(2.37650837701366,-226.619606954834,9.813926651359E-16));
#82193=CARTESIAN_POINT('Ctrl Pts',(2.39646858799471,-226.583567271918,-1.66443892832159E-16));
#82194=CARTESIAN_POINT('Ctrl Pts',(2.41564783026698,-226.54710385228,-5.55111512312578E-17));
#82195=CARTESIAN_POINT('Ctrl Pts',(2.42885133814525,-226.522001450339,2.08579412955737E-17));
#82196=CARTESIAN_POINT('Ctrl Pts',(2.44168468213581,-226.496698223146,-2.0325727317242E-15));
#82197=CARTESIAN_POINT('Ctrl Pts',(2.45413838324072,-226.471199984441,-2.41473507855972E-15));
#82198=CARTESIAN_POINT('Ctrl Pts',(2.4603528762171,-226.458476166518,-2.60543703938581E-15));
#82199=CARTESIAN_POINT('Ctrl Pts',(2.46647229162971,-226.445704742015,-5.19532788277858E-16));
#82200=CARTESIAN_POINT('Ctrl Pts',(2.47249024612966,-226.432897989824,-5.55111512312578E-16));
#82201=CARTESIAN_POINT('Ctrl Pts',(2.51269156419726,-226.347345944149,-7.92785559427772E-16));
#82202=CARTESIAN_POINT('Ctrl Pts',(2.54843636148031,-226.260082355034,-2.00368207205225E-16));
#82203=CARTESIAN_POINT('Ctrl Pts',(2.57947355676129,-226.171344793313,-4.71844785465692E-16));
#82204=CARTESIAN_POINT('Ctrl Pts',(2.60982489863058,-226.084568135563,-7.37322331413281E-16));
#82205=CARTESIAN_POINT('Ctrl Pts',(2.63567461225329,-225.99638125368,1.04889574150456E-16));
#82206=CARTESIAN_POINT('Ctrl Pts',(2.65673876288241,-225.906997538612,2.22044604925031E-15));
#82207=CARTESIAN_POINT('Ctrl Pts',(2.66036639126544,-225.891604043404,2.58478320435806E-15));
#82208=CARTESIAN_POINT('Ctrl Pts',(2.66385195947195,-225.876175043544,3.7568071414668E-15));
#82209=CARTESIAN_POINT('Ctrl Pts',(2.66719385858464,-225.860711623932,3.91353616180368E-15));
#82210=CARTESIAN_POINT('Ctrl Pts',(2.68732100412239,-225.767580596769,4.9129740133754E-15));
#82211=CARTESIAN_POINT('Ctrl Pts',(2.70224099955236,-225.673200037675,1.70107545693557E-15));
#82212=CARTESIAN_POINT('Ctrl Pts',(2.71203222946397,-225.577978516612,3.88578058618805E-16));
#82213=CARTESIAN_POINT('Ctrl Pts',(2.71529428522032,-225.546254421303,-4.86948613332932E-17));
#82214=CARTESIAN_POINT('Ctrl Pts',(2.71798665538282,-225.514437102176,2.56884507968682E-15));
#82215=CARTESIAN_POINT('Ctrl Pts',(2.72011103974616,-225.482542126578,2.33146835171283E-15));
#82216=CARTESIAN_POINT('Ctrl Pts',(2.72133536904072,-225.464160352711,2.19466293790962E-15));
#82217=CARTESIAN_POINT('Ctrl Pts',(2.72237103286684,-225.445752790738,1.60478203702852E-15));
#82218=CARTESIAN_POINT('Ctrl Pts',(2.72321827117276,-225.427322468988,1.4432899320127E-15));
#82219=CARTESIAN_POINT('Ctrl Pts',(2.72379256091328,-225.414829709134,1.33382455676117E-15));
#82220=CARTESIAN_POINT('Ctrl Pts',(2.72428015707703,-225.402328109628,7.25841149902439E-15));
#82221=CARTESIAN_POINT('Ctrl Pts',(2.72468101504371,-225.389828006928,7.16093850883226E-15));
#82222=CARTESIAN_POINT('Ctrl Pts',(2.7276693801058,-225.296640710458,6.43428492425922E-15));
#82223=CARTESIAN_POINT('Ctrl Pts',(2.72584874303933,-225.203390463169,-1.34546639841518E-16));
#82224=CARTESIAN_POINT('Ctrl Pts',(2.71935799045516,-225.110452110792,1.0547118733939E-15));
#82225=CARTESIAN_POINT('Ctrl Pts',(2.71285438848203,-225.017329773426,2.24632469685943E-15));
#82226=CARTESIAN_POINT('Ctrl Pts',(2.70166177912954,-224.924519586133,3.29155883824727E-15));
#82227=CARTESIAN_POINT('Ctrl Pts',(2.68586883845382,-224.832410644551,2.70616862252382E-15));
#82228=CARTESIAN_POINT('Ctrl Pts',(2.67029895478562,-224.741602635157,2.12904636603819E-15));
#82229=CARTESIAN_POINT('Ctrl Pts',(2.65025730337592,-224.651475356299,2.00810859991659E-15));
#82230=CARTESIAN_POINT('Ctrl Pts',(2.62578581077489,-224.562426807779,2.44249065417534E-15));
#82231=CARTESIAN_POINT('Ctrl Pts',(2.61627028276454,-224.527801050718,2.61139635485662E-15));
#82232=CARTESIAN_POINT('Ctrl Pts',(2.60608454518282,-224.493338733998,1.87075692833301E-15));
#82233=CARTESIAN_POINT('Ctrl Pts',(2.59522949564799,-224.459064719813,1.52655665885959E-15));
#82234=CARTESIAN_POINT('Ctrl Pts',(2.58886717656257,-224.438976168961,1.32481534605862E-15));
#82235=CARTESIAN_POINT('Ctrl Pts',(2.58227491151728,-224.418952323084,4.28946205561218E-15));
#82236=CARTESIAN_POINT('Ctrl Pts',(2.57545275110093,-224.398998344058,4.57966997657877E-15));
#82237=CARTESIAN_POINT('Ctrl Pts',(2.5704218465062,-224.384283567705,4.79367965590514E-15));
#82238=CARTESIAN_POINT('Ctrl Pts',(2.56526611083976,-224.369607571018,5.69313263505859E-15));
#82239=CARTESIAN_POINT('Ctrl Pts',(2.55999017666067,-224.354984576636,5.64825963778048E-15));
#82240=CARTESIAN_POINT('Ctrl Pts',(2.52758631659065,-224.265172716277,5.3726575784364E-15));
#82241=CARTESIAN_POINT('Ctrl Pts',(2.49061098433064,-224.177234165273,8.16050019748306E-15));
#82242=CARTESIAN_POINT('Ctrl Pts',(2.44913633387512,-224.091610553351,5.87724313660942E-15));
#82243=CARTESIAN_POINT('Ctrl Pts',(2.41803034603348,-224.02739284441,4.16480034095419E-15));
#82244=CARTESIAN_POINT('Ctrl Pts',(2.38439235385754,-223.964477823302,3.84165326499715E-15));
#82245=CARTESIAN_POINT('Ctrl Pts',(2.34823558025232,-223.903068833463,2.69922972861991E-15));
#82246=CARTESIAN_POINT('Ctrl Pts',(2.33711744989038,-223.884185700751,2.347936940589E-15));
#82247=CARTESIAN_POINT('Ctrl Pts',(2.32576105888447,-223.865445092701,7.90760064772973E-15));
#82248=CARTESIAN_POINT('Ctrl Pts',(2.3141665399975,-223.84685326456,8.88178419700125E-15));
#82249=CARTESIAN_POINT('Ctrl Pts',(2.30317844043336,-223.829233830698,9.80501576335647E-15));
#82250=CARTESIAN_POINT('Ctrl Pts',(2.29197545802167,-223.811746728186,9.82976587205289E-15));
#82251=CARTESIAN_POINT('Ctrl Pts',(2.28056965781359,-223.794414998359,9.61036805691151E-15));
#82252=CARTESIAN_POINT('Ctrl Pts',(2.23334862735917,-223.722660090588,8.70204152817875E-15));
#82253=CARTESIAN_POINT('Ctrl Pts',(2.18261057933454,-223.653494343049,7.7981406418901E-15));
#82254=CARTESIAN_POINT('Ctrl Pts',(2.12839132810104,-223.587269158508,5.40886779809568E-15));
#82255=CARTESIAN_POINT('Ctrl Pts',(2.07470602204923,-223.521696152249,3.04312424866893E-15));
#82256=CARTESIAN_POINT('Ctrl Pts',(2.01760738089684,-223.459005490671,5.95831660746538E-15));
#82257=CARTESIAN_POINT('Ctrl Pts',(1.95710205007443,-223.399580086106,4.69329436425525E-15));
#82258=CARTESIAN_POINT('Ctrl Pts',(1.94393780877166,-223.386650806081,4.39418859168102E-15));
#82259=CARTESIAN_POINT('Ctrl Pts',(1.93061220615115,-223.373876274008,9.21580020631812E-16));
#82260=CARTESIAN_POINT('Ctrl Pts',(1.91712862604369,-223.36125788605,9.43689570931383E-16));
#82261=CARTESIAN_POINT('Ctrl Pts',(1.91346599666507,-223.364012796625,20.));
#82262=CARTESIAN_POINT('Ctrl Pts',(1.97507204620631,-223.421907355683,20.));
#82263=CARTESIAN_POINT('Ctrl Pts',(2.0333066520343,-223.482952882657,20.));
#82264=CARTESIAN_POINT('Ctrl Pts',(2.08817311815043,-223.546764476174,20.));
#82265=CARTESIAN_POINT('Ctrl Pts',(2.14449280559963,-223.612266216252,20.));
#82266=CARTESIAN_POINT('Ctrl Pts',(2.19726400543086,-223.680682922028,20.));
#82267=CARTESIAN_POINT('Ctrl Pts',(2.2464647374009,-223.751646843991,20.));
#82268=CARTESIAN_POINT('Ctrl Pts',(2.29735442070123,-223.825046799029,20.));
#82269=CARTESIAN_POINT('Ctrl Pts',(2.3444248776897,-223.901172374798,20.));
#82270=CARTESIAN_POINT('Ctrl Pts',(2.38761687181107,-223.979660611969,20.));
#82271=CARTESIAN_POINT('Ctrl Pts',(2.40651336923917,-224.013999215731,20.));
#82272=CARTESIAN_POINT('Ctrl Pts',(2.42466701090125,-224.048790553719,20.));
#82273=CARTESIAN_POINT('Ctrl Pts',(2.44207039268086,-224.084006319604,20.));
#82274=CARTESIAN_POINT('Ctrl Pts',(2.45159423353378,-224.103277824076,20.));
#82275=CARTESIAN_POINT('Ctrl Pts',(2.46089336489712,-224.122676452755,20.));
#82276=CARTESIAN_POINT('Ctrl Pts',(2.46996636855114,-224.142197696102,20.));
#82277=CARTESIAN_POINT('Ctrl Pts',(2.47861912489588,-224.160814746053,20.));
#82278=CARTESIAN_POINT('Ctrl Pts',(2.48706870907561,-224.179549321891,20.));
#82279=CARTESIAN_POINT('Ctrl Pts',(2.49529978068773,-224.19836470108,20.));
#82280=CARTESIAN_POINT('Ctrl Pts',(2.5318521426381,-224.281919623545,20.));
#82281=CARTESIAN_POINT('Ctrl Pts',(2.56414460268445,-224.367158064701,20.));
#82282=CARTESIAN_POINT('Ctrl Pts',(2.59215310190908,-224.453681020382,20.));
#82283=CARTESIAN_POINT('Ctrl Pts',(2.6206247923598,-224.541634851514,20.));
#82284=CARTESIAN_POINT('Ctrl Pts',(2.64467014986719,-224.630916789565,20.));
#82285=CARTESIAN_POINT('Ctrl Pts',(2.66422479244635,-224.721144837958,20.));
#82286=CARTESIAN_POINT('Ctrl Pts',(2.68343404373964,-224.809779199249,20.));
#82287=CARTESIAN_POINT('Ctrl Pts',(2.69831007225569,-224.899327453851,20.));
#82288=CARTESIAN_POINT('Ctrl Pts',(2.70874920819526,-224.989450307808,20.));
#82289=CARTESIAN_POINT('Ctrl Pts',(2.71288525755108,-225.025157532449,20.));
#82290=CARTESIAN_POINT('Ctrl Pts',(2.71632430966266,-225.060955138582,20.));
#82291=CARTESIAN_POINT('Ctrl Pts',(2.71905787810446,-225.096822560585,20.));
#82292=CARTESIAN_POINT('Ctrl Pts',(2.72067784521375,-225.118078309317,20.));
#82293=CARTESIAN_POINT('Ctrl Pts',(2.72205002487447,-225.139358581396,20.));
#82294=CARTESIAN_POINT('Ctrl Pts',(2.72317244633848,-225.160659119609,20.));
#82295=CARTESIAN_POINT('Ctrl Pts',(2.72391546865431,-225.174759683202,20.));
#82296=CARTESIAN_POINT('Ctrl Pts',(2.72454895911028,-225.188869036708,20.));
#82297=CARTESIAN_POINT('Ctrl Pts',(2.72507200358104,-225.202971554569,20.));
#82298=CARTESIAN_POINT('Ctrl Pts',(2.72860218826004,-225.298153695426,20.));
#82299=CARTESIAN_POINT('Ctrl Pts',(2.72711435296688,-225.393186006008,20.));
#82300=CARTESIAN_POINT('Ctrl Pts',(2.72055005265772,-225.487669542712,20.));
#82301=CARTESIAN_POINT('Ctrl Pts',(2.71400792544162,-225.581833930055,20.));
#82302=CARTESIAN_POINT('Ctrl Pts',(2.70242392945975,-225.675454198458,20.));
#82303=CARTESIAN_POINT('Ctrl Pts',(2.68569220565089,-225.768153332782,20.));
#82304=CARTESIAN_POINT('Ctrl Pts',(2.68378820044636,-225.778702134341,20.));
#82305=CARTESIAN_POINT('Ctrl Pts',(2.6818174797233,-225.789239017697,20.));
#82306=CARTESIAN_POINT('Ctrl Pts',(2.6797798446426,-225.799763433399,20.));
#82307=CARTESIAN_POINT('Ctrl Pts',(2.66224922851865,-225.890309328171,20.));
#82308=CARTESIAN_POINT('Ctrl Pts',(2.63977008234293,-225.979932689554,20.));
#82309=CARTESIAN_POINT('Ctrl Pts',(2.61261752651431,-226.068395697362,20.));
#82310=CARTESIAN_POINT('Ctrl Pts',(2.6019190685787,-226.103251265798,20.));
#82311=CARTESIAN_POINT('Ctrl Pts',(2.59049450555523,-226.137926643292,20.));
#82312=CARTESIAN_POINT('Ctrl Pts',(2.57835850114292,-226.172406945337,20.));
#82313=CARTESIAN_POINT('Ctrl Pts',(2.57307177652304,-226.187427363552,20.));
#82314=CARTESIAN_POINT('Ctrl Pts',(2.56765002841871,-226.202410759174,20.));
#82315=CARTESIAN_POINT('Ctrl Pts',(2.56209440081032,-226.217355882885,20.));
#82316=CARTESIAN_POINT('Ctrl Pts',(2.5576754550037,-226.229243233227,20.));
#82317=CARTESIAN_POINT('Ctrl Pts',(2.5531721611383,-226.241105288201,20.));
#82318=CARTESIAN_POINT('Ctrl Pts',(2.54858887947735,-226.252932113005,20.));
#82319=CARTESIAN_POINT('Ctrl Pts',(2.5148395638014,-226.340019766195,20.));
#82320=CARTESIAN_POINT('Ctrl Pts',(2.47670681197659,-226.425334524189,20.));
#82321=CARTESIAN_POINT('Ctrl Pts',(2.43452410494245,-226.508645454499,20.));
#82322=CARTESIAN_POINT('Ctrl Pts',(2.39075655225714,-226.595086458123,20.));
#82323=CARTESIAN_POINT('Ctrl Pts',(2.34262888455579,-226.679370953022,20.));
#82324=CARTESIAN_POINT('Ctrl Pts',(2.2904575051027,-226.761237987111,20.));
#82325=CARTESIAN_POINT('Ctrl Pts',(2.23768209969329,-226.844052855319,20.));
#82326=CARTESIAN_POINT('Ctrl Pts',(2.18076839577045,-226.924394776583,20.));
#82327=CARTESIAN_POINT('Ctrl Pts',(2.11999199178509,-227.001978860565,20.));
#82328=CARTESIAN_POINT('Ctrl Pts',(2.07727651489662,-227.056507278322,20.));
#82329=CARTESIAN_POINT('Ctrl Pts',(2.03265187999783,-227.109673119658,20.));
#82330=CARTESIAN_POINT('Ctrl Pts',(1.98620043359043,-227.161369816309,20.));
#82331=CARTESIAN_POINT('Ctrl Pts',(1.9748368627249,-227.174016550078,20.));
#82332=CARTESIAN_POINT('Ctrl Pts',(1.96336316985503,-227.186576018518,20.));
#82333=CARTESIAN_POINT('Ctrl Pts',(1.95179223578434,-227.199034258492,20.));
#82334=CARTESIAN_POINT('Ctrl Pts',(1.88311834246096,-227.272974342998,20.));
#82335=CARTESIAN_POINT('Ctrl Pts',(1.81093148723848,-227.343453721762,20.));
#82336=CARTESIAN_POINT('Ctrl Pts',(1.73554509733181,-227.410185133041,20.));
#82337=CARTESIAN_POINT('Ctrl Pts',(1.67071538458667,-227.467571860668,20.));
#82338=CARTESIAN_POINT('Ctrl Pts',(1.60351843822465,-227.522186884759,20.));
#82339=CARTESIAN_POINT('Ctrl Pts',(1.53412735933154,-227.573832219717,20.));
#82340=CARTESIAN_POINT('Ctrl Pts',(1.50861560997377,-227.592819715833,20.));
#82341=CARTESIAN_POINT('Ctrl Pts',(1.48280707006451,-227.611405636062,20.));
#82342=CARTESIAN_POINT('Ctrl Pts',(1.45670963374051,-227.629579490491,20.));
#82343=CARTESIAN_POINT('Ctrl Pts',(1.43999804908724,-227.641217181758,20.));
#82344=CARTESIAN_POINT('Ctrl Pts',(1.42316693937207,-227.652686484956,20.));
#82345=CARTESIAN_POINT('Ctrl Pts',(1.40623320439776,-227.663974970311,20.));
#82346=CARTESIAN_POINT('Ctrl Pts',(1.32003064973545,-227.721439922805,20.));
#82347=CARTESIAN_POINT('Ctrl Pts',(1.23108709427863,-227.774282172299,20.));
#82348=CARTESIAN_POINT('Ctrl Pts',(1.13970922754748,-227.822182038463,20.));
#82349=CARTESIAN_POINT('Ctrl Pts',(1.04833136081634,-227.870081904628,20.));
#82350=CARTESIAN_POINT('Ctrl Pts',(0.95451854354455,-227.913040290229,20.));
#82351=CARTESIAN_POINT('Ctrl Pts',(0.858539654927881,-227.950697062107,
20.));
#82352=CARTESIAN_POINT('Ctrl Pts',(0.837654143889281,-227.958891373753,
20.));
#82353=CARTESIAN_POINT('Ctrl Pts',(0.816665943600311,-227.966834461527,
20.));
#82354=CARTESIAN_POINT('Ctrl Pts',(0.79557914645247,-227.974527555281,20.));
#82355=CARTESIAN_POINT('Ctrl Pts',(-2.51944981591128,-225.001988766476,
18.387416697508));
#82356=CARTESIAN_POINT('Ctrl Pts',(-2.52058771038653,-225.133540125377,
18.3957515808994));
#82357=CARTESIAN_POINT('Ctrl Pts',(-2.51117350858125,-225.264928190453,
18.4040864642907));
#82358=CARTESIAN_POINT('Ctrl Pts',(-2.4906388306482,-225.394554500649,18.4124213476821));
#82359=CARTESIAN_POINT('Ctrl Pts',(-2.36026141647998,-226.217569265554,
18.4653406360927));
#82360=CARTESIAN_POINT('Ctrl Pts',(-1.78160095331279,-226.969565052438,
18.5182599245033));
#82361=CARTESIAN_POINT('Ctrl Pts',(-1.01945099542026,-227.306439232042,
18.5711792129139));
#82362=CARTESIAN_POINT('Ctrl Pts',(-0.257301037527725,-227.643313411645,
18.6240985013245));
#82363=CARTESIAN_POINT('Ctrl Pts',(0.688338415090144,-227.565065983968,
18.6770177897351));
#82364=CARTESIAN_POINT('Ctrl Pts',(1.38473979760912,-227.107481384978,18.7299370781457));
#82365=CARTESIAN_POINT('Ctrl Pts',(2.0811411801281,-226.649896785989,18.7828563665563));
#82366=CARTESIAN_POINT('Ctrl Pts',(2.52830449254818,-225.812975015687,18.8357756549669));
#82367=CARTESIAN_POINT('Ctrl Pts',(2.52161384371424,-224.979735299399,18.8886949433774));
#82368=CARTESIAN_POINT('Ctrl Pts',(2.51492319488031,-224.14649558311,18.941614231788));
#82369=CARTESIAN_POINT('Ctrl Pts',(2.05437858479236,-223.316937920834,18.9945335201986));
#82370=CARTESIAN_POINT('Ctrl Pts',(1.35071296757332,-222.870578844268,19.0474528086093));
#82371=CARTESIAN_POINT('Ctrl Pts',(0.64704735035428,-222.424219767701,19.1003720970199));
#82372=CARTESIAN_POINT('Ctrl Pts',(-0.299739273995854,-222.361059276843,
19.1532913854304));
#82373=CARTESIAN_POINT('Ctrl Pts',(-1.05637248722117,-222.710180453557,
19.206210673841));
#82374=CARTESIAN_POINT('Ctrl Pts',(-1.81300570044648,-223.059301630271,
19.2591299622516));
#82375=CARTESIAN_POINT('Ctrl Pts',(-2.37948550254698,-223.820704474557,
19.3120492506622));
#82376=CARTESIAN_POINT('Ctrl Pts',(-2.49664124652711,-224.645603681732,
19.3649685390728));
#82377=CARTESIAN_POINT('Ctrl Pts',(-2.51320691839867,-224.762243371166,
19.3724512585512));
#82378=CARTESIAN_POINT('Ctrl Pts',(-2.52078898607152,-224.880152581298,
19.3799339780296));
#82379=CARTESIAN_POINT('Ctrl Pts',(-2.51981687702631,-224.998184138844,
19.387416697508));
#82380=CARTESIAN_POINT('Ctrl Pts',(-0.793799282532874,-227.969222953746,
20.));
#82381=CARTESIAN_POINT('Ctrl Pts',(-1.78107094869727,-227.70528334649,19.9470807115894));
#82382=CARTESIAN_POINT('Ctrl Pts',(-3.45438732992763,-226.118548905711,
19.8412421347682));
#82383=CARTESIAN_POINT('Ctrl Pts',(-2.8136366341492,-222.698855410048,19.6824842695364));
#82384=CARTESIAN_POINT('Ctrl Pts',(0.40726891511089,-221.390844838622,19.5237264043046));
#82385=CARTESIAN_POINT('Ctrl Pts',(3.25295021883841,-223.383185295634,19.3649685390728));
#82386=CARTESIAN_POINT('Ctrl Pts',(3.12275738725604,-226.856580639298,19.206210673841));
#82387=CARTESIAN_POINT('Ctrl Pts',(0.1340136609786,-228.63017093477,19.0474528086092));
#82388=CARTESIAN_POINT('Ctrl Pts',(-2.97708223483621,-227.08175512352,18.8886949433775));
#82389=CARTESIAN_POINT('Ctrl Pts',(-3.36369888730502,-223.627956495351,
18.7299370781457));
#82390=CARTESIAN_POINT('Ctrl Pts',(-0.671786414007324,-221.429931110442,
18.5711792129139));
#82391=CARTESIAN_POINT('Ctrl Pts',(2.63490948932574,-222.499193694183,18.4124213476821));
#82392=CARTESIAN_POINT('Ctrl Pts',(3.53015379637291,-225.857213283498,18.2536634824503));
#82393=CARTESIAN_POINT('Ctrl Pts',(1.19459288842475,-228.430701869046,18.0949056172185));
#82394=CARTESIAN_POINT('Ctrl Pts',(-2.23425514982848,-227.864416887275,
17.9361477519867));
#82395=CARTESIAN_POINT('Ctrl Pts',(-3.61831504767861,-224.676615394144,
17.7773898867549));
#82396=CARTESIAN_POINT('Ctrl Pts',(-1.69089212962583,-221.784776606531,
17.6186320215231));
#82397=CARTESIAN_POINT('Ctrl Pts',(1.78403469350766,-221.835509587289,17.4598741562913));
#82398=CARTESIAN_POINT('Ctrl Pts',(3.6262132841795,-224.782384342542,17.3011162910595));
#82399=CARTESIAN_POINT('Ctrl Pts',(2.14968149722227,-227.928420804412,17.1423584258278));
#82400=CARTESIAN_POINT('Ctrl Pts',(-1.29423865111908,-228.394366727483,
16.9836005605959));
#82401=CARTESIAN_POINT('Ctrl Pts',(-3.55367166656124,-225.753788322425,
16.8248426953642));
#82402=CARTESIAN_POINT('Ctrl Pts',(-2.56078449788238,-222.423342890386,
16.6660848301324));
#82403=CARTESIAN_POINT('Ctrl Pts',(0.775732535354965,-221.451053935833,
16.5073269649006));
#82404=CARTESIAN_POINT('Ctrl Pts',(3.40229918628707,-223.726760283541,16.3485690996688));
#82405=CARTESIAN_POINT('Ctrl Pts',(2.91508175397509,-227.167735567766,16.189811234437));
#82406=CARTESIAN_POINT('Ctrl Pts',(-0.240018384082209,-228.62479934656,
16.0310533692052));
#82407=CARTESIAN_POINT('Ctrl Pts',(-3.17545370688936,-226.764446905459,
15.8722955039734));
#82408=CARTESIAN_POINT('Ctrl Pts',(-3.20471392181458,-223.289272726097,
15.7135376387416));
#82409=CARTESIAN_POINT('Ctrl Pts',(-0.301020081620057,-221.379756080425,
15.5547797735098));
#82410=CARTESIAN_POINT('Ctrl Pts',(2.87816732548634,-222.783486527642,15.396021908278));
#82411=CARTESIAN_POINT('Ctrl Pts',(3.42325610946395,-226.21577001757,15.2372640430462));
#82412=CARTESIAN_POINT('Ctrl Pts',(0.835381036688694,-228.535380835242,
15.0785061778144));
#82413=CARTESIAN_POINT('Ctrl Pts',(-2.51703472801954,-227.619411251518,
14.9197483125827));
#82414=CARTESIAN_POINT('Ctrl Pts',(-3.5658604086213,-224.306156593415,14.7609904473508));
#82415=CARTESIAN_POINT('Ctrl Pts',(-1.35121078347837,-221.627907393731,
14.6022325821191));
#82416=CARTESIAN_POINT('Ctrl Pts',(2.10006689756961,-222.035797214701,14.4434747168873));
#82417=CARTESIAN_POINT('Ctrl Pts',(3.62936343654465,-225.156525308212,14.2847168516555));
#82418=CARTESIAN_POINT('Ctrl Pts',(1.83706670111546,-228.134001445802,14.1259589864237));
#82419=CARTESIAN_POINT('Ctrl Pts',(-1.6365134069338,-228.243239583436,13.9672011211919));
#82420=CARTESIAN_POINT('Ctrl Pts',(-3.61235650931153,-225.384264981846,
13.8084432559601));
#82421=CARTESIAN_POINT('Ctrl Pts',(-2.28217107641984,-222.173611083982,
13.6496853907283));
#82422=CARTESIAN_POINT('Ctrl Pts',(1.13665723586709,-221.549668210912,13.4909275254965));
#82423=CARTESIAN_POINT('Ctrl Pts',(3.51521689058642,-224.083468855535,13.3321696602647));
#82424=CARTESIAN_POINT('Ctrl Pts',(2.67665018527361,-227.45607876753,13.1734117950329));
#82425=CARTESIAN_POINT('Ctrl Pts',(-0.611586664344894,-228.580885488065,
13.0146539298011));
#82426=CARTESIAN_POINT('Ctrl Pts',(-3.34009942280501,-226.428465950738,
12.8558960645693));
#82427=CARTESIAN_POINT('Ctrl Pts',(-3.01175332086021,-222.968714431468,
12.6971381993376));
#82428=CARTESIAN_POINT('Ctrl Pts',(0.0729493019015324,-221.367995384641,
12.5383803341057));
#82429=CARTESIAN_POINT('Ctrl Pts',(3.09088872643165,-223.091286818965,12.379622468874));
#82430=CARTESIAN_POINT('Ctrl Pts',(3.28004691007777,-226.561432481514,12.2208646036422));
#82431=CARTESIAN_POINT('Ctrl Pts',(0.467306290605433,-228.602555198383,
12.0621067384104));
#82432=CARTESIAN_POINT('Ctrl Pts',(-2.77311302765262,-227.346619539359,
11.9033488731786));
#82433=CARTESIAN_POINT('Ctrl Pts',(-3.47557941205303,-223.943057770192,
11.7445910079468));
#82434=CARTESIAN_POINT('Ctrl Pts',(-0.997195655216347,-221.506809488182,
11.585833142715));
#82435=CARTESIAN_POINT('Ctrl Pts',(2.39382152606057,-222.267529025221,11.4270752774832));
#82436=CARTESIAN_POINT('Ctrl Pts',(3.5940133408216,-225.529005890927,11.2683174122514));
#82437=CARTESIAN_POINT('Ctrl Pts',(1.50496428739385,-228.306336586058,11.1095595470196));
#82438=CARTESIAN_POINT('Ctrl Pts',(-1.96142802267546,-228.057708167648,
10.9508016817878));
#82439=CARTESIAN_POINT('Ctrl Pts',(-3.63272148352348,-225.010665354448,
10.792043816556));
#82440=CARTESIAN_POINT('Ctrl Pts',(-1.97934838550411,-221.953861609276,
10.6332859513242));
#82441=CARTESIAN_POINT('Ctrl Pts',(1.48552427709262,-221.684883599509,10.4745280860925));
#82442=CARTESIAN_POINT('Ctrl Pts',(3.59084517971103,-224.449899989107,10.3157702208607));
#82443=CARTESIAN_POINT('Ctrl Pts',(2.40982471506444,-227.718367887042,10.1570123556289));
#82444=CARTESIAN_POINT('Ctrl Pts',(-0.97666723404505,-228.498985601654,
9.99825449039707));
#82445=CARTESIAN_POINT('Ctrl Pts',(-3.46931336896303,-226.077331831226,
9.83949662516529));
#82446=CARTESIAN_POINT('Ctrl Pts',(-2.78684404503348,-222.669704011225,
9.6807387599335));
#82447=CARTESIAN_POINT('Ctrl Pts',(0.446144839320715,-221.394762988514,
9.5219808947017));
#82448=CARTESIAN_POINT('Ctrl Pts',(3.27082198427282,-223.419334736943,9.36322302946992));
#82449=CARTESIAN_POINT('Ctrl Pts',(3.1020429778404,-226.890531271963,9.20446516423812));
#82450=CARTESIAN_POINT('Ctrl Pts',(0.0942743600733127,-228.631513661226,
9.04570729900632));
#82451=CARTESIAN_POINT('Ctrl Pts',(-2.99977414832561,-227.048934890541,
8.88694943377454));
#82452=CARTESIAN_POINT('Ctrl Pts',(-3.34842947414019,-223.591170988605,
8.72819156854274));
#82453=CARTESIAN_POINT('Ctrl Pts',(-0.632602276895449,-221.422767342497,
8.56943370331095));
#82454=CARTESIAN_POINT('Ctrl Pts',(2.6621824992875,-222.528246883865,8.41067583807915));
#82455=CARTESIAN_POINT('Ctrl Pts',(3.52053795681035,-225.89587477992,8.25191797284737));
#82456=CARTESIAN_POINT('Ctrl Pts',(1.15689721470216,-228.443598112622,8.09316010761557));
#82457=CARTESIAN_POINT('Ctrl Pts',(-2.26553581280758,-227.839740588069,
7.93440224238378));
#82458=CARTESIAN_POINT('Ctrl Pts',(-3.61455055352584,-224.636952588985,
7.77564437715198));
#82459=CARTESIAN_POINT('Ctrl Pts',(-1.655528769796,-221.766425566186,7.6168865119202));
#82460=CARTESIAN_POINT('Ctrl Pts',(1.81863287894903,-221.855265738056,7.4581286466884));
#82461=CARTESIAN_POINT('Ctrl Pts',(3.62838178839593,-224.822166582794,7.29937078145661));
#82462=CARTESIAN_POINT('Ctrl Pts',(2.11743582778552,-227.951820563965,7.14061291622481));
#82463=CARTESIAN_POINT('Ctrl Pts',(-1.33138731914806,-228.379968481073,
6.98185505099303));
#82464=CARTESIAN_POINT('Ctrl Pts',(-3.56172484395287,-225.714769377217,
6.82309718576123));
#82465=CARTESIAN_POINT('Ctrl Pts',(-2.53237193163343,-222.395413367439,
6.66433932052944));
#82466=CARTESIAN_POINT('Ctrl Pts',(0.814607672933798,-221.459774941358,
6.50558145529765));
#82467=CARTESIAN_POINT('Ctrl Pts',(3.41605836726569,-223.76415034973,6.34682359006585));
#82468=CARTESIAN_POINT('Ctrl Pts',(2.89113257820927,-227.19957530943,6.18806572483406));
#82469=CARTESIAN_POINT('Ctrl Pts',(-0.279757632733263,-228.621949032436,
6.02930785960227));
#82470=CARTESIAN_POINT('Ctrl Pts',(-3.19461366919951,-226.729515143386,
5.87054999437048));
#82471=CARTESIAN_POINT('Ctrl Pts',(-3.18575940123949,-223.254229063121,
5.71179212913868));
#82472=CARTESIAN_POINT('Ctrl Pts',(-0.261298254542071,-221.376672475636,
5.5530342639069));
#82473=CARTESIAN_POINT('Ctrl Pts',(2.90230304443695,-222.815185095966,5.3942763986751));
#82474=CARTESIAN_POINT('Ctrl Pts',(3.40971671127761,-226.253240230551,5.23551853344331));
#82475=CARTESIAN_POINT('Ctrl Pts',(0.796557778040768,-228.54432995542,5.07676066821151));
#82476=CARTESIAN_POINT('Ctrl Pts',(-2.54561080233497,-227.591649044464,
4.91800280297972));
#82477=CARTESIAN_POINT('Ctrl Pts',(-3.55803647651774,-224.267091029931,
4.75924493774793));
#82478=CARTESIAN_POINT('Ctrl Pts',(-1.31414730730727,-221.61329127598,4.60048707251613));
#82479=CARTESIAN_POINT('Ctrl Pts',(2.13244942587199,-222.059007213082,4.44172920728434));
#82480=CARTESIAN_POINT('Ctrl Pts',(3.62742852835224,-225.196319633101,4.28297134205255));
#82481=CARTESIAN_POINT('Ctrl Pts',(1.80258518432463,-228.153960332663,4.12421347682076));
#82482=CARTESIAN_POINT('Ctrl Pts',(-1.67198404950171,-228.225096659724,
3.96545561158897));
#82483=CARTESIAN_POINT('Ctrl Pts',(-3.61635354699401,-225.34462465078,3.80669774635717));
#82484=CARTESIAN_POINT('Ctrl Pts',(-2.25103642044492,-222.148752174688,
3.64793988112538));
#82485=CARTESIAN_POINT('Ctrl Pts',(1.17442914948988,-221.562341596822,3.48918201589359));
#82486=CARTESIAN_POINT('Ctrl Pts',(3.52505720816877,-224.122075853096,3.3304241506618));
#82487=CARTESIAN_POINT('Ctrl Pts',(2.64955304819789,-227.485286256663,3.17166628543001));
#82488=CARTESIAN_POINT('Ctrl Pts',(-0.650821956575191,-228.573962770645,
3.01290842019821));
#82489=CARTESIAN_POINT('Ctrl Pts',(-3.35556473374051,-226.391748708072,
2.85415055496642));
#82490=CARTESIAN_POINT('Ctrl Pts',(-2.98929479558205,-222.93580626108,2.69539268973463));
#82491=CARTESIAN_POINT('Ctrl Pts',(0.112777615932726,-221.369013886482,
2.53663482450283));
#82492=CARTESIAN_POINT('Ctrl Pts',(3.11163596998505,-223.125299771423,2.37787695927105));
#82493=CARTESIAN_POINT('Ctrl Pts',(3.26272518188304,-226.597311412118,2.21911909403925));
#82494=CARTESIAN_POINT('Ctrl Pts',(0.427768485964111,-228.607463345116,
2.06036122880746));
#82495=CARTESIAN_POINT('Ctrl Pts',(-2.79868201372234,-227.316065710128,
1.90160336357566));
#82496=CARTESIAN_POINT('Ctrl Pts',(-3.46377863687395,-223.905003318099,
1.74284549834387));
#82497=CARTESIAN_POINT('Ctrl Pts',(-0.958825609453758,-221.496084913414,
1.58408763311208));
#82498=CARTESIAN_POINT('Ctrl Pts',(2.42364543444732,-222.293943229063,1.42532976788028));
#82499=CARTESIAN_POINT('Ctrl Pts',(3.58799453273333,-225.568397245971,1.2665719026485));
#82500=CARTESIAN_POINT('Ctrl Pts',(1.46861470818642,-228.322628432602,1.1078140374167));
#82501=CARTESIAN_POINT('Ctrl Pts',(-1.9948484136595,-228.0360423893,0.949056172184909));
#82502=CARTESIAN_POINT('Ctrl Pts',(-3.63261177564012,-224.970764494873,
0.790298306953122));
#82503=CARTESIAN_POINT('Ctrl Pts',(-1.94583857424385,-221.93245816329,0.631540441721324));
#82504=CARTESIAN_POINT('Ctrl Pts',(1.52182610974532,-221.701128880727,0.472782576489534));
#82505=CARTESIAN_POINT('Ctrl Pts',(3.59659356700835,-224.489814123823,0.314024711257741));
#82506=CARTESIAN_POINT('Ctrl Pts',(2.38000639294467,-227.743617779076,0.155266846025945));
#82507=CARTESIAN_POINT('Ctrl Pts',(-1.0152596211774,-228.490138311657,-0.00349101920584169));
#82508=CARTESIAN_POINT('Ctrl Pts',(-3.48035985289286,-226.03491003184,-0.162248884437638));
#82509=CARTESIAN_POINT('Ctrl Pts',(-3.00016881161638,-223.779443237332,
-0.268087461258832));
#82510=CARTESIAN_POINT('Ctrl Pts',(-2.33606265769617,-223.002698443069,
-0.32100674966943));
#82511=CARTESIAN_POINT('Ctrl Pts',(-0.745932854346956,-227.790177569842,
20.1070022498898));
#82512=CARTESIAN_POINT('Ctrl Pts',(-1.67367162680847,-227.542153631111,
20.0540829614792));
#82513=CARTESIAN_POINT('Ctrl Pts',(-3.24608633156098,-226.051099939649,
19.948244384658));
#82514=CARTESIAN_POINT('Ctrl Pts',(-2.64397317028206,-222.83761538966,19.7894865194262));
#82515=CARTESIAN_POINT('Ctrl Pts',(0.382710429475444,-221.608478401848,
19.6307286541944));
#82516=CARTESIAN_POINT('Ctrl Pts',(3.05679596238007,-223.480679897405,19.4719707889627));
#82517=CARTESIAN_POINT('Ctrl Pts',(2.93445381290385,-226.744628051537,19.3132129237308));
#82518=CARTESIAN_POINT('Ctrl Pts',(0.125932581264471,-228.411270111633,
19.1544550584991));
#82519=CARTESIAN_POINT('Ctrl Pts',(-2.79756293300129,-226.95622442034,18.9956971932673));
#82520=CARTESIAN_POINT('Ctrl Pts',(-3.16086643989526,-223.710691291575,
18.8369393280355));
#82521=CARTESIAN_POINT('Ctrl Pts',(-0.631277412739705,-221.645207755157,
18.6781814628037));
#82522=CARTESIAN_POINT('Ctrl Pts',(2.4760233469186,-222.64999335863,18.5194235975719));
#82523=CARTESIAN_POINT('Ctrl Pts',(3.31728404844348,-225.805522964576,18.3606657323401));
#82524=CARTESIAN_POINT('Ctrl Pts',(1.12255843845303,-228.22382911386,18.2019078671083));
#82525=CARTESIAN_POINT('Ctrl Pts',(-2.09952863138538,-227.691691352941,
18.0431500018765));
#82526=CARTESIAN_POINT('Ctrl Pts',(-3.4001291394839,-224.696115620906,17.8843921366447));
#82527=CARTESIAN_POINT('Ctrl Pts',(-1.588930628181,-221.978655919667,17.7256342714129));
#82528=CARTESIAN_POINT('Ctrl Pts',(1.67645665656929,-222.026329680502,17.5668764061811));
#82529=CARTESIAN_POINT('Ctrl Pts',(3.4075511090259,-224.795506657551,17.4081185409493));
#82530=CARTESIAN_POINT('Ctrl Pts',(2.02005480534486,-227.751835807151,17.2493606757176));
#82531=CARTESIAN_POINT('Ctrl Pts',(-1.21619552005003,-228.189684996505,
17.0906028104857));
#82532=CARTESIAN_POINT('Ctrl Pts',(-3.33938378123961,-225.70833457184,16.931844945254));
#82533=CARTESIAN_POINT('Ctrl Pts',(-2.40636812341,-222.578716389973,16.7730870800222));
#82534=CARTESIAN_POINT('Ctrl Pts',(0.728955539567609,-221.665056865358,
16.6143292147904));
#82535=CARTESIAN_POINT('Ctrl Pts',(3.19713912473123,-223.803537170082,16.4555713495586));
#82536=CARTESIAN_POINT('Ctrl Pts',(2.73930110702426,-227.037020207896,16.2968134843268));
#82537=CARTESIAN_POINT('Ctrl Pts',(-0.225545175302894,-228.406222432435,
16.138055619095));
#82538=CARTESIAN_POINT('Ctrl Pts',(-2.98397252246004,-226.658050020319,
15.9792977538632));
#82539=CARTESIAN_POINT('Ctrl Pts',(-3.01146833420773,-223.392430295024,
15.8205398886314));
#82540=CARTESIAN_POINT('Ctrl Pts',(-0.282868445008073,-221.5980583004,15.6617820233996));
#82541=CARTESIAN_POINT('Ctrl Pts',(2.70461263398692,-222.917143215525,15.5030241581679));
#82542=CARTESIAN_POINT('Ctrl Pts',(3.21683233669003,-226.142458577869,15.344266292936));
#82543=CARTESIAN_POINT('Ctrl Pts',(0.785007211364801,-228.322195894686,
15.1855084277043));
#82544=CARTESIAN_POINT('Ctrl Pts',(-2.36525648293751,-227.461459659322,
15.0267505624725));
#82545=CARTESIAN_POINT('Ctrl Pts',(-3.35083753706407,-224.347995640544,
14.8679926972407));
#82546=CARTESIAN_POINT('Ctrl Pts',(-1.26973220903945,-221.831245985899,
14.7092348320089));
#82547=CARTESIAN_POINT('Ctrl Pts',(1.97343198676774,-222.214539880352,14.5504769667771));
#82548=CARTESIAN_POINT('Ctrl Pts',(3.41051130588809,-225.14708676677,14.3917191015453));
#82549=CARTESIAN_POINT('Ctrl Pts',(1.72629081197493,-227.945019850025,14.2329612363135));
#82550=CARTESIAN_POINT('Ctrl Pts',(-1.53783096517303,-228.047670882347,
14.0742033710817));
#82551=CARTESIAN_POINT('Ctrl Pts',(-3.39452990346833,-225.361093642992,
13.9154455058499));
#82552=CARTESIAN_POINT('Ctrl Pts',(-2.14455520759608,-222.34404351577,13.7566876406181));
#82553=CARTESIAN_POINT('Ctrl Pts',(1.06811632993552,-221.757724658473,13.5979297753863));
#82554=CARTESIAN_POINT('Ctrl Pts',(3.30324784431278,-224.138736066242,13.4391719101545));
#82555=CARTESIAN_POINT('Ctrl Pts',(2.51524706147206,-227.307976192318,13.2804140449227));
#82556=CARTESIAN_POINT('Ctrl Pts',(-0.574707733118198,-228.364956597944,
13.121656179691));
#82557=CARTESIAN_POINT('Ctrl Pts',(-3.13869003295852,-226.342328857455,
12.9628983144591));
#82558=CARTESIAN_POINT('Ctrl Pts',(-2.83014333806119,-223.091201799409,
12.8041404492274));
#82559=CARTESIAN_POINT('Ctrl Pts',(0.0685504285370491,-221.587006779483,
12.6453825839956));
#82560=CARTESIAN_POINT('Ctrl Pts',(2.90450684563386,-223.206383020761,12.4866247187638));
#82561=CARTESIAN_POINT('Ctrl Pts',(3.08225871182353,-226.467277450906,12.327866853532));
#82562=CARTESIAN_POINT('Ctrl Pts',(0.439127526159182,-228.385319615682,
12.1691089883002));
#82563=CARTESIAN_POINT('Ctrl Pts',(-2.60589315417777,-227.20511740131,12.0103511230684));
#82564=CARTESIAN_POINT('Ctrl Pts',(-3.2660005222855,-224.006791827973,11.8515932578366));
#82565=CARTESIAN_POINT('Ctrl Pts',(-0.937064340829889,-221.717450334619,
11.6928353926048));
#82566=CARTESIAN_POINT('Ctrl Pts',(2.24947308850407,-222.432298165938,11.534077527373));
#82567=CARTESIAN_POINT('Ctrl Pts',(3.3772928356975,-225.497106614819,11.3753196621412));
#82568=CARTESIAN_POINT('Ctrl Pts',(1.41421431246939,-228.106963109365,11.2165617969094));
#82569=CARTESIAN_POINT('Ctrl Pts',(-1.84315309391807,-227.8733270884,11.0578039316776));
#82570=CARTESIAN_POINT('Ctrl Pts',(-3.41366686123195,-225.010022229121,
10.8990460664459));
#82571=CARTESIAN_POINT('Ctrl Pts',(-1.85999285138554,-222.137545026145,
10.7402882012141));
#82572=CARTESIAN_POINT('Ctrl Pts',(1.39594654290646,-221.884786502678,10.5815303359823));
#82573=CARTESIAN_POINT('Ctrl Pts',(3.37431571602475,-224.483071249457,10.4227724707505));
#82574=CARTESIAN_POINT('Ctrl Pts',(2.26451127852891,-227.554449168405,10.2640146055187));
#82575=CARTESIAN_POINT('Ctrl Pts',(-0.917773792026828,-228.28799530888,
10.1052567402869));
#82576=CARTESIAN_POINT('Ctrl Pts',(-3.2601123242102,-226.012368271965,9.9464988750551));
#82577=CARTESIAN_POINT('Ctrl Pts',(-2.61879618547721,-222.810221832358,
9.7877410098233));
#82578=CARTESIAN_POINT('Ctrl Pts',(0.419242119222859,-221.612160285666,
9.62898314459151));
#82579=CARTESIAN_POINT('Ctrl Pts',(3.07359005289646,-223.514649512308,9.47022527935973));
#82580=CARTESIAN_POINT('Ctrl Pts',(2.91498849102523,-226.776531446877,9.31146741412793));
#82581=CARTESIAN_POINT('Ctrl Pts',(0.0885895767968314,-228.412531871123,
9.15270954889614));
#82582=CARTESIAN_POINT('Ctrl Pts',(-2.81888651463232,-226.925383261113,
8.99395168366434));
#82583=CARTESIAN_POINT('Ctrl Pts',(-3.14651777871999,-223.676123966246,
8.83519381843255));
#82584=CARTESIAN_POINT('Ctrl Pts',(-0.594456095456926,-221.63847596541,
8.67643595320076));
#82585=CARTESIAN_POINT('Ctrl Pts',(2.50165178299187,-222.677294628843,8.51767808796896));
#82586=CARTESIAN_POINT('Ctrl Pts',(3.30824804802161,-225.84185315662,8.35892022273718));
#82587=CARTESIAN_POINT('Ctrl Pts',(1.08713582959566,-228.235947708564,8.20016235750538));
#82588=CARTESIAN_POINT('Ctrl Pts',(-2.12892305732567,-227.66850304488,8.04140449227359));
#82589=CARTESIAN_POINT('Ctrl Pts',(-3.3965916459004,-224.658844499459,7.8826466270418));
#82590=CARTESIAN_POINT('Ctrl Pts',(-1.55569969371482,-221.961411454717,
7.72388876181));
#82591=CARTESIAN_POINT('Ctrl Pts',(1.70896855698215,-222.044894527128,7.56513089657821));
#82592=CARTESIAN_POINT('Ctrl Pts',(3.40958885153262,-224.832890012105,7.40637303134642));
#82593=CARTESIAN_POINT('Ctrl Pts',(1.98975356323926,-227.773824551432,7.24761516611463));
#82594=CARTESIAN_POINT('Ctrl Pts',(-1.25110410788551,-228.176154970366,
7.08885730088283));
#82595=CARTESIAN_POINT('Ctrl Pts',(-3.34695134867194,-225.671668485321,
6.93009943565104));
#82596=CARTESIAN_POINT('Ctrl Pts',(-2.37966884676946,-222.552471028922,
6.77134157041925));
#82597=CARTESIAN_POINT('Ctrl Pts',(0.765486490118206,-221.673251990608,
6.61258370518745));
#82598=CARTESIAN_POINT('Ctrl Pts',(3.21006862135173,-223.838672599668,6.45382583995566));
#82599=CARTESIAN_POINT('Ctrl Pts',(2.71679607655705,-227.066939999844,6.29506797472387));
#82600=CARTESIAN_POINT('Ctrl Pts',(-0.262888130667251,-228.403543993443,
6.13631010949208));
#82601=CARTESIAN_POINT('Ctrl Pts',(-3.00197713104269,-226.625224658085,
5.97755224426029));
#82602=CARTESIAN_POINT('Ctrl Pts',(-2.99365677913774,-223.359499779557,
5.81879437902849));
#82603=CARTESIAN_POINT('Ctrl Pts',(-0.245541860688655,-221.595160638268,
5.66003651379671));
#82604=CARTESIAN_POINT('Ctrl Pts',(2.72729295900699,-222.946930346944,5.50127864856491));
#82605=CARTESIAN_POINT('Ctrl Pts',(3.20410936986766,-226.177669321362,5.34252078333311));
#82606=CARTESIAN_POINT('Ctrl Pts',(0.748525011423917,-228.33060537918,5.18376291810133));
#82607=CARTESIAN_POINT('Ctrl Pts',(-2.39210940803985,-227.435371524945,
5.02500505286953));
#82608=CARTESIAN_POINT('Ctrl Pts',(-3.34348539133322,-224.311285746851,
4.86624718763774));
#82609=CARTESIAN_POINT('Ctrl Pts',(-1.23490367595725,-221.817511226152,
4.70748932240594));
#82610=CARTESIAN_POINT('Ctrl Pts',(2.00386183509223,-222.236350306138,4.54873145717416));
#82611=CARTESIAN_POINT('Ctrl Pts',(3.4086930734676,-225.184481477252,4.38997359194236));
#82612=CARTESIAN_POINT('Ctrl Pts',(1.69388854504428,-227.963775207674,4.23121572671057));
#82613=CARTESIAN_POINT('Ctrl Pts',(-1.57116271318341,-228.03062198451,4.07245786147877));
#82614=CARTESIAN_POINT('Ctrl Pts',(-3.3982859181096,-225.323843640441,3.91369999624699));
#82615=CARTESIAN_POINT('Ctrl Pts',(-2.11529798437666,-222.320683609087,
3.75494213101519));
#82616=CARTESIAN_POINT('Ctrl Pts',(1.10361058139527,-221.76963383392,3.5961842657834));
#82617=CARTESIAN_POINT('Ctrl Pts',(3.31249478663612,-224.17501504573,3.4374264005516));
#82618=CARTESIAN_POINT('Ctrl Pts',(2.48978389307636,-227.33542245766,3.27866853531981));
#82619=CARTESIAN_POINT('Ctrl Pts',(-0.611577120844398,-228.358451323275,
3.11991067008802));
#82620=CARTESIAN_POINT('Ctrl Pts',(-3.1532227791871,-226.307825679854,2.96115280485623));
#82621=CARTESIAN_POINT('Ctrl Pts',(-2.80903907123482,-223.060278005436,
2.80239493962444));
#82622=CARTESIAN_POINT('Ctrl Pts',(0.105977078601933,-221.587963865238,
2.64363707439264));
#82623=CARTESIAN_POINT('Ctrl Pts',(2.92400302173803,-223.238344977983,2.48487920916086));
#82624=CARTESIAN_POINT('Ctrl Pts',(3.06598149107159,-226.500992867014,2.32612134392906));
#82625=CARTESIAN_POINT('Ctrl Pts',(0.401973867646657,-228.389931799117,
2.16736347869727));
#82626=CARTESIAN_POINT('Ctrl Pts',(-2.62992031971121,-227.176405980739,
2.00860561346547));
#82627=CARTESIAN_POINT('Ctrl Pts',(-3.25491133877711,-223.971032075231,
1.84984774823368));
#82628=CARTESIAN_POINT('Ctrl Pts',(-0.901008024848114,-221.707372456188,
1.69108988300189));
#82629=CARTESIAN_POINT('Ctrl Pts',(2.2774986027622,-222.457119582258,1.53233201777009));
#82630=CARTESIAN_POINT('Ctrl Pts',(3.37163696425009,-225.534122654706,1.37357415253831));
#82631=CARTESIAN_POINT('Ctrl Pts',(1.38005662806585,-228.12227255076,1.21481628730651));
#82632=CARTESIAN_POINT('Ctrl Pts',(-1.87455822137116,-227.852967765532,
1.05605842207472));
#82633=CARTESIAN_POINT('Ctrl Pts',(-3.41356376877976,-224.97252740804,0.897300556842932));
#82634=CARTESIAN_POINT('Ctrl Pts',(-1.82850369573622,-222.117432216889,
0.738542691611134));
#82635=CARTESIAN_POINT('Ctrl Pts',(1.43005935989245,-221.900052186656,0.579784826379344));
#82636=CARTESIAN_POINT('Ctrl Pts',(3.37971747316782,-224.520578545184,0.421026961147552));
#82637=CARTESIAN_POINT('Ctrl Pts',(2.23649101368354,-227.578176481406,0.262269095915755));
#82638=CARTESIAN_POINT('Ctrl Pts',(-0.954039042100929,-228.279681514165,
0.103511230683968));
#82639=CARTESIAN_POINT('Ctrl Pts',(-3.27049270054663,-225.972504524796,
-0.0552466345478283));
#82640=CARTESIAN_POINT('Ctrl Pts',(-2.81925737956186,-223.853043319762,
-0.161085211369022));
#82641=CARTESIAN_POINT('Ctrl Pts',(-2.19519710401913,-223.123136560921,
-0.21400449977962));
#82642=CARTESIAN_POINT('Ctrl Pts',(-0.698066426161038,-227.611132185939,
20.2140044997796));
#82643=CARTESIAN_POINT('Ctrl Pts',(-1.56627230491967,-227.379023915733,
20.161085211369));
#82644=CARTESIAN_POINT('Ctrl Pts',(-3.03778533319432,-225.983650973587,
20.0552466345478));
#82645=CARTESIAN_POINT('Ctrl Pts',(-2.47430970641492,-222.976375369272,
19.896488769316));
#82646=CARTESIAN_POINT('Ctrl Pts',(0.358151943839997,-221.826111965074,
19.7377309040843));
#82647=CARTESIAN_POINT('Ctrl Pts',(2.86064170592173,-223.578174499175,19.5789730388525));
#82648=CARTESIAN_POINT('Ctrl Pts',(2.74615023855165,-226.632675463776,19.4202151736207));
#82649=CARTESIAN_POINT('Ctrl Pts',(0.117851501550342,-228.192369288497,
19.2614573083889));
#82650=CARTESIAN_POINT('Ctrl Pts',(-2.61804363116637,-226.830693717159,
19.1026994431571));
#82651=CARTESIAN_POINT('Ctrl Pts',(-2.95803399248552,-223.793426087799,
18.9439415779253));
#82652=CARTESIAN_POINT('Ctrl Pts',(-0.590768411472084,-221.860484399872,
18.7851837126935));
#82653=CARTESIAN_POINT('Ctrl Pts',(2.31713720451145,-222.800793023077,18.6264258474617));
#82654=CARTESIAN_POINT('Ctrl Pts',(3.10441430051404,-225.753832645653,18.4676679822299));
#82655=CARTESIAN_POINT('Ctrl Pts',(1.05052398848132,-228.016956358674,18.3089101169981));
#82656=CARTESIAN_POINT('Ctrl Pts',(-1.96480211294228,-227.518965818607,
18.1501522517663));
#82657=CARTESIAN_POINT('Ctrl Pts',(-3.1819432312892,-224.715615847668,17.9913943865345));
#82658=CARTESIAN_POINT('Ctrl Pts',(-1.48696912673618,-222.172535232803,
17.8326365213027));
#82659=CARTESIAN_POINT('Ctrl Pts',(1.56887861963092,-222.217149773714,17.673878656071));
#82660=CARTESIAN_POINT('Ctrl Pts',(3.1888889338723,-224.808628972561,17.5151207908391));
#82661=CARTESIAN_POINT('Ctrl Pts',(1.89042811346746,-227.575250809889,17.3563629256074));
#82662=CARTESIAN_POINT('Ctrl Pts',(-1.13815238898098,-227.985003265527,
17.1976050603756));
#82663=CARTESIAN_POINT('Ctrl Pts',(-3.12509589591799,-225.662880821255,
17.0388471951438));
#82664=CARTESIAN_POINT('Ctrl Pts',(-2.25195174893761,-222.73408988956,16.880089329912));
#82665=CARTESIAN_POINT('Ctrl Pts',(0.682178543780247,-221.879059794881,
16.7213314646802));
#82666=CARTESIAN_POINT('Ctrl Pts',(2.9919790631754,-223.880314056623,16.5625735994484));
#82667=CARTESIAN_POINT('Ctrl Pts',(2.56352046007342,-226.906304848026,16.4038157342166));
#82668=CARTESIAN_POINT('Ctrl Pts',(-0.211071966523578,-228.18764551831,
16.2450578689848));
#82669=CARTESIAN_POINT('Ctrl Pts',(-2.79249133803074,-226.551653135178,
16.086300003753));
#82670=CARTESIAN_POINT('Ctrl Pts',(-2.81822274660089,-223.49558786395,15.9275421385212));
#82671=CARTESIAN_POINT('Ctrl Pts',(-0.264716808396092,-221.816360520376,
15.7687842732894));
#82672=CARTESIAN_POINT('Ctrl Pts',(2.5310579424875,-223.050799903409,15.6100264080577));
#82673=CARTESIAN_POINT('Ctrl Pts',(3.01040856391611,-226.069147138167,15.4512685428258));
#82674=CARTESIAN_POINT('Ctrl Pts',(0.73463338604091,-228.10901095413,15.2925106775941));
#82675=CARTESIAN_POINT('Ctrl Pts',(-2.21347823785548,-227.303508067126,
15.1337528123623));
#82676=CARTESIAN_POINT('Ctrl Pts',(-3.13581466550684,-224.389834687674,
14.9749949471305));
#82677=CARTESIAN_POINT('Ctrl Pts',(-1.18825363460054,-222.034584578067,
14.8162370818987));
#82678=CARTESIAN_POINT('Ctrl Pts',(1.84679707596586,-222.393282546002,14.6574792166669));
#82679=CARTESIAN_POINT('Ctrl Pts',(3.19165917523153,-225.137648225328,14.4987213514351));
#82680=CARTESIAN_POINT('Ctrl Pts',(1.61551492283441,-227.756038254248,14.3399634862033));
#82681=CARTESIAN_POINT('Ctrl Pts',(-1.43914852341226,-227.852102181258,
14.1812056209715));
#82682=CARTESIAN_POINT('Ctrl Pts',(-3.17670329762513,-225.337922304137,
14.0224477557397));
#82683=CARTESIAN_POINT('Ctrl Pts',(-2.00693933877233,-222.514475947559,
13.8636898905079));
#82684=CARTESIAN_POINT('Ctrl Pts',(0.999575424003943,-221.965781106033,
13.7049320252761));
#82685=CARTESIAN_POINT('Ctrl Pts',(3.09127879803915,-224.194003276949,13.5461741600443));
#82686=CARTESIAN_POINT('Ctrl Pts',(2.35384393767052,-227.159873617105,13.3874162948125));
#82687=CARTESIAN_POINT('Ctrl Pts',(-0.537828801891506,-228.149027707822,
13.2286584295808));
#82688=CARTESIAN_POINT('Ctrl Pts',(-2.93728064311203,-226.256191764173,
13.069900564349));
#82689=CARTESIAN_POINT('Ctrl Pts',(-2.64853335526218,-223.213689167351,
12.9111426991172));
#82690=CARTESIAN_POINT('Ctrl Pts',(0.0641515551725655,-221.806018174325,
12.7523848338854));
#82691=CARTESIAN_POINT('Ctrl Pts',(2.71812496483608,-223.321479222556,12.5936269686536));
#82692=CARTESIAN_POINT('Ctrl Pts',(2.88447051356929,-226.373122420298,12.4348691034218));
#82693=CARTESIAN_POINT('Ctrl Pts',(0.410948761712932,-228.16808403298,12.27611123819));
#82694=CARTESIAN_POINT('Ctrl Pts',(-2.43867328070292,-227.063615263261,
12.1173533729582));
#82695=CARTESIAN_POINT('Ctrl Pts',(-3.05642163251797,-224.070525885755,
11.9585955077264));
#82696=CARTESIAN_POINT('Ctrl Pts',(-0.876933026443435,-221.928091181056,
11.7998376424946));
#82697=CARTESIAN_POINT('Ctrl Pts',(2.10512465094758,-222.597067306654,11.6410797772628));
#82698=CARTESIAN_POINT('Ctrl Pts',(3.16057233057339,-225.46520733871,11.482321912031));
#82699=CARTESIAN_POINT('Ctrl Pts',(1.32346433754493,-227.907589632672,11.3235640467992));
#82700=CARTESIAN_POINT('Ctrl Pts',(-1.72487816516068,-227.688946009151,
11.1648061815675));
#82701=CARTESIAN_POINT('Ctrl Pts',(-3.19461223894042,-225.009379103795,
11.0060483163357));
#82702=CARTESIAN_POINT('Ctrl Pts',(-1.74063731726696,-222.321228443015,
10.8472904511039));
#82703=CARTESIAN_POINT('Ctrl Pts',(1.30636880872031,-222.084689405847,10.6885325858721));
#82704=CARTESIAN_POINT('Ctrl Pts',(3.15778625233847,-224.516242509807,10.5297747206403));
#82705=CARTESIAN_POINT('Ctrl Pts',(2.11919784199338,-227.390530449768,10.3710168554085));
#82706=CARTESIAN_POINT('Ctrl Pts',(-0.858880350008606,-228.077005016107,
10.2122589901767));
#82707=CARTESIAN_POINT('Ctrl Pts',(-3.05091127945738,-225.947404712705,
10.0535011249449));
#82708=CARTESIAN_POINT('Ctrl Pts',(-2.45074832592093,-222.950739653492,
9.89474325971312));
#82709=CARTESIAN_POINT('Ctrl Pts',(0.392339399125002,-221.829557582818,
9.73598539448132));
#82710=CARTESIAN_POINT('Ctrl Pts',(2.87635812152011,-223.609964287674,9.57722752924953));
#82711=CARTESIAN_POINT('Ctrl Pts',(2.72793400421006,-226.66253162179,9.41846966401774));
#82712=CARTESIAN_POINT('Ctrl Pts',(0.0829047935203504,-228.193550081021,
9.25971179878595));
#82713=CARTESIAN_POINT('Ctrl Pts',(-2.63799888093902,-226.801831631685,
9.10095393355415));
#82714=CARTESIAN_POINT('Ctrl Pts',(-2.94460608329979,-223.761076943886,
8.94219606832236));
#82715=CARTESIAN_POINT('Ctrl Pts',(-0.556309914018403,-221.854184588324,
8.78343820309057));
#82716=CARTESIAN_POINT('Ctrl Pts',(2.34112106669625,-222.826342373821,8.62468033785877));
#82717=CARTESIAN_POINT('Ctrl Pts',(3.09595813923287,-225.78783153332,8.46592247262699));
#82718=CARTESIAN_POINT('Ctrl Pts',(1.01737444448917,-228.028297304506,8.30716460739519));
#82719=CARTESIAN_POINT('Ctrl Pts',(-1.99231030184375,-227.497265501692,
8.14840674216339));
#82720=CARTESIAN_POINT('Ctrl Pts',(-3.17863273827496,-224.680736409933,
7.98964887693161));
#82721=CARTESIAN_POINT('Ctrl Pts',(-1.45587061763363,-222.156397343248,
7.83089101169982));
#82722=CARTESIAN_POINT('Ctrl Pts',(1.59930423501526,-222.234523316201,7.67213314646802));
#82723=CARTESIAN_POINT('Ctrl Pts',(3.19079591466932,-224.843613441417,7.51337528123624));
#82724=CARTESIAN_POINT('Ctrl Pts',(1.862071298693,-227.595828538898,7.35461741600443));
#82725=CARTESIAN_POINT('Ctrl Pts',(-1.17082089662297,-227.972341459659,
7.19585955077264));
#82726=CARTESIAN_POINT('Ctrl Pts',(-3.13217785339102,-225.628567593424,
7.03710168554085));
#82727=CARTESIAN_POINT('Ctrl Pts',(-2.2269657619055,-222.709528690405,6.87834382030906));
#82728=CARTESIAN_POINT('Ctrl Pts',(0.716365307302614,-221.886729039857,
6.71958595507727));
#82729=CARTESIAN_POINT('Ctrl Pts',(3.00407887543776,-223.913194849605,6.56082808984548));
#82730=CARTESIAN_POINT('Ctrl Pts',(2.54245957490482,-226.934304690257,6.40207022461368));
#82731=CARTESIAN_POINT('Ctrl Pts',(-0.246018628601239,-228.18513895445,
6.24331235938189));
#82732=CARTESIAN_POINT('Ctrl Pts',(-2.80934059288588,-226.520934172783,
6.08455449415009));
#82733=CARTESIAN_POINT('Ctrl Pts',(-2.80155415703599,-223.464770495994,
5.9257966289183));
#82734=CARTESIAN_POINT('Ctrl Pts',(-0.22978546683524,-221.8136488009,5.76703876368652));
#82735=CARTESIAN_POINT('Ctrl Pts',(2.55228287357704,-223.078675597922,5.60828089845472));
#82736=CARTESIAN_POINT('Ctrl Pts',(2.99850202845772,-226.102098412171,5.44952303322292));
#82737=CARTESIAN_POINT('Ctrl Pts',(0.700492244807063,-228.116880802941,
5.29076516799113));
#82738=CARTESIAN_POINT('Ctrl Pts',(-2.23860801374472,-227.279094005426,
5.13200730275934));
#82739=CARTESIAN_POINT('Ctrl Pts',(-3.1289343061487,-224.355480463771,4.97324943752755));
#82740=CARTESIAN_POINT('Ctrl Pts',(-1.15566004460723,-222.021731176323,
4.81449157229576));
#82741=CARTESIAN_POINT('Ctrl Pts',(1.87527424431247,-222.413693399195,4.65573370706397));
#82742=CARTESIAN_POINT('Ctrl Pts',(3.18995761858296,-225.172643321403,4.49697584183217));
#82743=CARTESIAN_POINT('Ctrl Pts',(1.58519190576392,-227.773590082685,4.33821797660038));
#82744=CARTESIAN_POINT('Ctrl Pts',(-1.4703413768651,-227.836147309296,4.17946011136858));
#82745=CARTESIAN_POINT('Ctrl Pts',(-3.1802182892252,-225.303062630102,4.0207022461368));
#82746=CARTESIAN_POINT('Ctrl Pts',(-1.9795595483084,-222.492615043485,3.861944380905));
#82747=CARTESIAN_POINT('Ctrl Pts',(1.03279201330066,-221.976926071019,3.70318651567321));
#82748=CARTESIAN_POINT('Ctrl Pts',(3.09993236510347,-224.227954238364,3.54442865044142));
#82749=CARTESIAN_POINT('Ctrl Pts',(2.33001473795483,-227.185558658658,3.38567078520963));
#82750=CARTESIAN_POINT('Ctrl Pts',(-0.572332285113605,-228.142939875904,
3.22691291997783));
#82751=CARTESIAN_POINT('Ctrl Pts',(-2.95088082463369,-226.223902651636,
3.06815505474604));
#82752=CARTESIAN_POINT('Ctrl Pts',(-2.62878334688759,-223.184749749793,
2.90939718951425));
#82753=CARTESIAN_POINT('Ctrl Pts',(0.0991765412711432,-221.806913843993,
2.75063932428246));
#82754=CARTESIAN_POINT('Ctrl Pts',(2.73637007349101,-223.351390184544,2.59188145905066));
#82755=CARTESIAN_POINT('Ctrl Pts',(2.86923780026014,-226.404674321909,2.43312359381887));
#82756=CARTESIAN_POINT('Ctrl Pts',(0.376179249329203,-228.172400253118,
2.27436572858708));
#82757=CARTESIAN_POINT('Ctrl Pts',(-2.46115862570008,-227.03674625135,2.11560786335528));
#82758=CARTESIAN_POINT('Ctrl Pts',(-3.04604404068027,-224.037060832363,
1.95684999812349));
#82759=CARTESIAN_POINT('Ctrl Pts',(-0.843190440242474,-221.918659998961,
1.7980921328917));
#82760=CARTESIAN_POINT('Ctrl Pts',(2.13135177107707,-222.620295935454,1.6393342676599));
#82761=CARTESIAN_POINT('Ctrl Pts',(3.15527939576685,-225.499848063441,1.48057640242812));
#82762=CARTESIAN_POINT('Ctrl Pts',(1.29149854794529,-227.921916668918,1.32181853719632));
#82763=CARTESIAN_POINT('Ctrl Pts',(-1.75426802908282,-227.669893141764,
1.16306067196453));
#82764=CARTESIAN_POINT('Ctrl Pts',(-3.19451576191941,-224.974290321206,
1.00430280673274));
#82765=CARTESIAN_POINT('Ctrl Pts',(-1.71116881722859,-222.302406270488,
0.845544941500944));
#82766=CARTESIAN_POINT('Ctrl Pts',(1.33829261003958,-222.098975492584,0.686787076269154));
#82767=CARTESIAN_POINT('Ctrl Pts',(3.16284137932728,-224.551342966544,0.528029211037361));
#82768=CARTESIAN_POINT('Ctrl Pts',(2.09297563442241,-227.412735183736,0.369271345805565));
#82769=CARTESIAN_POINT('Ctrl Pts',(-0.892818463024459,-228.069224716672,
0.210513480573778));
#82770=CARTESIAN_POINT('Ctrl Pts',(-3.0606255482004,-225.910099017751,0.0517556153419817));
#82771=CARTESIAN_POINT('Ctrl Pts',(-2.63834594750734,-223.926643402192,
-0.0540829614792118));
#82772=CARTESIAN_POINT('Ctrl Pts',(-2.0543315503421,-223.243574678773,-0.10700224988981));
#82773=CARTESIAN_POINT('Ctrl Pts',(-0.65019999797512,-227.432086802035,
20.3210067496694));
#82774=CARTESIAN_POINT('Ctrl Pts',(-1.45887298303087,-227.215894200354,
20.2680874612588));
#82775=CARTESIAN_POINT('Ctrl Pts',(-2.82948433482767,-225.916202007525,
20.1622488844376));
#82776=CARTESIAN_POINT('Ctrl Pts',(-2.30464624254778,-223.115135348884,
20.0034910192059));
#82777=CARTESIAN_POINT('Ctrl Pts',(0.333593458204553,-222.0437455283,19.844733153974));
#82778=CARTESIAN_POINT('Ctrl Pts',(2.66448744946339,-223.675669100946,19.6859752887423));
#82779=CARTESIAN_POINT('Ctrl Pts',(2.55784666419947,-226.520722876015,19.5272174235105));
#82780=CARTESIAN_POINT('Ctrl Pts',(0.109770421836213,-227.97346846536,19.3684595582787));
#82781=CARTESIAN_POINT('Ctrl Pts',(-2.43852432933144,-226.705163013978,
19.2097016930469));
#82782=CARTESIAN_POINT('Ctrl Pts',(-2.75520154507576,-223.876160884024,
19.0509438278151));
#82783=CARTESIAN_POINT('Ctrl Pts',(-0.550259410204463,-222.075761044586,
18.8921859625833));
#82784=CARTESIAN_POINT('Ctrl Pts',(2.1582510621043,-222.951592687525,18.7334280973515));
#82785=CARTESIAN_POINT('Ctrl Pts',(2.89154455258461,-225.702142326731,18.5746702321197));
#82786=CARTESIAN_POINT('Ctrl Pts',(0.978489538509605,-227.810083603489,
18.4159123668879));
#82787=CARTESIAN_POINT('Ctrl Pts',(-1.83007559449918,-227.346240284273,
18.2571545016561));
#82788=CARTESIAN_POINT('Ctrl Pts',(-2.96375732309449,-224.735116074429,
18.0983966364243));
#82789=CARTESIAN_POINT('Ctrl Pts',(-1.38500762529136,-222.366414545939,
17.9396387711926));
#82790=CARTESIAN_POINT('Ctrl Pts',(1.46130058269256,-222.407969866927,17.7808809059608));
#82791=CARTESIAN_POINT('Ctrl Pts',(2.97022675871869,-224.821751287571,17.6221230407289));
#82792=CARTESIAN_POINT('Ctrl Pts',(1.76080142159005,-227.398665812627,17.4633651754972));
#82793=CARTESIAN_POINT('Ctrl Pts',(-1.06010925791193,-227.780321534549,
17.3046073102654));
#82794=CARTESIAN_POINT('Ctrl Pts',(-2.91080801059636,-225.61742707067,17.1458494450336));
#82795=CARTESIAN_POINT('Ctrl Pts',(-2.09753537446523,-222.889463389148,
16.9870915798018));
#82796=CARTESIAN_POINT('Ctrl Pts',(0.635401547992891,-222.093062724406,
16.82833371457));
#82797=CARTESIAN_POINT('Ctrl Pts',(2.78681900161956,-223.957090943164,16.6695758493382));
#82798=CARTESIAN_POINT('Ctrl Pts',(2.38773981312259,-226.775589488157,16.5108179841064));
#82799=CARTESIAN_POINT('Ctrl Pts',(-0.196598757744262,-227.969068604185,
16.3520601188746));
#82800=CARTESIAN_POINT('Ctrl Pts',(-2.60101015360142,-226.445256250038,
16.1933022536428));
#82801=CARTESIAN_POINT('Ctrl Pts',(-2.62497715899404,-223.598745432877,
16.034544388411));
#82802=CARTESIAN_POINT('Ctrl Pts',(-0.246565171784112,-222.034662740351,
15.8757865231792));
#82803=CARTESIAN_POINT('Ctrl Pts',(2.35750325098809,-223.184456591293,15.7170286579475));
#82804=CARTESIAN_POINT('Ctrl Pts',(2.80398479114218,-225.995835698465,15.5582707927156));
#82805=CARTESIAN_POINT('Ctrl Pts',(0.684259560717021,-227.895826013575,
15.3995129274839));
#82806=CARTESIAN_POINT('Ctrl Pts',(-2.06169999277346,-227.14555647493,15.2407550622521));
#82807=CARTESIAN_POINT('Ctrl Pts',(-2.9207917939496,-224.431673734804,15.0819971970203));
#82808=CARTESIAN_POINT('Ctrl Pts',(-1.10677506016163,-222.237923170235,
14.9232393317885));
#82809=CARTESIAN_POINT('Ctrl Pts',(1.72016216516399,-222.572025211652,14.7644814665567));
#82810=CARTESIAN_POINT('Ctrl Pts',(2.97280704457497,-225.128209683886,14.6057236013249));
#82811=CARTESIAN_POINT('Ctrl Pts',(1.50473903369388,-227.56705665847,14.4469657360931));
#82812=CARTESIAN_POINT('Ctrl Pts',(-1.34046608165149,-227.656533480169,
14.2882078708613));
#82813=CARTESIAN_POINT('Ctrl Pts',(-2.95887669178193,-225.314750965283,
14.1294500056295));
#82814=CARTESIAN_POINT('Ctrl Pts',(-1.86932346994857,-222.684908379347,
13.9706921403977));
#82815=CARTESIAN_POINT('Ctrl Pts',(0.931034518072369,-222.173837553594,
13.8119342751659));
#82816=CARTESIAN_POINT('Ctrl Pts',(2.87930975176552,-224.249270487656,13.6531764099341));
#82817=CARTESIAN_POINT('Ctrl Pts',(2.19244081386897,-227.011771041893,13.4944185447024));
#82818=CARTESIAN_POINT('Ctrl Pts',(-0.50094987066481,-227.933098817701,
13.3356606794706));
#82819=CARTESIAN_POINT('Ctrl Pts',(-2.73587125326554,-226.17005467089,13.1769028142388));
#82820=CARTESIAN_POINT('Ctrl Pts',(-2.46692337246317,-223.336176535292,
13.018144949007));
#82821=CARTESIAN_POINT('Ctrl Pts',(0.059752681808081,-222.025029569166,
12.8593870837752));
#82822=CARTESIAN_POINT('Ctrl Pts',(2.53174308403829,-223.436575424352,12.7006292185434));
#82823=CARTESIAN_POINT('Ctrl Pts',(2.68668231531504,-226.27896738969,12.5418713533116));
#82824=CARTESIAN_POINT('Ctrl Pts',(0.382769997266682,-227.950848450278,
12.3831134880798));
#82825=CARTESIAN_POINT('Ctrl Pts',(-2.27145340722807,-226.922113125211,
12.224355622848));
#82826=CARTESIAN_POINT('Ctrl Pts',(-2.84684274275044,-224.134259943536,
12.0655977576162));
#82827=CARTESIAN_POINT('Ctrl Pts',(-0.816801712056979,-222.138732027492,
11.9068398923844));
#82828=CARTESIAN_POINT('Ctrl Pts',(1.96077621339108,-222.761836447371,11.7480820271526));
#82829=CARTESIAN_POINT('Ctrl Pts',(2.94385182544929,-225.433308062602,11.5893241619208));
#82830=CARTESIAN_POINT('Ctrl Pts',(1.23271436262047,-227.708216155979,11.4305662966891));
#82831=CARTESIAN_POINT('Ctrl Pts',(-1.60660323640329,-227.504564929902,
11.2718084314573));
#82832=CARTESIAN_POINT('Ctrl Pts',(-2.97555761664889,-225.008735978468,
11.1130505662255));
#82833=CARTESIAN_POINT('Ctrl Pts',(-1.62128178314839,-222.504911859884,
10.9542927009937));
#82834=CARTESIAN_POINT('Ctrl Pts',(1.21679107453415,-222.284592309017,10.7955348357619));
#82835=CARTESIAN_POINT('Ctrl Pts',(2.94125678865219,-224.549413770157,10.6367769705301));
#82836=CARTESIAN_POINT('Ctrl Pts',(1.97388440545785,-227.22661173113,10.4780191052983));
#82837=CARTESIAN_POINT('Ctrl Pts',(-0.799986907990383,-227.866014723333,
10.3192612400665));
#82838=CARTESIAN_POINT('Ctrl Pts',(-2.84171023470455,-225.882441153445,
10.1605033748347));
#82839=CARTESIAN_POINT('Ctrl Pts',(-2.28270046636465,-223.091257474625,
10.0017455096029));
#82840=CARTESIAN_POINT('Ctrl Pts',(0.365436679027144,-222.046954879969,
9.84298764437113));
#82841=CARTESIAN_POINT('Ctrl Pts',(2.67912619014375,-223.70527906304,9.68422977913934));
#82842=CARTESIAN_POINT('Ctrl Pts',(2.54087951739489,-226.548531796703,9.52547191390754));
#82843=CARTESIAN_POINT('Ctrl Pts',(0.0772200102438696,-227.974568290918,
9.36671404867575));
#82844=CARTESIAN_POINT('Ctrl Pts',(-2.45711124724573,-226.678280002257,
9.20795618344397));
#82845=CARTESIAN_POINT('Ctrl Pts',(-2.74269438787959,-223.846029921527,
9.04919831821217));
#82846=CARTESIAN_POINT('Ctrl Pts',(-0.518163732579882,-222.069893211237,
8.89044045298037));
#82847=CARTESIAN_POINT('Ctrl Pts',(2.18059035040062,-222.975390118799,8.73168258774859));
#82848=CARTESIAN_POINT('Ctrl Pts',(2.88366823044413,-225.733809910021,8.57292472251679));
#82849=CARTESIAN_POINT('Ctrl Pts',(0.947613059382676,-227.820646900448,
8.41416685728501));
#82850=CARTESIAN_POINT('Ctrl Pts',(-1.85569754636184,-227.326027958504,
8.2554089920532));
#82851=CARTESIAN_POINT('Ctrl Pts',(-2.96067383064952,-224.702628320407,
8.09665112682142));
#82852=CARTESIAN_POINT('Ctrl Pts',(-1.35604154155244,-222.351383231779,
7.93789326158962));
#82853=CARTESIAN_POINT('Ctrl Pts',(1.48963991304838,-222.424152105273,7.77913539635783));
#82854=CARTESIAN_POINT('Ctrl Pts',(2.97200297780601,-224.854336870728,7.62037753112604));
#82855=CARTESIAN_POINT('Ctrl Pts',(1.73438903414674,-227.417832526365,7.46161966589424));
#82856=CARTESIAN_POINT('Ctrl Pts',(-1.09053768536042,-227.768527948952,
7.30286180066246));
#82857=CARTESIAN_POINT('Ctrl Pts',(-2.91740435811009,-225.585466701527,
7.14410393543065));
#82858=CARTESIAN_POINT('Ctrl Pts',(-2.07426267704153,-222.866586351888,
6.98534607019887));
#82859=CARTESIAN_POINT('Ctrl Pts',(0.667244124487021,-222.100206089107,
6.82658820496707));
#82860=CARTESIAN_POINT('Ctrl Pts',(2.7980891295238,-223.987717099543,6.66783033973529));
#82861=CARTESIAN_POINT('Ctrl Pts',(2.36812307325259,-226.801669380671,6.50907247450349));
#82862=CARTESIAN_POINT('Ctrl Pts',(-0.229149126535227,-227.966733915457,
6.3503146092717));
#82863=CARTESIAN_POINT('Ctrl Pts',(-2.61670405472906,-226.416643687482,
6.19155674403991));
#82864=CARTESIAN_POINT('Ctrl Pts',(-2.60945153493425,-223.570041212431,
6.03279887880811));
#82865=CARTESIAN_POINT('Ctrl Pts',(-0.214029072981824,-222.032136963532,
5.87404101357633));
#82866=CARTESIAN_POINT('Ctrl Pts',(2.37727278814708,-223.2104208489,5.71528314834453));
#82867=CARTESIAN_POINT('Ctrl Pts',(2.79289468704778,-226.026527502981,5.55652528311273));
#82868=CARTESIAN_POINT('Ctrl Pts',(0.652459478190211,-227.903156226702,
5.39776741788094));
#82869=CARTESIAN_POINT('Ctrl Pts',(-2.08510661944959,-227.122816485908,
5.23900955264915));
#82870=CARTESIAN_POINT('Ctrl Pts',(-2.91438322096418,-224.39967518069,5.08025168741736));
#82871=CARTESIAN_POINT('Ctrl Pts',(-1.07641641325721,-222.225951126495,
4.92149382218557));
#82872=CARTESIAN_POINT('Ctrl Pts',(1.7466866535327,-222.591036492251,4.76273595695378));
#82873=CARTESIAN_POINT('Ctrl Pts',(2.97122216369831,-225.160805165555,4.60397809172198));
#82874=CARTESIAN_POINT('Ctrl Pts',(1.47649526648357,-227.583404957696,4.44522022649019));
#82875=CARTESIAN_POINT('Ctrl Pts',(-1.3695200405468,-227.641672634083,4.28646236125839));
#82876=CARTESIAN_POINT('Ctrl Pts',(-2.96215066034079,-225.282281619762,
4.12770449602661));
#82877=CARTESIAN_POINT('Ctrl Pts',(-1.84382111224014,-222.664546477884,
3.96894663079481));
#82878=CARTESIAN_POINT('Ctrl Pts',(0.961973445206051,-222.184218308117,
3.81018876556302));
#82879=CARTESIAN_POINT('Ctrl Pts',(2.88736994357081,-224.280893430997,3.65143090033123));
#82880=CARTESIAN_POINT('Ctrl Pts',(2.1702455828333,-227.035694859655,3.49267303509943));
#82881=CARTESIAN_POINT('Ctrl Pts',(-0.53308744938281,-227.927428428534,
3.33391516986764));
#82882=CARTESIAN_POINT('Ctrl Pts',(-2.74853887008028,-226.139979623417,
3.17515730463585));
#82883=CARTESIAN_POINT('Ctrl Pts',(-2.44852762254036,-223.309221494149,
3.01639943940406));
#82884=CARTESIAN_POINT('Ctrl Pts',(0.0923760039403491,-222.025863822749,
2.85764157417226));
#82885=CARTESIAN_POINT('Ctrl Pts',(2.54873712524399,-223.464435391104,2.69888370894047));
#82886=CARTESIAN_POINT('Ctrl Pts',(2.67249410944869,-226.308355776804,2.54012584370868));
#82887=CARTESIAN_POINT('Ctrl Pts',(0.350384631011751,-227.954868707119,
2.38136797847689));
#82888=CARTESIAN_POINT('Ctrl Pts',(-2.29239693168896,-226.897086521961,
2.22261011324509));
#82889=CARTESIAN_POINT('Ctrl Pts',(-2.83717674258343,-224.103089589495,
2.0638522480133));
#82890=CARTESIAN_POINT('Ctrl Pts',(-0.785372855636834,-222.129947541734,
1.90509438278151));
#82891=CARTESIAN_POINT('Ctrl Pts',(1.98520493939195,-222.78347228865,1.74633651754971));
#82892=CARTESIAN_POINT('Ctrl Pts',(2.9389218272836,-225.465573472176,1.58757865231793));
#82893=CARTESIAN_POINT('Ctrl Pts',(1.20294046782472,-227.721560787075,1.42882078708613));
#82894=CARTESIAN_POINT('Ctrl Pts',(-1.63397783679448,-227.486818517997,
1.27006292185434));
#82895=CARTESIAN_POINT('Ctrl Pts',(-2.97546775505905,-224.976053234372,
1.11130505662255));
#82896=CARTESIAN_POINT('Ctrl Pts',(-1.59383393872096,-222.487380324087,
0.952547191390754));
#82897=CARTESIAN_POINT('Ctrl Pts',(1.24652586018671,-222.297898798513,0.793789326158964));
#82898=CARTESIAN_POINT('Ctrl Pts',(2.94596528548675,-224.582107387905,0.635031460927171));
#82899=CARTESIAN_POINT('Ctrl Pts',(1.94946025516128,-227.247293886066,0.476273595695376));
#82900=CARTESIAN_POINT('Ctrl Pts',(-0.831597883947986,-227.858767919179,
0.317515730463588));
#82901=CARTESIAN_POINT('Ctrl Pts',(-2.85075839585417,-225.847693510707,
0.158757865231792));
#82902=CARTESIAN_POINT('Ctrl Pts',(-2.45743451545282,-224.000243484622,
0.0529192884105984));
#82903=CARTESIAN_POINT('Ctrl Pts',(-1.91346599666507,-223.364012796625,
0.));
#82904=CARTESIAN_POINT('Ctrl Pts',(-1.91346599666507,-223.364012796625,
0.));
#82905=CARTESIAN_POINT('Ctrl Pts',(-1.97507205842691,-223.421907367167,
4.15794293990103E-16));
#82906=CARTESIAN_POINT('Ctrl Pts',(-2.03330667709052,-223.482952904785,
4.29084976747441E-15));
#82907=CARTESIAN_POINT('Ctrl Pts',(-2.08817315626043,-223.546764508293,
4.10782519111308E-15));
#82908=CARTESIAN_POINT('Ctrl Pts',(-2.1444928557844,-223.612266257087,3.91995293646646E-15));
#82909=CARTESIAN_POINT('Ctrl Pts',(-2.19726406808799,-223.680682970755,
1.5045519229708E-16));
#82910=CARTESIAN_POINT('Ctrl Pts',(-2.24646481250915,-223.751646900022,
-2.05391259555654E-15));
#82911=CARTESIAN_POINT('Ctrl Pts',(-2.2973544975264,-223.825046846515,-4.33395091013519E-15));
#82912=CARTESIAN_POINT('Ctrl Pts',(-2.34442495788414,-223.901172411917,
4.72218969058781E-15));
#82913=CARTESIAN_POINT('Ctrl Pts',(-2.38761695660309,-223.979660637394,
5.32907051820075E-15));
#82914=CARTESIAN_POINT('Ctrl Pts',(-2.40651345604263,-224.01399923604,5.59458088028141E-15));
#82915=CARTESIAN_POINT('Ctrl Pts',(-2.42466709995156,-224.048790568658,
4.43801222596687E-15));
#82916=CARTESIAN_POINT('Ctrl Pts',(-2.44207048417908,-224.084006328958,
3.99680288865056E-15));
#82917=CARTESIAN_POINT('Ctrl Pts',(-2.45159432012311,-224.10327781773,3.75535528911235E-15));
#82918=CARTESIAN_POINT('Ctrl Pts',(-2.46089344693261,-224.122676430478,
-1.57841351860035E-15));
#82919=CARTESIAN_POINT('Ctrl Pts',(-2.46996644638514,-224.142197657679,
-2.05391259555654E-15));
#82920=CARTESIAN_POINT('Ctrl Pts',(-2.47861919862404,-224.160814692018,
-2.50738729532423E-15));
#82921=CARTESIAN_POINT('Ctrl Pts',(-2.4870687790189,-224.179549252033,-4.26985750199731E-15));
#82922=CARTESIAN_POINT('Ctrl Pts',(-2.49529984718043,-224.198364615252,
-3.88578058618805E-15));
#82923=CARTESIAN_POINT('Ctrl Pts',(-2.53185222452328,-224.28191953701,-2.18017882468746E-15));
#82924=CARTESIAN_POINT('Ctrl Pts',(-2.56414469936887,-224.367157977321,
1.02042468065935E-14));
#82925=CARTESIAN_POINT('Ctrl Pts',(-2.59215321235953,-224.453680932318,
9.04831765069503E-15));
#82926=CARTESIAN_POINT('Ctrl Pts',(-2.62062491493274,-224.541634756973,
7.87327236594828E-15));
#82927=CARTESIAN_POINT('Ctrl Pts',(-2.64467028407739,-224.630916688536,
3.55782650275821E-15));
#82928=CARTESIAN_POINT('Ctrl Pts',(-2.66422493735634,-224.721144730816,
3.52495810318487E-15));
#82929=CARTESIAN_POINT('Ctrl Pts',(-2.68343419721698,-224.809779077134,
3.49267025744293E-15));
#82930=CARTESIAN_POINT('Ctrl Pts',(-2.69831023427265,-224.89932731694,4.43043718819613E-15));
#82931=CARTESIAN_POINT('Ctrl Pts',(-2.7087493783213,-224.989450156742,4.91273688396632E-15));
#82932=CARTESIAN_POINT('Ctrl Pts',(-2.71288543016613,-225.025157369526,
5.1038269328395E-15));
#82933=CARTESIAN_POINT('Ctrl Pts',(-2.71632448494311,-225.06095496387,4.19046218398344E-15));
#82934=CARTESIAN_POINT('Ctrl Pts',(-2.71905805620622,-225.096822374193,
3.83026943495679E-15));
#82935=CARTESIAN_POINT('Ctrl Pts',(-2.72067802537057,-225.11807812103,3.61681198662921E-15));
#82936=CARTESIAN_POINT('Ctrl Pts',(-2.72205020702394,-225.139358391265,
8.83539236091481E-15));
#82937=CARTESIAN_POINT('Ctrl Pts',(-2.72317263041263,-225.160658927688,
9.27036225562006E-15));
#82938=CARTESIAN_POINT('Ctrl Pts',(-2.72391565392553,-225.174759488635,
9.55830427681055E-15));
#82939=CARTESIAN_POINT('Ctrl Pts',(-2.72454914557126,-225.188868839512,
5.13496310570189E-15));
#82940=CARTESIAN_POINT('Ctrl Pts',(-2.72507219122218,-225.202971354773,
4.94049245958195E-15));
#82941=CARTESIAN_POINT('Ctrl Pts',(-2.72860238425918,-225.298153488667,
3.62795134651196E-15));
#82942=CARTESIAN_POINT('Ctrl Pts',(-2.72711455578113,-225.393185793488,
7.04171290797418E-15));
#82943=CARTESIAN_POINT('Ctrl Pts',(-2.72055026029093,-225.487669326062,
5.82867087928207E-15));
#82944=CARTESIAN_POINT('Ctrl Pts',(-2.71400813842156,-225.581833701457,
4.61972640135258E-15));
#82945=CARTESIAN_POINT('Ctrl Pts',(-2.70242414664252,-225.675453959622,
3.25016722958927E-15));
#82946=CARTESIAN_POINT('Ctrl Pts',(-2.68569242546438,-225.768153085937,
3.30291349825984E-15));
#82947=CARTESIAN_POINT('Ctrl Pts',(-2.68378842047261,-225.778701887065,
3.30891581910756E-15));
#82948=CARTESIAN_POINT('Ctrl Pts',(-2.68181769993591,-225.789238770017,
7.06369997675108E-17));
#82949=CARTESIAN_POINT('Ctrl Pts',(-2.67978006501446,-225.799763185344,
5.55111512312578E-17));
#82950=CARTESIAN_POINT('Ctrl Pts',(-2.662249451615,-225.890309069892,-7.2557142862657E-17));
#82951=CARTESIAN_POINT('Ctrl Pts',(-2.63977030692457,-225.979932423301,
9.99427761194622E-15));
#82952=CARTESIAN_POINT('Ctrl Pts',(-2.61261775161457,-226.06839542511,1.12687636999453E-14));
#82953=CARTESIAN_POINT('Ctrl Pts',(-2.60191929570249,-226.103250985255,
1.17709276056017E-14));
#82954=CARTESIAN_POINT('Ctrl Pts',(-2.59049473479936,-226.137926354826,
5.52161406979016E-15));
#82955=CARTESIAN_POINT('Ctrl Pts',(-2.57835873261334,-226.172406649309,
5.07927033766009E-15));
#82956=CARTESIAN_POINT('Ctrl Pts',(-2.57307203674103,-226.187426985308,
4.8865761747103E-15));
#82957=CARTESIAN_POINT('Ctrl Pts',(-2.56765031882317,-226.202410299172,
1.43913399914977E-14));
#82958=CARTESIAN_POINT('Ctrl Pts',(-2.56209472282316,-226.217355341601,
1.50435219836709E-14));
#82959=CARTESIAN_POINT('Ctrl Pts',(-2.5576757777398,-226.229242692979,1.55622703605811E-14));
#82960=CARTESIAN_POINT('Ctrl Pts',(-2.55317248450269,-226.241104749176,
7.04610913755306E-15));
#82961=CARTESIAN_POINT('Ctrl Pts',(-2.54858920344051,-226.252931575211,
7.04991620636974E-15));
#82962=CARTESIAN_POINT('Ctrl Pts',(-2.51483989794928,-226.340019222562,
7.07794981957767E-15));
#82963=CARTESIAN_POINT('Ctrl Pts',(-2.47670715576013,-226.425333977051,
1.5520638419296E-15));
#82964=CARTESIAN_POINT('Ctrl Pts',(-2.43452445807767,-226.508644905945,
3.17801340798951E-15));
#82965=CARTESIAN_POINT('Ctrl Pts',(-2.3907569116245,-226.595085914954,4.8650516268052E-15));
#82966=CARTESIAN_POINT('Ctrl Pts',(-2.34262924915847,-226.679370417143,
1.31883169502519E-14));
#82967=CARTESIAN_POINT('Ctrl Pts',(-2.29045787431518,-226.761237460125,
1.41137102005473E-14));
#82968=CARTESIAN_POINT('Ctrl Pts',(-2.23768247068651,-226.844052341854,
1.50498174518185E-14));
#82969=CARTESIAN_POINT('Ctrl Pts',(-2.18076876745232,-226.924394278009,
6.05769873306914E-15));
#82970=CARTESIAN_POINT('Ctrl Pts',(-2.11999236348112,-227.001978377933,
6.13398221105399E-15));
#82971=CARTESIAN_POINT('Ctrl Pts',(-2.0772769846332,-227.056506681752,6.18759640092123E-15));
#82972=CARTESIAN_POINT('Ctrl Pts',(-2.03265245620046,-227.109672415922,
5.62971077108756E-15));
#82973=CARTESIAN_POINT('Ctrl Pts',(-1.9862011242703,-227.161369012814,5.27355936696949E-15));
#82974=CARTESIAN_POINT('Ctrl Pts',(-1.97483735729176,-227.174015971604,
5.18643115347578E-15));
#82975=CARTESIAN_POINT('Ctrl Pts',(-1.96336346430018,-227.186575662225,
1.11966090312159E-14));
#82976=CARTESIAN_POINT('Ctrl Pts',(-1.9517923266943,-227.199034120884,1.14630527292547E-14));
#82977=CARTESIAN_POINT('Ctrl Pts',(-1.88311842249801,-227.272974214377,
1.3044377713544E-14));
#82978=CARTESIAN_POINT('Ctrl Pts',(-1.81093155645743,-227.343453602481,
1.5011818698465E-14));
#82979=CARTESIAN_POINT('Ctrl Pts',(-1.73554515615118,-227.410185023087,
1.47104550762833E-14));
#82980=CARTESIAN_POINT('Ctrl Pts',(-1.67071543344256,-227.467571759637,
1.44512926811943E-14));
#82981=CARTESIAN_POINT('Ctrl Pts',(-1.60351847735171,-227.522186792558,
1.4270685325907E-14));
#82982=CARTESIAN_POINT('Ctrl Pts',(-1.53412738920272,-227.573832136014,
1.57721058435811E-14));
#82983=CARTESIAN_POINT('Ctrl Pts',(-1.50861563521692,-227.592819636165,
1.63241057026105E-14));
#82984=CARTESIAN_POINT('Ctrl Pts',(-1.48280709071513,-227.611405560347,
1.28582553745796E-14));
#82985=CARTESIAN_POINT('Ctrl Pts',(-1.456709649847,-227.629579418633,1.27953203588049E-14));
#82986=CARTESIAN_POINT('Ctrl Pts',(-1.43999806640841,-227.641217109496,
1.27550197112187E-14));
#82987=CARTESIAN_POINT('Ctrl Pts',(-1.42316695798824,-227.652686412334,
1.13266969957101E-14));
#82988=CARTESIAN_POINT('Ctrl Pts',(-1.40623322438547,-227.663974897373,
1.14491749414469E-14));
#82989=CARTESIAN_POINT('Ctrl Pts',(-1.32003065852118,-227.72143986038,1.20726590136525E-14));
#82990=CARTESIAN_POINT('Ctrl Pts',(-1.23108709270465,-227.774282119576,
6.07164638895382E-15));
#82991=CARTESIAN_POINT('Ctrl Pts',(-1.13970921686585,-227.822181994227,
5.06192310290032E-15));
#82992=CARTESIAN_POINT('Ctrl Pts',(-1.04833134102704,-227.870081868879,
4.05219981684683E-15));
#82993=CARTESIAN_POINT('Ctrl Pts',(-0.95451851589892,-227.913040261751,
1.85386244543852E-15));
#82994=CARTESIAN_POINT('Ctrl Pts',(-0.858539621091319,-227.950697039278,
2.63894808782972E-15));
#82995=CARTESIAN_POINT('Ctrl Pts',(-0.837654108775876,-227.958891352125,
2.84162983745592E-15));
#82996=CARTESIAN_POINT('Ctrl Pts',(-0.816665907289689,-227.966834441025,
1.13024051429371E-15));
#82997=CARTESIAN_POINT('Ctrl Pts',(-0.795579109021723,-227.974527535833,
9.43689570931383E-16));
#82998=CARTESIAN_POINT('Ctrl Pts',(-2.51426761094033,-224.998573473955,
19.112583302492));
#82999=CARTESIAN_POINT('Ctrl Pts',(-2.51595724505903,-224.672576259975,
19.092036810933));
#83000=CARTESIAN_POINT('Ctrl Pts',(-2.45712156548907,-224.347163909734,
19.0714903193741));
#83001=CARTESIAN_POINT('Ctrl Pts',(-2.33493165330648,-224.04759459911,19.0509438278151));
#83002=CARTESIAN_POINT('Ctrl Pts',(-2.02022083345199,-223.276027604211,
18.9980245394045));
#83003=CARTESIAN_POINT('Ctrl Pts',(-1.28524012182822,-222.675894324399,
18.9451052509939));
#83004=CARTESIAN_POINT('Ctrl Pts',(-0.466331353964879,-222.521799624982,
18.8921859625833));
#83005=CARTESIAN_POINT('Ctrl Pts',(0.352577413898463,-222.367704925566,
18.8392666741727));
#83006=CARTESIAN_POINT('Ctrl Pts',(1.25541423800138,-222.659648806545,18.7863473857621));
#83007=CARTESIAN_POINT('Ctrl Pts',(1.82904823179956,-223.264045686903,18.7334280973515));
#83008=CARTESIAN_POINT('Ctrl Pts',(2.40268222559773,-223.86844256726,18.6805088089409));
#83009=CARTESIAN_POINT('Ctrl Pts',(2.64711338909116,-224.785292446995,18.6275895205303));
#83010=CARTESIAN_POINT('Ctrl Pts',(2.45048646849204,-225.595040932989,18.5746702321197));
#83011=CARTESIAN_POINT('Ctrl Pts',(2.25385954789293,-226.404789418983,18.5217509437091));
#83012=CARTESIAN_POINT('Ctrl Pts',(1.61617454320126,-227.107436511236,18.4688316552985));
#83013=CARTESIAN_POINT('Ctrl Pts',(0.829237852020633,-227.381452837493,
18.4159123668879));
#83014=CARTESIAN_POINT('Ctrl Pts',(0.0423011608400069,-227.65546916375,
18.3629930784773));
#83015=CARTESIAN_POINT('Ctrl Pts',(-0.89388721682958,-227.500854724012,
18.3100737900667));
#83016=CARTESIAN_POINT('Ctrl Pts',(-1.55092836043026,-226.988360135835,
18.2571545016561));
#83017=CARTESIAN_POINT('Ctrl Pts',(-2.14925604575053,-226.521662268176,
18.2089641019348));
#83018=CARTESIAN_POINT('Ctrl Pts',(-2.51609684399047,-225.758187103811,
18.1607737022134));
#83019=CARTESIAN_POINT('Ctrl Pts',(-2.52086477440939,-224.998703164308,
18.112583302492));
#83020=CARTESIAN_POINT('Ctrl Pts',(-0.793799282532874,-227.969222953746,
20.));
#83021=CARTESIAN_POINT('Ctrl Pts',(-0.886846222511741,-227.935185967463,
20.));
#83022=CARTESIAN_POINT('Ctrl Pts',(-0.977826056161207,-227.896378578773,
20.));
#83023=CARTESIAN_POINT('Ctrl Pts',(-1.0665310835594,-227.853129769234,20.));
#83024=CARTESIAN_POINT('Ctrl Pts',(-1.15720918642954,-227.808918971769,
20.));
#83025=CARTESIAN_POINT('Ctrl Pts',(-1.24551082699134,-227.760066356736,
20.));
#83026=CARTESIAN_POINT('Ctrl Pts',(-1.33118520242785,-227.706877790385,
20.));
#83027=CARTESIAN_POINT('Ctrl Pts',(-1.414118896504,-227.655390700253,20.));
#83028=CARTESIAN_POINT('Ctrl Pts',(-1.49459105090855,-227.599839768124,
20.));
#83029=CARTESIAN_POINT('Ctrl Pts',(-1.57234048325287,-227.540471761617,
20.));
#83030=CARTESIAN_POINT('Ctrl Pts',(-1.64037123655415,-227.488524755923,
20.));
#83031=CARTESIAN_POINT('Ctrl Pts',(-1.7063171091793,-227.433654585998,20.));
#83032=CARTESIAN_POINT('Ctrl Pts',(-1.76997788546532,-227.376013601272,
20.));
#83033=CARTESIAN_POINT('Ctrl Pts',(-1.78334881537323,-227.363907032494,
20.));
#83034=CARTESIAN_POINT('Ctrl Pts',(-1.79662074549451,-227.351676294922,
20.));
#83035=CARTESIAN_POINT('Ctrl Pts',(-1.80977455173367,-227.339339189254,
20.));
#83036=CARTESIAN_POINT('Ctrl Pts',(-1.88220127158014,-227.271409338402,
20.));
#83037=CARTESIAN_POINT('Ctrl Pts',(-1.95116225702347,-227.200157915227,
20.));
#83038=CARTESIAN_POINT('Ctrl Pts',(-2.01641820370584,-227.125876415728,
20.));
#83039=CARTESIAN_POINT('Ctrl Pts',(-2.08131431772935,-227.052004517359,
20.));
#83040=CARTESIAN_POINT('Ctrl Pts',(-2.14254662606162,-226.97513506864,20.));
#83041=CARTESIAN_POINT('Ctrl Pts',(-2.19983614514141,-226.895528023604,
20.));
#83042=CARTESIAN_POINT('Ctrl Pts',(-2.25566849653972,-226.817945795936,
20.));
#83043=CARTESIAN_POINT('Ctrl Pts',(-2.30775634501805,-226.737762722758,
20.));
#83044=CARTESIAN_POINT('Ctrl Pts',(-2.35579466209043,-226.655205328684,
20.));
#83045=CARTESIAN_POINT('Ctrl Pts',(-2.37650841258532,-226.619607219371,
20.));
#83046=CARTESIAN_POINT('Ctrl Pts',(-2.39646862341355,-226.583567543625,
20.));
#83047=CARTESIAN_POINT('Ctrl Pts',(-2.41564786554802,-226.547104130923,
20.));
#83048=CARTESIAN_POINT('Ctrl Pts',(-2.42885136523054,-226.522001749157,
20.));
#83049=CARTESIAN_POINT('Ctrl Pts',(-2.44168470148669,-226.496698542274,
20.));
#83050=CARTESIAN_POINT('Ctrl Pts',(-2.45413839533455,-226.471200323988,
20.));
#83051=CARTESIAN_POINT('Ctrl Pts',(-2.46035289057376,-226.458476504206,
20.));
#83052=CARTESIAN_POINT('Ctrl Pts',(-2.46647230820266,-226.445705077751,
20.));
#83053=CARTESIAN_POINT('Ctrl Pts',(-2.4724902648514,-226.43289832355,20.));
#83054=CARTESIAN_POINT('Ctrl Pts',(-2.51269158383526,-226.347346293045,
20.));
#83055=CARTESIAN_POINT('Ctrl Pts',(-2.54843638213312,-226.26008271746,20.));
#83056=CARTESIAN_POINT('Ctrl Pts',(-2.57947357847436,-226.171345167024,
20.));
#83057=CARTESIAN_POINT('Ctrl Pts',(-2.6098249216307,-226.084568519594,20.));
#83058=CARTESIAN_POINT('Ctrl Pts',(-2.63567463650983,-225.99638164586,20.));
#83059=CARTESIAN_POINT('Ctrl Pts',(-2.65673878831304,-225.906997936184,
20.));
#83060=CARTESIAN_POINT('Ctrl Pts',(-2.66036642238348,-225.891604418629,
20.));
#83061=CARTESIAN_POINT('Ctrl Pts',(-2.66385199584536,-225.876175396232,
20.));
#83062=CARTESIAN_POINT('Ctrl Pts',(-2.6671938997738,-225.860711953896,20.));
#83063=CARTESIAN_POINT('Ctrl Pts',(-2.68732104473893,-225.767580926726,
20.));
#83064=CARTESIAN_POINT('Ctrl Pts',(-2.70224103896547,-225.673200364495,
20.));
#83065=CARTESIAN_POINT('Ctrl Pts',(-2.71203226714566,-225.577978837703,
20.));
#83066=CARTESIAN_POINT('Ctrl Pts',(-2.71529432210383,-225.546254742638,
20.));
#83067=CARTESIAN_POINT('Ctrl Pts',(-2.71798669148681,-225.514437423479,
20.));
#83068=CARTESIAN_POINT('Ctrl Pts',(-2.72011107509275,-225.482542447591,
20.));
#83069=CARTESIAN_POINT('Ctrl Pts',(-2.72133540379954,-225.464160675827,
20.));
#83070=CARTESIAN_POINT('Ctrl Pts',(-2.72237106709187,-225.445753115879,
20.));
#83071=CARTESIAN_POINT('Ctrl Pts',(-2.72321830491854,-225.427322796075,
20.));
#83072=CARTESIAN_POINT('Ctrl Pts',(-2.72379259438604,-225.414830036413,
20.));
#83073=CARTESIAN_POINT('Ctrl Pts',(-2.72428019028657,-225.402328437053,
20.));
#83074=CARTESIAN_POINT('Ctrl Pts',(-2.72468104799973,-225.389828334462,
20.));
#83075=CARTESIAN_POINT('Ctrl Pts',(-2.72766941146398,-225.296641029703,
20.));
#83076=CARTESIAN_POINT('Ctrl Pts',(-2.72584877239909,-225.203390772035,
20.));
#83077=CARTESIAN_POINT('Ctrl Pts',(-2.71935801752115,-225.110452407722,
20.));
#83078=CARTESIAN_POINT('Ctrl Pts',(-2.71285441326256,-225.017330058581,
20.));
#83079=CARTESIAN_POINT('Ctrl Pts',(-2.70166180134637,-224.924519857946,
20.));
#83080=CARTESIAN_POINT('Ctrl Pts',(-2.68586885793089,-224.832410901971,
20.));
#83081=CARTESIAN_POINT('Ctrl Pts',(-2.67029897206218,-224.741602881307,
20.));
#83082=CARTESIAN_POINT('Ctrl Pts',(-2.65025731856795,-224.651475590115,
20.));
#83083=CARTESIAN_POINT('Ctrl Pts',(-2.62578582409315,-224.562427028653,
20.));
#83084=CARTESIAN_POINT('Ctrl Pts',(-2.6162702977942,-224.527801275439,20.));
#83085=CARTESIAN_POINT('Ctrl Pts',(-2.60608456229951,-224.49333896239,20.));
#83086=CARTESIAN_POINT('Ctrl Pts',(-2.5952295152326,-224.459064951709,20.));
#83087=CARTESIAN_POINT('Ctrl Pts',(-2.58886662729354,-224.438974602229,
20.));
#83088=CARTESIAN_POINT('Ctrl Pts',(-2.58227375230166,-224.418948969267,
20.));
#83089=CARTESIAN_POINT('Ctrl Pts',(-2.57545094085638,-224.398993216091,
20.));
#83090=CARTESIAN_POINT('Ctrl Pts',(-2.57042017973329,-224.384278955252,
20.));
#83091=CARTESIAN_POINT('Ctrl Pts',(-2.56526459701236,-224.369603474027,
20.));
#83092=CARTESIAN_POINT('Ctrl Pts',(-2.55998882406935,-224.354980991355,
20.));
#83093=CARTESIAN_POINT('Ctrl Pts',(-2.52758494590353,-224.265169478969,
20.));
#83094=CARTESIAN_POINT('Ctrl Pts',(-2.49060962869267,-224.177231268765,
20.));
#83095=CARTESIAN_POINT('Ctrl Pts',(-2.44913502518246,-224.091607986908,
20.));
#83096=CARTESIAN_POINT('Ctrl Pts',(-2.41802907254981,-224.027390525516,
20.));
#83097=CARTESIAN_POINT('Ctrl Pts',(-2.38439113354255,-223.964475745917,
20.));
#83098=CARTESIAN_POINT('Ctrl Pts',(-2.34823443080839,-223.903066989878,
20.));
#83099=CARTESIAN_POINT('Ctrl Pts',(-2.33711427891036,-223.884180458658,
20.));
#83100=CARTESIAN_POINT('Ctrl Pts',(-2.32575578046286,-223.865436503756,
20.));
#83101=CARTESIAN_POINT('Ctrl Pts',(-2.31415906828801,-223.846841383834,
20.));
#83102=CARTESIAN_POINT('Ctrl Pts',(-2.3031725094525,-223.829224633845,20.));
#83103=CARTESIAN_POINT('Ctrl Pts',(-2.29197113405253,-223.81174018047,20.));
#83104=CARTESIAN_POINT('Ctrl Pts',(-2.28056700193948,-223.794411054613,
20.));
#83105=CARTESIAN_POINT('Ctrl Pts',(-2.23334585426799,-223.722656255296,
20.));
#83106=CARTESIAN_POINT('Ctrl Pts',(-2.1826076926359,-223.653490621674,20.));
#83107=CARTESIAN_POINT('Ctrl Pts',(-2.12838833087224,-223.587265557295,
20.));
#83108=CARTESIAN_POINT('Ctrl Pts',(-2.07470388645401,-223.521693856114,
20.));
#83109=CARTESIAN_POINT('Ctrl Pts',(-2.01760623335831,-223.45900440161,20.));
#83110=CARTESIAN_POINT('Ctrl Pts',(-1.95710201649547,-223.399580085816,
20.));
#83111=CARTESIAN_POINT('Ctrl Pts',(-1.94393777493637,-223.386650804384,
20.));
#83112=CARTESIAN_POINT('Ctrl Pts',(-1.93061217207899,-223.373876270997,
20.));
#83113=CARTESIAN_POINT('Ctrl Pts',(-1.91712859175369,-223.361257881811,
20.));
#83114=CARTESIAN_POINT('Origin',(0.,0.,20.));
#83115=CARTESIAN_POINT('',(-325.,275.,20.));
#83116=CARTESIAN_POINT('',(-325.,-275.,20.));
#83117=CARTESIAN_POINT('',(-325.,275.,20.));
#83118=CARTESIAN_POINT('',(325.,-275.,20.));
#83119=CARTESIAN_POINT('',(-325.,-275.,20.));
#83120=CARTESIAN_POINT('',(325.,275.,20.));
#83121=CARTESIAN_POINT('',(325.,-275.,20.));
#83122=CARTESIAN_POINT('',(325.,275.,20.));
#83123=CARTESIAN_POINT('Ctrl Pts',(161.913465996665,226.635987203375,20.));
#83124=CARTESIAN_POINT('Ctrl Pts',(161.975061800004,226.578102273232,20.));
#83125=CARTESIAN_POINT('Ctrl Pts',(162.0332856474,226.517065654258,20.));
#83126=CARTESIAN_POINT('Ctrl Pts',(162.088141171723,226.453262405738,20.));
#83127=CARTESIAN_POINT('Ctrl Pts',(162.144450720438,226.387767960555,20.));
#83128=CARTESIAN_POINT('Ctrl Pts',(162.19721144993,226.319357843406,20.));
#83129=CARTESIAN_POINT('Ctrl Pts',(162.246401727216,226.248399999785,20.));
#83130=CARTESIAN_POINT('Ctrl Pts',(162.29728997268,226.174992807083,20.));
#83131=CARTESIAN_POINT('Ctrl Pts',(162.344357601167,226.098858443986,20.));
#83132=CARTESIAN_POINT('Ctrl Pts',(162.387545727347,226.020360285483,20.));
#83133=CARTESIAN_POINT('Ctrl Pts',(162.406440532551,225.986017341139,20.));
#83134=CARTESIAN_POINT('Ctrl Pts',(162.424592282786,225.951221445178,20.));
#83135=CARTESIAN_POINT('Ctrl Pts',(162.441993602386,225.916000937453,20.));
#83136=CARTESIAN_POINT('Ctrl Pts',(162.451521583465,225.896716174059,20.));
#83137=CARTESIAN_POINT('Ctrl Pts',(162.460824555144,225.877304090621,20.));
#83138=CARTESIAN_POINT('Ctrl Pts',(162.469901101426,225.857769209579,20.));
#83139=CARTESIAN_POINT('Ctrl Pts',(162.478557268221,225.839139084926,20.));
#83140=CARTESIAN_POINT('Ctrl Pts',(162.487009994063,225.820391256647,20.));
#83141=CARTESIAN_POINT('Ctrl Pts',(162.495243927467,225.801562500441,20.));
#83142=CARTESIAN_POINT('Ctrl Pts',(162.53178332527,225.718006880125,20.));
#83143=CARTESIAN_POINT('Ctrl Pts',(162.564063310772,225.63276760616,20.));
#83144=CARTESIAN_POINT('Ctrl Pts',(162.592060189714,225.546243928286,20.));
#83145=CARTESIAN_POINT('Ctrl Pts',(162.620521622014,225.458284559485,20.));
#83146=CARTESIAN_POINT('Ctrl Pts',(162.64455712023,225.368997053047,20.));
#83147=CARTESIAN_POINT('Ctrl Pts',(162.664102677438,225.278763725346,20.));
#83148=CARTESIAN_POINT('Ctrl Pts',(162.683304662781,225.190116519363,20.));
#83149=CARTESIAN_POINT('Ctrl Pts',(162.69817342338,225.100555540895,20.));
#83150=CARTESIAN_POINT('Ctrl Pts',(162.70860562281,225.010420473573,20.));
#83151=CARTESIAN_POINT('Ctrl Pts',(162.71273953757,224.974703107576,20.));
#83152=CARTESIAN_POINT('Ctrl Pts',(162.716176300128,224.938895413385,20.));
#83153=CARTESIAN_POINT('Ctrl Pts',(162.718907440897,224.90301799008,20.));
#83154=CARTESIAN_POINT('Ctrl Pts',(162.720525638553,224.881760659461,20.));
#83155=CARTESIAN_POINT('Ctrl Pts',(162.721896101523,224.860478845972,20.));
#83156=CARTESIAN_POINT('Ctrl Pts',(162.723016863678,224.839176811201,20.));
#83157=CARTESIAN_POINT('Ctrl Pts',(162.723758858197,224.825073914374,20.));
#83158=CARTESIAN_POINT('Ctrl Pts',(162.724391325361,224.810962241637,20.));
#83159=CARTESIAN_POINT('Ctrl Pts',(162.724913352953,224.796857427549,20.));
#83160=CARTESIAN_POINT('Ctrl Pts',(162.728436324273,224.701669249314,20.));
#83161=CARTESIAN_POINT('Ctrl Pts',(162.726942555487,224.606631878699,20.));
#83162=CARTESIAN_POINT('Ctrl Pts',(162.720373977506,224.51214461544,20.));
#83163=CARTESIAN_POINT('Ctrl Pts',(162.713827131361,224.417969958907,20.));
#83164=CARTESIAN_POINT('Ctrl Pts',(162.702239359173,224.324340821208,20.));
#83165=CARTESIAN_POINT('Ctrl Pts',(162.685505157103,224.231634650513,20.));
#83166=CARTESIAN_POINT('Ctrl Pts',(162.683600867107,224.221085032865,20.));
#83167=CARTESIAN_POINT('Ctrl Pts',(162.681629878204,224.210547357196,20.));
#83168=CARTESIAN_POINT('Ctrl Pts',(162.67959199208,224.200022173605,20.));
#83169=CARTESIAN_POINT('Ctrl Pts',(162.662058769681,224.109467366597,20.));
#83170=CARTESIAN_POINT('Ctrl Pts',(162.639578033128,224.019836946214,20.));
#83171=CARTESIAN_POINT('Ctrl Pts',(162.612424683658,223.931368511278,20.));
#83172=CARTESIAN_POINT('Ctrl Pts',(162.601724422561,223.896505948419,20.));
#83173=CARTESIAN_POINT('Ctrl Pts',(162.59029797784,223.86182388033,20.));
#83174=CARTESIAN_POINT('Ctrl Pts',(162.578160005908,223.827337185001,20.));
#83175=CARTESIAN_POINT('Ctrl Pts',(162.572849528586,223.812248930187,20.));
#83176=CARTESIAN_POINT('Ctrl Pts',(162.567402839519,223.797198076188,20.));
#83177=CARTESIAN_POINT('Ctrl Pts',(162.561821096873,223.782185888141,20.));
#83178=CARTESIAN_POINT('Ctrl Pts',(162.557400342449,223.770296196883,20.));
#83179=CARTESIAN_POINT('Ctrl Pts',(162.552895274848,223.7584319722,20.));
#83180=CARTESIAN_POINT('Ctrl Pts',(162.548310201456,223.746603001261,20.));
#83181=CARTESIAN_POINT('Ctrl Pts',(162.514551802678,223.659510149315,20.));
#83182=CARTESIAN_POINT('Ctrl Pts',(162.476410434573,223.574192137851,20.));
#83183=CARTESIAN_POINT('Ctrl Pts',(162.434219363372,223.490879700338,20.));
#83184=CARTESIAN_POINT('Ctrl Pts',(162.390445975646,223.404442747548,20.));
#83185=CARTESIAN_POINT('Ctrl Pts',(162.342313310282,223.320163902973,20.));
#83186=CARTESIAN_POINT('Ctrl Pts',(162.290137469479,223.238303878085,20.));
#83187=CARTESIAN_POINT('Ctrl Pts',(162.2373599398,223.155499847971,20.));
#83188=CARTESIAN_POINT('Ctrl Pts',(162.18044503493,223.075169931722,20.));
#83189=CARTESIAN_POINT('Ctrl Pts',(162.119668013951,222.997598761584,20.));
#83190=CARTESIAN_POINT('Ctrl Pts',(162.076868402372,222.942972590408,20.));
#83191=CARTESIAN_POINT('Ctrl Pts',(162.032152436797,222.889714789462,20.));
#83192=CARTESIAN_POINT('Ctrl Pts',(161.985602823726,222.83793247878,20.));
#83193=CARTESIAN_POINT('Ctrl Pts',(161.974397260002,222.825467284252,20.));
#83194=CARTESIAN_POINT('Ctrl Pts',(161.963084797841,222.813087095521,20.));
#83195=CARTESIAN_POINT('Ctrl Pts',(161.951677829852,222.800805336977,20.));
#83196=CARTESIAN_POINT('Ctrl Pts',(161.88301156409,222.726873114409,20.));
#83197=CARTESIAN_POINT('Ctrl Pts',(161.810832354244,222.656401977612,20.));
#83198=CARTESIAN_POINT('Ctrl Pts',(161.7354533295,222.589678899564,20.));
#83199=CARTESIAN_POINT('Ctrl Pts',(161.670633416166,222.532302405889,20.));
#83200=CARTESIAN_POINT('Ctrl Pts',(161.603446315265,222.477697387466,20.));
#83201=CARTESIAN_POINT('Ctrl Pts',(161.534064912603,222.42606161964,20.));
#83202=CARTESIAN_POINT('Ctrl Pts',(161.508545124964,222.407069010973,20.));
#83203=CARTESIAN_POINT('Ctrl Pts',(161.482728254045,222.388478284016,20.));
#83204=CARTESIAN_POINT('Ctrl Pts',(161.456622194046,222.37029993255,20.));
#83205=CARTESIAN_POINT('Ctrl Pts',(161.439929880381,222.358676625755,20.));
#83206=CARTESIAN_POINT('Ctrl Pts',(161.423118286825,222.347221341864,20.));
#83207=CARTESIAN_POINT('Ctrl Pts',(161.406204262001,222.335946470941,20.));
#83208=CARTESIAN_POINT('Ctrl Pts',(161.3200106339,222.278489890305,20.));
#83209=CARTESIAN_POINT('Ctrl Pts',(161.23107534457,222.225655428716,20.));
#83210=CARTESIAN_POINT('Ctrl Pts',(161.139704755267,222.177762443093,20.));
#83211=CARTESIAN_POINT('Ctrl Pts',(161.048334165963,222.12986945747,20.));
#83212=CARTESIAN_POINT('Ctrl Pts',(160.95452763806,222.086917045673,20.));
#83213=CARTESIAN_POINT('Ctrl Pts',(160.858553719049,222.049265014674,20.));
#83214=CARTESIAN_POINT('Ctrl Pts',(160.837669284144,222.041071732598,20.));
#83215=CARTESIAN_POINT('Ctrl Pts',(160.816682097409,222.033129616109,20.));
#83216=CARTESIAN_POINT('Ctrl Pts',(160.795596253159,222.025437437374,20.));
#83217=CARTESIAN_POINT('Ctrl Pts',(159.206200717467,222.030777046254,20.));
#83218=CARTESIAN_POINT('Ctrl Pts',(159.113164826053,222.064809990922,20.));
#83219=CARTESIAN_POINT('Ctrl Pts',(159.022195938487,222.10361488715,20.));
#83220=CARTESIAN_POINT('Ctrl Pts',(158.933501595931,222.146862343058,20.));
#83221=CARTESIAN_POINT('Ctrl Pts',(158.842828942866,222.191074425278,20.));
#83222=CARTESIAN_POINT('Ctrl Pts',(158.754532766168,222.239930075798,20.));
#83223=CARTESIAN_POINT('Ctrl Pts',(158.668863733849,222.293122937636,20.));
#83224=CARTESIAN_POINT('Ctrl Pts',(158.585928500332,222.344618353173,20.));
#83225=CARTESIAN_POINT('Ctrl Pts',(158.505455091515,222.400179449777,20.));
#83226=CARTESIAN_POINT('Ctrl Pts',(158.42770462389,222.459558956778,20.));
#83227=CARTESIAN_POINT('Ctrl Pts',(158.359672964719,222.511516025404,20.));
#83228=CARTESIAN_POINT('Ctrl Pts',(158.293726354064,222.566397281688,20.));
#83229=CARTESIAN_POINT('Ctrl Pts',(158.230064964185,222.62405003757,20.));
#83230=CARTESIAN_POINT('Ctrl Pts',(158.216686188916,222.636166066864,20.));
#83231=CARTESIAN_POINT('Ctrl Pts',(158.203406524907,222.648406446606,20.));
#83232=CARTESIAN_POINT('Ctrl Pts',(158.190245124516,222.660753343364,20.));
#83233=CARTESIAN_POINT('Ctrl Pts',(158.117820209736,222.728696185234,20.));
#83234=CARTESIAN_POINT('Ctrl Pts',(158.048861054711,222.799961146741,20.));
#83235=CARTESIAN_POINT('Ctrl Pts',(157.983606877175,222.874256209938,20.));
#83236=CARTESIAN_POINT('Ctrl Pts',(157.918710344149,222.948144077421,20.));
#83237=CARTESIAN_POINT('Ctrl Pts',(157.85747780208,223.025029722442,20.));
#83238=CARTESIAN_POINT('Ctrl Pts',(157.80018817671,223.1046526491,20.));
#83239=CARTESIAN_POINT('Ctrl Pts',(157.744357459177,223.182247939675,20.));
#83240=CARTESIAN_POINT('Ctrl Pts',(157.692271132893,223.262443615976,20.));
#83241=CARTESIAN_POINT('Ctrl Pts',(157.644234146577,223.345012659254,20.));
#83242=CARTESIAN_POINT('Ctrl Pts',(157.62352025824,223.380617014851,20.));
#83243=CARTESIAN_POINT('Ctrl Pts',(157.603559925696,223.416662789586,20.));
#83244=CARTESIAN_POINT('Ctrl Pts',(157.584380574184,223.453132111068,20.));
#83245=CARTESIAN_POINT('Ctrl Pts',(157.571170252012,223.478251390303,20.));
#83246=CARTESIAN_POINT('Ctrl Pts',(157.558330477497,223.503571609699,20.));
#83247=CARTESIAN_POINT('Ctrl Pts',(157.545870743057,223.52908693229,20.));
#83248=CARTESIAN_POINT('Ctrl Pts',(157.539658096197,223.541809329346,20.));
#83249=CARTESIAN_POINT('Ctrl Pts',(157.533540489381,223.554579256024,20.));
#83250=CARTESIAN_POINT('Ctrl Pts',(157.527524288537,223.56738446368,20.));
#83251=CARTESIAN_POINT('Ctrl Pts',(157.487323756338,223.652949453292,20.));
#83252=CARTESIAN_POINT('Ctrl Pts',(157.451579825719,223.740224649066,20.));
#83253=CARTESIAN_POINT('Ctrl Pts',(157.420543535262,223.828971978343,20.));
#83254=CARTESIAN_POINT('Ctrl Pts',(157.390193276996,223.915757619425,20.));
#83255=CARTESIAN_POINT('Ctrl Pts',(157.36434462463,224.003951708281,20.));
#83256=CARTESIAN_POINT('Ctrl Pts',(157.343281471526,224.09334036721,20.));
#83257=CARTESIAN_POINT('Ctrl Pts',(157.339658550573,224.108715465315,20.));
#83258=CARTESIAN_POINT('Ctrl Pts',(157.336177332896,224.124125912316,20.));
#83259=CARTESIAN_POINT('Ctrl Pts',(157.332839421148,224.139570624809,20.));
#83260=CARTESIAN_POINT('Ctrl Pts',(157.31271183051,224.232702161571,20.));
#83261=CARTESIAN_POINT('Ctrl Pts',(157.297790873772,224.327080661966,20.));
#83262=CARTESIAN_POINT('Ctrl Pts',(157.287998249313,224.422297987317,20.));
#83263=CARTESIAN_POINT('Ctrl Pts',(157.284735553856,224.454022387265,20.));
#83264=CARTESIAN_POINT('Ctrl Pts',(157.282042557023,224.485839783746,20.));
#83265=CARTESIAN_POINT('Ctrl Pts',(157.279917561785,224.517734622728,20.));
#83266=CARTESIAN_POINT('Ctrl Pts',(157.278692761054,224.536118109621,20.));
#83267=CARTESIAN_POINT('Ctrl Pts',(157.277656667823,224.554527318563,20.));
#83268=CARTESIAN_POINT('Ctrl Pts',(157.276809042623,224.572959222881,20.));
#83269=CARTESIAN_POINT('Ctrl Pts',(157.276234517208,224.585452477542,20.));
#83270=CARTESIAN_POINT('Ctrl Pts',(157.275746697198,224.597954534638,20.));
#83271=CARTESIAN_POINT('Ctrl Pts',(157.275345627116,224.61045506494,20.));
#83272=CARTESIAN_POINT('Ctrl Pts',(157.272355985663,224.703636045658,20.));
#83273=CARTESIAN_POINT('Ctrl Pts',(157.274175017621,224.7968782471,20.));
#83274=CARTESIAN_POINT('Ctrl Pts',(157.280663921379,224.889807250199,20.));
#83275=CARTESIAN_POINT('Ctrl Pts',(157.2871656766,224.982920301909,20.));
#83276=CARTESIAN_POINT('Ctrl Pts',(157.298356202607,225.07571989352,20.));
#83277=CARTESIAN_POINT('Ctrl Pts',(157.314146905939,225.167817345856,20.));
#83278=CARTESIAN_POINT('Ctrl Pts',(157.329714980876,225.258616343805,20.));
#83279=CARTESIAN_POINT('Ctrl Pts',(157.349754901625,225.348733707285,20.));
#83280=CARTESIAN_POINT('Ctrl Pts',(157.3742248181,225.437771805825,20.));
#83281=CARTESIAN_POINT('Ctrl Pts',(157.383741654276,225.472400489504,20.));
#83282=CARTESIAN_POINT('Ctrl Pts',(157.393928994079,225.506865586047,20.));
#83283=CARTESIAN_POINT('Ctrl Pts',(157.404785944163,225.541142240111,20.));
#83284=CARTESIAN_POINT('Ctrl Pts',(157.410770474058,225.560036096983,20.));
#83285=CARTESIAN_POINT('Ctrl Pts',(157.416958472911,225.578872681468,20.));
#83286=CARTESIAN_POINT('Ctrl Pts',(157.423349897143,225.597647704039,20.));
#83287=CARTESIAN_POINT('Ctrl Pts',(157.428585354712,225.613027035854,20.));
#83288=CARTESIAN_POINT('Ctrl Pts',(157.433957583455,225.628365578923,20.));
#83289=CARTESIAN_POINT('Ctrl Pts',(157.439461066734,225.643646297879,20.));
#83290=CARTESIAN_POINT('Ctrl Pts',(157.471856101309,225.73359286331,20.));
#83291=CARTESIAN_POINT('Ctrl Pts',(157.508836086653,225.821663133571,20.));
#83292=CARTESIAN_POINT('Ctrl Pts',(157.550328404654,225.907414260252,20.));
#83293=CARTESIAN_POINT('Ctrl Pts',(157.581447643154,225.971727605262,20.));
#83294=CARTESIAN_POINT('Ctrl Pts',(157.61510621399,226.034735896424,20.));
#83295=CARTESIAN_POINT('Ctrl Pts',(157.651290808751,226.096235211794,20.));
#83296=CARTESIAN_POINT('Ctrl Pts',(157.665718308263,226.120756181238,20.));
#83297=CARTESIAN_POINT('Ctrl Pts',(157.680547541966,226.145037068919,20.));
#83298=CARTESIAN_POINT('Ctrl Pts',(157.695778254971,226.169064140891,20.));
#83299=CARTESIAN_POINT('Ctrl Pts',(157.706207067959,226.18551601942,20.));
#83300=CARTESIAN_POINT('Ctrl Pts',(157.716819725857,226.201841855266,20.));
#83301=CARTESIAN_POINT('Ctrl Pts',(157.727611766764,226.218031728238,20.));
#83302=CARTESIAN_POINT('Ctrl Pts',(157.775201490332,226.289424302256,20.));
#83303=CARTESIAN_POINT('Ctrl Pts',(157.826300374104,226.35821312358,20.));
#83304=CARTESIAN_POINT('Ctrl Pts',(157.880874545296,226.424045717618,20.));
#83305=CARTESIAN_POINT('Ctrl Pts',(157.931843171733,226.485528958125,20.));
#83306=CARTESIAN_POINT('Ctrl Pts',(157.985843573699,226.544433813733,20.));
#83307=CARTESIAN_POINT('Ctrl Pts',(158.042870872967,226.60043887372,20.));
#83308=CARTESIAN_POINT('Ctrl Pts',(158.056034905552,226.613366935264,20.));
#83309=CARTESIAN_POINT('Ctrl Pts',(158.069360315117,226.6261403196,20.));
#83310=CARTESIAN_POINT('Ctrl Pts',(158.082843717471,226.638757628308,20.));
#83311=CARTESIAN_POINT('Ctrl Pts',(-158.086534003335,226.635987203375,20.));
#83312=CARTESIAN_POINT('Ctrl Pts',(-158.02493815882,226.578102234536,20.));
#83313=CARTESIAN_POINT('Ctrl Pts',(-157.966714268211,226.517065579823,20.));
#83314=CARTESIAN_POINT('Ctrl Pts',(-157.911858699942,226.45326229789,20.));
#83315=CARTESIAN_POINT('Ctrl Pts',(-157.855549110443,226.387767823441,20.));
#83316=CARTESIAN_POINT('Ctrl Pts',(-157.802788338847,226.319357679923,20.));
#83317=CARTESIAN_POINT('Ctrl Pts',(-157.753598019515,226.248399812053,20.));
#83318=CARTESIAN_POINT('Ctrl Pts',(-157.702709768307,226.174992648725,20.));
#83319=CARTESIAN_POINT('Ctrl Pts',(-157.655642128471,226.098858321311,20.));
#83320=CARTESIAN_POINT('Ctrl Pts',(-157.612453986729,226.020360203137,20.));
#83321=CARTESIAN_POINT('Ctrl Pts',(-157.593559174717,225.986017276436,20.));
#83322=CARTESIAN_POINT('Ctrl Pts',(-157.575407416866,225.95122139901,20.));
#83323=CARTESIAN_POINT('Ctrl Pts',(-157.558006088956,225.916000910576,20.));
#83324=CARTESIAN_POINT('Ctrl Pts',(-157.548478124627,225.896716200858,20.));
#83325=CARTESIAN_POINT('Ctrl Pts',(-157.539175168484,225.877304171892,20.));
#83326=CARTESIAN_POINT('Ctrl Pts',(-157.530098636533,225.857769346065,20.));
#83327=CARTESIAN_POINT('Ctrl Pts',(-157.521442483325,225.8391392739,20.));
#83328=CARTESIAN_POINT('Ctrl Pts',(-157.512989769992,225.820391498827,20.));
#83329=CARTESIAN_POINT('Ctrl Pts',(-157.504755847974,225.80156279633,20.));
#83330=CARTESIAN_POINT('Ctrl Pts',(-157.468216397868,225.718007179217,20.));
#83331=CARTESIAN_POINT('Ctrl Pts',(-157.435936362002,225.632767909081,20.));
#83332=CARTESIAN_POINT('Ctrl Pts',(-157.407939436079,225.546244234685,20.));
#83333=CARTESIAN_POINT('Ctrl Pts',(-157.379477962203,225.458284888532,20.));
#83334=CARTESIAN_POINT('Ctrl Pts',(-157.355442423985,225.368997404955,20.));
#83335=CARTESIAN_POINT('Ctrl Pts',(-157.335896829832,225.278764099056,20.));
#83336=CARTESIAN_POINT('Ctrl Pts',(-157.316694814992,225.190116945868,20.));
#83337=CARTESIAN_POINT('Ctrl Pts',(-157.301826024782,225.10055601982,20.));
#83338=CARTESIAN_POINT('Ctrl Pts',(-157.291393796945,225.010421002983,20.));
#83339=CARTESIAN_POINT('Ctrl Pts',(-157.287259873426,224.974703678566,20.));
#83340=CARTESIAN_POINT('Ctrl Pts',(-157.283823101457,224.93889602576,20.));
#83341=CARTESIAN_POINT('Ctrl Pts',(-157.281091950689,224.903018643511,20.));
#83342=CARTESIAN_POINT('Ctrl Pts',(-157.279473745741,224.881761319259,20.));
#83343=CARTESIAN_POINT('Ctrl Pts',(-157.278103275693,224.86047951198,20.));
#83344=CARTESIAN_POINT('Ctrl Pts',(-157.27698250669,224.839177483244,20.));
#83345=CARTESIAN_POINT('Ctrl Pts',(-157.276240507937,224.825074596109,20.));
#83346=CARTESIAN_POINT('Ctrl Pts',(-157.275608036552,224.810962933012,20.));
#83347=CARTESIAN_POINT('Ctrl Pts',(-157.275086004761,224.796858128474,20.));
#83348=CARTESIAN_POINT('Ctrl Pts',(-157.271563003652,224.701669975447,20.));
#83349=CARTESIAN_POINT('Ctrl Pts',(-157.273056747714,224.606632626241,20.));
#83350=CARTESIAN_POINT('Ctrl Pts',(-157.279625307528,224.512145379171,20.));
#83351=CARTESIAN_POINT('Ctrl Pts',(-157.286172133748,224.417970764943,20.));
#83352=CARTESIAN_POINT('Ctrl Pts',(-157.297759889722,224.324341664064,20.));
#83353=CARTESIAN_POINT('Ctrl Pts',(-157.3144940807,224.23163552298,20.));
#83354=CARTESIAN_POINT('Ctrl Pts',(-157.316398369121,224.22108591044,20.));
#83355=CARTESIAN_POINT('Ctrl Pts',(-157.318369356492,224.210548239782,20.));
#83356=CARTESIAN_POINT('Ctrl Pts',(-157.320407241131,224.200023061102,20.));
#83357=CARTESIAN_POINT('Ctrl Pts',(-157.337940451736,224.109468291248,20.));
#83358=CARTESIAN_POINT('Ctrl Pts',(-157.360421180481,224.019837900717,20.));
#83359=CARTESIAN_POINT('Ctrl Pts',(-157.387574525284,223.931369489181,20.));
#83360=CARTESIAN_POINT('Ctrl Pts',(-157.39827477871,223.896506954546,20.));
#83361=CARTESIAN_POINT('Ctrl Pts',(-157.409701215456,223.86182491348,20.));
#83362=CARTESIAN_POINT('Ctrl Pts',(-157.421839179082,223.827338244001,20.));
#83363=CARTESIAN_POINT('Ctrl Pts',(-157.427149562768,223.812250256212,20.));
#83364=CARTESIAN_POINT('Ctrl Pts',(-157.432596153518,223.797199667747,20.));
#83365=CARTESIAN_POINT('Ctrl Pts',(-157.438177793222,223.782187743678,20.));
#83366=CARTESIAN_POINT('Ctrl Pts',(-157.442598536132,223.770298073187,20.));
#83367=CARTESIAN_POINT('Ctrl Pts',(-157.447103592198,223.758433868541,20.));
#83368=CARTESIAN_POINT('Ctrl Pts',(-157.451688653832,223.746604917481,20.));
#83369=CARTESIAN_POINT('Ctrl Pts',(-157.485447014203,223.659512087652,20.));
#83370=CARTESIAN_POINT('Ctrl Pts',(-157.523588345799,223.574194090561,20.));
#83371=CARTESIAN_POINT('Ctrl Pts',(-157.565779381558,223.490881660441,20.));
#83372=CARTESIAN_POINT('Ctrl Pts',(-157.609552743621,223.404444693386,20.));
#83373=CARTESIAN_POINT('Ctrl Pts',(-157.657685386683,223.320165828126,20.));
#83374=CARTESIAN_POINT('Ctrl Pts',(-157.709861207378,223.238305777056,20.));
#83375=CARTESIAN_POINT('Ctrl Pts',(-157.762638726167,223.155501705632,20.));
#83376=CARTESIAN_POINT('Ctrl Pts',(-157.819553623873,223.075171743332,20.));
#83377=CARTESIAN_POINT('Ctrl Pts',(-157.880330640098,222.997600523389,20.));
#83378=CARTESIAN_POINT('Ctrl Pts',(-157.923129908507,222.942974750863,20.));
#83379=CARTESIAN_POINT('Ctrl Pts',(-157.967845501693,222.889717324985,20.));
#83380=CARTESIAN_POINT('Ctrl Pts',(-158.014394714637,222.837935363524,20.));
#83381=CARTESIAN_POINT('Ctrl Pts',(-158.025600881673,222.825469474782,20.));
#83382=CARTESIAN_POINT('Ctrl Pts',(-158.036913959438,222.813088600348,20.));
#83383=CARTESIAN_POINT('Ctrl Pts',(-158.048321553421,222.800806166716,20.));
#83384=CARTESIAN_POINT('Ctrl Pts',(-158.116987843626,222.72687391128,20.));
#83385=CARTESIAN_POINT('Ctrl Pts',(-158.189167078244,222.656402739744,20.));
#83386=CARTESIAN_POINT('Ctrl Pts',(-158.26454612692,222.589679626182,20.));
#83387=CARTESIAN_POINT('Ctrl Pts',(-158.329366085462,222.532303080167,20.));
#83388=CARTESIAN_POINT('Ctrl Pts',(-158.396553232748,222.477698010934,20.));
#83389=CARTESIAN_POINT('Ctrl Pts',(-158.465934682045,222.426062194725,20.));
#83390=CARTESIAN_POINT('Ctrl Pts',(-158.491454388474,222.407069641467,20.));
#83391=CARTESIAN_POINT('Ctrl Pts',(-158.517271175927,222.388478967149,20.));
#83392=CARTESIAN_POINT('Ctrl Pts',(-158.54337715025,222.370300665476,20.));
#83393=CARTESIAN_POINT('Ctrl Pts',(-158.560069624725,222.358677240396,20.));
#83394=CARTESIAN_POINT('Ctrl Pts',(-158.576881381361,222.347221841334,20.));
#83395=CARTESIAN_POINT('Ctrl Pts',(-158.593795571103,222.335946858683,20.));
#83396=CARTESIAN_POINT('Ctrl Pts',(-158.67998923295,222.278490246407,20.));
#83397=CARTESIAN_POINT('Ctrl Pts',(-158.768924553551,222.225655755127,20.));
#83398=CARTESIAN_POINT('Ctrl Pts',(-158.860295170393,222.177762742994,20.));
#83399=CARTESIAN_POINT('Ctrl Pts',(-158.951665787236,222.129869730861,20.));
#83400=CARTESIAN_POINT('Ctrl Pts',(-159.045472338951,222.086917295733,20.));
#83401=CARTESIAN_POINT('Ctrl Pts',(-159.141446276778,222.049265245825,20.));
#83402=CARTESIAN_POINT('Ctrl Pts',(-159.162330715998,222.041071959548,20.));
#83403=CARTESIAN_POINT('Ctrl Pts',(-159.183317906813,222.033129839072,20.));
#83404=CARTESIAN_POINT('Ctrl Pts',(-159.204403754918,222.025437656558,20.));
#83405=CARTESIAN_POINT('Ctrl Pts',(-160.793799282533,222.030777046254,20.));
#83406=CARTESIAN_POINT('Ctrl Pts',(-160.886835157066,222.064809984747,20.));
#83407=CARTESIAN_POINT('Ctrl Pts',(-160.97780402793,222.103614877177,20.));
#83408=CARTESIAN_POINT('Ctrl Pts',(-161.066498354202,222.146862331045,20.));
#83409=CARTESIAN_POINT('Ctrl Pts',(-161.157170998911,222.191074415223,20.));
#83410=CARTESIAN_POINT('Ctrl Pts',(-161.245467167254,222.239930070387,20.));
#83411=CARTESIAN_POINT('Ctrl Pts',(-161.331136191421,222.293122938813,20.));
#83412=CARTESIAN_POINT('Ctrl Pts',(-161.414071427374,222.344618367142,20.));
#83413=CARTESIAN_POINT('Ctrl Pts',(-161.494544838205,222.400179479374,20.));
#83414=CARTESIAN_POINT('Ctrl Pts',(-161.572295307516,222.459559004075,20.));
#83415=CARTESIAN_POINT('Ctrl Pts',(-161.640326968163,222.511516088189,20.));
#83416=CARTESIAN_POINT('Ctrl Pts',(-161.706273580043,222.566397361551,20.));
#83417=CARTESIAN_POINT('Ctrl Pts',(-161.76993497096,222.624050135585,20.));
#83418=CARTESIAN_POINT('Ctrl Pts',(-161.783313758306,222.636166179433,20.));
#83419=CARTESIAN_POINT('Ctrl Pts',(-161.79659343422,222.648406574009,20.));
#83420=CARTESIAN_POINT('Ctrl Pts',(-161.809754846302,222.660753485833,20.));
#83421=CARTESIAN_POINT('Ctrl Pts',(-161.88217975833,222.728696347667,20.));
#83422=CARTESIAN_POINT('Ctrl Pts',(-161.951138910575,222.799961330003,20.));
#83423=CARTESIAN_POINT('Ctrl Pts',(-162.016393085433,222.874256414107,20.));
#83424=CARTESIAN_POINT('Ctrl Pts',(-162.081289619105,222.94814430615,20.));
#83425=CARTESIAN_POINT('Ctrl Pts',(-162.142522161547,223.025029976113,20.));
#83426=CARTESIAN_POINT('Ctrl Pts',(-162.199811787101,223.104652927277,20.));
#83427=CARTESIAN_POINT('Ctrl Pts',(-162.255642502291,223.182248238225,20.));
#83428=CARTESIAN_POINT('Ctrl Pts',(-162.307728826392,223.262443934253,20.));
#83429=CARTESIAN_POINT('Ctrl Pts',(-162.355765810799,223.34501299586,20.));
#83430=CARTESIAN_POINT('Ctrl Pts',(-162.376479699321,223.380617361091,20.));
#83431=CARTESIAN_POINT('Ctrl Pts',(-162.396440032026,223.416663145243,20.));
#83432=CARTESIAN_POINT('Ctrl Pts',(-162.415619383683,223.453132475859,20.));
#83433=CARTESIAN_POINT('Ctrl Pts',(-162.428829714613,223.478251777848,20.));
#83434=CARTESIAN_POINT('Ctrl Pts',(-162.441669497393,223.503572020127,20.));
#83435=CARTESIAN_POINT('Ctrl Pts',(-162.454129239588,223.529087365697,20.));
#83436=CARTESIAN_POINT('Ctrl Pts',(-162.460341884048,223.54180976138,20.));
#83437=CARTESIAN_POINT('Ctrl Pts',(-162.466459488514,223.554579686581,20.));
#83438=CARTESIAN_POINT('Ctrl Pts',(-162.472475687079,223.567384892693,20.));
#83439=CARTESIAN_POINT('Ctrl Pts',(-162.512676218372,223.652949902466,20.));
#83440=CARTESIAN_POINT('Ctrl Pts',(-162.548420147964,223.740225116418,20.));
#83441=CARTESIAN_POINT('Ctrl Pts',(-162.579456437337,223.828972461131,20.));
#83442=CARTESIAN_POINT('Ctrl Pts',(-162.609806694244,223.91575811645,20.));
#83443=CARTESIAN_POINT('Ctrl Pts',(-162.635655345283,224.003952216894,20.));
#83444=CARTESIAN_POINT('Ctrl Pts',(-162.656718497157,224.093340884024,20.));
#83445=CARTESIAN_POINT('Ctrl Pts',(-162.660341411732,224.108715957369,20.));
#83446=CARTESIAN_POINT('Ctrl Pts',(-162.663822623516,224.124126379391,20.));
#83447=CARTESIAN_POINT('Ctrl Pts',(-162.667160529864,224.139571066685,20.));
#83448=CARTESIAN_POINT('Ctrl Pts',(-162.687288121125,224.232702605024,20.));
#83449=CARTESIAN_POINT('Ctrl Pts',(-162.702209079259,224.327081103144,20.));
#83450=CARTESIAN_POINT('Ctrl Pts',(-162.712001705764,224.422298423,20.));
#83451=CARTESIAN_POINT('Ctrl Pts',(-162.715264402153,224.454022823543,20.));
#83452=CARTESIAN_POINT('Ctrl Pts',(-162.717957399902,224.485840220276,20.));
#83453=CARTESIAN_POINT('Ctrl Pts',(-162.720082396037,224.517735059187,20.));
#83454=CARTESIAN_POINT('Ctrl Pts',(-162.721307197425,224.536118548139,20.));
#83455=CARTESIAN_POINT('Ctrl Pts',(-162.722343291264,224.554527759039,20.));
#83456=CARTESIAN_POINT('Ctrl Pts',(-162.723190917022,224.572959665217,20.));
#83457=CARTESIAN_POINT('Ctrl Pts',(-162.723765442786,224.585452920495,20.));
#83458=CARTESIAN_POINT('Ctrl Pts',(-162.724253263129,224.597954978153,20.));
#83459=CARTESIAN_POINT('Ctrl Pts',(-162.72465433353,224.610455508973,20.));
#83460=CARTESIAN_POINT('Ctrl Pts',(-162.727643976961,224.703636480985,20.));
#83461=CARTESIAN_POINT('Ctrl Pts',(-162.725824947473,224.796878671104,20.));
#83462=CARTESIAN_POINT('Ctrl Pts',(-162.719336046552,224.889807660892,20.));
#83463=CARTESIAN_POINT('Ctrl Pts',(-162.71283429417,224.982920699303,20.));
#83464=CARTESIAN_POINT('Ctrl Pts',(-162.701643771368,225.075720275617,20.));
#83465=CARTESIAN_POINT('Ctrl Pts',(-162.685853071485,225.167817711271,20.));
#83466=CARTESIAN_POINT('Ctrl Pts',(-162.670284999373,225.258616696131,20.));
#83467=CARTESIAN_POINT('Ctrl Pts',(-162.650245081355,225.348734045122,20.));
#83468=CARTESIAN_POINT('Ctrl Pts',(-162.625775167407,225.437772128322,20.));
#83469=CARTESIAN_POINT('Ctrl Pts',(-162.616258329812,225.472400814772,20.));
#83470=CARTESIAN_POINT('Ctrl Pts',(-162.606070988221,225.506865913873,20.));
#83471=CARTESIAN_POINT('Ctrl Pts',(-162.595214035973,225.541142570298,20.));
#83472=CARTESIAN_POINT('Ctrl Pts',(-162.589229904893,225.560035165602,20.));
#83473=CARTESIAN_POINT('Ctrl Pts',(-162.583042331939,225.578870496113,20.));
#83474=CARTESIAN_POINT('Ctrl Pts',(-162.576651360682,225.59764427317,20.));
#83475=CARTESIAN_POINT('Ctrl Pts',(-162.57141557596,225.613024635739,20.));
#83476=CARTESIAN_POINT('Ctrl Pts',(-162.566043001402,225.628364205394,20.));
#83477=CARTESIAN_POINT('Ctrl Pts',(-162.560539154716,225.643645943324,20.));
#83478=CARTESIAN_POINT('Ctrl Pts',(-162.528144126739,225.733592549036,20.));
#83479=CARTESIAN_POINT('Ctrl Pts',(-162.491164142524,225.821662858184,20.));
#83480=CARTESIAN_POINT('Ctrl Pts',(-162.449671820276,225.907414022356,20.));
#83481=CARTESIAN_POINT('Ctrl Pts',(-162.41855257859,225.971727395484,20.));
#83482=CARTESIAN_POINT('Ctrl Pts',(-162.384894001541,226.034735713979,20.));
#83483=CARTESIAN_POINT('Ctrl Pts',(-162.348709397534,226.096235055875,20.));
#83484=CARTESIAN_POINT('Ctrl Pts',(-162.334282224949,226.120755473986,20.));
#83485=CARTESIAN_POINT('Ctrl Pts',(-162.319453336099,226.145035821206,20.));
#83486=CARTESIAN_POINT('Ctrl Pts',(-162.304222985861,226.169062364537,20.));
#83487=CARTESIAN_POINT('Ctrl Pts',(-162.293793871983,226.185514747611,20.));
#83488=CARTESIAN_POINT('Ctrl Pts',(-162.283180901156,226.20184108192,20.));
#83489=CARTESIAN_POINT('Ctrl Pts',(-162.27238853677,226.218031444641,20.));
#83490=CARTESIAN_POINT('Ctrl Pts',(-162.224798823911,226.289424022337,20.));
#83491=CARTESIAN_POINT('Ctrl Pts',(-162.173699949597,226.358212848466,20.));
#83492=CARTESIAN_POINT('Ctrl Pts',(-162.11912578658,226.424045448902,20.));
#83493=CARTESIAN_POINT('Ctrl Pts',(-162.068157074919,226.485528807399,20.));
#83494=CARTESIAN_POINT('Ctrl Pts',(-162.014156575569,226.544433773001,20.));
#83495=CARTESIAN_POINT('Ctrl Pts',(-161.957129166719,226.600438933592,20.));
#83496=CARTESIAN_POINT('Ctrl Pts',(-161.943965134441,226.613366993215,20.));
#83497=CARTESIAN_POINT('Ctrl Pts',(-161.930639725161,226.626140375729,20.));
#83498=CARTESIAN_POINT('Ctrl Pts',(-161.917156323069,226.638757682714,20.));
#83499=CARTESIAN_POINT('Ctrl Pts',(-158.086534003335,-223.364012796625,
20.));
#83500=CARTESIAN_POINT('Ctrl Pts',(-158.024938173881,-223.42189775131,20.));
#83501=CARTESIAN_POINT('Ctrl Pts',(-157.966714299078,-223.482934392949,
20.));
#83502=CARTESIAN_POINT('Ctrl Pts',(-157.911858746884,-223.54673766266,20.));
#83503=CARTESIAN_POINT('Ctrl Pts',(-157.8555491723,-223.612232126406,20.));
#83504=CARTESIAN_POINT('Ctrl Pts',(-157.802788416102,-223.680642260279,
20.));
#83505=CARTESIAN_POINT('Ctrl Pts',(-157.753598112148,-223.751600119281,
20.));
#83506=CARTESIAN_POINT('Ctrl Pts',(-157.70270986304,-223.825007293352,20.));
#83507=CARTESIAN_POINT('Ctrl Pts',(-157.655642227354,-223.901141633816,
20.));
#83508=CARTESIAN_POINT('Ctrl Pts',(-157.612454091303,-223.979639766739,
20.));
#83509=CARTESIAN_POINT('Ctrl Pts',(-157.593559281781,-224.013982699893,
20.));
#83510=CARTESIAN_POINT('Ctrl Pts',(-157.575407526715,-224.048778584098,
20.));
#83511=CARTESIAN_POINT('Ctrl Pts',(-157.558006201844,-224.083999079587,
20.));
#83512=CARTESIAN_POINT('Ctrl Pts',(-157.548478231389,-224.103283808936,
20.));
#83513=CARTESIAN_POINT('Ctrl Pts',(-157.539175269563,-224.122695857825,
20.));
#83514=CARTESIAN_POINT('Ctrl Pts',(-157.530098732371,-224.142230703846,
20.));
#83515=CARTESIAN_POINT('Ctrl Pts',(-157.52144257418,-224.160860795237,20.));
#83516=CARTESIAN_POINT('Ctrl Pts',(-157.512989856259,-224.179608589799,
20.));
#83517=CARTESIAN_POINT('Ctrl Pts',(-157.504755930064,-224.198437311969,
20.));
#83518=CARTESIAN_POINT('Ctrl Pts',(-157.468216499089,-224.281992930256,
20.));
#83519=CARTESIAN_POINT('Ctrl Pts',(-157.435936481645,-224.367232201794,
20.));
#83520=CARTESIAN_POINT('Ctrl Pts',(-157.407939572907,-224.453755877463,
20.));
#83521=CARTESIAN_POINT('Ctrl Pts',(-157.37947811424,-224.5417152319,20.));
#83522=CARTESIAN_POINT('Ctrl Pts',(-157.355442590654,-224.631002723839,
20.));
#83523=CARTESIAN_POINT('Ctrl Pts',(-157.335897010016,-224.721236037712,
20.));
#83524=CARTESIAN_POINT('Ctrl Pts',(-157.316695005968,-224.809883210201,
20.));
#83525=CARTESIAN_POINT('Ctrl Pts',(-157.301826226592,-224.899444155411,
20.));
#83526=CARTESIAN_POINT('Ctrl Pts',(-157.291394009147,-224.989579190703,
20.));
#83527=CARTESIAN_POINT('Ctrl Pts',(-157.287260088834,-225.025296530308,
20.));
#83528=CARTESIAN_POINT('Ctrl Pts',(-157.283823320309,-225.06110419823,20.));
#83529=CARTESIAN_POINT('Ctrl Pts',(-157.281092173199,-225.096981595475,
20.));
#83530=CARTESIAN_POINT('Ctrl Pts',(-157.279473970919,-225.118238922047,
20.));
#83531=CARTESIAN_POINT('Ctrl Pts',(-157.27810350346,-225.139520731589,20.));
#83532=CARTESIAN_POINT('Ctrl Pts',(-157.276982736962,-225.160822762524,
20.));
#83533=CARTESIAN_POINT('Ctrl Pts',(-157.276240739759,-225.174925653178,
20.));
#83534=CARTESIAN_POINT('Ctrl Pts',(-157.275608269918,-225.189037319775,
20.));
#83535=CARTESIAN_POINT('Ctrl Pts',(-157.275086239663,-225.203142127781,
20.));
#83536=CARTESIAN_POINT('Ctrl Pts',(-157.271563249445,-225.298330290024,
20.));
#83537=CARTESIAN_POINT('Ctrl Pts',(-157.273057002546,-225.393367647058,
20.));
#83538=CARTESIAN_POINT('Ctrl Pts',(-157.279625569,-225.487854900047,20.));
#83539=CARTESIAN_POINT('Ctrl Pts',(-157.286172402503,-225.582029529748,
20.));
#83540=CARTESIAN_POINT('Ctrl Pts',(-157.297760164404,-225.675658644094,
20.));
#83541=CARTESIAN_POINT('Ctrl Pts',(-157.314494359435,-225.768364796008,
20.));
#83542=CARTESIAN_POINT('Ctrl Pts',(-157.316398648436,-225.778914410441,
20.));
#83543=CARTESIAN_POINT('Ctrl Pts',(-157.318369636371,-225.789452082957,
20.));
#83544=CARTESIAN_POINT('Ctrl Pts',(-157.320407521558,-225.799977263458,
20.));
#83545=CARTESIAN_POINT('Ctrl Pts',(-157.337940736475,-225.890532046898,
20.));
#83546=CARTESIAN_POINT('Ctrl Pts',(-157.360421468074,-225.980162448345,
20.));
#83547=CARTESIAN_POINT('Ctrl Pts',(-157.387574814582,-226.068630868437,
20.));
#83548=CARTESIAN_POINT('Ctrl Pts',(-157.398275070813,-226.103493413393,
20.));
#83549=CARTESIAN_POINT('Ctrl Pts',(-157.409701510474,-226.13817546434,20.));
#83550=CARTESIAN_POINT('Ctrl Pts',(-157.421839477138,-226.172662143273,
20.));
#83551=CARTESIAN_POINT('Ctrl Pts',(-157.427149894992,-226.187750228502,
20.));
#83552=CARTESIAN_POINT('Ctrl Pts',(-157.432596521619,-226.202800913864,
20.));
#83553=CARTESIAN_POINT('Ctrl Pts',(-157.438178198887,-226.217812934261,
20.));
#83554=CARTESIAN_POINT('Ctrl Pts',(-157.442598945982,-226.229702612288,
20.));
#83555=CARTESIAN_POINT('Ctrl Pts',(-157.44710400624,-226.241566824203,20.));
#83556=CARTESIAN_POINT('Ctrl Pts',(-157.451689072148,-226.253395782476,
20.));
#83557=CARTESIAN_POINT('Ctrl Pts',(-157.485447446532,-226.340488620394,
20.));
#83558=CARTESIAN_POINT('Ctrl Pts',(-157.523588791448,-226.425806622743,
20.));
#83559=CARTESIAN_POINT('Ctrl Pts',(-157.565779840137,-226.50911905557,20.));
#83560=CARTESIAN_POINT('Ctrl Pts',(-157.609553211554,-226.595556017415,
20.));
#83561=CARTESIAN_POINT('Ctrl Pts',(-157.657685862741,-226.679834875118,
20.));
#83562=CARTESIAN_POINT('Ctrl Pts',(-157.70986169076,-226.761694916622,20.));
#83563=CARTESIAN_POINT('Ctrl Pts',(-157.762639213503,-226.844498972949,
20.));
#83564=CARTESIAN_POINT('Ctrl Pts',(-157.8195541138,-226.92482891842,20.));
#83565=CARTESIAN_POINT('Ctrl Pts',(-157.880331131737,-227.002400120161,
20.));
#83566=CARTESIAN_POINT('Ctrl Pts',(-157.923130525395,-227.057026038192,
20.));
#83567=CARTESIAN_POINT('Ctrl Pts',(-157.967846254496,-227.110283600964,
20.));
#83568=CARTESIAN_POINT('Ctrl Pts',(-158.01439561348,-227.162065689885,20.));
#83569=CARTESIAN_POINT('Ctrl Pts',(-158.025601560259,-227.174531325184,
20.));
#83570=CARTESIAN_POINT('Ctrl Pts',(-158.036914413278,-227.186911949283,
20.));
#83571=CARTESIAN_POINT('Ctrl Pts',(-158.048321778722,-227.199194136455,
20.));
#83572=CARTESIAN_POINT('Ctrl Pts',(-158.116988059975,-227.273126379872,
20.));
#83573=CARTESIAN_POINT('Ctrl Pts',(-158.189167285521,-227.343597538705,
20.));
#83574=CARTESIAN_POINT('Ctrl Pts',(-158.264546325432,-227.410320639282,
20.));
#83575=CARTESIAN_POINT('Ctrl Pts',(-158.329366267453,-227.467697166178,
20.));
#83576=CARTESIAN_POINT('Ctrl Pts',(-158.396553397789,-227.522302216849,
20.));
#83577=CARTESIAN_POINT('Ctrl Pts',(-158.465934830046,-227.573938015384,
20.));
#83578=CARTESIAN_POINT('Ctrl Pts',(-158.491454566082,-227.592930588839,
20.));
#83579=CARTESIAN_POINT('Ctrl Pts',(-158.517271383963,-227.611521282344,
20.));
#83580=CARTESIAN_POINT('Ctrl Pts',(-158.543377389521,-227.629699602166,
20.));
#83581=CARTESIAN_POINT('Ctrl Pts',(-158.560069805416,-227.641322984153,
20.));
#83582=CARTESIAN_POINT('Ctrl Pts',(-158.576881502645,-227.652778341256,
20.));
#83583=CARTESIAN_POINT('Ctrl Pts',(-158.593795632311,-227.664053283202,
20.));
#83584=CARTESIAN_POINT('Ctrl Pts',(-158.679989281783,-227.721509883872,
20.));
#83585=CARTESIAN_POINT('Ctrl Pts',(-158.76892459091,-227.774344364263,20.));
#83586=CARTESIAN_POINT('Ctrl Pts',(-158.860295197642,-227.822237366675,
20.));
#83587=CARTESIAN_POINT('Ctrl Pts',(-158.951665804375,-227.870130369087,
20.));
#83588=CARTESIAN_POINT('Ctrl Pts',(-159.045472347341,-227.913082795661,
20.));
#83589=CARTESIAN_POINT('Ctrl Pts',(-159.141446278244,-227.950734838636,
20.));
#83590=CARTESIAN_POINT('Ctrl Pts',(-159.162330715886,-227.958928123377,
20.));
#83591=CARTESIAN_POINT('Ctrl Pts',(-159.183317905209,-227.966870242395,
20.));
#83592=CARTESIAN_POINT('Ctrl Pts',(-159.204403751904,-227.974562423528,
20.));
#83593=CARTESIAN_POINT('Ctrl Pts',(-160.793799282533,-227.969222953746,
20.));
#83594=CARTESIAN_POINT('Ctrl Pts',(-160.886835141626,-227.935190020901,
20.));
#83595=CARTESIAN_POINT('Ctrl Pts',(-160.977803997214,-227.896385131945,
20.));
#83596=CARTESIAN_POINT('Ctrl Pts',(-161.066498308592,-227.853137679943,
20.));
#83597=CARTESIAN_POINT('Ctrl Pts',(-161.157170945659,-227.808925593975,
20.));
#83598=CARTESIAN_POINT('Ctrl Pts',(-161.245467106361,-227.760069934564,
20.));
#83599=CARTESIAN_POINT('Ctrl Pts',(-161.331136123072,-227.706877060112,
20.));
#83600=CARTESIAN_POINT('Ctrl Pts',(-161.414071361254,-227.655381620085,
20.));
#83601=CARTESIAN_POINT('Ctrl Pts',(-161.494544773927,-227.599820493561,
20.));
#83602=CARTESIAN_POINT('Ctrl Pts',(-161.57229524478,-227.540440952671,20.));
#83603=CARTESIAN_POINT('Ctrl Pts',(-161.640326906778,-227.488483854392,
20.));
#83604=CARTESIAN_POINT('Ctrl Pts',(-161.706273519779,-227.433602565413,
20.));
#83605=CARTESIAN_POINT('Ctrl Pts',(-161.769934911645,-227.375949774776,
20.));
#83606=CARTESIAN_POINT('Ctrl Pts',(-161.783313710025,-227.363833717628,
20.));
#83607=CARTESIAN_POINT('Ctrl Pts',(-161.796593396817,-227.351593309494,
20.));
#83608=CARTESIAN_POINT('Ctrl Pts',(-161.80975481958,-227.339246383904,20.));
#83609=CARTESIAN_POINT('Ctrl Pts',(-161.882179729091,-227.271303503813,
20.));
#83610=CARTESIAN_POINT('Ctrl Pts',(-161.951138878795,-227.200038502427,
20.));
#83611=CARTESIAN_POINT('Ctrl Pts',(-162.016393051206,-227.125743399203,
20.));
#83612=CARTESIAN_POINT('Ctrl Pts',(-162.081289585469,-227.051855484701,
20.));
#83613=CARTESIAN_POINT('Ctrl Pts',(-162.142522128253,-226.974969791928,
20.));
#83614=CARTESIAN_POINT('Ctrl Pts',(-162.199811753977,-226.895346818353,
20.));
#83615=CARTESIAN_POINT('Ctrl Pts',(-162.255642467028,-226.817751488767,
20.));
#83616=CARTESIAN_POINT('Ctrl Pts',(-162.307728789136,-226.737555774695,
20.));
#83617=CARTESIAN_POINT('Ctrl Pts',(-162.355765771803,-226.65498669632,20.));
#83618=CARTESIAN_POINT('Ctrl Pts',(-162.376479660491,-226.619382322281,
20.));
#83619=CARTESIAN_POINT('Ctrl Pts',(-162.396439993344,-226.583336529519,
20.));
#83620=CARTESIAN_POINT('Ctrl Pts',(-162.415619345134,-226.546867190551,
20.));
#83621=CARTESIAN_POINT('Ctrl Pts',(-162.428829684002,-226.52174786789,20.));
#83622=CARTESIAN_POINT('Ctrl Pts',(-162.441669474272,-226.496427604822,
20.));
#83623=CARTESIAN_POINT('Ctrl Pts',(-162.454129223494,-226.470912238378,
20.));
#83624=CARTESIAN_POINT('Ctrl Pts',(-162.460341865666,-226.458189844148,
20.));
#83625=CARTESIAN_POINT('Ctrl Pts',(-162.466459467892,-226.445419920498,
20.));
#83626=CARTESIAN_POINT('Ctrl Pts',(-162.472475664286,-226.432614715998,
20.));
#83627=CARTESIAN_POINT('Ctrl Pts',(-162.512676194786,-226.3470496878,20.));
#83628=CARTESIAN_POINT('Ctrl Pts',(-162.548420123478,-226.259774457234,
20.));
#83629=CARTESIAN_POINT('Ctrl Pts',(-162.579456411898,-226.171027098414,
20.));
#83630=CARTESIAN_POINT('Ctrl Pts',(-162.6098066676,-226.084241430083,20.));
#83631=CARTESIAN_POINT('Ctrl Pts',(-162.635655317466,-225.996047319049,
20.));
#83632=CARTESIAN_POINT('Ctrl Pts',(-162.656718468256,-225.906658644424,
20.));
#83633=CARTESIAN_POINT('Ctrl Pts',(-162.660341377093,-225.891283593348,
20.));
#83634=CARTESIAN_POINT('Ctrl Pts',(-162.663822583577,-225.875873193796,
20.));
#83635=CARTESIAN_POINT('Ctrl Pts',(-162.667160485068,-225.860428529169,
20.));
#83636=CARTESIAN_POINT('Ctrl Pts',(-162.6872880769,-225.767296989379,20.));
#83637=CARTESIAN_POINT('Ctrl Pts',(-162.702209036311,-225.67291849333,20.));
#83638=CARTESIAN_POINT('Ctrl Pts',(-162.712001664687,-225.577701178491,
20.));
#83639=CARTESIAN_POINT('Ctrl Pts',(-162.715264361927,-225.545976777395,
20.));
#83640=CARTESIAN_POINT('Ctrl Pts',(-162.717957360515,-225.514159380424,
20.));
#83641=CARTESIAN_POINT('Ctrl Pts',(-162.72008235747,-225.48226454157,20.));
#83642=CARTESIAN_POINT('Ctrl Pts',(-162.721307159468,-225.463881050598,
20.));
#83643=CARTESIAN_POINT('Ctrl Pts',(-162.722343253869,-225.445471837771,
20.));
#83644=CARTESIAN_POINT('Ctrl Pts',(-162.72319088014,-225.427039929757,20.));
#83645=CARTESIAN_POINT('Ctrl Pts',(-162.723765406226,-225.414546673798,
20.));
#83646=CARTESIAN_POINT('Ctrl Pts',(-162.724253226876,-225.402044615508,
20.));
#83647=CARTESIAN_POINT('Ctrl Pts',(-162.724654297569,-225.389544084099,
20.));
#83648=CARTESIAN_POINT('Ctrl Pts',(-162.727643942782,-225.296363120045,
20.));
#83649=CARTESIAN_POINT('Ctrl Pts',(-162.725824915524,-225.203120940277,
20.));
#83650=CARTESIAN_POINT('Ctrl Pts',(-162.719336017171,-225.11019196266,20.));
#83651=CARTESIAN_POINT('Ctrl Pts',(-162.712834267359,-225.017078936413,
20.));
#83652=CARTESIAN_POINT('Ctrl Pts',(-162.701643747461,-224.924279374092,
20.));
#83653=CARTESIAN_POINT('Ctrl Pts',(-162.685853050706,-224.832181953698,
20.));
#83654=CARTESIAN_POINT('Ctrl Pts',(-162.670284981152,-224.74138298082,20.));
#83655=CARTESIAN_POINT('Ctrl Pts',(-162.650245065609,-224.65126564509,20.));
#83656=CARTESIAN_POINT('Ctrl Pts',(-162.625775153949,-224.562227575932,
20.));
#83657=CARTESIAN_POINT('Ctrl Pts',(-162.616258314973,-224.52759888668,20.));
#83658=CARTESIAN_POINT('Ctrl Pts',(-162.606070971652,-224.493133784971,
20.));
#83659=CARTESIAN_POINT('Ctrl Pts',(-162.595214017321,-224.458857126123,
20.));
#83660=CARTESIAN_POINT('Ctrl Pts',(-162.589230261228,-224.43996571699,20.));
#83661=CARTESIAN_POINT('Ctrl Pts',(-162.583043088727,-224.421131565508,
20.));
#83662=CARTESIAN_POINT('Ctrl Pts',(-162.576652543383,-224.402358959524,
20.));
#83663=CARTESIAN_POINT('Ctrl Pts',(-162.57141645097,-224.386977627499,20.));
#83664=CARTESIAN_POINT('Ctrl Pts',(-162.56604355117,-224.371637092308,20.));
#83665=CARTESIAN_POINT('Ctrl Pts',(-162.560539362696,-224.356354396001,
20.));
#83666=CARTESIAN_POINT('Ctrl Pts',(-162.528144340813,-224.266407751976,
20.));
#83667=CARTESIAN_POINT('Ctrl Pts',(-162.491164357556,-224.178337405817,
20.));
#83668=CARTESIAN_POINT('Ctrl Pts',(-162.449672031221,-224.092586205957,
20.));
#83669=CARTESIAN_POINT('Ctrl Pts',(-162.41855278647,-224.028272806063,20.));
#83670=CARTESIAN_POINT('Ctrl Pts',(-162.384894203516,-223.965264461546,
20.));
#83671=CARTESIAN_POINT('Ctrl Pts',(-162.348709590758,-223.903765094401,
20.));
#83672=CARTESIAN_POINT('Ctrl Pts',(-162.334282725247,-223.879245194058,
20.));
#83673=CARTESIAN_POINT('Ctrl Pts',(-162.319454160314,-223.854965354395,
20.));
#83674=CARTESIAN_POINT('Ctrl Pts',(-162.304224150818,-223.830939307521,
20.));
#83675=CARTESIAN_POINT('Ctrl Pts',(-162.293794754286,-223.814486450417,
20.));
#83676=CARTESIAN_POINT('Ctrl Pts',(-162.283181489495,-223.798159647794,
20.));
#83677=CARTESIAN_POINT('Ctrl Pts',(-162.272388821235,-223.781968824945,
20.));
#83678=CARTESIAN_POINT('Ctrl Pts',(-162.224799118483,-223.710576243596,
20.));
#83679=CARTESIAN_POINT('Ctrl Pts',(-162.173700253124,-223.64178741277,20.));
#83680=CARTESIAN_POINT('Ctrl Pts',(-162.119126097886,-223.575954806167,
20.));
#83681=CARTESIAN_POINT('Ctrl Pts',(-162.068157305994,-223.514471336365,
20.));
#83682=CARTESIAN_POINT('Ctrl Pts',(-162.014156714983,-223.455566267017,
20.));
#83683=CARTESIAN_POINT('Ctrl Pts',(-161.957129203007,-223.399561011565,
20.));
#83684=CARTESIAN_POINT('Ctrl Pts',(-161.943965171011,-223.3866329537,20.));
#83685=CARTESIAN_POINT('Ctrl Pts',(-161.930639761992,-223.373859572851,
20.));
#83686=CARTESIAN_POINT('Ctrl Pts',(-161.91715636014,-223.361242267443,20.));
#83687=CARTESIAN_POINT('Ctrl Pts',(161.913465996665,-223.364012796625,20.));
#83688=CARTESIAN_POINT('Ctrl Pts',(161.975061812394,-223.421897738412,20.));
#83689=CARTESIAN_POINT('Ctrl Pts',(162.033285672793,-223.482934368139,20.));
#83690=CARTESIAN_POINT('Ctrl Pts',(162.088141210339,-223.546737626713,20.));
#83691=CARTESIAN_POINT('Ctrl Pts',(162.144450771328,-223.612232080702,20.));
#83692=CARTESIAN_POINT('Ctrl Pts',(162.19721151349,-223.680642205787,20.));
#83693=CARTESIAN_POINT('Ctrl Pts',(162.246401803429,-223.751600056706,20.));
#83694=CARTESIAN_POINT('Ctrl Pts',(162.297290050622,-223.825007240568,20.));
#83695=CARTESIAN_POINT('Ctrl Pts',(162.344357682524,-223.901141592927,20.));
#83696=CARTESIAN_POINT('Ctrl Pts',(162.387545813387,-223.979639739294,20.));
#83697=CARTESIAN_POINT('Ctrl Pts',(162.40644062064,-224.013982678329,20.));
#83698=CARTESIAN_POINT('Ctrl Pts',(162.424592373166,-224.048778568712,20.));
#83699=CARTESIAN_POINT('Ctrl Pts',(162.441993695267,-224.083999070632,20.));
#83700=CARTESIAN_POINT('Ctrl Pts',(162.451521671306,-224.103283817873,20.));
#83701=CARTESIAN_POINT('Ctrl Pts',(162.46082463831,-224.122695884918,20.));
#83702=CARTESIAN_POINT('Ctrl Pts',(162.469901180279,-224.142230749344,20.));
#83703=CARTESIAN_POINT('Ctrl Pts',(162.478557342987,-224.160860858206,20.));
#83704=CARTESIAN_POINT('Ctrl Pts',(162.487010065066,-224.179608670477,20.));
#83705=CARTESIAN_POINT('Ctrl Pts',(162.495243995045,-224.198437410524,20.));
#83706=CARTESIAN_POINT('Ctrl Pts',(162.531783408589,-224.281993029878,20.));
#83707=CARTESIAN_POINT('Ctrl Pts',(162.564063409247,-224.367232302693,20.));
#83708=CARTESIAN_POINT('Ctrl Pts',(162.592060302327,-224.453755979522,20.));
#83709=CARTESIAN_POINT('Ctrl Pts',(162.620521747138,-224.541715341508,20.));
#83710=CARTESIAN_POINT('Ctrl Pts',(162.644557257391,-224.631002841067,20.));
#83711=CARTESIAN_POINT('Ctrl Pts',(162.664102825717,-224.721236162207,20.));
#83712=CARTESIAN_POINT('Ctrl Pts',(162.683304819936,-224.809883352301,20.));
#83713=CARTESIAN_POINT('Ctrl Pts',(162.698173589444,-224.899444314992,20.));
#83714=CARTESIAN_POINT('Ctrl Pts',(162.708605797423,-224.989579367119,20.));
#83715=CARTESIAN_POINT('Ctrl Pts',(162.712739714819,-225.0252967206,20.));
#83716=CARTESIAN_POINT('Ctrl Pts',(162.716176480208,-225.061104402333,20.));
#83717=CARTESIAN_POINT('Ctrl Pts',(162.718907623986,-225.09698181328,20.));
#83718=CARTESIAN_POINT('Ctrl Pts',(162.720525823836,-225.118239141982,20.));
#83719=CARTESIAN_POINT('Ctrl Pts',(162.721896288936,-225.139520953601,20.));
#83720=CARTESIAN_POINT('Ctrl Pts',(162.723017053152,-225.160822986555,20.));
#83721=CARTESIAN_POINT('Ctrl Pts',(162.72375904895,-225.174925880562,20.));
#83722=CARTESIAN_POINT('Ctrl Pts',(162.724391517388,-225.189037550495,20.));
#83723=CARTESIAN_POINT('Ctrl Pts',(162.724913546246,-225.203142361806,20.));
#83724=CARTESIAN_POINT('Ctrl Pts',(162.728436526521,-225.298330532454,20.));
#83725=CARTESIAN_POINT('Ctrl Pts',(162.726942765165,-225.393367896624,20.));
#83726=CARTESIAN_POINT('Ctrl Pts',(162.720374192642,-225.487855155009,20.));
#83727=CARTESIAN_POINT('Ctrl Pts',(162.713827352484,-225.582029798809,20.));
#83728=CARTESIAN_POINT('Ctrl Pts',(162.702239585165,-225.675658925426,20.));
#83729=CARTESIAN_POINT('Ctrl Pts',(162.685505386423,-225.768365087207,20.));
#83730=CARTESIAN_POINT('Ctrl Pts',(162.683601096917,-225.778914703222,20.));
#83731=CARTESIAN_POINT('Ctrl Pts',(162.681630108493,-225.789452377287,20.));
#83732=CARTESIAN_POINT('Ctrl Pts',(162.679592222834,-225.799977559304,20.));
#83733=CARTESIAN_POINT('Ctrl Pts',(162.662059003986,-225.890532355132,20.));
#83734=CARTESIAN_POINT('Ctrl Pts',(162.639578269783,-225.98016276653,20.));
#83735=CARTESIAN_POINT('Ctrl Pts',(162.612424921719,-226.068631194424,20.));
#83736=CARTESIAN_POINT('Ctrl Pts',(162.60172466293,-226.10349374879,20.));
#83737=CARTESIAN_POINT('Ctrl Pts',(162.590298220609,-226.138175808748,20.));
#83738=CARTESIAN_POINT('Ctrl Pts',(162.578160251176,-226.172662496298,20.));
#83739=CARTESIAN_POINT('Ctrl Pts',(162.572849802005,-226.187750670834,20.));
#83740=CARTESIAN_POINT('Ctrl Pts',(162.567403142496,-226.202801445002,20.));
#83741=CARTESIAN_POINT('Ctrl Pts',(162.5618214308,-226.217813553686,20.));
#83742=CARTESIAN_POINT('Ctrl Pts',(162.55740067986,-226.22970323864,20.));
#83743=CARTESIAN_POINT('Ctrl Pts',(162.55289561575,-226.241567457238,20.));
#83744=CARTESIAN_POINT('Ctrl Pts',(162.548310545917,-226.253396422141,20.));
#83745=CARTESIAN_POINT('Ctrl Pts',(162.514552158695,-226.34048926743,20.));
#83746=CARTESIAN_POINT('Ctrl Pts',(162.476410801576,-226.425807274567,20.));
#83747=CARTESIAN_POINT('Ctrl Pts',(162.434219741038,-226.509119709854,20.));
#83748=CARTESIAN_POINT('Ctrl Pts',(162.390446361034,-226.595556666934,20.));
#83749=CARTESIAN_POINT('Ctrl Pts',(162.342313702381,-226.67983551773,20.));
#83750=CARTESIAN_POINT('Ctrl Pts',(162.290137867628,-226.761695550495,20.));
#83751=CARTESIAN_POINT('Ctrl Pts',(162.237360341227,-226.844499593035,20.));
#83752=CARTESIAN_POINT('Ctrl Pts',(162.180445438513,-226.924829523137,20.));
#83753=CARTESIAN_POINT('Ctrl Pts',(162.119668418965,-227.002400708259,20.));
#83754=CARTESIAN_POINT('Ctrl Pts',(162.076868910637,-227.057026759491,20.));
#83755=CARTESIAN_POINT('Ctrl Pts',(162.032153057103,-227.110284447588,20.));
#83756=CARTESIAN_POINT('Ctrl Pts',(161.98560356442,-227.162066653199,20.));
#83757=CARTESIAN_POINT('Ctrl Pts',(161.974397819258,-227.174532056505,20.));
#83758=CARTESIAN_POINT('Ctrl Pts',(161.963085171963,-227.186912451454,20.));
#83759=CARTESIAN_POINT('Ctrl Pts',(161.951678015715,-227.199194413025,20.));
#83760=CARTESIAN_POINT('Ctrl Pts',(161.883011742611,-227.273126645486,20.));
#83761=CARTESIAN_POINT('Ctrl Pts',(161.810832525324,-227.343597792739,20.));
#83762=CARTESIAN_POINT('Ctrl Pts',(161.735453493392,-227.410320881478,20.));
#83763=CARTESIAN_POINT('Ctrl Pts',(161.670633566439,-227.46769739093,20.));
#83764=CARTESIAN_POINT('Ctrl Pts',(161.603446451563,-227.522302424667,20.));
#83765=CARTESIAN_POINT('Ctrl Pts',(161.534065034849,-227.573938207076,20.));
#83766=CARTESIAN_POINT('Ctrl Pts',(161.508545271754,-227.592930798994,20.));
#83767=CARTESIAN_POINT('Ctrl Pts',(161.48272842606,-227.611521510039,20.));
#83768=CARTESIAN_POINT('Ctrl Pts',(161.456622391953,-227.629699846453,20.));
#83769=CARTESIAN_POINT('Ctrl Pts',(161.439930029612,-227.641323189046,20.));
#83770=CARTESIAN_POINT('Ctrl Pts',(161.423118386691,-227.652778507793,20.));
#83771=CARTESIAN_POINT('Ctrl Pts',(161.406204311947,-227.66405341253,20.));
#83772=CARTESIAN_POINT('Ctrl Pts',(161.320010673739,-227.721510002638,20.));
#83773=CARTESIAN_POINT('Ctrl Pts',(161.231075375052,-227.774344473118,20.));
#83774=CARTESIAN_POINT('Ctrl Pts',(161.139704777517,-227.822237466682,20.));
#83775=CARTESIAN_POINT('Ctrl Pts',(161.048334179982,-227.870130460245,20.));
#83776=CARTESIAN_POINT('Ctrl Pts',(160.954527644971,-227.913082879032,20.));
#83777=CARTESIAN_POINT('Ctrl Pts',(160.858553720359,-227.950734915697,20.));
#83778=CARTESIAN_POINT('Ctrl Pts',(160.837669284155,-227.958928199038,20.));
#83779=CARTESIAN_POINT('Ctrl Pts',(160.816682096193,-227.966870316727,20.));
#83780=CARTESIAN_POINT('Ctrl Pts',(160.795596250783,-227.974562496599,20.));
#83781=CARTESIAN_POINT('Ctrl Pts',(159.206200717467,-227.969222953746,20.));
#83782=CARTESIAN_POINT('Ctrl Pts',(159.113164807739,-227.935190002378,20.));
#83783=CARTESIAN_POINT('Ctrl Pts',(159.022195902054,-227.89638510203,20.));
#83784=CARTESIAN_POINT('Ctrl Pts',(158.933501541831,-227.853137643908,20.));
#83785=CARTESIAN_POINT('Ctrl Pts',(158.842828879704,-227.808925563812,20.));
#83786=CARTESIAN_POINT('Ctrl Pts',(158.754532693946,-227.76006991833,20.));
#83787=CARTESIAN_POINT('Ctrl Pts',(158.668863652786,-227.706877063639,20.));
#83788=CARTESIAN_POINT('Ctrl Pts',(158.585928421912,-227.655381661977,20.));
#83789=CARTESIAN_POINT('Ctrl Pts',(158.505455015278,-227.599820582323,20.));
#83790=CARTESIAN_POINT('Ctrl Pts',(158.427704549483,-227.540441094521,20.));
#83791=CARTESIAN_POINT('Ctrl Pts',(158.359672891912,-227.488484042695,20.));
#83792=CARTESIAN_POINT('Ctrl Pts',(158.293726282585,-227.433602804933,20.));
#83793=CARTESIAN_POINT('Ctrl Pts',(158.230064893832,-227.375950068741,20.));
#83794=CARTESIAN_POINT('Ctrl Pts',(158.216686131675,-227.363834055246,20.));
#83795=CARTESIAN_POINT('Ctrl Pts',(158.203406480592,-227.351593691606,20.));
#83796=CARTESIAN_POINT('Ctrl Pts',(158.190245092894,-227.3392468112,20.));
#83797=CARTESIAN_POINT('Ctrl Pts',(158.117820175126,-227.271303990985,20.));
#83798=CARTESIAN_POINT('Ctrl Pts',(158.048861017085,-227.200039052072,20.));
#83799=CARTESIAN_POINT('Ctrl Pts',(157.983606836642,-227.125744011552,20.));
#83800=CARTESIAN_POINT('Ctrl Pts',(157.918710304314,-227.051856170708,20.));
#83801=CARTESIAN_POINT('Ctrl Pts',(157.857477762648,-226.974970552741,20.));
#83802=CARTESIAN_POINT('Ctrl Pts',(157.800188137478,-226.895347652663,20.));
#83803=CARTESIAN_POINT('Ctrl Pts',(157.744357417399,-226.817752384185,20.));
#83804=CARTESIAN_POINT('Ctrl Pts',(157.692271088743,-226.737556729277,20.));
#83805=CARTESIAN_POINT('Ctrl Pts',(157.644234100355,-226.654987705877,20.));
#83806=CARTESIAN_POINT('Ctrl Pts',(157.623520212217,-226.619383360731,20.));
#83807=CARTESIAN_POINT('Ctrl Pts',(157.603559879849,-226.583337596211,20.));
#83808=CARTESIAN_POINT('Ctrl Pts',(157.584380528496,-226.54686828464,20.));
#83809=CARTESIAN_POINT('Ctrl Pts',(157.571170215891,-226.521749030213,20.));
#83810=CARTESIAN_POINT('Ctrl Pts',(157.558330450404,-226.496428835769,20.));
#83811=CARTESIAN_POINT('Ctrl Pts',(157.545870724434,-226.470913538237,20.));
#83812=CARTESIAN_POINT('Ctrl Pts',(157.539658074865,-226.458191139478,20.));
#83813=CARTESIAN_POINT('Ctrl Pts',(157.533540465395,-226.44542121098,20.));
#83814=CARTESIAN_POINT('Ctrl Pts',(157.527524261978,-226.432616001431,20.));
#83815=CARTESIAN_POINT('Ctrl Pts',(157.487323728804,-226.347051033682,20.));
#83816=CARTESIAN_POINT('Ctrl Pts',(157.451579797078,-226.259775857621,20.));
#83817=CARTESIAN_POINT('Ctrl Pts',(157.420543505454,-226.171028545081,20.));
#83818=CARTESIAN_POINT('Ctrl Pts',(157.390193245719,-226.084242919436,20.));
#83819=CARTESIAN_POINT('Ctrl Pts',(157.364344591923,-225.996048843143,20.));
#83820=CARTESIAN_POINT('Ctrl Pts',(157.343281437493,-225.906660193104,20.));
#83821=CARTESIAN_POINT('Ctrl Pts',(157.339658509642,-225.891285068221,20.));
#83822=CARTESIAN_POINT('Ctrl Pts',(157.336177285591,-225.875874594203,20.));
#83823=CARTESIAN_POINT('Ctrl Pts',(157.332839368005,-225.860429854456,20.));
#83824=CARTESIAN_POINT('Ctrl Pts',(157.312711778046,-225.767298319419,20.));
#83825=CARTESIAN_POINT('Ctrl Pts',(157.297790822823,-225.672919816567,20.));
#83826=CARTESIAN_POINT('Ctrl Pts',(157.287998200584,-225.57770248527,20.));
#83827=CARTESIAN_POINT('Ctrl Pts',(157.284735506138,-225.545978085985,20.));
#83828=CARTESIAN_POINT('Ctrl Pts',(157.2820425103,-225.514160689795,20.));
#83829=CARTESIAN_POINT('Ctrl Pts',(157.279917516036,-225.482265850753,20.));
#83830=CARTESIAN_POINT('Ctrl Pts',(157.278692716036,-225.463882366374,20.));
#83831=CARTESIAN_POINT('Ctrl Pts',(157.277656623476,-225.445473159836,20.));
#83832=CARTESIAN_POINT('Ctrl Pts',(157.276808998887,-225.427041257816,20.));
#83833=CARTESIAN_POINT('Ctrl Pts',(157.276234473842,-225.414548003757,20.));
#83834=CARTESIAN_POINT('Ctrl Pts',(157.275746654189,-225.402045947204,20.));
#83835=CARTESIAN_POINT('Ctrl Pts',(157.275345584448,-225.389545417394,20.));
#83836=CARTESIAN_POINT('Ctrl Pts',(157.272355945115,-225.296364427232,20.));
#83837=CARTESIAN_POINT('Ctrl Pts',(157.274174979727,-225.203122213506,20.));
#83838=CARTESIAN_POINT('Ctrl Pts',(157.280663886537,-225.110193195966,20.));
#83839=CARTESIAN_POINT('Ctrl Pts',(157.287165644814,-225.017080129825,20.));
#83840=CARTESIAN_POINT('Ctrl Pts',(157.298356174273,-224.924280521615,20.));
#83841=CARTESIAN_POINT('Ctrl Pts',(157.314146881321,-224.832183051177,20.));
#83842=CARTESIAN_POINT('Ctrl Pts',(157.329714959299,-224.741384039015,20.));
#83843=CARTESIAN_POINT('Ctrl Pts',(157.349754882989,-224.651266659807,20.));
#83844=CARTESIAN_POINT('Ctrl Pts',(157.374224802182,-224.562228544611,20.));
#83845=CARTESIAN_POINT('Ctrl Pts',(157.383741636739,-224.527599864197,20.));
#83846=CARTESIAN_POINT('Ctrl Pts',(157.393928974511,-224.493134770686,20.));
#83847=CARTESIAN_POINT('Ctrl Pts',(157.404785922147,-224.458858119435,20.));
#83848=CARTESIAN_POINT('Ctrl Pts',(157.410770895666,-224.439962859281,20.));
#83849=CARTESIAN_POINT('Ctrl Pts',(157.416959368274,-224.421124879963,20.));
#83850=CARTESIAN_POINT('Ctrl Pts',(157.423351296383,-224.402348471971,20.));
#83851=CARTESIAN_POINT('Ctrl Pts',(157.428586390486,-224.386970285439,20.));
#83852=CARTESIAN_POINT('Ctrl Pts',(157.433958235031,-224.371632883023,20.));
#83853=CARTESIAN_POINT('Ctrl Pts',(157.439461314568,-224.356353296267,20.));
#83854=CARTESIAN_POINT('Ctrl Pts',(157.471856356384,-224.266406776585,20.));
#83855=CARTESIAN_POINT('Ctrl Pts',(157.508836342851,-224.17833655052,20.));
#83856=CARTESIAN_POINT('Ctrl Pts',(157.550328655963,-224.09258546646,20.));
#83857=CARTESIAN_POINT('Ctrl Pts',(157.581447890797,-224.028272153415,20.));
#83858=CARTESIAN_POINT('Ctrl Pts',(157.615106454581,-223.96526389333,20.));
#83859=CARTESIAN_POINT('Ctrl Pts',(157.651291038901,-223.903764608115,20.));
#83860=CARTESIAN_POINT('Ctrl Pts',(157.665718904402,-223.879243021583,20.));
#83861=CARTESIAN_POINT('Ctrl Pts',(157.680548524169,-223.854961528985,20.));
#83862=CARTESIAN_POINT('Ctrl Pts',(157.695779643291,-223.830933865326,20.));
#83863=CARTESIAN_POINT('Ctrl Pts',(157.706208119446,-223.814482551703,20.));
#83864=CARTESIAN_POINT('Ctrl Pts',(157.71682042703,-223.798157273954,20.));
#83865=CARTESIAN_POINT('Ctrl Pts',(157.727612105819,-223.781967949323,20.));
#83866=CARTESIAN_POINT('Ctrl Pts',(157.775201841441,-223.710575379717,20.));
#83867=CARTESIAN_POINT('Ctrl Pts',(157.8263007359,-223.641786564049,20.));
#83868=CARTESIAN_POINT('Ctrl Pts',(157.88087491638,-223.575953977412,20.));
#83869=CARTESIAN_POINT('Ctrl Pts',(157.931843447117,-223.514470869724,20.));
#83870=CARTESIAN_POINT('Ctrl Pts',(157.985843739753,-223.45556613791,20.));
#83871=CARTESIAN_POINT('Ctrl Pts',(158.04287091602,-223.399561191111,20.));
#83872=CARTESIAN_POINT('Ctrl Pts',(158.056034948939,-223.386633127483,20.));
#83873=CARTESIAN_POINT('Ctrl Pts',(158.069360358813,-223.373859741172,20.));
#83874=CARTESIAN_POINT('Ctrl Pts',(158.082843761452,-223.361242430594,20.));
#83875=CARTESIAN_POINT('Ctrl Pts',(1.91346599666507,226.635987203375,20.));
#83876=CARTESIAN_POINT('Ctrl Pts',(1.97507202942767,226.578092660085,20.));
#83877=CARTESIAN_POINT('Ctrl Pts',(2.03330661763037,226.517047147721,20.));
#83878=CARTESIAN_POINT('Ctrl Pts',(2.08817306581981,226.453235567918,20.));
#83879=CARTESIAN_POINT('Ctrl Pts',(2.14449273668366,226.387733839805,20.));
#83880=CARTESIAN_POINT('Ctrl Pts',(2.19726391938203,226.31931714486,20.));
#83881=CARTESIAN_POINT('Ctrl Pts',(2.24646463424728,226.248353232921,20.));
#83882=CARTESIAN_POINT('Ctrl Pts',(2.29735431518303,226.174953266143,20.));
#83883=CARTESIAN_POINT('Ctrl Pts',(2.34442476753679,226.098827676128,20.));
#83884=CARTESIAN_POINT('Ctrl Pts',(2.38761675533576,226.020339422889,20.));
#83885=CARTESIAN_POINT('Ctrl Pts',(2.40651324999781,225.986000812098,20.));
#83886=CARTESIAN_POINT('Ctrl Pts',(2.4246668885704,225.951209466731,20.));
#83887=CARTESIAN_POINT('Ctrl Pts',(2.44207026698428,225.915993693173,20.));
#83888=CARTESIAN_POINT('Ctrl Pts',(2.45159411457209,225.896722167146,20.));
#83889=CARTESIAN_POINT('Ctrl Pts',(2.46089325218288,225.877323516596,20.));
#83890=CARTESIAN_POINT('Ctrl Pts',(2.46996626160065,225.857802251082,20.));
#83891=CARTESIAN_POINT('Ctrl Pts',(2.47861902358291,225.839185179688,20.));
#83892=CARTESIAN_POINT('Ctrl Pts',(2.48706861295929,225.820450582116,20.));
#83893=CARTESIAN_POINT('Ctrl Pts',(2.49529968930897,225.801635180991,20.));
#83894=CARTESIAN_POINT('Ctrl Pts',(2.53185203011613,225.718080257535,20.));
#83895=CARTESIAN_POINT('Ctrl Pts',(2.56414446983256,225.6328418152,20.));
#83896=CARTESIAN_POINT('Ctrl Pts',(2.59215295014503,225.546318858556,20.));
#83897=CARTESIAN_POINT('Ctrl Pts',(2.62062462394071,225.458365018508,20.));
#83898=CARTESIAN_POINT('Ctrl Pts',(2.64466996545821,225.369083071526,20.));
#83899=CARTESIAN_POINT('Ctrl Pts',(2.66422459333411,225.278855014715,20.));
#83900=CARTESIAN_POINT('Ctrl Pts',(2.68343383284957,225.190220632855,20.));
#83901=CARTESIAN_POINT('Ctrl Pts',(2.69830984962651,225.100672357925,20.));
#83902=CARTESIAN_POINT('Ctrl Pts',(2.70874897441918,225.010549484523,20.));
#83903=CARTESIAN_POINT('Ctrl Pts',(2.71288502035126,224.974842243607,20.));
#83904=CARTESIAN_POINT('Ctrl Pts',(2.71632406879747,224.939044621295,20.));
#83905=CARTESIAN_POINT('Ctrl Pts',(2.7190576333604,224.903177183262,20.));
#83906=CARTESIAN_POINT('Ctrl Pts',(2.72067759764398,224.881921431946,20.));
#83907=CARTESIAN_POINT('Ctrl Pts',(2.72204977456521,224.860641157351,20.));
#83908=CARTESIAN_POINT('Ctrl Pts',(2.72317219338359,224.839340616697,20.));
#83909=CARTESIAN_POINT('Ctrl Pts',(2.72391521405841,224.825240049394,20.));
#83910=CARTESIAN_POINT('Ctrl Pts',(2.7245487028823,224.811130692204,20.));
#83911=CARTESIAN_POINT('Ctrl Pts',(2.72507174573303,224.797028170696,20.));
#83912=CARTESIAN_POINT('Ctrl Pts',(2.72860191891809,224.701846020323,20.));
#83913=CARTESIAN_POINT('Ctrl Pts',(2.72711407425655,224.606813701877,20.));
#83914=CARTESIAN_POINT('Ctrl Pts',(2.72054976732745,224.512330159547,20.));
#83915=CARTESIAN_POINT('Ctrl Pts',(2.71400763276353,224.418165755798,20.));
#83916=CARTESIAN_POINT('Ctrl Pts',(2.70242363100706,224.324545473338,20.));
#83917=CARTESIAN_POINT('Ctrl Pts',(2.68569190358529,224.23184632802,20.));
#83918=CARTESIAN_POINT('Ctrl Pts',(2.68378789808642,224.221297525857,20.));
#83919=CARTESIAN_POINT('Ctrl Pts',(2.6818171771052,224.210760641935,20.));
#83920=CARTESIAN_POINT('Ctrl Pts',(2.67977954180341,224.200236225707,20.));
#83921=CARTESIAN_POINT('Ctrl Pts',(2.66224892193235,224.109690316875,20.));
#83922=CARTESIAN_POINT('Ctrl Pts',(2.63976977371118,224.020066944523,20.));
#83923=CARTESIAN_POINT('Ctrl Pts',(2.61261721716453,223.93160392846,20.));
#83924=CARTESIAN_POINT('Ctrl Pts',(2.60191875644486,223.896748348623,20.));
#83925=CARTESIAN_POINT('Ctrl Pts',(2.590494190504,223.862072960234,20.));
#83926=CARTESIAN_POINT('Ctrl Pts',(2.57835818302837,223.827592647788,20.));
#83927=CARTESIAN_POINT('Ctrl Pts',(2.5730714188911,223.812572116558,20.));
#83928=CARTESIAN_POINT('Ctrl Pts',(2.56764962929132,223.797588608551,20.));
#83929=CARTESIAN_POINT('Ctrl Pts',(2.56209395823295,223.782643373109,20.));
#83930=CARTESIAN_POINT('Ctrl Pts',(2.55767501123199,223.770756023652,20.));
#83931=CARTESIAN_POINT('Ctrl Pts',(2.55317171629538,223.758893969826,20.));
#83932=CARTESIAN_POINT('Ctrl Pts',(2.54858843359649,223.747067146183,20.));
#83933=CARTESIAN_POINT('Ctrl Pts',(2.51483910385201,223.659979484958,20.));
#83934=CARTESIAN_POINT('Ctrl Pts',(2.47670633871247,223.574664722143,20.));
#83935=CARTESIAN_POINT('Ctrl Pts',(2.43452361875301,223.491353789882,20.));
#83936=CARTESIAN_POINT('Ctrl Pts',(2.39075605743655,223.404912793674,20.));
#83937=CARTESIAN_POINT('Ctrl Pts',(2.34262838247497,223.320628308811,20.));
#83938=CARTESIAN_POINT('Ctrl Pts',(2.29045699662235,223.238761286965,20.));
#83939=CARTESIAN_POINT('Ctrl Pts',(2.23768158870514,223.155946437364,20.));
#83940=CARTESIAN_POINT('Ctrl Pts',(2.18076788377723,223.075604536594,20.));
#83941=CARTESIAN_POINT('Ctrl Pts',(2.11999147971506,222.998020474552,20.));
#83942=CARTESIAN_POINT('Ctrl Pts',(2.07727586754496,222.94349189959,20.));
#83943=CARTESIAN_POINT('Ctrl Pts',(2.03265108574106,222.890325910386,20.));
#83944=CARTESIAN_POINT('Ctrl Pts',(1.98619948137722,222.838629076086,20.));
#83945=CARTESIAN_POINT('Ctrl Pts',(1.97483618125597,222.825982652964,20.));
#83946=CARTESIAN_POINT('Ctrl Pts',(1.96336276466422,222.81342349125,20.));
#83947=CARTESIAN_POINT('Ctrl Pts',(1.95179211158417,222.800965553175,20.));
#83948=CARTESIAN_POINT('Ctrl Pts',(1.88311823323209,222.727025480997,20.));
#83949=CARTESIAN_POINT('Ctrl Pts',(1.81093139290505,222.656546115043,20.));
#83950=CARTESIAN_POINT('Ctrl Pts',(1.73554501731834,222.589814716556,20.));
#83951=CARTESIAN_POINT('Ctrl Pts',(1.67071531821197,222.532428001103,20.));
#83952=CARTESIAN_POINT('Ctrl Pts',(1.60351838516032,222.477812989059,20.));
#83953=CARTESIAN_POINT('Ctrl Pts',(1.53412731892236,222.426167665699,20.));
#83954=CARTESIAN_POINT('Ctrl Pts',(1.50861557622552,222.407180175343,20.));
#83955=CARTESIAN_POINT('Ctrl Pts',(1.48280704293535,222.388594260749,20.));
#83956=CARTESIAN_POINT('Ctrl Pts',(1.4567096131704,222.370420411812,20.));
#83957=CARTESIAN_POINT('Ctrl Pts',(1.43999802584827,222.35878271928,20.));
#83958=CARTESIAN_POINT('Ctrl Pts',(1.42316691333928,222.347313414893,20.));
#83959=CARTESIAN_POINT('Ctrl Pts',(1.40623317545358,222.336024928434,20.));
#83960=CARTESIAN_POINT('Ctrl Pts',(1.32003063638968,222.278559990595,20.));
#83961=CARTESIAN_POINT('Ctrl Pts',(1.23108709539103,222.225717754617,20.));
#83962=CARTESIAN_POINT('Ctrl Pts',(1.13970924141191,222.177817900273,20.));
#83963=CARTESIAN_POINT('Ctrl Pts',(1.0483313874328,222.129918045928,20.));
#83964=CARTESIAN_POINT('Ctrl Pts',(0.954518581207992,222.086959670452,20.));
#83965=CARTESIAN_POINT('Ctrl Pts',(0.858539701362015,222.049302906438,20.));
#83966=CARTESIAN_POINT('Ctrl Pts',(0.83765419207808,222.041108596444,20.));
#83967=CARTESIAN_POINT('Ctrl Pts',(0.816665993434418,222.033165510218,20.));
#83968=CARTESIAN_POINT('Ctrl Pts',(0.795579197825938,222.025472417912,20.));
#83969=CARTESIAN_POINT('Ctrl Pts',(-0.793799282532863,222.030777046254,
20.));
#83970=CARTESIAN_POINT('Ctrl Pts',(-0.886846243364189,222.064814040164,
20.));
#83971=CARTESIAN_POINT('Ctrl Pts',(-0.977826097699112,222.103621433571,
20.));
#83972=CARTESIAN_POINT('Ctrl Pts',(-1.06653114531038,222.146870245696,20.));
#83973=CARTESIAN_POINT('Ctrl Pts',(-1.15720925843237,222.191081040729,20.));
#83974=CARTESIAN_POINT('Ctrl Pts',(-1.24551090929842,222.23993365004,20.));
#83975=CARTESIAN_POINT('Ctrl Pts',(-1.3311852948319,222.293122208313,20.));
#83976=CARTESIAN_POINT('Ctrl Pts',(-1.41411898609942,222.344609282814,20.));
#83977=CARTESIAN_POINT('Ctrl Pts',(-1.49459113824758,222.40016019587,20.));
#83978=CARTESIAN_POINT('Ctrl Pts',(-1.57234056875799,222.459528180822,20.));
#83979=CARTESIAN_POINT('Ctrl Pts',(-1.6403713204546,222.511475167654,20.));
#83980=CARTESIAN_POINT('Ctrl Pts',(-1.70631719179868,222.566345316816,20.));
#83981=CARTESIAN_POINT('Ctrl Pts',(-1.76997796704167,222.623986279521,20.));
#83982=CARTESIAN_POINT('Ctrl Pts',(-1.78334888221234,222.636092830529,20.));
#83983=CARTESIAN_POINT('Ctrl Pts',(-1.79662079780618,222.64832354999,20.));
#83984=CARTESIAN_POINT('Ctrl Pts',(-1.80977458978086,222.660660637269,20.));
#83985=CARTESIAN_POINT('Ctrl Pts',(-1.88220131303961,222.728590463733,20.));
#83986=CARTESIAN_POINT('Ctrl Pts',(-1.95116230195733,222.799841861522,20.));
#83987=CARTESIAN_POINT('Ctrl Pts',(-2.01641825200817,222.874123335633,20.));
#83988=CARTESIAN_POINT('Ctrl Pts',(-2.08131436524733,222.947995204048,20.));
#83989=CARTESIAN_POINT('Ctrl Pts',(-2.1425466731571,223.024864622427,20.));
#83990=CARTESIAN_POINT('Ctrl Pts',(-2.1998361920632,223.10447163777,20.));
#83991=CARTESIAN_POINT('Ctrl Pts',(-2.25566854673307,223.182053841282,20.));
#83992=CARTESIAN_POINT('Ctrl Pts',(-2.30775639825841,223.262236891238,20.));
#83993=CARTESIAN_POINT('Ctrl Pts',(-2.35579471799653,223.344794263963,20.));
#83994=CARTESIAN_POINT('Ctrl Pts',(-2.37650846819571,223.380392361587,20.));
#83995=CARTESIAN_POINT('Ctrl Pts',(-2.39646867876236,223.416432025931,20.));
#83996=CARTESIAN_POINT('Ctrl Pts',(-2.41564792066214,223.452895427602,20.));
#83997=CARTESIAN_POINT('Ctrl Pts',(-2.42885140531378,223.477997773503,20.));
#83998=CARTESIAN_POINT('Ctrl Pts',(-2.44168472738545,223.503300944244,20.));
#83999=CARTESIAN_POINT('Ctrl Pts',(-2.45413840792515,223.528799126159,20.));
#84000=CARTESIAN_POINT('Ctrl Pts',(-2.46035290716359,223.541522949576,20.));
#84001=CARTESIAN_POINT('Ctrl Pts',(-2.46647232871111,223.554294379828,20.));
#84002=CARTESIAN_POINT('Ctrl Pts',(-2.47249028915989,223.56710113792,20.));
#84003=CARTESIAN_POINT('Ctrl Pts',(-2.51269161001993,223.652653144387,20.));
#84004=CARTESIAN_POINT('Ctrl Pts',(-2.54843641035125,223.739916698538,20.));
#84005=CARTESIAN_POINT('Ctrl Pts',(-2.57947360880066,223.828654231103,20.));
#84006=CARTESIAN_POINT('Ctrl Pts',(-2.60982495439825,223.915430862143,20.));
#84007=CARTESIAN_POINT('Ctrl Pts',(-2.63567467167773,224.003617722926,20.));
#84008=CARTESIAN_POINT('Ctrl Pts',(-2.6567388257605,224.093001424021,20.));
#84009=CARTESIAN_POINT('Ctrl Pts',(-2.66036646980286,224.108394980747,20.));
#84010=CARTESIAN_POINT('Ctrl Pts',(-2.66385205248285,224.123824042632,20.));
#84011=CARTESIAN_POINT('Ctrl Pts',(-2.66719396486238,224.13928752477,20.));
#84012=CARTESIAN_POINT('Ctrl Pts',(-2.6873211089196,224.23241855194,20.));
#84013=CARTESIAN_POINT('Ctrl Pts',(-2.70224110124294,224.326799119115,20.));
#84014=CARTESIAN_POINT('Ctrl Pts',(-2.7120323266871,224.422020654949,20.));
#84015=CARTESIAN_POINT('Ctrl Pts',(-2.71529438038166,224.453744749603,20.));
#84016=CARTESIAN_POINT('Ctrl Pts',(-2.71798674853152,224.485562068786,20.));
#84017=CARTESIAN_POINT('Ctrl Pts',(-2.72011113094023,224.517457045106,20.));
#84018=CARTESIAN_POINT('Ctrl Pts',(-2.72133545868555,224.535838813042,20.));
#84019=CARTESIAN_POINT('Ctrl Pts',(-2.722371121112,224.554246369289,20.));
#84020=CARTESIAN_POINT('Ctrl Pts',(-2.7232183581693,224.572676685511,20.));
#84021=CARTESIAN_POINT('Ctrl Pts',(-2.72379264716902,224.585169443914,20.));
#84022=CARTESIAN_POINT('Ctrl Pts',(-2.72428024263059,224.597671042088,20.));
#84023=CARTESIAN_POINT('Ctrl Pts',(-2.7246810999333,224.610171143549,20.));
#84024=CARTESIAN_POINT('Ctrl Pts',(-2.72766946102712,224.703358461389,20.));
#84025=CARTESIAN_POINT('Ctrl Pts',(-2.72584881895818,224.796608735442,20.));
#84026=CARTESIAN_POINT('Ctrl Pts',(-2.71935806060957,224.88954711861,20.));
#84027=CARTESIAN_POINT('Ctrl Pts',(-2.71285445289211,224.982669486376,20.));
#84028=CARTESIAN_POINT('Ctrl Pts',(-2.70166183707515,225.075479708117,20.));
#84029=CARTESIAN_POINT('Ctrl Pts',(-2.68586888947921,225.167588686864,20.));
#84030=CARTESIAN_POINT('Ctrl Pts',(-2.67029900027931,225.258396725369,20.));
#84031=CARTESIAN_POINT('Ctrl Pts',(-2.65025734363534,225.348524036092,20.));
#84032=CARTESIAN_POINT('Ctrl Pts',(-2.62578584634267,225.437572618048,20.));
#84033=CARTESIAN_POINT('Ctrl Pts',(-2.61627032324279,225.472198363604,20.));
#84034=CARTESIAN_POINT('Ctrl Pts',(-2.60608459160239,225.506660669287,20.));
#84035=CARTESIAN_POINT('Ctrl Pts',(-2.59522954905329,225.540934672887,20.));
#84036=CARTESIAN_POINT('Ctrl Pts',(-2.58886565516187,225.561028202799,20.));
#84037=CARTESIAN_POINT('Ctrl Pts',(-2.5822717015305,225.581056995775,20.));
#84038=CARTESIAN_POINT('Ctrl Pts',(-2.57544773877719,225.601015886081,20.));
#84039=CARTESIAN_POINT('Ctrl Pts',(-2.57041723007358,225.615729238868,20.));
#84040=CARTESIAN_POINT('Ctrl Pts',(-2.56526191645706,225.630403812104,20.));
#84041=CARTESIAN_POINT('Ctrl Pts',(-2.5599864272113,225.645025393398,20.));
#84042=CARTESIAN_POINT('Ctrl Pts',(-2.52758251764902,225.734836285968,20.));
#84043=CARTESIAN_POINT('Ctrl Pts',(-2.49060722777199,225.822773889061,20.));
#84044=CARTESIAN_POINT('Ctrl Pts',(-2.44913270809182,225.90839658293,20.));
#84045=CARTESIAN_POINT('Ctrl Pts',(-2.41802681833168,225.972613603331,20.));
#84046=CARTESIAN_POINT('Ctrl Pts',(-2.38438897400814,226.035527952701,20.));
#84047=CARTESIAN_POINT('Ctrl Pts',(-2.34823239730369,226.096936292273,20.));
#84048=CARTESIAN_POINT('Ctrl Pts',(-2.33710865887614,226.115828852602,20.));
#84049=CARTESIAN_POINT('Ctrl Pts',(-2.32574642144184,226.134578744948,20.));
#84050=CARTESIAN_POINT('Ctrl Pts',(-2.31414581792787,226.153179704593,20.));
#84051=CARTESIAN_POINT('Ctrl Pts',(-2.30316198797025,226.170791700172,20.));
#84052=CARTESIAN_POINT('Ctrl Pts',(-2.29196345883308,226.188271460635,20.));
#84053=CARTESIAN_POINT('Ctrl Pts',(-2.28056228114764,226.205595973582,20.));
#84054=CARTESIAN_POINT('Ctrl Pts',(-2.23334092463296,226.277350578666,20.));
#84055=CARTESIAN_POINT('Ctrl Pts',(-2.18260256041263,226.346516008461,20.));
#84056=CARTESIAN_POINT('Ctrl Pts',(-2.12838300135328,226.41274085809,20.));
#84057=CARTESIAN_POINT('Ctrl Pts',(-2.07470009109681,226.47831023418,20.));
#84058=CARTESIAN_POINT('Ctrl Pts',(-2.01760419713431,226.540997538338,20.));
#84059=CARTESIAN_POINT('Ctrl Pts',(-1.95710196343274,226.600419914749,20.));
#84060=CARTESIAN_POINT('Ctrl Pts',(-1.94393772146859,226.613349198402,20.));
#84061=CARTESIAN_POINT('Ctrl Pts',(-1.93061211823694,226.626123733867,20.));
#84062=CARTESIAN_POINT('Ctrl Pts',(-1.91712853756743,226.638742124992,20.));
#84063=CARTESIAN_POINT('Origin',(160.,-225.,22.2084234471774));
#84064=CARTESIAN_POINT('Ctrl Pts',(156.923621975382,-224.997773684101,19.7084234471775));
#84065=CARTESIAN_POINT('Ctrl Pts',(156.922437084912,-224.853669211175,19.7009407276991));
#84066=CARTESIAN_POINT('Ctrl Pts',(156.997172963777,-223.691638871918,19.6405387198101));
#84067=CARTESIAN_POINT('Ctrl Pts',(158.478135150588,-221.701106223228,19.5272174235105));
#84068=CARTESIAN_POINT('Ctrl Pts',(161.945877027117,-221.932389138002,19.3684595582787));
#84069=CARTESIAN_POINT('Ctrl Pts',(163.63266934599,-224.970773983768,19.2097016930469));
#84070=CARTESIAN_POINT('Ctrl Pts',(161.994882807082,-228.036087395469,19.0509438278151));
#84071=CARTESIAN_POINT('Ctrl Pts',(158.531360332167,-228.322686556747,18.8921859625833));
#84072=CARTESIAN_POINT('Ctrl Pts',(157.007146995965,-226.341897506019,18.7780125023707));
#84073=CARTESIAN_POINT('Ctrl Pts',(156.922679362106,-225.163035208244,18.7167583305688));
#84074=CARTESIAN_POINT('Ctrl Pts',(156.924068591467,-225.002427532313,18.7084234471774));
#84075=CARTESIAN_POINT('Ctrl Pts',(156.929637641087,-225.003026239314,19.7915765528225));
#84076=CARTESIAN_POINT('Ctrl Pts',(156.934919294579,-224.29968971933,19.7552124583938));
#84077=CARTESIAN_POINT('Ctrl Pts',(157.522174149263,-222.562575364414,19.6659290755545));
#84078=CARTESIAN_POINT('Ctrl Pts',(160.407275465985,-221.390670340075,19.5237264043046));
#84079=CARTESIAN_POINT('Ctrl Pts',(163.253011317767,-223.383220872305,19.3649685390728));
#84080=CARTESIAN_POINT('Ctrl Pts',(163.122801873322,-226.856577342785,19.2062106738411));
#84081=CARTESIAN_POINT('Ctrl Pts',(160.134021031603,-228.6302491553,19.0474528086092));
#84082=CARTESIAN_POINT('Ctrl Pts',(157.42551199164,-227.28218313637,18.9092414349364));
#84083=CARTESIAN_POINT('Ctrl Pts',(156.933644953762,-225.625342150596,18.8239493496742));
#84084=CARTESIAN_POINT('Ctrl Pts',(156.93039533859,-224.998257313349,18.7915765528225));
#84085=CARTESIAN_POINT('Ctrl Pts',(161.913465996665,-223.364012796625,20.));
#84086=CARTESIAN_POINT('Ctrl Pts',(162.457434515453,-224.000243484621,19.9470807115894));
#84087=CARTESIAN_POINT('Ctrl Pts',(162.850433814982,-225.848044833187,19.8412421347682));
#84088=CARTESIAN_POINT('Ctrl Pts',(160.831717845445,-227.858697877144,19.6824842695364));
#84089=CARTESIAN_POINT('Ctrl Pts',(158.050453908468,-227.24740924583,19.5237264043046));
#84090=CARTESIAN_POINT('Ctrl Pts',(157.054009795468,-224.582054764982,19.3649685390728));
#84091=CARTESIAN_POINT('Ctrl Pts',(158.753442408201,-222.297880239784,19.206210673841));
#84092=CARTESIAN_POINT('Ctrl Pts',(161.593865435422,-222.48732378556,19.0474528086093));
#84093=CARTESIAN_POINT('Ctrl Pts',(162.975514910861,-224.976061006714,18.8886949433774));
#84094=CARTESIAN_POINT('Ctrl Pts',(161.634006008404,-227.486855382494,18.7299370781457));
#84095=CARTESIAN_POINT('Ctrl Pts',(158.79703908776,-227.72160839649,18.5711792129139));
#84096=CARTESIAN_POINT('Ctrl Pts',(157.061029552932,-225.465579927985,18.4124213476821));
#84097=CARTESIAN_POINT('Ctrl Pts',(158.014761990161,-222.783436142778,18.2536634824503));
#84098=CARTESIAN_POINT('Ctrl Pts',(160.785385942383,-222.129899504983,18.0949056172185));
#84099=CARTESIAN_POINT('Ctrl Pts',(162.837223859747,-224.10307487572,17.9361477519867));
#84100=CARTESIAN_POINT('Ctrl Pts',(162.29243502248,-226.897117941075,17.7773898867549));
#84101=CARTESIAN_POINT('Ctrl Pts',(159.649609545089,-227.954917846864,17.6186320215231));
#84102=CARTESIAN_POINT('Ctrl Pts',(157.327461493527,-226.30837748647,17.4598741562913));
#84103=CARTESIAN_POINT('Ctrl Pts',(157.451220532081,-223.464409894173,17.3011162910595));
#84104=CARTESIAN_POINT('Ctrl Pts',(159.907622461572,-222.025814406454,17.1423584258277));
#84105=CARTESIAN_POINT('Ctrl Pts',(162.448568299937,-223.309193408747,16.9836005605959));
#84106=CARTESIAN_POINT('Ctrl Pts',(162.748584531626,-226.139998560115,16.8248426953641));
#84107=CARTESIAN_POINT('Ctrl Pts',(160.53309630558,-227.927477062891,16.6660848301324));
#84108=CARTESIAN_POINT('Ctrl Pts',(157.829718362824,-227.035728678229,16.5073269649006));
#84109=CARTESIAN_POINT('Ctrl Pts',(157.112582088492,-224.280881484703,16.3485690996688));
#84110=CARTESIAN_POINT('Ctrl Pts',(159.038010573505,-222.184171529352,16.189811234437));
#84111=CARTESIAN_POINT('Ctrl Pts',(161.843851743683,-222.664507679004,16.0310533692052));
#84112=CARTESIAN_POINT('Ctrl Pts',(162.962199870615,-225.282286309282,15.8722955039734));
#84113=CARTESIAN_POINT('Ctrl Pts',(161.369542792414,-227.641716520265,15.7135376387416));
#84114=CARTESIAN_POINT('Ctrl Pts',(158.523480204468,-227.583447875852,15.5547797735098));
#84115=CARTESIAN_POINT('Ctrl Pts',(157.028728475322,-225.160807837019,15.396021908278));
#84116=CARTESIAN_POINT('Ctrl Pts',(158.253284328723,-222.590996472085,15.2372640430462));
#84117=CARTESIAN_POINT('Ctrl Pts',(161.076434295787,-222.22590504116,15.0785061778144));
#84118=CARTESIAN_POINT('Ctrl Pts',(162.914431637677,-224.39966520748,14.9197483125826));
#84119=CARTESIAN_POINT('Ctrl Pts',(162.085141259372,-227.122851752306,14.7609904473509));
#84120=CARTESIAN_POINT('Ctrl Pts',(159.347529682486,-227.903204456901,14.6022325821191));
#84121=CARTESIAN_POINT('Ctrl Pts',(157.207058914531,-226.026544556706,14.4434747168873));
#84122=CARTESIAN_POINT('Ctrl Pts',(157.622687718167,-223.210391118582,14.2847168516555));
#84123=CARTESIAN_POINT('Ctrl Pts',(160.214032628651,-222.032087658357,14.1259589864237));
#84124=CARTESIAN_POINT('Ctrl Pts',(162.609494885811,-223.570017456494,13.9672011211919));
#84125=CARTESIAN_POINT('Ctrl Pts',(162.616747526092,-226.416667222215,13.8084432559601));
#84126=CARTESIAN_POINT('Ctrl Pts',(160.229152933395,-227.966783201874,13.6496853907283));
#84127=CARTESIAN_POINT('Ctrl Pts',(157.631837585066,-226.801699311844,13.4909275254965));
#84128=CARTESIAN_POINT('Ctrl Pts',(157.201864385759,-223.987700282465,13.3321696602647));
#84129=CARTESIAN_POINT('Ctrl Pts',(159.332744790571,-222.100157914766,13.1734117950329));
#84130=CARTESIAN_POINT('Ctrl Pts',(162.074297136814,-222.86655090944,13.0146539298011));
#84131=CARTESIAN_POINT('Ctrl Pts',(162.917452825014,-225.585476427899,12.8558960645693));
#84132=CARTESIAN_POINT('Ctrl Pts',(161.090555802487,-227.768573942568,12.6971381993376));
#84133=CARTESIAN_POINT('Ctrl Pts',(158.26558215241,-227.417872693871,12.5383803341057));
#84134=CARTESIAN_POINT('Ctrl Pts',(157.027947648243,-224.854334450823,12.379622468874));
#84135=CARTESIAN_POINT('Ctrl Pts',(158.51033533953,-222.424109312655,12.2208646036422));
#84136=CARTESIAN_POINT('Ctrl Pts',(161.356064069501,-222.35133923025,12.0621067384104));
#84137=CARTESIAN_POINT('Ctrl Pts',(162.96072301639,-224.702623380164,11.9033488731786));
#84138=CARTESIAN_POINT('Ctrl Pts',(161.855728375107,-227.326066600858,11.7445910079468));
#84139=CARTESIAN_POINT('Ctrl Pts',(159.052371197901,-227.820693759917,11.585833142715));
#84140=CARTESIAN_POINT('Ctrl Pts',(157.116283863111,-225.733822100821,11.4270752774832));
#84141=CARTESIAN_POINT('Ctrl Pts',(157.819373423403,-222.97535648391,11.2683174122514));
#84142=CARTESIAN_POINT('Ctrl Pts',(160.518172340845,-222.069844533308,11.1095595470196));
#84143=CARTESIAN_POINT('Ctrl Pts',(162.742739952322,-223.846010750597,10.9508016817878));
#84144=CARTESIAN_POINT('Ctrl Pts',(162.457152067289,-226.67830788356,10.792043816556));
#84145=CARTESIAN_POINT('Ctrl Pts',(159.922778706899,-227.974617707487,10.6332859513243));
#84146=CARTESIAN_POINT('Ctrl Pts',(157.459078270917,-226.548557522496,10.4745280860924));
#84147=CARTESIAN_POINT('Ctrl Pts',(157.320829301473,-223.705257553812,10.3157702208607));
#84148=CARTESIAN_POINT('Ctrl Pts',(159.634557249965,-222.046905820965,10.1570123556289));
#84149=CARTESIAN_POINT('Ctrl Pts',(162.282738388918,-223.091225764643,9.99825449039707));
#84150=CARTESIAN_POINT('Ctrl Pts',(162.8417574441,-225.882455813459,9.83949662516529));
#84151=CARTESIAN_POINT('Ctrl Pts',(160.800000198191,-227.866062336499,9.68073875993349));
#84152=CARTESIAN_POINT('Ctrl Pts',(158.026082802357,-227.226648721881,9.52198089470171));
#84153=CARTESIAN_POINT('Ctrl Pts',(157.058694348183,-224.549406284558,9.36322302946991));
#84154=CARTESIAN_POINT('Ctrl Pts',(158.783188710889,-222.284547197889,9.20446516423812));
#84155=CARTESIAN_POINT('Ctrl Pts',(161.621308717539,-222.504870408929,9.04570729900632));
#84156=CARTESIAN_POINT('Ctrl Pts',(162.975607049654,-225.008736123599,8.88694943377453));
#84157=CARTESIAN_POINT('Ctrl Pts',(161.606629926939,-227.504606538295,8.72819156854274));
#84158=CARTESIAN_POINT('Ctrl Pts',(158.767265158268,-227.708261147634,8.56943370331095));
#84159=CARTESIAN_POINT('Ctrl Pts',(157.056099268275,-225.433315261159,8.41067583807915));
#84160=CARTESIAN_POINT('Ctrl Pts',(158.03919121219,-222.76179926471,8.25191797284736));
#84161=CARTESIAN_POINT('Ctrl Pts',(160.816815281602,-222.138684493184,8.09316010761556));
#84162=CARTESIAN_POINT('Ctrl Pts',(162.846890037412,-224.134245560977,7.93440224238378));
#84163=CARTESIAN_POINT('Ctrl Pts',(162.271491142934,-226.922145057319,7.77564437715198));
#84164=CARTESIAN_POINT('Ctrl Pts',(159.617223643767,-227.950897472789,7.6168865119202));
#84165=CARTESIAN_POINT('Ctrl Pts',(157.313273050772,-226.278988637203,7.45812864668839));
#84166=CARTESIAN_POINT('Ctrl Pts',(157.468214856058,-223.436549451145,7.29937078145661));
#84167=CARTESIAN_POINT('Ctrl Pts',(159.940246325519,-222.024980145917,7.14061291622482));
#84168=CARTESIAN_POINT('Ctrl Pts',(162.466964355516,-223.336148894156,6.98185505099302));
#84169=CARTESIAN_POINT('Ctrl Pts',(162.735916704355,-226.170074109035,6.82309718576123));
#84170=CARTESIAN_POINT('Ctrl Pts',(160.500958192956,-227.933147545337,6.66433932052944));
#84171=CARTESIAN_POINT('Ctrl Pts',(157.807522763063,-227.01180446349,6.50558145529765));
#84172=CARTESIAN_POINT('Ctrl Pts',(157.120642414198,-224.249258015769,6.34682359006585));
#84173=CARTESIAN_POINT('Ctrl Pts',(159.06895001463,-222.173790602495,6.18806572483406));
#84174=CARTESIAN_POINT('Ctrl Pts',(161.869354525061,-222.684869918679,6.02930785960226));
#84175=CARTESIAN_POINT('Ctrl Pts',(162.958925847666,-225.314756194248,5.87054999437047));
#84176=CARTESIAN_POINT('Ctrl Pts',(161.340488350845,-227.656577613219,5.71179212913869));
#84177=CARTESIAN_POINT('Ctrl Pts',(158.495235968043,-227.567099305039,5.55303426390689));
#84178=CARTESIAN_POINT('Ctrl Pts',(157.027143568115,-225.128211813837,5.3942763986751));
#84179=CARTESIAN_POINT('Ctrl Pts',(158.279809257744,-222.571984875653,5.2355185334433));
#84180=CARTESIAN_POINT('Ctrl Pts',(161.10679344704,-222.237877283792,5.07676066821151));
#84181=CARTESIAN_POINT('Ctrl Pts',(162.920840317129,-224.431664293187,4.91800280297972));
#84182=CARTESIAN_POINT('Ctrl Pts',(162.061734243841,-227.145592119108,4.75924493774793));
#84183=CARTESIAN_POINT('Ctrl Pts',(159.315729071664,-227.895874121996,4.60048707251614));
#84184=CARTESIAN_POINT('Ctrl Pts',(157.195968626195,-225.995852242308,4.44172920728434));
#84185=CARTESIAN_POINT('Ctrl Pts',(157.64245758376,-223.184426429626,4.28297134205255));
#84186=CARTESIAN_POINT('Ctrl Pts',(160.246569267972,-222.034613477144,4.12421347682076));
#84187=CARTESIAN_POINT('Ctrl Pts',(162.625020767807,-223.598722153791,3.96545561158897));
#84188=CARTESIAN_POINT('Ctrl Pts',(162.601053364222,-226.445280260137,3.80669774635717));
#84189=CARTESIAN_POINT('Ctrl Pts',(160.19660202388,-227.969117929339,3.64793988112538));
#84190=CARTESIAN_POINT('Ctrl Pts',(157.612220519232,-226.775618986163,3.48918201589359));
#84191=CARTESIAN_POINT('Ctrl Pts',(157.213134701033,-223.957073617098,3.3304241506618));
#84192=CARTESIAN_POINT('Ctrl Pts',(159.364587895797,-222.093014431776,3.17166628543));
#84193=CARTESIAN_POINT('Ctrl Pts',(162.097570221393,-222.889428325998,3.01290842019821));
#84194=CARTESIAN_POINT('Ctrl Pts',(162.910856366896,-225.617437329495,2.85415055496642));
#84195=CARTESIAN_POINT('Ctrl Pts',(161.060126871497,-227.78036772115,2.69539268973463));
#84196=CARTESIAN_POINT('Ctrl Pts',(158.239169322395,-227.398705667494,2.53663482450284));
#84197=CARTESIAN_POINT('Ctrl Pts',(157.02972390408,-224.821748314993,2.37787695927104));
#84198=CARTESIAN_POINT('Ctrl Pts',(158.538675126888,-222.407926827632,2.21911909403925));
#84199=CARTESIAN_POINT('Ctrl Pts',(161.385030660596,-222.366370750881,2.06036122880746));
#84200=CARTESIAN_POINT('Ctrl Pts',(162.96380651088,-224.735111758081,1.90160336357567));
#84201=CARTESIAN_POINT('Ctrl Pts',(161.830106089352,-227.346279099041,1.74284549834387));
#84202=CARTESIAN_POINT('Ctrl Pts',(159.021494036293,-227.810130603545,1.58408763311208));
#84203=CARTESIAN_POINT('Ctrl Pts',(157.108407719473,-225.702153382141,1.42532976788029));
#84204=CARTESIAN_POINT('Ctrl Pts',(157.841712527075,-222.951559827016,1.2665719026485));
#84205=CARTESIAN_POINT('Ctrl Pts',(160.55026952987,-222.07571022901,1.1078140374167));
#84206=CARTESIAN_POINT('Ctrl Pts',(162.755245642935,-223.876146461489,0.94905617218491));
#84207=CARTESIAN_POINT('Ctrl Pts',(162.438567593097,-226.705183319779,0.790298306953122));
#84208=CARTESIAN_POINT('Ctrl Pts',(159.890223508887,-227.973532899909,0.631540441721324));
#84209=CARTESIAN_POINT('Ctrl Pts',(157.442116673283,-226.520720196198,0.472782576489534));
#84210=CARTESIAN_POINT('Ctrl Pts',(157.335462206895,-223.675698352418,0.314024711257741));
#84211=CARTESIAN_POINT('Ctrl Pts',(159.666401148433,-222.043601838811,0.155266846025946));
#84212=CARTESIAN_POINT('Ctrl Pts',(162.304705428334,-223.115261021833,-0.0034910192058423));
#84213=CARTESIAN_POINT('Ctrl Pts',(162.829415850734,-225.915728625906,-0.162248884437638));
#84214=CARTESIAN_POINT('Ctrl Pts',(161.458872983031,-227.215894200354,-0.268087461258832));
#84215=CARTESIAN_POINT('Ctrl Pts',(160.650199997975,-227.432086802035,-0.32100674966943));
#84216=CARTESIAN_POINT('Ctrl Pts',(162.054331550342,-223.243574678773,20.1070022498898));
#84217=CARTESIAN_POINT('Ctrl Pts',(162.638345947507,-223.926643402192,20.0540829614792));
#84218=CARTESIAN_POINT('Ctrl Pts',(163.060277072331,-225.910476203892,19.948244384658));
#84219=CARTESIAN_POINT('Ctrl Pts',(160.892947255847,-228.069149518281,19.7894865194262));
#84220=CARTESIAN_POINT('Ctrl Pts',(157.906932210104,-227.412859036056,19.6307286541944));
#84221=CARTESIAN_POINT('Ctrl Pts',(156.837131867137,-224.551286469627,19.4719707889626));
#84222=CARTESIAN_POINT('Ctrl Pts',(158.66167332233,-222.098955567599,19.3132129237308));
#84223=CARTESIAN_POINT('Ctrl Pts',(161.711202632654,-222.302345569707,19.1544550584991));
#84224=CARTESIAN_POINT('Ctrl Pts',(163.194566389237,-224.974298665732,18.9956971932673));
#84225=CARTESIAN_POINT('Ctrl Pts',(161.75429827463,-227.669932720152,18.8369393280355));
#84226=CARTESIAN_POINT('Ctrl Pts',(158.708479502562,-227.921967783242,18.6781814628037));
#84227=CARTESIAN_POINT('Ctrl Pts',(156.844668405157,-225.499854994514,18.5194235975719));
#84228=CARTESIAN_POINT('Ctrl Pts',(157.868612723895,-222.620257128595,18.3606657323401));
#84229=CARTESIAN_POINT('Ctrl Pts',(160.843204490409,-221.918608425839,18.2019078671083));
#84230=CARTESIAN_POINT('Ctrl Pts',(163.046094626516,-224.037045035389,18.0431500018765));
#84231=CARTESIAN_POINT('Ctrl Pts',(162.461199520659,-227.036779983476,17.8843921366447));
#84232=CARTESIAN_POINT('Ctrl Pts',(159.623814498028,-228.172453010433,17.7256342714129));
#84233=CARTESIAN_POINT('Ctrl Pts',(157.130714534295,-226.404697629797,17.5668764061811));
#84234=CARTESIAN_POINT('Ctrl Pts',(157.26358446665,-223.35136281058,17.4081185409493));
#84235=CARTESIAN_POINT('Ctrl Pts',(159.900821811276,-221.806860789769,17.2493606757176));
#84236=CARTESIAN_POINT('Ctrl Pts',(162.628827018873,-223.184719596799,17.0906028104858));
#84237=CARTESIAN_POINT('Ctrl Pts',(162.950929847691,-226.223922982415,16.931844945254));
#84238=CARTESIAN_POINT('Ctrl Pts',(160.572341793286,-228.142992090625,16.7730870800222));
#84239=CARTESIAN_POINT('Ctrl Pts',(157.669946553453,-227.185594966888,16.6143292147904));
#84240=CARTESIAN_POINT('Ctrl Pts',(156.900016135656,-224.227941412607,16.4555713495586));
#84241=CARTESIAN_POINT('Ctrl Pts',(158.9671908289,-221.976875848494,16.2968134843268));
#84242=CARTESIAN_POINT('Ctrl Pts',(161.979592434777,-222.492573388309,16.138055619095));
#84243=CARTESIAN_POINT('Ctrl Pts',(163.180271122261,-225.303067664855,15.9792977538632));
#84244=CARTESIAN_POINT('Ctrl Pts',(161.47036580368,-227.836194426292,15.8205398886314));
#84245=CARTESIAN_POINT('Ctrl Pts',(158.414781759407,-227.77363616039,15.6617820233996));
#84246=CARTESIAN_POINT('Ctrl Pts',(156.80998938658,-225.172646189535,15.5030241581678));
#84247=CARTESIAN_POINT('Ctrl Pts',(158.124694601715,-222.413650432824,15.344266292936));
#84248=CARTESIAN_POINT('Ctrl Pts',(161.155679243613,-222.021681698278,15.1855084277043));
#84249=CARTESIAN_POINT('Ctrl Pts',(163.128986287204,-224.355469756353,15.0267505624724));
#84250=CARTESIAN_POINT('Ctrl Pts',(162.238645203789,-227.279131868066,14.8679926972407));
#84251=CARTESIAN_POINT('Ctrl Pts',(159.2994961179,-228.116932583751,14.7092348320089));
#84252=CARTESIAN_POINT('Ctrl Pts',(157.001448157361,-226.102116721357,14.5504769667771));
#84253=CARTESIAN_POINT('Ctrl Pts',(157.447674725291,-223.078643678917,14.3917191015453));
#84254=CARTESIAN_POINT('Ctrl Pts',(160.229789284266,-221.813595865977,14.2329612363135));
#84255=CARTESIAN_POINT('Ctrl Pts',(162.801600699318,-223.464744991192,14.0742033710817));
#84256=CARTESIAN_POINT('Ctrl Pts',(162.809387264524,-226.520959440096,13.9154455058499));
#84257=CARTESIAN_POINT('Ctrl Pts',(160.246022715714,-228.185191869234,13.7566876406181));
#84258=CARTESIAN_POINT('Ctrl Pts',(157.457498187158,-226.934336824904,13.5979297753863));
#84259=CARTESIAN_POINT('Ctrl Pts',(156.995871217733,-223.913176794487,13.4391719101545));
#84260=CARTESIAN_POINT('Ctrl Pts',(159.283622791705,-221.886677319018,13.2804140449227));
#84261=CARTESIAN_POINT('Ctrl Pts',(162.227002758537,-222.709490638754,13.1216561796909));
#84262=CARTESIAN_POINT('Ctrl Pts',(163.132229888331,-225.628578035831,12.9628983144592));
#84263=CARTESIAN_POINT('Ctrl Pts',(161.170840347497,-227.972390839234,12.8041404492274));
#84264=CARTESIAN_POINT('Ctrl Pts',(158.137897766675,-227.595871663456,12.6453825839956));
#84265=CARTESIAN_POINT('Ctrl Pts',(156.809151076567,-224.843610843364,12.4866247187638));
#84266=CARTESIAN_POINT('Ctrl Pts',(158.400669195708,-222.234477373275,12.327866853532));
#84267=CARTESIAN_POINT('Ctrl Pts',(161.455894804045,-222.156350102414,12.1691089883002));
#84268=CARTESIAN_POINT('Ctrl Pts',(163.178685544971,-224.680731106,12.0103511230684));
#84269=CARTESIAN_POINT('Ctrl Pts',(161.992343400139,-227.49730698882,11.8515932578366));
#84270=CARTESIAN_POINT('Ctrl Pts',(158.982608653847,-228.028347613676,11.6928353926048));
#84271=CARTESIAN_POINT('Ctrl Pts',(156.903990427546,-225.787844621583,11.534077527373));
#84272=CARTESIAN_POINT('Ctrl Pts',(157.658840040207,-222.826306262798,11.3753196621412));
#84273=CARTESIAN_POINT('Ctrl Pts',(160.556319156007,-221.854132326822,11.2165617969094));
#84274=CARTESIAN_POINT('Ctrl Pts',(162.944655002106,-223.76105636163,11.0578039316776));
#84275=CARTESIAN_POINT('Ctrl Pts',(162.638042706073,-226.801861565554,10.8990460664459));
#84276=CARTESIAN_POINT('Ctrl Pts',(159.917093829181,-228.193603135539,10.7402882012141));
#84277=CARTESIAN_POINT('Ctrl Pts',(157.272020676562,-226.662559241464,10.5815303359823));
#84278=CARTESIAN_POINT('Ctrl Pts',(157.123594093479,-223.60994119498,10.4227724707505));
#84279=CARTESIAN_POINT('Ctrl Pts',(159.607654082932,-221.829504912187,10.2640146055187));
#84280=CARTESIAN_POINT('Ctrl Pts',(162.450789040257,-222.950705609084,10.1052567402869));
#84281=CARTESIAN_POINT('Ctrl Pts',(163.050961964314,-225.94742045196,9.9464988750551));
#84282=CARTESIAN_POINT('Ctrl Pts',(160.858894618607,-228.077056134459,9.7877410098233));
#84283=CARTESIAN_POINT('Ctrl Pts',(157.880766951726,-227.390570163703,9.62898314459151));
#84284=CARTESIAN_POINT('Ctrl Pts',(156.842161287288,-224.516234473133,9.47022527935971));
#84285=CARTESIAN_POINT('Ctrl Pts',(158.693609488546,-222.084640973728,9.31146741412793));
#84286=CARTESIAN_POINT('Ctrl Pts',(161.740666234513,-222.321183940523,9.15270954889614));
#84287=CARTESIAN_POINT('Ctrl Pts',(163.194665311105,-225.00937925961,8.99395168366434));
#84288=CARTESIAN_POINT('Ctrl Pts',(161.7249068206,-227.688990680671,8.83519381843255));
#84289=CARTESIAN_POINT('Ctrl Pts',(158.676513675713,-227.907637936523,8.67643595320076));
#84290=CARTESIAN_POINT('Ctrl Pts',(156.839375162768,-225.46521506721,8.51767808796896));
#84291=CARTESIAN_POINT('Ctrl Pts',(157.89484037657,-222.59702738668,8.35892022273718));
#84292=CARTESIAN_POINT('Ctrl Pts',(160.876947594951,-221.928040147366,8.20016235750537));
#84293=CARTESIAN_POINT('Ctrl Pts',(163.056472408918,-224.070510444381,8.04140449227359));
#84294=CARTESIAN_POINT('Ctrl Pts',(162.438713794436,-227.063649546147,7.88264662704179));
#84295=CARTESIAN_POINT('Ctrl Pts',(159.589044411186,-228.16813666443,7.72388876181001));
#84296=CARTESIAN_POINT('Ctrl Pts',(157.115481566658,-226.373145232011,7.56513089657821));
#84297=CARTESIAN_POINT('Ctrl Pts',(157.281829878894,-223.321451337253,7.40637303134642));
#84298=CARTESIAN_POINT('Ctrl Pts',(159.935847379076,-221.805965112634,7.24761516611462));
#84299=CARTESIAN_POINT('Ctrl Pts',(162.648577355406,-223.213659491329,7.08885730088284));
#84300=CARTESIAN_POINT('Ctrl Pts',(162.937329440221,-226.256212633314,6.93009943565103));
#84301=CARTESIAN_POINT('Ctrl Pts',(160.537837736853,-228.149080022689,6.77134157041925));
#84302=CARTESIAN_POINT('Ctrl Pts',(157.646116957868,-227.159909499134,6.61258370518745));
#84303=CARTESIAN_POINT('Ctrl Pts',(156.908669846477,-224.193989886907,6.45382583995567));
#84304=CARTESIAN_POINT('Ctrl Pts',(159.000407970027,-221.965730698488,6.29506797472386));
#84305=CARTESIAN_POINT('Ctrl Pts',(162.0069726801,-222.514434655492,6.13631010949208));
#84306=CARTESIAN_POINT('Ctrl Pts',(163.176756072268,-225.337927918048,5.97755224426028));
#84307=CARTESIAN_POINT('Ctrl Pts',(161.439172432019,-227.852149563295,5.8187943790285));
#84308=CARTESIAN_POINT('Ctrl Pts',(158.38445823858,-227.756084040372,5.66003651379669));
#84309=CARTESIAN_POINT('Ctrl Pts',(156.808287801664,-225.137650512081,5.50127864856492));
#84310=CARTESIAN_POINT('Ctrl Pts',(158.153172243153,-222.393239240547,5.34252078333311));
#84311=CARTESIAN_POINT('Ctrl Pts',(161.188273375084,-222.034535313555,5.18376291810133));
#84312=CARTESIAN_POINT('Ctrl Pts',(163.135866760866,-224.389824550984,5.02500505286953));
#84313=CARTESIAN_POINT('Ctrl Pts',(162.213515010418,-227.303546335358,4.86624718763774));
#84314=CARTESIAN_POINT('Ctrl Pts',(159.265354409479,-228.109062604197,4.70748932240594));
#84315=CARTESIAN_POINT('Ctrl Pts',(156.989541424098,-226.069164899934,4.54873145717415));
#84316=CARTESIAN_POINT('Ctrl Pts',(157.468900008993,-223.050767521301,4.38997359194236));
#84317=CARTESIAN_POINT('Ctrl Pts',(160.264721206137,-221.816307630509,4.23121572671057));
#84318=CARTESIAN_POINT('Ctrl Pts',(162.818269565808,-223.495562871105,4.07245786147878));
#84319=CARTESIAN_POINT('Ctrl Pts',(162.792537729731,-226.551678912853,3.91369999624698));
#84320=CARTESIAN_POINT('Ctrl Pts',(160.211075473106,-228.187698474683,3.75494213101519));
#84321=CARTESIAN_POINT('Ctrl Pts',(157.436436952028,-226.906336517617,3.5961842657834));
#84322=CARTESIAN_POINT('Ctrl Pts',(157.007971231159,-223.880295455047,3.43742640055161));
#84323=CARTESIAN_POINT('Ctrl Pts',(159.317810122882,-221.879007947045,3.27866853531981));
#84324=CARTESIAN_POINT('Ctrl Pts',(162.251989161226,-222.734052245131,3.11991067008802));
#84325=CARTESIAN_POINT('Ctrl Pts',(163.125147812112,-225.662891835315,2.96115280485623));
#84326=CARTESIAN_POINT('Ctrl Pts',(161.138171299243,-227.985052852294,2.80239493962444));
#84327=CARTESIAN_POINT('Ctrl Pts',(158.109540476748,-227.575293598792,2.64363707439265));
#84328=CARTESIAN_POINT('Ctrl Pts',(156.81105809682,-224.808625781148,2.48487920916085));
#84329=CARTESIAN_POINT('Ctrl Pts',(158.431095301738,-222.217103565952,2.32612134392906));
#84330=CARTESIAN_POINT('Ctrl Pts',(161.486993857854,-222.17248821364,2.16736347869727));
#84331=CARTESIAN_POINT('Ctrl Pts',(163.181996040181,-224.715611213558,2.00860561346547));
#84332=CARTESIAN_POINT('Ctrl Pts',(161.964834852766,-227.519007490841,1.84984774823368));
#84333=CARTESIAN_POINT('Ctrl Pts',(158.949458377131,-228.017006818781,1.69108988300189));
#84334=CARTESIAN_POINT('Ctrl Pts',(156.895534457907,-225.753844514941,1.5323320177701));
#84335=CARTESIAN_POINT('Ctrl Pts',(157.682823704176,-222.800757743443,1.37357415253831));
#84336=CARTESIAN_POINT('Ctrl Pts',(160.590779276128,-221.860429843354,1.21481628730651));
#84337=CARTESIAN_POINT('Ctrl Pts',(162.958081336741,-223.793410603506,1.05605842207472));
#84338=CARTESIAN_POINT('Ctrl Pts',(162.618090079924,-226.830715517833,0.897300556842932));
#84339=CARTESIAN_POINT('Ctrl Pts',(159.882141982365,-228.192438466589,0.738542691611134));
#84340=CARTESIAN_POINT('Ctrl Pts',(157.253810399909,-226.632672586676,0.579784826379344));
#84341=CARTESIAN_POINT('Ctrl Pts',(157.139304244238,-223.578205904082,0.421026961147551));
#84342=CARTESIAN_POINT('Ctrl Pts',(159.641842265749,-221.825957697451,0.262269095915756));
#84343=CARTESIAN_POINT('Ctrl Pts',(162.474373249341,-222.976510294013,0.103511230683968));
#84344=CARTESIAN_POINT('Ctrl Pts',(163.037711807438,-225.983142742557,-0.055246634547828));
#84345=CARTESIAN_POINT('Ctrl Pts',(161.56627230492,-227.379023915733,-0.161085211369022));
#84346=CARTESIAN_POINT('Ctrl Pts',(160.698066426161,-227.611132185939,-0.21400449977962));
#84347=CARTESIAN_POINT('Ctrl Pts',(162.195197104019,-223.123136560921,20.2140044997796));
#84348=CARTESIAN_POINT('Ctrl Pts',(162.819257379562,-223.853043319762,20.161085211369));
#84349=CARTESIAN_POINT('Ctrl Pts',(163.270120329681,-225.972907574598,20.0552466345478));
#84350=CARTESIAN_POINT('Ctrl Pts',(160.95417666625,-228.279601159419,19.896488769316));
#84351=CARTESIAN_POINT('Ctrl Pts',(157.76341051174,-227.578308826282,19.7377309040842));
#84352=CARTESIAN_POINT('Ctrl Pts',(156.620253938806,-224.520518174272,19.5789730388525));
#84353=CARTESIAN_POINT('Ctrl Pts',(158.569904236459,-221.900030895413,19.4202151736206));
#84354=CARTESIAN_POINT('Ctrl Pts',(161.828539829886,-222.117367353854,19.2614573083889));
#84355=CARTESIAN_POINT('Ctrl Pts',(163.413617867613,-224.97253632475,19.1026994431571));
#84356=CARTESIAN_POINT('Ctrl Pts',(161.874590540856,-227.853010057811,18.9439415779253));
#84357=CARTESIAN_POINT('Ctrl Pts',(158.619919917364,-228.122327169995,18.7851837126935));
#84358=CARTESIAN_POINT('Ctrl Pts',(156.628307257382,-225.534130061043,18.6264258474617));
#84359=CARTESIAN_POINT('Ctrl Pts',(157.722463457629,-222.457078114412,18.4676679822299));
#84360=CARTESIAN_POINT('Ctrl Pts',(160.901023038434,-221.707317346696,18.3089101169981));
#84361=CARTESIAN_POINT('Ctrl Pts',(163.254965393284,-223.971015195058,18.1501522517663));
#84362=CARTESIAN_POINT('Ctrl Pts',(162.629964018838,-227.176442025878,17.9913943865345));
#84363=CARTESIAN_POINT('Ctrl Pts',(159.598019450966,-228.389988174002,17.8326365213027));
#84364=CARTESIAN_POINT('Ctrl Pts',(156.933967575063,-226.501017773124,17.6738786560709));
#84365=CARTESIAN_POINT('Ctrl Pts',(157.07594840122,-223.238315726986,17.5151207908392));
#84366=CARTESIAN_POINT('Ctrl Pts',(159.894021160979,-221.587907173084,17.3563629256074));
#84367=CARTESIAN_POINT('Ctrl Pts',(162.80908573781,-223.060245784851,17.1976050603756));
#84368=CARTESIAN_POINT('Ctrl Pts',(163.153275163757,-226.307847404716,17.0388471951438));
#84369=CARTESIAN_POINT('Ctrl Pts',(160.611587280992,-228.358507118361,16.880089329912));
#84370=CARTESIAN_POINT('Ctrl Pts',(157.510174744083,-227.335461255546,16.7213314646802));
#84371=CARTESIAN_POINT('Ctrl Pts',(156.687450182819,-224.175001340511,16.5625735994484));
#84372=CARTESIAN_POINT('Ctrl Pts',(158.896371084294,-221.769580167636,16.4038157342166));
#84373=CARTESIAN_POINT('Ctrl Pts',(162.115333125871,-222.320639097614,16.2450578689848));
#84374=CARTESIAN_POINT('Ctrl Pts',(163.398342373908,-225.323849020427,16.086300003753));
#84375=CARTESIAN_POINT('Ctrl Pts',(161.571188814945,-228.030672332319,15.9275421385212));
#84376=CARTESIAN_POINT('Ctrl Pts',(158.306083314347,-227.963824444928,15.7687842732894));
#84377=CARTESIAN_POINT('Ctrl Pts',(156.591250297839,-225.184484542052,15.6100264080576));
#84378=CARTESIAN_POINT('Ctrl Pts',(157.996104874706,-222.236304393562,15.4512685428259));
#84379=CARTESIAN_POINT('Ctrl Pts',(161.23492419144,-221.817458355396,15.2925106775941));
#84380=CARTESIAN_POINT('Ctrl Pts',(163.34354093673,-224.311274305225,15.1337528123623));
#84381=CARTESIAN_POINT('Ctrl Pts',(162.392149148207,-227.435411983827,14.9749949471305));
#84382=CARTESIAN_POINT('Ctrl Pts',(159.251462553313,-228.330660710601,14.8162370818987));
#84383=CARTESIAN_POINT('Ctrl Pts',(156.795837400192,-226.177688886008,14.6574792166669));
#84384=CARTESIAN_POINT('Ctrl Pts',(157.272661732414,-222.946896239252,14.4987213514351));
#84385=CARTESIAN_POINT('Ctrl Pts',(160.245545939881,-221.595104073596,14.3399634862033));
#84386=CARTESIAN_POINT('Ctrl Pts',(162.993706512824,-223.359472525891,14.1812056209715));
#84387=CARTESIAN_POINT('Ctrl Pts',(163.002027002956,-226.625251657978,14.0224477557397));
#84388=CARTESIAN_POINT('Ctrl Pts',(160.262892498034,-228.403600536596,13.8636898905079));
#84389=CARTESIAN_POINT('Ctrl Pts',(157.283158789249,-227.066974337964,13.7049320252761));
#84390=CARTESIAN_POINT('Ctrl Pts',(156.789878049707,-223.83865330651,13.5461741600443));
#84391=CARTESIAN_POINT('Ctrl Pts',(159.234500792838,-221.673196723269,13.3874162948126));
#84392=CARTESIAN_POINT('Ctrl Pts',(162.379708380261,-222.552430368069,13.2286584295807));
#84393=CARTESIAN_POINT('Ctrl Pts',(163.347006951649,-225.671679643764,13.069900564349));
#84394=CARTESIAN_POINT('Ctrl Pts',(161.251124892506,-228.176207735899,12.9111426991172));
#84395=CARTESIAN_POINT('Ctrl Pts',(158.010213380941,-227.773870633041,12.7523848338854));
#84396=CARTESIAN_POINT('Ctrl Pts',(156.590354504892,-224.832887235903,12.5936269686536));
#84397=CARTESIAN_POINT('Ctrl Pts',(158.291003051885,-222.044845433895,12.4348691034218));
#84398=CARTESIAN_POINT('Ctrl Pts',(161.555725538588,-221.961360974578,12.27611123819));
#84399=CARTESIAN_POINT('Ctrl Pts',(163.396648073553,-224.658838831835,12.1173533729582));
#84400=CARTESIAN_POINT('Ctrl Pts',(162.128958425172,-227.668547376781,11.9585955077264));
#84401=CARTESIAN_POINT('Ctrl Pts',(158.912846109793,-228.236001467435,11.7998376424946));
#84402=CARTESIAN_POINT('Ctrl Pts',(156.69169699198,-225.841867142345,11.6410797772628));
#84403=CARTESIAN_POINT('Ctrl Pts',(157.498306657011,-222.677256041687,11.482321912031));
#84404=CARTESIAN_POINT('Ctrl Pts',(160.594465971169,-221.638420120337,11.3235640467992));
#84405=CARTESIAN_POINT('Ctrl Pts',(163.14657005189,-223.676101972664,11.1648061815675));
#84406=CARTESIAN_POINT('Ctrl Pts',(162.818933344857,-226.925415247548,11.0060483163357));
#84407=CARTESIAN_POINT('Ctrl Pts',(159.911408951463,-228.412588563591,10.8472904511039));
#84408=CARTESIAN_POINT('Ctrl Pts',(157.084963082206,-226.776560960433,10.6885325858721));
#84409=CARTESIAN_POINT('Ctrl Pts',(156.926358885484,-223.514624836148,10.5297747206403));
#84410=CARTESIAN_POINT('Ctrl Pts',(159.580750915898,-221.612104003409,10.3710168554085));
#84411=CARTESIAN_POINT('Ctrl Pts',(162.618839691596,-222.810185453525,10.2122589901767));
#84412=CARTESIAN_POINT('Ctrl Pts',(163.260166484529,-226.012385090462,10.0535011249449));
#84413=CARTESIAN_POINT('Ctrl Pts',(160.917789039023,-228.288049932419,9.89474325971311));
#84414=CARTESIAN_POINT('Ctrl Pts',(157.735451101095,-227.554491605526,9.73598539448133));
#84415=CARTESIAN_POINT('Ctrl Pts',(156.625628226393,-224.483062661708,9.57722752924952));
#84416=CARTESIAN_POINT('Ctrl Pts',(158.604030266202,-221.884734749567,9.41846966401774));
#84417=CARTESIAN_POINT('Ctrl Pts',(161.860023751488,-222.137497472117,9.25971179878594));
#84418=CARTESIAN_POINT('Ctrl Pts',(163.413723572555,-225.010022395621,9.10095393355415));
#84419=CARTESIAN_POINT('Ctrl Pts',(161.843183714261,-227.873374823046,8.94219606832236));
#84420=CARTESIAN_POINT('Ctrl Pts',(158.585762193157,-228.107014725413,8.78343820309056));
#84421=CARTESIAN_POINT('Ctrl Pts',(156.622651057262,-225.497114873262,8.62468033785878));
#84422=CARTESIAN_POINT('Ctrl Pts',(157.750489540949,-222.43225550865,8.46592247262698));
#84423=CARTESIAN_POINT('Ctrl Pts',(160.937079908301,-221.717395801548,8.30716460739519));
#84424=CARTESIAN_POINT('Ctrl Pts',(163.266054780425,-224.006775327784,8.14840674216339));
#84425=CARTESIAN_POINT('Ctrl Pts',(162.605936445939,-227.205154034974,7.9896488769316));
#84426=CARTESIAN_POINT('Ctrl Pts',(159.560865178606,-228.385375856072,7.83089101169981));
#84427=CARTESIAN_POINT('Ctrl Pts',(156.917690082544,-226.467301826819,7.67213314646802));
#84428=CARTESIAN_POINT('Ctrl Pts',(157.095444901729,-223.206353223362,7.51337528123623));
#84429=CARTESIAN_POINT('Ctrl Pts',(159.931448432633,-221.58695007935,7.35461741600444));
#84430=CARTESIAN_POINT('Ctrl Pts',(162.830190355295,-223.091170088503,7.19585955077264));
#84431=CARTESIAN_POINT('Ctrl Pts',(163.138742176086,-226.342351157594,7.03710168554085));
#84432=CARTESIAN_POINT('Ctrl Pts',(160.574717280751,-228.365012500042,6.87834382030906));
#84433=CARTESIAN_POINT('Ctrl Pts',(157.484711152673,-227.308014534778,6.71958595507727));
#84434=CARTESIAN_POINT('Ctrl Pts',(156.696697278757,-224.138721758045,6.56082808984547));
#84435=CARTESIAN_POINT('Ctrl Pts',(158.931865925424,-221.757670794481,6.40207022461368));
#84436=CARTESIAN_POINT('Ctrl Pts',(162.144590835139,-222.343999392306,6.24331235938189));
#84437=CARTESIAN_POINT('Ctrl Pts',(163.394586296869,-225.361099641848,6.08455449415009));
#84438=CARTESIAN_POINT('Ctrl Pts',(161.537856513193,-228.047721513371,5.9257966289183));
#84439=CARTESIAN_POINT('Ctrl Pts',(158.273680509117,-227.945068775705,5.76703876368651));
#84440=CARTESIAN_POINT('Ctrl Pts',(156.589432035212,-225.147089210326,5.60828089845471));
#84441=CARTESIAN_POINT('Ctrl Pts',(158.026535228563,-222.214493605441,5.44952303322293));
#84442=CARTESIAN_POINT('Ctrl Pts',(161.269753303129,-221.831193343318,5.29076516799113));
#84443=CARTESIAN_POINT('Ctrl Pts',(163.350893204603,-224.347984808781,5.13200730275934));
#84444=CARTESIAN_POINT('Ctrl Pts',(162.365295776996,-227.461500551607,4.97324943752755));
#84445=CARTESIAN_POINT('Ctrl Pts',(159.214979747294,-228.322251086399,4.81449157229575));
#84446=CARTESIAN_POINT('Ctrl Pts',(156.783114222002,-226.142477557561,4.65573370706396));
#84447=CARTESIAN_POINT('Ctrl Pts',(157.295342434226,-222.917108612975,4.49697584183217));
#84448=CARTESIAN_POINT('Ctrl Pts',(160.282873144302,-221.598001783875,4.33821797660038));
#84449=CARTESIAN_POINT('Ctrl Pts',(163.011518363809,-223.392403588418,4.17946011136858));
#84450=CARTESIAN_POINT('Ctrl Pts',(162.984022095241,-226.658077565569,4.0207022461368));
#84451=CARTESIAN_POINT('Ctrl Pts',(160.225548922332,-228.406279020027,3.861944380905));
#84452=CARTESIAN_POINT('Ctrl Pts',(157.260653384824,-227.037054049071,3.70318651567321));
#84453=CARTESIAN_POINT('Ctrl Pts',(156.802807761284,-223.803517292995,3.54442865044142));
#84454=CARTESIAN_POINT('Ctrl Pts',(159.271032349968,-221.665001462314,3.38567078520962));
#84455=CARTESIAN_POINT('Ctrl Pts',(162.40640810106,-222.578676164264,3.22691291997783));
#84456=CARTESIAN_POINT('Ctrl Pts',(163.339439257329,-225.708346341134,3.06815505474604));
#84457=CARTESIAN_POINT('Ctrl Pts',(161.216215726989,-228.189737983437,2.90939718951425));
#84458=CARTESIAN_POINT('Ctrl Pts',(157.979911631102,-227.75188153009,2.75063932428245));
#84459=CARTESIAN_POINT('Ctrl Pts',(156.59239228956,-224.795503247303,2.59188145905066));
#84460=CARTESIAN_POINT('Ctrl Pts',(158.323515476587,-222.026280304273,2.43312359381887));
#84461=CARTESIAN_POINT('Ctrl Pts',(161.588957055112,-221.978605676399,2.27436572858708));
#84462=CARTESIAN_POINT('Ctrl Pts',(163.400185569483,-224.696110669036,2.11560786335528));
#84463=CARTESIAN_POINT('Ctrl Pts',(162.099563616179,-227.691735882641,1.95684999812349));
#84464=CARTESIAN_POINT('Ctrl Pts',(158.877422717969,-228.223883034018,1.7980921328917));
#84465=CARTESIAN_POINT('Ctrl Pts',(156.682661196342,-225.80553564774,1.63933426765991));
#84466=CARTESIAN_POINT('Ctrl Pts',(157.523934881276,-222.649955659871,1.48057640242812));
#84467=CARTESIAN_POINT('Ctrl Pts',(160.631289022385,-221.645149457697,1.32181853719632));
#84468=CARTESIAN_POINT('Ctrl Pts',(163.160917030547,-223.710674745524,1.16306067196453));
#84469=CARTESIAN_POINT('Ctrl Pts',(162.797612566751,-226.956247715886,1.00430280673274));
#84470=CARTESIAN_POINT('Ctrl Pts',(159.874060455843,-228.411344033269,0.845544941500945));
#84471=CARTESIAN_POINT('Ctrl Pts',(157.065504126535,-226.744624977154,0.686787076269154));
#84472=CARTESIAN_POINT('Ctrl Pts',(156.943146281581,-223.480713455746,0.528029211037361));
#84473=CARTESIAN_POINT('Ctrl Pts',(159.617283383065,-221.608313556091,0.369271345805566));
#84474=CARTESIAN_POINT('Ctrl Pts',(162.644041070348,-222.837759566193,0.210513480573778));
#84475=CARTESIAN_POINT('Ctrl Pts',(163.246007764142,-226.050556859208,0.0517556153419821));
#84476=CARTESIAN_POINT('Ctrl Pts',(161.673671626809,-227.542153631111,-0.0540829614792118));
#84477=CARTESIAN_POINT('Ctrl Pts',(160.745932854347,-227.790177569842,-0.10700224988981));
#84478=CARTESIAN_POINT('Ctrl Pts',(162.336062657696,-223.002698443069,20.3210067496694));
#84479=CARTESIAN_POINT('Ctrl Pts',(163.000168811616,-223.779443237332,20.2680874612588));
#84480=CARTESIAN_POINT('Ctrl Pts',(163.47996358703,-226.035338945303,20.1622488844376));
#84481=CARTESIAN_POINT('Ctrl Pts',(161.015406076653,-228.490052800557,20.0034910192058));
#84482=CARTESIAN_POINT('Ctrl Pts',(157.619888813377,-227.743758616508,19.844733153974));
#84483=CARTESIAN_POINT('Ctrl Pts',(156.403376010475,-224.489749878917,19.6859752887423));
#84484=CARTESIAN_POINT('Ctrl Pts',(158.478135150588,-221.701106223228,19.5272174235105));
#84485=CARTESIAN_POINT('Ctrl Pts',(161.945877027117,-221.932389138002,19.3684595582787));
#84486=CARTESIAN_POINT('Ctrl Pts',(163.63266934599,-224.970773983768,19.2097016930469));
#84487=CARTESIAN_POINT('Ctrl Pts',(161.994882807082,-228.036087395469,19.0509438278151));
#84488=CARTESIAN_POINT('Ctrl Pts',(158.531360332167,-228.322686556747,18.8921859625833));
#84489=CARTESIAN_POINT('Ctrl Pts',(156.411946109607,-225.568405127571,18.7334280973515));
#84490=CARTESIAN_POINT('Ctrl Pts',(157.576314191364,-222.293899100229,18.5746702321197));
#84491=CARTESIAN_POINT('Ctrl Pts',(160.95884158646,-221.496026267553,18.4159123668879));
#84492=CARTESIAN_POINT('Ctrl Pts',(163.463836160053,-223.904985354727,18.2571545016561));
#84493=CARTESIAN_POINT('Ctrl Pts',(162.798728517017,-227.31610406828,18.0983966364243));
#84494=CARTESIAN_POINT('Ctrl Pts',(159.572224403905,-228.607523337571,17.9396387711925));
#84495=CARTESIAN_POINT('Ctrl Pts',(156.737220615831,-226.597337916451,17.7808809059608));
#84496=CARTESIAN_POINT('Ctrl Pts',(156.88831233579,-223.125268643393,17.622123040729));
#84497=CARTESIAN_POINT('Ctrl Pts',(159.887220510682,-221.3689535564,17.4633651754972));
#84498=CARTESIAN_POINT('Ctrl Pts',(162.989344456746,-222.935771972903,17.3046073102654));
#84499=CARTESIAN_POINT('Ctrl Pts',(163.355620479822,-226.391771827016,17.1458494450336));
#84500=CARTESIAN_POINT('Ctrl Pts',(160.650832768699,-228.574022146095,16.9870915798018));
#84501=CARTESIAN_POINT('Ctrl Pts',(157.350402934712,-227.485327544205,16.82833371457));
#84502=CARTESIAN_POINT('Ctrl Pts',(156.474884229982,-224.122061268415,16.6695758493382));
#84503=CARTESIAN_POINT('Ctrl Pts',(158.825551339689,-221.562284486778,16.5108179841064));
#84504=CARTESIAN_POINT('Ctrl Pts',(162.251073816965,-222.14870480692,16.3520601188746));
#84505=CARTESIAN_POINT('Ctrl Pts',(163.616413625555,-225.344630375999,16.1933022536428));
#84506=CARTESIAN_POINT('Ctrl Pts',(161.672011826211,-228.225150238345,16.034544388411));
#84507=CARTESIAN_POINT('Ctrl Pts',(158.197384869287,-228.154012729466,15.8757865231792));
#84508=CARTESIAN_POINT('Ctrl Pts',(156.372511209097,-225.196322894569,15.7170286579475));
#84509=CARTESIAN_POINT('Ctrl Pts',(157.867515147698,-222.058958354301,15.5582707927157));
#84510=CARTESIAN_POINT('Ctrl Pts',(161.314169139266,-221.613235012514,15.3995129274839));
#84511=CARTESIAN_POINT('Ctrl Pts',(163.558095586257,-224.267078854098,15.2407550622521));
#84512=CARTESIAN_POINT('Ctrl Pts',(162.545653092624,-227.591692099587,15.0819971970203));
#84513=CARTESIAN_POINT('Ctrl Pts',(159.203428988727,-228.544388837452,14.9232393317885));
#84514=CARTESIAN_POINT('Ctrl Pts',(156.590226643023,-226.253261050659,14.7644814665567));
#84515=CARTESIAN_POINT('Ctrl Pts',(157.097648739538,-222.815148799587,14.6057236013249));
#84516=CARTESIAN_POINT('Ctrl Pts',(160.261302595496,-221.376612281216,14.4469657360931));
#84517=CARTESIAN_POINT('Ctrl Pts',(163.185812326331,-223.254200060589,14.2882078708613));
#84518=CARTESIAN_POINT('Ctrl Pts',(163.194666741387,-226.72954387586,14.1294500056295));
#84519=CARTESIAN_POINT('Ctrl Pts',(160.279762280353,-228.622009203956,13.9706921403977));
#84520=CARTESIAN_POINT('Ctrl Pts',(157.108819391341,-227.199611851024,13.8119342751659));
#84521=CARTESIAN_POINT('Ctrl Pts',(156.583884881681,-223.764129818532,13.6531764099342));
#84522=CARTESIAN_POINT('Ctrl Pts',(159.185378793971,-221.459716127521,13.4944185447024));
#84523=CARTESIAN_POINT('Ctrl Pts',(162.532414001985,-222.395370097384,13.3356606794706));
#84524=CARTESIAN_POINT('Ctrl Pts',(163.561784014967,-225.714781251697,13.1769028142388));
#84525=CARTESIAN_POINT('Ctrl Pts',(161.331409437515,-228.380024632565,13.018144949007));
#84526=CARTESIAN_POINT('Ctrl Pts',(157.882528995206,-227.951869602626,12.8593870837752));
#84527=CARTESIAN_POINT('Ctrl Pts',(156.371557933217,-224.822163628443,12.7006292185434));
#84528=CARTESIAN_POINT('Ctrl Pts',(158.181336908062,-221.855213494516,12.5418713533116));
#84529=CARTESIAN_POINT('Ctrl Pts',(161.655556273132,-221.766371846742,12.3831134880798));
#84530=CARTESIAN_POINT('Ctrl Pts',(163.614610602134,-224.63694655767,12.224355622848));
#84531=CARTESIAN_POINT('Ctrl Pts',(162.265573450205,-227.839787764742,12.0655977576162));
#84532=CARTESIAN_POINT('Ctrl Pts',(158.843083565739,-228.443655321194,11.9068398923844));
#84533=CARTESIAN_POINT('Ctrl Pts',(156.479403556414,-225.895889663108,11.7480820271526));
#84534=CARTESIAN_POINT('Ctrl Pts',(157.337773273815,-222.528205820575,11.5893241619208));
#84535=CARTESIAN_POINT('Ctrl Pts',(160.632612786331,-221.422707913851,11.4305662966891));
#84536=CARTESIAN_POINT('Ctrl Pts',(163.348485101673,-223.591147583697,11.2718084314573));
#84537=CARTESIAN_POINT('Ctrl Pts',(162.99982398364,-227.048968929542,11.1130505662255));
#84538=CARTESIAN_POINT('Ctrl Pts',(159.905724073745,-228.631573991643,10.9542927009937));
#84539=CARTESIAN_POINT('Ctrl Pts',(156.897905487851,-226.890562679401,10.7955348357619));
#84540=CARTESIAN_POINT('Ctrl Pts',(156.729123677489,-223.419308477316,10.6367769705301));
#84541=CARTESIAN_POINT('Ctrl Pts',(159.553847748865,-221.394703094632,10.4780191052983));
#84542=CARTESIAN_POINT('Ctrl Pts',(162.786890342936,-222.669665297966,10.3192612400665));
#84543=CARTESIAN_POINT('Ctrl Pts',(163.469371004743,-226.077349728964,10.1605033748347));
#84544=CARTESIAN_POINT('Ctrl Pts',(160.97668345944,-228.499043730379,10.0017455096029));
#84545=CARTESIAN_POINT('Ctrl Pts',(157.590135250464,-227.718413047349,9.84298764437114));
#84546=CARTESIAN_POINT('Ctrl Pts',(156.409095165498,-224.449890850283,9.68422977913933));
#84547=CARTESIAN_POINT('Ctrl Pts',(158.514451043859,-221.684828525406,9.52547191390756));
#84548=CARTESIAN_POINT('Ctrl Pts',(161.979381268463,-221.953811003712,9.36671404867575));
#84549=CARTESIAN_POINT('Ctrl Pts',(163.632781834006,-225.010665531631,9.20795618344396));
#84550=CARTESIAN_POINT('Ctrl Pts',(161.961460607923,-228.057758965422,9.04919831821217));
#84551=CARTESIAN_POINT('Ctrl Pts',(158.495010710601,-228.306391514302,8.89044045298037));
#84552=CARTESIAN_POINT('Ctrl Pts',(156.405926951755,-225.529014679313,8.73168258774859));
#84553=CARTESIAN_POINT('Ctrl Pts',(157.606138705329,-222.26748363062,8.5729247225168));
#84554=CARTESIAN_POINT('Ctrl Pts',(160.99721222165,-221.50675145573,8.41416685728499));
#84555=CARTESIAN_POINT('Ctrl Pts',(163.475637151931,-223.943040211187,8.25540899205321));
#84556=CARTESIAN_POINT('Ctrl Pts',(162.773159097441,-227.346658523802,8.09665112682141));
#84557=CARTESIAN_POINT('Ctrl Pts',(159.532685946025,-228.602615047713,7.93789326158963));
#84558=CARTESIAN_POINT('Ctrl Pts',(156.71989859843,-226.561458421627,7.77913539635782));
#84559=CARTESIAN_POINT('Ctrl Pts',(156.909059924565,-223.091255109471,7.62037753112604));
#84560=CARTESIAN_POINT('Ctrl Pts',(159.92704948619,-221.367935046067,7.46161966589424));
#84561=CARTESIAN_POINT('Ctrl Pts',(163.011803355185,-222.968680685676,7.30286180066245));
#84562=CARTESIAN_POINT('Ctrl Pts',(163.340154911951,-226.428489681874,7.14410393543066));
#84563=CARTESIAN_POINT('Ctrl Pts',(160.611596824648,-228.580944977395,6.98534607019887));
#84564=CARTESIAN_POINT('Ctrl Pts',(157.323305347477,-227.456119570422,6.82658820496707));
#84565=CARTESIAN_POINT('Ctrl Pts',(156.484724711037,-224.083453629183,6.66783033973528));
#84566=CARTESIAN_POINT('Ctrl Pts',(158.863323880821,-221.549610890473,6.50907247450349));
#84567=CARTESIAN_POINT('Ctrl Pts',(162.282208990179,-222.17356412912,6.3503146092717));
#84568=CARTESIAN_POINT('Ctrl Pts',(163.61241652147,-225.384271365649,6.19155674403991));
#84569=CARTESIAN_POINT('Ctrl Pts',(161.636540594368,-228.243293463447,6.03279887880811));
#84570=CARTESIAN_POINT('Ctrl Pts',(158.162902779655,-228.134053511038,5.87404101357632));
#84571=CARTESIAN_POINT('Ctrl Pts',(156.37057626876,-225.156527908571,5.71528314834453));
#84572=CARTESIAN_POINT('Ctrl Pts',(157.899898213972,-222.035747970335,5.55652528311273));
#84573=CARTESIAN_POINT('Ctrl Pts',(161.351233231173,-221.627851373082,5.39776741788094));
#84574=CARTESIAN_POINT('Ctrl Pts',(163.56591964834,-224.306145066578,5.23900955264915));
#84575=CARTESIAN_POINT('Ctrl Pts',(162.517076543573,-227.619454767856,5.08025168741736));
#84576=CARTESIAN_POINT('Ctrl Pts',(159.164605085109,-228.535439568601,4.92149382218557));
#84577=CARTESIAN_POINT('Ctrl Pts',(156.576687019905,-226.215790215187,4.76273595695377));
#84578=CARTESIAN_POINT('Ctrl Pts',(157.121784859459,-222.78344970465,4.60397809172198));
#84579=CARTESIAN_POINT('Ctrl Pts',(160.301025082467,-221.37969593724,4.44522022649019));
#84580=CARTESIAN_POINT('Ctrl Pts',(163.20476716181,-223.289244305731,4.2864623612584));
#84581=CARTESIAN_POINT('Ctrl Pts',(163.17550646075,-226.764476218285,4.1277044960266));
#84582=CARTESIAN_POINT('Ctrl Pts',(160.240022371557,-228.624859565371,3.96894663079482));
#84583=CARTESIAN_POINT('Ctrl Pts',(157.08486981762,-227.167771580525,3.81018876556302));
#84584=CARTESIAN_POINT('Ctrl Pts',(156.59764429141,-223.726739130944,3.65143090033123));
#84585=CARTESIAN_POINT('Ctrl Pts',(159.224254577053,-221.450994977583,3.49267303509943));
#84586=CARTESIAN_POINT('Ctrl Pts',(162.560827040894,-222.423300083398,3.33391516986764));
#84587=CARTESIAN_POINT('Ctrl Pts',(163.553730702545,-225.753800846953,3.17515730463585));
#84588=CARTESIAN_POINT('Ctrl Pts',(161.294260154735,-228.39442311458,3.01639943940406));
#84589=CARTESIAN_POINT('Ctrl Pts',(157.850282785455,-227.928469461388,2.85764157417226));
#84590=CARTESIAN_POINT('Ctrl Pts',(156.3737264823,-224.782380713458,2.69888370894047));
#84591=CARTESIAN_POINT('Ctrl Pts',(158.215935651436,-221.835457042593,2.54012584370868));
#84592=CARTESIAN_POINT('Ctrl Pts',(161.69092025237,-221.784723139159,2.38136797847689));
#84593=CARTESIAN_POINT('Ctrl Pts',(163.618375098784,-224.676610124513,2.22261011324509));
#84594=CARTESIAN_POINT('Ctrl Pts',(162.234292379592,-227.864464274441,2.0638522480133));
#84595=CARTESIAN_POINT('Ctrl Pts',(158.805387058807,-228.430759249254,1.90509438278151));
#84596=CARTESIAN_POINT('Ctrl Pts',(156.469787934776,-225.85722678054,1.74633651754972));
#84597=CARTESIAN_POINT('Ctrl Pts',(157.365046058377,-222.499153576299,1.58757865231793));
#84598=CARTESIAN_POINT('Ctrl Pts',(160.671798768642,-221.429869072041,1.42882078708613));
#84599=CARTESIAN_POINT('Ctrl Pts',(163.363752724354,-223.627938887541,1.27006292185434));
#84600=CARTESIAN_POINT('Ctrl Pts',(162.977135053578,-227.081779913939,1.11130505662255));
#84601=CARTESIAN_POINT('Ctrl Pts',(159.865978929321,-228.630249599949,0.952547191390754));
#84602=CARTESIAN_POINT('Ctrl Pts',(156.877197853162,-226.856577367632,0.793789326158964));
#84603=CARTESIAN_POINT('Ctrl Pts',(156.746988318924,-223.38322100741,0.635031460927171));
#84604=CARTESIAN_POINT('Ctrl Pts',(159.592724500381,-221.390669414731,0.476273595695376));
#84605=CARTESIAN_POINT('Ctrl Pts',(162.813708891355,-222.699008838373,0.317515730463588));
#84606=CARTESIAN_POINT('Ctrl Pts',(163.454303720846,-226.117970975858,0.158757865231792));
#84607=CARTESIAN_POINT('Ctrl Pts',(161.781070948697,-227.70528334649,0.0529192884105984));
#84608=CARTESIAN_POINT('Ctrl Pts',(160.793799282533,-227.969222953746,0.));
#84609=CARTESIAN_POINT('Ctrl Pts',(160.793799282533,-227.969222953746,0.));
#84610=CARTESIAN_POINT('Ctrl Pts',(160.886835131854,-227.935190024475,-3.02457214913811E-16));
#84611=CARTESIAN_POINT('Ctrl Pts',(160.977803977775,-227.896385137717,-1.37333377546448E-15));
#84612=CARTESIAN_POINT('Ctrl Pts',(161.066498279727,-227.853137686896,-6.66133814775094E-16));
#84613=CARTESIAN_POINT('Ctrl Pts',(161.157170911953,-227.808925599797,5.68402718963673E-17));
#84614=CARTESIAN_POINT('Ctrl Pts',(161.245467067815,-227.7600699377,-1.69277578169131E-15));
#84615=CARTESIAN_POINT('Ctrl Pts',(161.331136079803,-227.706877059437,-1.27675647831893E-15));
#84616=CARTESIAN_POINT('Ctrl Pts',(161.414071319396,-227.655381612005,-8.7401271135087E-16));
#84617=CARTESIAN_POINT('Ctrl Pts',(161.494544733236,-227.599820476436,1.75893653509998E-15));
#84618=CARTESIAN_POINT('Ctrl Pts',(161.572295205067,-227.540440925299,1.88737914186277E-15));
#84619=CARTESIAN_POINT('Ctrl Pts',(161.640326867919,-227.488483818054,1.9997664227802E-15));
#84620=CARTESIAN_POINT('Ctrl Pts',(161.70627348163,-227.433602519189,4.82523262324037E-15));
#84621=CARTESIAN_POINT('Ctrl Pts',(161.769934874098,-227.375949718044,5.32907051820075E-15));
#84622=CARTESIAN_POINT('Ctrl Pts',(161.783313679488,-227.363833652454,5.43495493077293E-15));
#84623=CARTESIAN_POINT('Ctrl Pts',(161.79659337319,-227.351593235715,6.17321314109589E-15));
#84624=CARTESIAN_POINT('Ctrl Pts',(161.809754802739,-227.339246301387,6.0507154842071E-15));
#84625=CARTESIAN_POINT('Ctrl Pts',(161.882179710651,-227.271303409741,5.37663357792855E-15));
#84626=CARTESIAN_POINT('Ctrl Pts',(161.951138858742,-227.200038396299,1.6501302217819E-15));
#84627=CARTESIAN_POINT('Ctrl Pts',(162.016393029598,-227.125743280976,1.83186799063151E-15));
#84628=CARTESIAN_POINT('Ctrl Pts',(162.081289564234,-227.051855352256,2.01260971573651E-15));
#84629=CARTESIAN_POINT('Ctrl Pts',(162.142522107232,-226.974969645043,4.08055444834208E-16));
#84630=CARTESIAN_POINT('Ctrl Pts',(162.199811733062,-226.895346657282,-8.60422844084496E-16));
#84631=CARTESIAN_POINT('Ctrl Pts',(162.255642444754,-226.817751315904,-2.09659858463182E-15));
#84632=CARTESIAN_POINT('Ctrl Pts',(162.307728765594,-226.737555590414,-1.2543397869325E-15));
#84633=CARTESIAN_POINT('Ctrl Pts',(162.355765747154,-226.65498650143,-1.36002320516582E-15));
#84634=CARTESIAN_POINT('Ctrl Pts',(162.376479635949,-226.619382121811,-1.40559464828665E-15));
#84635=CARTESIAN_POINT('Ctrl Pts',(162.396439968897,-226.583336323596,-1.93777603934293E-15));
#84636=CARTESIAN_POINT('Ctrl Pts',(162.415619320772,-226.546866979337,-2.02615701994091E-15));
#84637=CARTESIAN_POINT('Ctrl Pts',(162.428829664771,-226.521747643385,-2.08703202574327E-15));
#84638=CARTESIAN_POINT('Ctrl Pts',(162.441669459883,-226.496427366951,-3.53414151482419E-15));
#84639=CARTESIAN_POINT('Ctrl Pts',(162.454129213649,-226.470911987081,-3.1641356201817E-15));
#84640=CARTESIAN_POINT('Ctrl Pts',(162.460341854643,-226.45818959321,-2.97964451127121E-15));
#84641=CARTESIAN_POINT('Ctrl Pts',(162.466459455713,-226.445419669975,-1.69354284525896E-15));
#84642=CARTESIAN_POINT('Ctrl Pts',(162.472475650985,-226.432614465927,-1.63757896132211E-15));
#84643=CARTESIAN_POINT('Ctrl Pts',(162.512676180897,-226.347049426042,-1.26362537626533E-15));
#84644=CARTESIAN_POINT('Ctrl Pts',(162.548420108931,-226.259774184938,-2.83979563700065E-18));
#84645=CARTESIAN_POINT('Ctrl Pts',(162.579456396658,-226.171026817168,-7.7715611723761E-16));
#84646=CARTESIAN_POINT('Ctrl Pts',(162.609806651508,-226.084241140585,-1.53435678186565E-15));
#84647=CARTESIAN_POINT('Ctrl Pts',(162.635655300542,-225.996047022835,-1.68477216875799E-15));
#84648=CARTESIAN_POINT('Ctrl Pts',(162.656718450553,-225.906658343455,-1.9151347174784E-15));
#84649=CARTESIAN_POINT('Ctrl Pts',(162.660341355547,-225.891283307301,-1.95475754824121E-15));
#84650=CARTESIAN_POINT('Ctrl Pts',(162.66382255848,-225.875872922801,-1.31552826697175E-15));
#84651=CARTESIAN_POINT('Ctrl Pts',(162.667160456718,-225.860428273356,-1.30451205393456E-15));
#84652=CARTESIAN_POINT('Ctrl Pts',(162.687288048911,-225.767296732645,-1.2092570774105E-15));
#84653=CARTESIAN_POINT('Ctrl Pts',(162.70220900913,-225.672918237907,3.95464250160003E-15));
#84654=CARTESIAN_POINT('Ctrl Pts',(162.71200163869,-225.577700926241,5.27355936696949E-15));
#84655=CARTESIAN_POINT('Ctrl Pts',(162.71526433647,-225.545976524792,5.71299466904966E-15));
#84656=CARTESIAN_POINT('Ctrl Pts',(162.717957335588,-225.514159127666,1.08684253548423E-14));
#84657=CARTESIAN_POINT('Ctrl Pts',(162.720082333063,-225.482264288845,1.15463194561016E-14));
#84658=CARTESIAN_POINT('Ctrl Pts',(162.721307135479,-225.463880796112,1.19370429005596E-14));
#84659=CARTESIAN_POINT('Ctrl Pts',(162.722343230258,-225.445471581581,4.25907006365195E-15));
#84660=CARTESIAN_POINT('Ctrl Pts',(162.723190856866,-225.427039671918,4.35762537165374E-15));
#84661=CARTESIAN_POINT('Ctrl Pts',(162.723765383164,-225.414546415178,4.42442673887179E-15));
#84662=CARTESIAN_POINT('Ctrl Pts',(162.724253204013,-225.40204435614,3.39829207989485E-15));
#84663=CARTESIAN_POINT('Ctrl Pts',(162.724654274891,-225.389543824009,3.19189119579733E-15));
#84664=CARTESIAN_POINT('Ctrl Pts',(162.727643921145,-225.296362864977,1.65334610634577E-15));
#84665=CARTESIAN_POINT('Ctrl Pts',(162.725824895213,-225.203120691748,6.39634240367912E-16));
#84666=CARTESIAN_POINT('Ctrl Pts',(162.719335998398,-225.110191721826,2.4980018054066E-16));
#84667=CARTESIAN_POINT('Ctrl Pts',(162.712834250128,-225.017078703282,-1.40805957372921E-16));
#84668=CARTESIAN_POINT('Ctrl Pts',(162.701643731984,-224.924279149824,1.77023230634299E-15));
#84669=CARTESIAN_POINT('Ctrl Pts',(162.685853037124,-224.8321817391,1.60982338570648E-15));
#84670=CARTESIAN_POINT('Ctrl Pts',(162.670284969111,-224.741382773839,1.45167600786084E-15));
#84671=CARTESIAN_POINT('Ctrl Pts',(162.650245055058,-224.651265446538,2.60240118438736E-15));
#84672=CARTESIAN_POINT('Ctrl Pts',(162.625775144772,-224.562227386308,4.16333634234434E-15));
#84673=CARTESIAN_POINT('Ctrl Pts',(162.616258304647,-224.527598694405,4.77041541085431E-15));
#84674=CARTESIAN_POINT('Ctrl Pts',(162.606070959923,-224.493133590178,6.71445756624556E-15));
#84675=CARTESIAN_POINT('Ctrl Pts',(162.595214003931,-224.45885692894,6.66133814775094E-15));
#84676=CARTESIAN_POINT('Ctrl Pts',(162.589230527729,-224.439966405027,6.63206301974616E-15));
#84677=CARTESIAN_POINT('Ctrl Pts',(162.583043654131,-224.421133133431,-2.06375398258952E-15));
#84678=CARTESIAN_POINT('Ctrl Pts',(162.576653426697,-224.402361401392,-1.97064586870965E-15));
#84679=CARTESIAN_POINT('Ctrl Pts',(162.57141710462,-224.386979345604,-1.8943506073516E-15));
#84680=CARTESIAN_POINT('Ctrl Pts',(162.566043962058,-224.371638089573,6.8029554114436E-15));
#84681=CARTESIAN_POINT('Ctrl Pts',(162.560539518476,-224.356354677768,6.38378239159465E-15));
#84682=CARTESIAN_POINT('Ctrl Pts',(162.528144500718,-224.266408002972,3.91684504924636E-15));
#84683=CARTESIAN_POINT('Ctrl Pts',(162.491164517742,-224.178337626994,4.67507282145047E-15));
#84684=CARTESIAN_POINT('Ctrl Pts',(162.449672187927,-224.092586398355,7.09848846369709E-15));
#84685=CARTESIAN_POINT('Ctrl Pts',(162.418552940565,-224.028272976875,8.91605019538206E-15));
#84686=CARTESIAN_POINT('Ctrl Pts',(162.384894352882,-223.965264611358,4.96167796900426E-15));
#84687=CARTESIAN_POINT('Ctrl Pts',(162.348709733279,-223.903765223849,5.12090370108353E-15));
#84688=CARTESIAN_POINT('Ctrl Pts',(162.334283097957,-223.879245711253,5.18438624133952E-15));
#84689=CARTESIAN_POINT('Ctrl Pts',(162.319454775845,-223.854966251689,1.42974040300608E-15));
#84690=CARTESIAN_POINT('Ctrl Pts',(162.304225021793,-223.830940576599,6.80011602582908E-16));
#84691=CARTESIAN_POINT('Ctrl Pts',(162.293795413291,-223.814487363743,1.66583884431403E-16));
#84692=CARTESIAN_POINT('Ctrl Pts',(162.28318192805,-223.798160209656,4.27605544559612E-15));
#84693=CARTESIAN_POINT('Ctrl Pts',(162.272389031914,-223.781969041488,4.02455846426619E-15));
#84694=CARTESIAN_POINT('Ctrl Pts',(162.224799336923,-223.710576456493,2.91561935445547E-15));
#84695=CARTESIAN_POINT('Ctrl Pts',(162.173700478564,-223.641787621303,5.11345936751299E-15));
#84696=CARTESIAN_POINT('Ctrl Pts',(162.119126329557,-223.575955009348,4.88151186139874E-15));
#84697=CARTESIAN_POINT('Ctrl Pts',(162.068157476713,-223.514471453999,4.66488735104534E-15));
#84698=CARTESIAN_POINT('Ctrl Pts',(162.014156816139,-223.45556630499,3.49062128769292E-15));
#84699=CARTESIAN_POINT('Ctrl Pts',(161.957129225973,-223.39956097681,4.09394740330526E-15));
#84700=CARTESIAN_POINT('Ctrl Pts',(161.943965194155,-223.386632920057,4.23408426879927E-15));
#84701=CARTESIAN_POINT('Ctrl Pts',(161.930639785301,-223.373859540263,5.90640714698764E-16));
#84702=CARTESIAN_POINT('Ctrl Pts',(161.9171563836,-223.361242235853,7.21644966006352E-16));
#84703=CARTESIAN_POINT('Ctrl Pts',(157.480508436316,-225.001988388677,18.387416697508));
#84704=CARTESIAN_POINT('Ctrl Pts',(157.479370520287,-225.133541934848,18.3957515808994));
#84705=CARTESIAN_POINT('Ctrl Pts',(157.488784872591,-225.264932202126,18.4040864642907));
#84706=CARTESIAN_POINT('Ctrl Pts',(157.509319881608,-225.394560708534,18.4124213476821));
#84707=CARTESIAN_POINT('Ctrl Pts',(157.639699397875,-226.217589417486,18.4653406360927));
#84708=CARTESIAN_POINT('Ctrl Pts',(158.218369242817,-226.969598906988,18.5182599245033));
#84709=CARTESIAN_POINT('Ctrl Pts',(158.980531985396,-227.306478149406,18.5711792129139));
#84710=CARTESIAN_POINT('Ctrl Pts',(159.742694727975,-227.643357391824,18.6240985013245));
#84711=CARTESIAN_POINT('Ctrl Pts',(160.688350368189,-227.565106387159,18.6770177897351));
#84712=CARTESIAN_POINT('Ctrl Pts',(161.384763005373,-227.10751515553,18.7299370781457));
#84713=CARTESIAN_POINT('Ctrl Pts',(162.081175642556,-226.6499239239,18.7828563665563));
#84714=CARTESIAN_POINT('Ctrl Pts',(162.528345276708,-225.812992465307,18.8357756549668));
#84715=CARTESIAN_POINT('Ctrl Pts',(162.521655181211,-224.979737199152,18.8886949433774));
#84716=CARTESIAN_POINT('Ctrl Pts',(162.514965085714,-224.146481932996,18.941614231788));
#84717=CARTESIAN_POINT('Ctrl Pts',(162.054415260568,-223.316902859278,18.9945335201987));
#84718=CARTESIAN_POINT('Ctrl Pts',(161.350736510125,-222.870539398123,19.0474528086093));
#84719=CARTESIAN_POINT('Ctrl Pts',(160.647057759681,-222.424175936968,19.1003720970199));
#84720=CARTESIAN_POINT('Ctrl Pts',(159.700250083941,-222.361028088376,19.1532913854304));
#84721=CARTESIAN_POINT('Ctrl Pts',(158.943607477282,-222.71014991828,19.206210673841));
#84722=CARTESIAN_POINT('Ctrl Pts',(158.186964870623,-223.059271748183,19.2591299622516));
#84723=CARTESIAN_POINT('Ctrl Pts',(157.620487333045,-223.820663256583,19.3120492506622));
#84724=CARTESIAN_POINT('Ctrl Pts',(157.50332258309,-224.64558475759,19.3649685390728));
#84725=CARTESIAN_POINT('Ctrl Pts',(157.486755637785,-224.762227599343,19.3724512585512));
#84726=CARTESIAN_POINT('Ctrl Pts',(157.479172071341,-224.880140634173,19.3799339780296));
#84727=CARTESIAN_POINT('Ctrl Pts',(157.48014261364,-224.998176427436,19.387416697508));
#84728=CARTESIAN_POINT('Ctrl Pts',(159.206200717467,-227.969222953746,20.));
#84729=CARTESIAN_POINT('Ctrl Pts',(158.218929051303,-227.70528334649,19.9470807115894));
#84730=CARTESIAN_POINT('Ctrl Pts',(156.545695841364,-226.117974132338,19.8412421347682));
#84731=CARTESIAN_POINT('Ctrl Pts',(157.186291485908,-222.699008209422,19.6824842695364));
#84732=CARTESIAN_POINT('Ctrl Pts',(160.407275465985,-221.390670340075,19.5237264043046));
#84733=CARTESIAN_POINT('Ctrl Pts',(163.253011317767,-223.383220872305,19.3649685390728));
#84734=CARTESIAN_POINT('Ctrl Pts',(163.122801873322,-226.856577342785,19.2062106738411));
#84735=CARTESIAN_POINT('Ctrl Pts',(160.134021031603,-228.6302491553,19.0474528086092));
#84736=CARTESIAN_POINT('Ctrl Pts',(157.022865258248,-227.081779751736,18.8886949433775));
#84737=CARTESIAN_POINT('Ctrl Pts',(156.636247599646,-223.627939000525,18.7299370781456));
#84738=CARTESIAN_POINT('Ctrl Pts',(159.328201303672,-221.429869438357,18.5711792129139));
#84739=CARTESIAN_POINT('Ctrl Pts',(162.634953676974,-222.499153818262,18.4124213476821));
#84740=CARTESIAN_POINT('Ctrl Pts',(163.530211716637,-225.857226698665,18.2536634824503));
#84741=CARTESIAN_POINT('Ctrl Pts',(161.194612821702,-228.430758907163,18.0949056172185));
#84742=CARTESIAN_POINT('Ctrl Pts',(157.765707842634,-227.864463991016,17.9361477519867));
#84743=CARTESIAN_POINT('Ctrl Pts',(156.381625260024,-224.676610156181,17.7773898867549));
#84744=CARTESIAN_POINT('Ctrl Pts',(158.309079915571,-221.784723458447,17.6186320215231));
#84745=CARTESIAN_POINT('Ctrl Pts',(161.784064171446,-221.835457356522,17.4598741562913));
#84746=CARTESIAN_POINT('Ctrl Pts',(163.626273157879,-224.782380735109,17.3011162910595));
#84747=CARTESIAN_POINT('Ctrl Pts',(162.149717001196,-227.928469170749,17.1423584258277));
#84748=CARTESIAN_POINT('Ctrl Pts',(158.705739973713,-228.394422777744,16.983600560596));
#84749=CARTESIAN_POINT('Ctrl Pts',(156.44626965011,-225.753800772142,16.8248426953641));
#84750=CARTESIAN_POINT('Ctrl Pts',(157.439173213236,-222.423300339104,16.6660848301324));
#84751=CARTESIAN_POINT('Ctrl Pts',(160.775745345963,-221.450995329772,16.5073269649006));
#84752=CARTESIAN_POINT('Ctrl Pts',(163.402355370953,-223.726739257298,16.3485690996688));
#84753=CARTESIAN_POINT('Ctrl Pts',(162.915129893092,-227.167771365402,16.189811234437));
#84754=CARTESIAN_POINT('Ctrl Pts',(159.759977652262,-228.624859205653,16.0310533692052));
#84755=CARTESIAN_POINT('Ctrl Pts',(156.824493854376,-226.764476043185,15.8722955039734));
#84756=CARTESIAN_POINT('Ctrl Pts',(156.79523315622,-223.2892444755,15.7135376387416));
#84757=CARTESIAN_POINT('Ctrl Pts',(159.698974947405,-221.379696296506,15.5547797735098));
#84758=CARTESIAN_POINT('Ctrl Pts',(162.878214854917,-222.783449924613,15.396021908278));
#84759=CARTESIAN_POINT('Ctrl Pts',(163.423312640378,-226.215790094536,15.2372640430462));
#84760=CARTESIAN_POINT('Ctrl Pts',(160.83539483199,-228.535439217757,15.0785061778144));
#84761=CARTESIAN_POINT('Ctrl Pts',(157.482923706213,-227.619454507911,14.9197483125826));
#84762=CARTESIAN_POINT('Ctrl Pts',(156.43408070553,-224.306145135434,14.7609904473509));
#84763=CARTESIAN_POINT('Ctrl Pts',(158.648766902918,-221.627851707722,14.6022325821191));
#84764=CARTESIAN_POINT('Ctrl Pts',(162.100101577621,-222.035748264497,14.4434747168873));
#84765=CARTESIAN_POINT('Ctrl Pts',(163.629423371069,-225.156527893037,14.2847168516555));
#84766=CARTESIAN_POINT('Ctrl Pts',(161.837097038039,-228.134053200026,14.1259589864237));
#84767=CARTESIAN_POINT('Ctrl Pts',(158.363459568037,-228.243293141594,13.9672011211919));
#84768=CARTESIAN_POINT('Ctrl Pts',(156.387583837013,-225.384271327515,13.8084432559601));
#84769=CARTESIAN_POINT('Ctrl Pts',(157.7177912363,-222.173564409605,13.6496853907283));
#84770=CARTESIAN_POINT('Ctrl Pts',(161.136676006379,-221.549611232878,13.4909275254965));
#84771=CARTESIAN_POINT('Ctrl Pts',(163.515274940119,-224.083453720138,13.3321696602647));
#84772=CARTESIAN_POINT('Ctrl Pts',(162.676694386897,-227.456119326685,13.1734117950329));
#84773=CARTESIAN_POINT('Ctrl Pts',(159.388403236045,-228.580944622035,13.0146539298011));
#84774=CARTESIAN_POINT('Ctrl Pts',(156.659845419514,-226.428489540116,12.8558960645693));
#84775=CARTESIAN_POINT('Ctrl Pts',(156.988196943696,-222.968680887257,12.6971381993375));
#84776=CARTESIAN_POINT('Ctrl Pts',(160.072950506571,-221.367935406501,12.5383803341058));
#84777=CARTESIAN_POINT('Ctrl Pts',(163.090939768701,-223.091255298888,12.379622468874));
#84778=CARTESIAN_POINT('Ctrl Pts',(163.280101076064,-226.561458266673,12.2208646036422));
#84779=CARTESIAN_POINT('Ctrl Pts',(160.467314007601,-228.602614690202,12.0621067384104));
#84780=CARTESIAN_POINT('Ctrl Pts',(157.226841177757,-227.346658290928,11.9033488731786));
#84781=CARTESIAN_POINT('Ctrl Pts',(156.524363192979,-223.943040316076,11.7445910079468));
#84782=CARTESIAN_POINT('Ctrl Pts',(159.00278787731,-221.506751802388,11.585833142715));
#84783=CARTESIAN_POINT('Ctrl Pts',(162.393861057113,-222.267483901785,11.4270752774832));
#84784=CARTESIAN_POINT('Ctrl Pts',(163.594072691582,-225.529014626816,11.2683174122514));
#84785=CARTESIAN_POINT('Ctrl Pts',(161.504989140049,-228.306391186187,11.1095595470196));
#84786=CARTESIAN_POINT('Ctrl Pts',(158.038539586726,-228.057758661981,10.9508016817878));
#84787=CARTESIAN_POINT('Ctrl Pts',(156.367218526498,-225.010665530573,10.792043816556));
#84788=CARTESIAN_POINT('Ctrl Pts',(158.020618927964,-221.953811306005,10.6332859513243));
#84789=CARTESIAN_POINT('Ctrl Pts',(161.48554880872,-221.684828854392,10.4745280860924));
#84790=CARTESIAN_POINT('Ctrl Pts',(163.590904478153,-224.449890904874,10.3157702208607));
#84791=CARTESIAN_POINT('Ctrl Pts',(162.40986451039,-227.718412777583,10.1570123556289));
#84792=CARTESIAN_POINT('Ctrl Pts',(159.023316637483,-228.499043383147,9.99825449039708));
#84793=CARTESIAN_POINT('Ctrl Pts',(156.530629339545,-226.077349622051,9.83949662516528));
#84794=CARTESIAN_POINT('Ctrl Pts',(157.213109933626,-222.66966552922,9.6807387599335));
#84795=CARTESIAN_POINT('Ctrl Pts',(160.44615220686,-221.394703452409,9.52198089470169));
#84796=CARTESIAN_POINT('Ctrl Pts',(163.270875997921,-223.419308634178,9.36322302946991));
#84797=CARTESIAN_POINT('Ctrl Pts',(163.102094204308,-226.890562491788,9.20446516423811));
#84798=CARTESIAN_POINT('Ctrl Pts',(160.0942759169,-228.631573631259,9.04570729900633));
#84799=CARTESIAN_POINT('Ctrl Pts',(157.000176314052,-227.048968726209,8.88694943377452));
#84800=CARTESIAN_POINT('Ctrl Pts',(156.651515230618,-223.591147723507,8.72819156854274));
#84801=CARTESIAN_POINT('Ctrl Pts',(159.367387276447,-221.422708268849,8.56943370331094));
#84802=CARTESIAN_POINT('Ctrl Pts',(162.662226461995,-222.528206065867,8.41067583807915));
#84803=CARTESIAN_POINT('Ctrl Pts',(163.520596094214,-225.895889574202,8.25191797284736));
#84804=CARTESIAN_POINT('Ctrl Pts',(161.156916319453,-228.443654979458,8.09316010761556));
#84805=CARTESIAN_POINT('Ctrl Pts',(157.734426774623,-227.839787482932,7.93440224238378));
#84806=CARTESIAN_POINT('Ctrl Pts',(156.385389756567,-224.636946593699,7.77564437715197));
#84807=CARTESIAN_POINT('Ctrl Pts',(158.344443891159,-221.766372167636,7.6168865119202));
#84808=CARTESIAN_POINT('Ctrl Pts',(161.81866291146,-221.855213806593,7.45812864668839));
#84809=CARTESIAN_POINT('Ctrl Pts',(163.628441706709,-224.822163646091,7.29937078145661));
#84810=CARTESIAN_POINT('Ctrl Pts',(162.117470794664,-227.951869309693,7.14061291622481));
#84811=CARTESIAN_POINT('Ctrl Pts',(158.668590694609,-228.380024297143,6.98185505099302));
#84812=CARTESIAN_POINT('Ctrl Pts',(156.438216338492,-225.714781180764,6.82309718576122));
#84813=CARTESIAN_POINT('Ctrl Pts',(157.467586249323,-222.395370355858,6.66433932052943));
#84814=CARTESIAN_POINT('Ctrl Pts',(160.814621125189,-221.459716478846,6.50558145529765));
#84815=CARTESIAN_POINT('Ctrl Pts',(163.416114779316,-223.764129941176,6.34682359006585));
#84816=CARTESIAN_POINT('Ctrl Pts',(162.891180321749,-227.199611632742,6.18806572483406));
#84817=CARTESIAN_POINT('Ctrl Pts',(159.72023774741,-228.622008844521,6.02930785960227));
#84818=CARTESIAN_POINT('Ctrl Pts',(156.80533357564,-226.729543704226,5.87054999437047));
#84819=CARTESIAN_POINT('Ctrl Pts',(156.814187989818,-223.254200233836,5.71179212913868));
#84820=CARTESIAN_POINT('Ctrl Pts',(159.738697430435,-221.376612640788,5.55303426390689));
#84821=CARTESIAN_POINT('Ctrl Pts',(162.902350972443,-222.815149016404,5.39427639867509));
#84822=CARTESIAN_POINT('Ctrl Pts',(163.409773018603,-226.25326092629,5.23551853344331));
#84823=CARTESIAN_POINT('Ctrl Pts',(160.796570932224,-228.544388485719,5.07676066821151));
#84824=CARTESIAN_POINT('Ctrl Pts',(157.454347159998,-227.591691842397,4.91800280297972));
#84825=CARTESIAN_POINT('Ctrl Pts',(156.441904766836,-224.26707892683,4.75924493774792));
#84826=CARTESIAN_POINT('Ctrl Pts',(158.685830991148,-221.613235348605,4.60048707251613));
#84827=CARTESIAN_POINT('Ctrl Pts',(162.132484640682,-222.05895864616,4.44172920728435));
#84828=CARTESIAN_POINT('Ctrl Pts',(163.627488430923,-225.196322875086,4.28297134205254));
#84829=CARTESIAN_POINT('Ctrl Pts',(161.802614951828,-228.154012416474,4.12421347682076));
#84830=CARTESIAN_POINT('Ctrl Pts',(158.327988339714,-228.225149918293,3.96545561158896));
#84831=CARTESIAN_POINT('Ctrl Pts',(156.383586733325,-225.344630341799,3.80669774635717));
#84832=CARTESIAN_POINT('Ctrl Pts',(157.748926406423,-222.148705089872,3.64793988112538));
#84833=CARTESIAN_POINT('Ctrl Pts',(161.174448543763,-221.562284827925,3.48918201589358));
#84834=CARTESIAN_POINT('Ctrl Pts',(163.525115420198,-224.122061355537,3.33042415066179));
#84835=CARTESIAN_POINT('Ctrl Pts',(162.649596802351,-227.485327297572,3.17166628543));
#84836=CARTESIAN_POINT('Ctrl Pts',(159.349167295888,-228.574021791418,3.01290842019821));
#84837=CARTESIAN_POINT('Ctrl Pts',(156.644379853178,-226.39177168891,2.85415055496641));
#84838=CARTESIAN_POINT('Ctrl Pts',(157.010655839907,-222.935772177733,2.69539268973463));
#84839=CARTESIAN_POINT('Ctrl Pts',(160.112779478126,-221.368953916766,2.53663482450283));
#84840=CARTESIAN_POINT('Ctrl Pts',(163.111687355417,-223.125268829368,2.37787695927104));
#84841=CARTESIAN_POINT('Ctrl Pts',(163.262779060384,-226.597337758068,2.21911909403925));
#84842=CARTESIAN_POINT('Ctrl Pts',(160.427775553637,-228.607522979317,2.06036122880745));
#84843=CARTESIAN_POINT('Ctrl Pts',(157.201271760739,-227.316103838939,1.90160336357566));
#84844=CARTESIAN_POINT('Ctrl Pts',(156.536164183628,-223.904985462419,1.74284549834387));
#84845=CARTESIAN_POINT('Ctrl Pts',(159.041158508843,-221.496026617155,1.58408763311207));
#84846=CARTESIAN_POINT('Ctrl Pts',(162.423685567743,-222.293899365156,1.42532976788028));
#84847=CARTESIAN_POINT('Ctrl Pts',(163.588053535237,-225.568405078077,1.26657190264849));
#84848=CARTESIAN_POINT('Ctrl Pts',(161.468639519931,-228.322686213904,1.1078140374167));
#84849=CARTESIAN_POINT('Ctrl Pts',(158.005117395928,-228.036087118832,0.949056172184905));
#84850=CARTESIAN_POINT('Ctrl Pts',(156.367331002864,-224.970773940809,0.790298306953113));
#84851=CARTESIAN_POINT('Ctrl Pts',(158.054123192547,-221.932389526572,0.631540441721319));
#84852=CARTESIAN_POINT('Ctrl Pts',(161.52186463808,-221.701106398635,0.472782576489526));
#84853=CARTESIAN_POINT('Ctrl Pts',(163.596623766652,-224.489750196051,0.314024711257736));
#84854=CARTESIAN_POINT('Ctrl Pts',(162.380110634752,-227.743757872981,0.15526684602594));
#84855=CARTESIAN_POINT('Ctrl Pts',(158.984594590514,-228.490053105179,-0.00349101920584808));
#84856=CARTESIAN_POINT('Ctrl Pts',(156.520034264226,-226.035336592024,-0.162248884437644));
#84857=CARTESIAN_POINT('Ctrl Pts',(156.999831188384,-223.779443237332,-0.268087461258838));
#84858=CARTESIAN_POINT('Ctrl Pts',(157.663937342304,-223.002698443069,-0.321006749669435));
#84859=CARTESIAN_POINT('Ctrl Pts',(159.254067145653,-227.790177569842,20.1070022498898));
#84860=CARTESIAN_POINT('Ctrl Pts',(158.326328373192,-227.542153631111,20.0540829614792));
#84861=CARTESIAN_POINT('Ctrl Pts',(156.753991824467,-226.05055982535,19.948244384658));
#84862=CARTESIAN_POINT('Ctrl Pts',(157.355959284165,-222.837758975168,19.7894865194262));
#84863=CARTESIAN_POINT('Ctrl Pts',(160.382716585329,-221.608314425637,19.6307286541944));
#84864=CARTESIAN_POINT('Ctrl Pts',(163.056853377018,-223.480713328787,19.4719707889626));
#84865=CARTESIAN_POINT('Ctrl Pts',(162.934495616441,-226.744624953805,19.3132129237309));
#84866=CARTESIAN_POINT('Ctrl Pts',(160.125939507437,-228.411343615433,19.154455058499));
#84867=CARTESIAN_POINT('Ctrl Pts',(157.202387726272,-226.956247563464,18.9956971932673));
#84868=CARTESIAN_POINT('Ctrl Pts',(156.839083273915,-223.710674851695,18.8369393280355));
#84869=CARTESIAN_POINT('Ctrl Pts',(159.368711045569,-221.645149801924,18.6781814628037));
#84870=CARTESIAN_POINT('Ctrl Pts',(162.476064870033,-222.649955887244,18.5194235975719));
#84871=CARTESIAN_POINT('Ctrl Pts',(163.317338476092,-225.805535570802,18.3606657323401));
#84872=CARTESIAN_POINT('Ctrl Pts',(161.122577169746,-228.223882712554,18.2019078671083));
#84873=CARTESIAN_POINT('Ctrl Pts',(157.900436592647,-227.691735616307,18.0431500018765));
#84874=CARTESIAN_POINT('Ctrl Pts',(156.599814767689,-224.696110698794,17.8843921366447));
#84875=CARTESIAN_POINT('Ctrl Pts',(158.411043102702,-221.978605976434,17.7256342714129));
#84876=CARTESIAN_POINT('Ctrl Pts',(161.676484356976,-222.026280599272,17.5668764061811));
#84877=CARTESIAN_POINT('Ctrl Pts',(163.407607372316,-224.795503267648,17.4081185409493));
#84878=CARTESIAN_POINT('Ctrl Pts',(162.020088168414,-227.751881256977,17.2493606757175));
#84879=CARTESIAN_POINT('Ctrl Pts',(158.783784393714,-228.189737666912,17.0906028104858));
#84880=CARTESIAN_POINT('Ctrl Pts',(156.66056107406,-225.708346270834,16.9318449452539));
#84881=CARTESIAN_POINT('Ctrl Pts',(157.593592137746,-222.578676404551,16.7730870800222));
#84882=CARTESIAN_POINT('Ctrl Pts',(160.728967577691,-221.665001793266,16.6143292147904));
#84883=CARTESIAN_POINT('Ctrl Pts',(163.197191921438,-223.803517411731,16.4555713495586));
#84884=CARTESIAN_POINT('Ctrl Pts',(162.739346343332,-227.03705384692,16.2968134843268));
#84885=CARTESIAN_POINT('Ctrl Pts',(159.774451100051,-228.406278682,16.138055619095));
#84886=CARTESIAN_POINT('Ctrl Pts',(157.015978200883,-226.658077401028,15.9792977538632));
#84887=CARTESIAN_POINT('Ctrl Pts',(156.988481935044,-223.39240374795,15.8205398886314));
#84888=CARTESIAN_POINT('Ctrl Pts',(159.717126883769,-221.598002121477,15.6617820233996));
#84889=CARTESIAN_POINT('Ctrl Pts',(162.704657297373,-222.917108819674,15.5030241581678));
#84890=CARTESIAN_POINT('Ctrl Pts',(163.216885458766,-226.142477444185,15.344266292936));
#84891=CARTESIAN_POINT('Ctrl Pts',(160.785020174804,-228.322250756711,15.1855084277043));
#84892=CARTESIAN_POINT('Ctrl Pts',(157.634704457728,-227.461500307336,15.0267505624724));
#84893=CARTESIAN_POINT('Ctrl Pts',(156.649107127928,-224.347984873485,14.8679926972407));
#84894=CARTESIAN_POINT('Ctrl Pts',(158.730246822877,-221.83119365778,14.7092348320089));
#84895=CARTESIAN_POINT('Ctrl Pts',(161.973464575598,-222.214493881865,14.5504769667771));
#84896=CARTESIAN_POINT('Ctrl Pts',(163.410567626335,-225.147089195729,14.3917191015453));
#84897=CARTESIAN_POINT('Ctrl Pts',(161.726319319569,-227.945068483447,14.2329612363135));
#84898=CARTESIAN_POINT('Ctrl Pts',(158.462143639418,-228.047721210926,14.0742033710817));
#84899=CARTESIAN_POINT('Ctrl Pts',(156.605414039998,-225.361099606014,13.9154455058499));
#84900=CARTESIAN_POINT('Ctrl Pts',(157.855409377682,-222.343999655878,13.7566876406181));
#84901=CARTESIAN_POINT('Ctrl Pts',(161.068133968578,-221.757671116238,13.5979297753863));
#84902=CARTESIAN_POINT('Ctrl Pts',(163.303302393434,-224.138721843515,13.4391719101545));
#84903=CARTESIAN_POINT('Ctrl Pts',(162.515288597719,-227.308014305738,13.2804140449227));
#84904=CARTESIAN_POINT('Ctrl Pts',(159.425282776282,-228.36501216611,13.1216561796909));
#84905=CARTESIAN_POINT('Ctrl Pts',(156.861258135392,-226.342351024384,12.9628983144591));
#84906=CARTESIAN_POINT('Ctrl Pts',(157.169809925563,-223.091170277928,12.8041404492273));
#84907=CARTESIAN_POINT('Ctrl Pts',(160.068551560564,-221.586950418049,12.6453825839956));
#84908=CARTESIAN_POINT('Ctrl Pts',(162.904554810033,-223.206353401357,12.4866247187638));
#84909=CARTESIAN_POINT('Ctrl Pts',(163.082309611578,-226.467301681209,12.327866853532));
#84910=CARTESIAN_POINT('Ctrl Pts',(160.439134777816,-228.385375520119,12.1691089883002));
#84911=CARTESIAN_POINT('Ctrl Pts',(157.394063812665,-227.205153816143,12.0103511230684));
#84912=CARTESIAN_POINT('Ctrl Pts',(156.733945543687,-224.006775426348,11.8515932578366));
#84913=CARTESIAN_POINT('Ctrl Pts',(159.062920184692,-221.717396127302,11.6928353926048));
#84914=CARTESIAN_POINT('Ctrl Pts',(162.249510235817,-222.432255763464,11.534077527373));
#84915=CARTESIAN_POINT('Ctrl Pts',(163.377348607582,-225.49711482393,11.3753196621412));
#84916=CARTESIAN_POINT('Ctrl Pts',(161.414237666499,-228.107014417083,11.2165617969094));
#84917=CARTESIAN_POINT('Ctrl Pts',(158.15681646865,-227.873374537903,11.0578039316776));
#84918=CARTESIAN_POINT('Ctrl Pts',(156.586276766211,-225.010022394626,10.8990460664458));
#84919=CARTESIAN_POINT('Ctrl Pts',(158.139976433094,-222.137497756182,10.7402882012141));
#84920=CARTESIAN_POINT('Ctrl Pts',(161.395969595266,-221.884735058715,10.5815303359823));
#84921=CARTESIAN_POINT('Ctrl Pts',(163.374371438746,-224.483062713007,10.4227724707505));
#84922=CARTESIAN_POINT('Ctrl Pts',(162.264548674179,-227.554491352027,10.2640146055187));
#84923=CARTESIAN_POINT('Ctrl Pts',(159.082211052055,-228.288049606125,10.1052567402869));
#84924=CARTESIAN_POINT('Ctrl Pts',(156.739833838999,-226.012384989997,9.94649887505509));
#84925=CARTESIAN_POINT('Ctrl Pts',(157.381160568288,-222.810185670835,9.78774100982331));
#84926=CARTESIAN_POINT('Ctrl Pts',(160.419249042497,-221.612104339612,9.6289831445915));
#84927=CARTESIAN_POINT('Ctrl Pts',(163.073640809499,-223.514624983551,9.47022527935972));
#84928=CARTESIAN_POINT('Ctrl Pts',(162.915036628516,-226.776560784133,9.31146741412792));
#84929=CARTESIAN_POINT('Ctrl Pts',(160.088591039746,-228.412588224938,9.15270954889613));
#84930=CARTESIAN_POINT('Ctrl Pts',(157.181066934884,-226.925415056476,8.99395168366434));
#84931=CARTESIAN_POINT('Ctrl Pts',(156.853430260365,-223.676102104043,8.83519381843255));
#84932=CARTESIAN_POINT('Ctrl Pts',(159.405534087823,-221.638420453928,8.67643595320075));
#84933=CARTESIAN_POINT('Ctrl Pts',(162.501693094729,-222.677256272187,8.51767808796897));
#84934=CARTESIAN_POINT('Ctrl Pts',(163.308302679716,-225.841867058801,8.35892022273717));
#84935=CARTESIAN_POINT('Ctrl Pts',(161.087153782322,-228.236001146306,8.20016235750538));
#84936=CARTESIAN_POINT('Ctrl Pts',(157.871041786099,-227.668547111964,8.04140449227359));
#84937=CARTESIAN_POINT('Ctrl Pts',(156.603352263518,-224.658838865691,7.88264662704179));
#84938=CARTESIAN_POINT('Ctrl Pts',(158.444274615796,-221.961361276122,7.72388876181));
#84939=CARTESIAN_POINT('Ctrl Pts',(161.70899677852,-222.044845727154,7.56513089657821));
#84940=CARTESIAN_POINT('Ctrl Pts',(163.409645156747,-224.832887252487,7.40637303134642));
#84941=CARTESIAN_POINT('Ctrl Pts',(161.9897864216,-227.773870357772,7.24761516611462));
#84942=CARTESIAN_POINT('Ctrl Pts',(158.748875231651,-228.176207420704,7.08885730088284));
#84943=CARTESIAN_POINT('Ctrl Pts',(156.652993380496,-225.671679577109,6.93009943565103));
#84944=CARTESIAN_POINT('Ctrl Pts',(157.620291855893,-222.552430610957,6.77134157041925));
#84945=CARTESIAN_POINT('Ctrl Pts',(160.765499131197,-221.673197053409,6.61258370518745));
#84946=CARTESIAN_POINT('Ctrl Pts',(163.210121631732,-223.838653421758,6.45382583995566));
#84947=CARTESIAN_POINT('Ctrl Pts',(162.716840941141,-227.066974132844,6.29506797472387));
#84948=CARTESIAN_POINT('Ctrl Pts',(159.737107528055,-228.403600198834,6.13631010949207));
#84949=CARTESIAN_POINT('Ctrl Pts',(156.997973294955,-226.625251496694,5.97755224426028));
#84950=CARTESIAN_POINT('Ctrl Pts',(157.006293784261,-223.359472688691,5.81879437902849));
#84951=CARTESIAN_POINT('Ctrl Pts',(159.754454084486,-221.595104411486,5.6600365137967));
#84952=CARTESIAN_POINT('Ctrl Pts',(162.727337996934,-222.946896442995,5.5012786485649));
#84953=CARTESIAN_POINT('Ctrl Pts',(163.204162281838,-226.177688769139,5.34252078333312));
#84954=CARTESIAN_POINT('Ctrl Pts',(160.748537372404,-228.330660380078,5.18376291810132));
#84955=CARTESIAN_POINT('Ctrl Pts',(157.607851089182,-227.435411742145,5.02500505286953));
#84956=CARTESIAN_POINT('Ctrl Pts',(156.656459395071,-224.311274373572,4.86624718763773));
#84957=CARTESIAN_POINT('Ctrl Pts',(158.76507593111,-221.81745867122,4.70748932240594));
#84958=CARTESIAN_POINT('Ctrl Pts',(162.003894926434,-222.236304667822,4.54873145717415));
#84959=CARTESIAN_POINT('Ctrl Pts',(163.408749363889,-225.184484523744,4.38997359194236));
#84960=CARTESIAN_POINT('Ctrl Pts',(161.693916517555,-227.963824150809,4.23121572671057));
#84961=CARTESIAN_POINT('Ctrl Pts',(158.428811340974,-228.030672031565,4.07245786147877));
#84962=CARTESIAN_POINT('Ctrl Pts',(156.601657963332,-225.323848988289,3.91369999624698));
#84963=CARTESIAN_POINT('Ctrl Pts',(157.884667084047,-222.320639363504,3.75494213101519));
#84964=CARTESIAN_POINT('Ctrl Pts',(161.103628806185,-221.769580488212,3.5961842657834));
#84965=CARTESIAN_POINT('Ctrl Pts',(163.312549488455,-224.17500142238,3.4374264005516));
#84966=CARTESIAN_POINT('Ctrl Pts',(162.489825008836,-227.335461023785,3.27866853531981));
#84967=CARTESIAN_POINT('Ctrl Pts',(159.3884127797,-228.35850678507,3.11991067008802));
#84968=CARTESIAN_POINT('Ctrl Pts',(156.846725149163,-226.307847274938,2.96115280485623));
#84969=CARTESIAN_POINT('Ctrl Pts',(157.190914540955,-223.060245977329,2.80239493962443));
#84970=CARTESIAN_POINT('Ctrl Pts',(160.105978828504,-221.58790751172,2.64363707439264));
#84971=CARTESIAN_POINT('Ctrl Pts',(162.924051308607,-223.238315901747,2.48487920916085));
#84972=CARTESIAN_POINT('Ctrl Pts',(163.066032120677,-226.501017624291,2.32612134392906));
#84973=CARTESIAN_POINT('Ctrl Pts',(160.401980509136,-228.38998783735,2.16736347869726));
#84974=CARTESIAN_POINT('Ctrl Pts',(157.37003624217,-227.176441810367,2.00860561346547));
#84975=CARTESIAN_POINT('Ctrl Pts',(156.745034929673,-223.971015296256,1.84984774823368));
#84976=CARTESIAN_POINT('Ctrl Pts',(159.098977051121,-221.707317675217,1.69108988300188));
#84977=CARTESIAN_POINT('Ctrl Pts',(162.277536316003,-222.457078363364,1.53233201777009));
#84978=CARTESIAN_POINT('Ctrl Pts',(163.371692408878,-225.534130014532,1.3735741525383));
#84979=CARTESIAN_POINT('Ctrl Pts',(161.380079943652,-228.122326847825,1.21481628730651));
#84980=CARTESIAN_POINT('Ctrl Pts',(158.125409649912,-227.853009797855,1.05605842207471));
#84981=CARTESIAN_POINT('Ctrl Pts',(156.586382460205,-224.972536284381,0.897300556842924));
#84982=CARTESIAN_POINT('Ctrl Pts',(158.171460376533,-222.117367718994,0.738542691611129));
#84983=CARTESIAN_POINT('Ctrl Pts',(161.430095564953,-221.900031060243,0.579784826379336));
#84984=CARTESIAN_POINT('Ctrl Pts',(163.37974585176,-224.520518472282,0.421026961147546));
#84985=CARTESIAN_POINT('Ctrl Pts',(162.236588969666,-227.57830812759,0.26226909591575));
#84986=CARTESIAN_POINT('Ctrl Pts',(159.045823960686,-228.279601445673,0.103511230683962));
#84987=CARTESIAN_POINT('Ctrl Pts',(156.729877651146,-225.972905363223,-0.0552466345478339));
#84988=CARTESIAN_POINT('Ctrl Pts',(157.180742620438,-223.853043319762,-0.161085211369028));
#84989=CARTESIAN_POINT('Ctrl Pts',(157.804802895981,-223.123136560921,-0.214004499779625));
#84990=CARTESIAN_POINT('Ctrl Pts',(159.301933573839,-227.611132185939,20.2140044997796));
#84991=CARTESIAN_POINT('Ctrl Pts',(158.43372769508,-227.379023915733,20.161085211369));
#84992=CARTESIAN_POINT('Ctrl Pts',(156.96228780757,-225.983145518363,20.0552466345478));
#84993=CARTESIAN_POINT('Ctrl Pts',(157.525627082423,-222.976509740914,19.896488769316));
#84994=CARTESIAN_POINT('Ctrl Pts',(160.358157704673,-221.825958511198,19.7377309040842));
#84995=CARTESIAN_POINT('Ctrl Pts',(162.860695436269,-223.57820578527,19.5789730388524));
#84996=CARTESIAN_POINT('Ctrl Pts',(162.746189359561,-226.632672564826,19.4202151736207));
#84997=CARTESIAN_POINT('Ctrl Pts',(160.117857983271,-228.192438075565,19.2614573083889));
#84998=CARTESIAN_POINT('Ctrl Pts',(157.381910194295,-226.830715375192,19.1026994431571));
#84999=CARTESIAN_POINT('Ctrl Pts',(157.041918948184,-223.793410702864,18.9439415779253));
#85000=CARTESIAN_POINT('Ctrl Pts',(159.409220787465,-221.860430165491,18.7851837126935));
#85001=CARTESIAN_POINT('Ctrl Pts',(162.317176063092,-222.800757956226,18.6264258474617));
#85002=CARTESIAN_POINT('Ctrl Pts',(163.104465235546,-225.75384444294,18.4676679822299));
#85003=CARTESIAN_POINT('Ctrl Pts',(161.050541517789,-228.017006517946,18.3089101169981));
#85004=CARTESIAN_POINT('Ctrl Pts',(158.03516534266,-227.519007241598,18.1501522517663));
#85005=CARTESIAN_POINT('Ctrl Pts',(156.818004275354,-224.715611241407,17.9913943865345));
#85006=CARTESIAN_POINT('Ctrl Pts',(158.513006289833,-222.172488494422,17.8326365213027));
#85007=CARTESIAN_POINT('Ctrl Pts',(161.568904542505,-222.217103842021,17.673878656071));
#85008=CARTESIAN_POINT('Ctrl Pts',(163.188941586754,-224.808625800187,17.5151207908391));
#85009=CARTESIAN_POINT('Ctrl Pts',(161.890459335632,-227.575293343204,17.3563629256074));
#85010=CARTESIAN_POINT('Ctrl Pts',(158.861828813714,-227.98505255608,17.1976050603756));
#85011=CARTESIAN_POINT('Ctrl Pts',(156.874852498011,-225.662891769525,17.0388471951438));
#85012=CARTESIAN_POINT('Ctrl Pts',(157.748011062256,-222.734052469999,16.880089329912));
#85013=CARTESIAN_POINT('Ctrl Pts',(160.682189809418,-221.87900825676,16.7213314646802));
#85014=CARTESIAN_POINT('Ctrl Pts',(162.992028471923,-223.880295566163,16.5625735994484));
#85015=CARTESIAN_POINT('Ctrl Pts',(162.563562793573,-226.906336328438,16.4038157342166));
#85016=CARTESIAN_POINT('Ctrl Pts',(159.788924547841,-228.187698158347,16.2450578689848));
#85017=CARTESIAN_POINT('Ctrl Pts',(157.20746254739,-226.55167875887,16.086300003753));
#85018=CARTESIAN_POINT('Ctrl Pts',(157.181730713867,-223.4955630204,15.9275421385212));
#85019=CARTESIAN_POINT('Ctrl Pts',(159.735278820133,-221.816307946447,15.7687842732894));
#85020=CARTESIAN_POINT('Ctrl Pts',(162.531099739829,-223.050767714736,15.6100264080576));
#85021=CARTESIAN_POINT('Ctrl Pts',(163.010458277155,-226.069164793834,15.4512685428258));
#85022=CARTESIAN_POINT('Ctrl Pts',(160.734645517617,-228.109062295665,15.2925106775941));
#85023=CARTESIAN_POINT('Ctrl Pts',(157.786485209243,-227.303546106762,15.1337528123623));
#85024=CARTESIAN_POINT('Ctrl Pts',(156.864133550327,-224.389824611536,14.9749949471305));
#85025=CARTESIAN_POINT('Ctrl Pts',(158.811726742836,-222.034535607837,14.8162370818987));
#85026=CARTESIAN_POINT('Ctrl Pts',(161.846827573574,-222.393239499232,14.6574792166669));
#85027=CARTESIAN_POINT('Ctrl Pts',(163.191711881602,-225.137650498421,14.4987213514351));
#85028=CARTESIAN_POINT('Ctrl Pts',(161.615541601099,-227.756083766868,14.3399634862033));
#85029=CARTESIAN_POINT('Ctrl Pts',(158.5608277108,-227.852149280258,14.1812056209715));
#85030=CARTESIAN_POINT('Ctrl Pts',(156.823244242982,-225.337927884513,14.0224477557397));
#85031=CARTESIAN_POINT('Ctrl Pts',(157.993027519065,-222.514434902151,13.8636898905079));
#85032=CARTESIAN_POINT('Ctrl Pts',(160.999591930777,-221.965730999598,13.7049320252761));
#85033=CARTESIAN_POINT('Ctrl Pts',(163.09132984675,-224.193989966893,13.5461741600443));
#85034=CARTESIAN_POINT('Ctrl Pts',(162.353882808541,-227.159909284792,13.3874162948125));
#85035=CARTESIAN_POINT('Ctrl Pts',(159.46216231652,-228.149079710186,13.2286584295808));
#85036=CARTESIAN_POINT('Ctrl Pts',(157.06267085127,-226.256212508652,13.069900564349));
#85037=CARTESIAN_POINT('Ctrl Pts',(157.35142290743,-223.2136596686,12.9111426991172));
#85038=CARTESIAN_POINT('Ctrl Pts',(160.064152614558,-221.805965429598,12.7523848338854));
#85039=CARTESIAN_POINT('Ctrl Pts',(162.718169851365,-223.321451503826,12.5936269686536));
#85040=CARTESIAN_POINT('Ctrl Pts',(162.884518147092,-226.373145095745,12.4348691034218));
#85041=CARTESIAN_POINT('Ctrl Pts',(160.410955548032,-228.168136350036,12.27611123819));
#85042=CARTESIAN_POINT('Ctrl Pts',(157.561286447573,-227.063649341357,12.1173533729582));
#85043=CARTESIAN_POINT('Ctrl Pts',(156.943527894395,-224.07051053662,11.9585955077264));
#85044=CARTESIAN_POINT('Ctrl Pts',(159.123052492074,-221.928040452216,11.7998376424946));
#85045=CARTESIAN_POINT('Ctrl Pts',(162.105159414521,-222.597027625143,11.6410797772628));
#85046=CARTESIAN_POINT('Ctrl Pts',(163.160624523583,-225.465215021044,11.482321912031));
#85047=CARTESIAN_POINT('Ctrl Pts',(161.323486192949,-227.90763764798,11.3235640467992));
#85048=CARTESIAN_POINT('Ctrl Pts',(158.275093350574,-227.688990413825,11.1648061815675));
#85049=CARTESIAN_POINT('Ctrl Pts',(156.805335005923,-225.009379258679,11.0060483163357));
#85050=CARTESIAN_POINT('Ctrl Pts',(158.259333938224,-222.32118420636,10.8472904511039));
#85051=CARTESIAN_POINT('Ctrl Pts',(161.306390381813,-222.084641263038,10.6885325858721));
#85052=CARTESIAN_POINT('Ctrl Pts',(163.157838399339,-224.51623452114,10.5297747206403));
#85053=CARTESIAN_POINT('Ctrl Pts',(162.119232837969,-227.390569926471,10.3710168554085));
#85054=CARTESIAN_POINT('Ctrl Pts',(159.141105466627,-228.077055829103,10.2122589901767));
#85055=CARTESIAN_POINT('Ctrl Pts',(156.949038338452,-225.947420357942,10.0535011249449));
#85056=CARTESIAN_POINT('Ctrl Pts',(157.54921120295,-222.950705812449,9.89474325971312));
#85057=CARTESIAN_POINT('Ctrl Pts',(160.392345878133,-221.829505226816,9.73598539448132));
#85058=CARTESIAN_POINT('Ctrl Pts',(162.876405621077,-223.609941332924,9.57722752924953));
#85059=CARTESIAN_POINT('Ctrl Pts',(162.727979052723,-226.662559076478,9.41846966401773));
#85060=CARTESIAN_POINT('Ctrl Pts',(160.082906162592,-228.193602818617,9.25971179878594));
#85061=CARTESIAN_POINT('Ctrl Pts',(157.361957555717,-226.801861386744,9.10095393355414));
#85062=CARTESIAN_POINT('Ctrl Pts',(157.055345290111,-223.761056484579,8.94219606832236));
#85063=CARTESIAN_POINT('Ctrl Pts',(159.4436808992,-221.854132639007,8.78343820309056));
#85064=CARTESIAN_POINT('Ctrl Pts',(162.341159727464,-222.826306478508,8.62468033785878));
#85065=CARTESIAN_POINT('Ctrl Pts',(163.096009265217,-225.7878445434,8.46592247262697));
#85066=CARTESIAN_POINT('Ctrl Pts',(161.017391245191,-228.028347313154,8.30716460739519));
#85067=CARTESIAN_POINT('Ctrl Pts',(158.007656797574,-227.497306740996,8.1484067421634));
#85068=CARTESIAN_POINT('Ctrl Pts',(156.82131477047,-224.680731137683,7.9896488769316));
#85069=CARTESIAN_POINT('Ctrl Pts',(158.544105340433,-222.156350384608,7.83089101169981));
#85070=CARTESIAN_POINT('Ctrl Pts',(161.59933064558,-222.234477647715,7.67213314646802));
#85071=CARTESIAN_POINT('Ctrl Pts',(163.190848606784,-224.843610858883,7.51337528123622));
#85072=CARTESIAN_POINT('Ctrl Pts',(161.862102048537,-227.595871405851,7.35461741600443));
#85073=CARTESIAN_POINT('Ctrl Pts',(158.829159768693,-227.972390544264,7.19585955077264));
#85074=CARTESIAN_POINT('Ctrl Pts',(156.8677704225,-225.628577973453,7.03710168554085));
#85075=CARTESIAN_POINT('Ctrl Pts',(157.772997462463,-222.709490866057,6.87834382030905));
#85076=CARTESIAN_POINT('Ctrl Pts',(160.716377137205,-221.886677627973,6.71958595507726));
#85077=CARTESIAN_POINT('Ctrl Pts',(163.004128484148,-223.91317690234,6.56082808984547));
#85078=CARTESIAN_POINT('Ctrl Pts',(162.542501560533,-226.934336632947,6.40207022461368));
#85079=CARTESIAN_POINT('Ctrl Pts',(159.7539773087,-228.185191553147,6.24331235938189));
#85080=CARTESIAN_POINT('Ctrl Pts',(157.19061301427,-226.520959289162,6.08455449415009));
#85081=CARTESIAN_POINT('Ctrl Pts',(157.198399578703,-223.464745143546,5.9257966289183));
#85082=CARTESIAN_POINT('Ctrl Pts',(159.770210738537,-221.813596182184,5.76703876368651));
#85083=CARTESIAN_POINT('Ctrl Pts',(162.552325021425,-223.078643869585,5.60828089845471));
#85084=CARTESIAN_POINT('Ctrl Pts',(162.998551545073,-226.102116611987,5.44952303322292));
#85085=CARTESIAN_POINT('Ctrl Pts',(160.700503812585,-228.116932274438,5.29076516799113));
#85086=CARTESIAN_POINT('Ctrl Pts',(157.761355018366,-227.279131641893,5.13200730275934));
#85087=CARTESIAN_POINT('Ctrl Pts',(156.871014023306,-224.355469820314,4.97324943752755));
#85088=CARTESIAN_POINT('Ctrl Pts',(158.844320871072,-222.021681993836,4.81449157229575));
#85089=CARTESIAN_POINT('Ctrl Pts',(161.875305212187,-222.413650689484,4.65573370706397));
#85090=CARTESIAN_POINT('Ctrl Pts',(163.190010296854,-225.172646172402,4.49697584183216));
#85091=CARTESIAN_POINT('Ctrl Pts',(161.585218083281,-227.773635885145,4.33821797660038));
#85092=CARTESIAN_POINT('Ctrl Pts',(158.529634342234,-227.836194144838,4.17946011136858));
#85093=CARTESIAN_POINT('Ctrl Pts',(156.819729193338,-225.303067634779,4.02070224613679));
#85094=CARTESIAN_POINT('Ctrl Pts',(158.020407761671,-222.492573637137,3.861944380905));
#85095=CARTESIAN_POINT('Ctrl Pts',(161.032809068608,-221.976876148499,3.70318651567321));
#85096=CARTESIAN_POINT('Ctrl Pts',(163.099983556713,-224.227941489222,3.54442865044141));
#85097=CARTESIAN_POINT('Ctrl Pts',(162.33005321532,-227.185594749999,3.38567078520962));
#85098=CARTESIAN_POINT('Ctrl Pts',(159.427658263512,-228.142991778722,3.22691291997783));
#85099=CARTESIAN_POINT('Ctrl Pts',(157.049070445148,-226.223922860965,3.06815505474604));
#85100=CARTESIAN_POINT('Ctrl Pts',(157.371173242002,-223.184719776926,2.90939718951424));
#85101=CARTESIAN_POINT('Ctrl Pts',(160.099178178882,-221.806861106675,2.75063932428245));
#85102=CARTESIAN_POINT('Ctrl Pts',(162.736415261797,-223.351362974126,2.59188145905066));
#85103=CARTESIAN_POINT('Ctrl Pts',(162.869285180969,-226.404697490515,2.43312359381887));
#85104=CARTESIAN_POINT('Ctrl Pts',(160.376185464635,-228.172452695384,2.27436572858707));
#85105=CARTESIAN_POINT('Ctrl Pts',(157.5388007236,-227.036779781794,2.11560786335528));
#85106=CARTESIAN_POINT('Ctrl Pts',(156.953905675717,-224.037045130094,1.95684999812349));
#85107=CARTESIAN_POINT('Ctrl Pts',(159.156795593401,-221.918608733279,1.79809213289169));
#85108=CARTESIAN_POINT('Ctrl Pts',(162.131387064264,-222.620257361572,1.6393342676599));
#85109=CARTESIAN_POINT('Ctrl Pts',(163.155331282519,-225.499854950988,1.48057640242811));
#85110=CARTESIAN_POINT('Ctrl Pts',(161.291520367372,-227.921967481746,1.32181853719632));
#85111=CARTESIAN_POINT('Ctrl Pts',(158.245701903897,-227.669932476878,1.16306067196452));
#85112=CARTESIAN_POINT('Ctrl Pts',(156.805433917545,-224.974298627954,1.00430280673273));
#85113=CARTESIAN_POINT('Ctrl Pts',(158.28879756052,-222.302345911416,0.845544941500939));
#85114=CARTESIAN_POINT('Ctrl Pts',(161.338326491825,-222.098955721852,0.686787076269146));
#85115=CARTESIAN_POINT('Ctrl Pts',(163.162867936868,-224.551286748514,0.528029211037356));
#85116=CARTESIAN_POINT('Ctrl Pts',(162.093067304581,-227.412858382199,0.36927134580556));
#85117=CARTESIAN_POINT('Ctrl Pts',(159.107053330859,-228.069149786166,0.210513480573772));
#85118=CARTESIAN_POINT('Ctrl Pts',(156.939721038065,-225.910474134421,0.0517556153419763));
#85119=CARTESIAN_POINT('Ctrl Pts',(157.361654052493,-223.926643402192,-0.0540829614792177));
#85120=CARTESIAN_POINT('Ctrl Pts',(157.945668449658,-223.243574678773,-0.107002249889815));
#85121=CARTESIAN_POINT('Ctrl Pts',(159.349800002025,-227.432086802035,20.3210067496694));
#85122=CARTESIAN_POINT('Ctrl Pts',(158.541127016969,-227.215894200354,20.2680874612588));
#85123=CARTESIAN_POINT('Ctrl Pts',(157.170583790673,-225.915731211375,20.1622488844376));
#85124=CARTESIAN_POINT('Ctrl Pts',(157.695294880681,-223.11526050666,20.0034910192058));
#85125=CARTESIAN_POINT('Ctrl Pts',(160.333598824017,-222.043602596759,19.8447331539741));
#85126=CARTESIAN_POINT('Ctrl Pts',(162.664537495519,-223.675698241753,19.6859752887422));
#85127=CARTESIAN_POINT('Ctrl Pts',(162.55788310268,-226.520720175846,19.5272174235105));
#85128=CARTESIAN_POINT('Ctrl Pts',(160.109776459105,-227.973532535698,19.3684595582787));
#85129=CARTESIAN_POINT('Ctrl Pts',(157.561432662319,-226.705183186919,19.2097016930469));
#85130=CARTESIAN_POINT('Ctrl Pts',(157.244754622453,-223.876146554034,19.0509438278151));
#85131=CARTESIAN_POINT('Ctrl Pts',(159.449730529362,-222.075710529059,18.8921859625833));
#85132=CARTESIAN_POINT('Ctrl Pts',(162.158287256151,-222.951560025208,18.7334280973515));
#85133=CARTESIAN_POINT('Ctrl Pts',(162.891591995001,-225.702153315077,18.5746702321197));
#85134=CARTESIAN_POINT('Ctrl Pts',(160.978505865832,-227.810130323338,18.4159123668879));
#85135=CARTESIAN_POINT('Ctrl Pts',(158.169894092673,-227.346278866889,18.2571545016561));
#85136=CARTESIAN_POINT('Ctrl Pts',(157.03619378302,-224.73511178402,18.0983966364243));
#85137=CARTESIAN_POINT('Ctrl Pts',(158.614969476964,-222.366371012409,17.9396387711925));
#85138=CARTESIAN_POINT('Ctrl Pts',(161.461324728035,-222.407927084771,17.7808809059608));
#85139=CARTESIAN_POINT('Ctrl Pts',(162.970275801191,-224.821748332727,17.622123040729));
#85140=CARTESIAN_POINT('Ctrl Pts',(161.76083050285,-227.398705429432,17.4633651754972));
#85141=CARTESIAN_POINT('Ctrl Pts',(158.939873233715,-227.780367445248,17.3046073102654));
#85142=CARTESIAN_POINT('Ctrl Pts',(157.089143921962,-225.617437268217,17.1458494450336));
#85143=CARTESIAN_POINT('Ctrl Pts',(157.902429986765,-222.889428535446,16.9870915798018));
#85144=CARTESIAN_POINT('Ctrl Pts',(160.635412041146,-222.093014720254,16.82833371457));
#85145=CARTESIAN_POINT('Ctrl Pts',(162.786865022409,-223.957073720595,16.6695758493382));
#85146=CARTESIAN_POINT('Ctrl Pts',(162.387779243813,-226.775618809956,16.5108179841064));
#85147=CARTESIAN_POINT('Ctrl Pts',(159.80339799563,-227.969117634694,16.3520601188746));
#85148=CARTESIAN_POINT('Ctrl Pts',(157.398946893897,-226.445280116713,16.1933022536428));
#85149=CARTESIAN_POINT('Ctrl Pts',(157.37497949269,-223.598722292849,16.034544388411));
#85150=CARTESIAN_POINT('Ctrl Pts',(159.753430756497,-222.034613771418,15.8757865231792));
#85151=CARTESIAN_POINT('Ctrl Pts',(162.357542182285,-223.184426609798,15.7170286579475));
#85152=CARTESIAN_POINT('Ctrl Pts',(162.804031095543,-225.995852143483,15.5582707927156));
#85153=CARTESIAN_POINT('Ctrl Pts',(160.684270860431,-227.89587383462,15.3995129274839));
#85154=CARTESIAN_POINT('Ctrl Pts',(157.938265960758,-227.145591906187,15.2407550622521));
#85155=CARTESIAN_POINT('Ctrl Pts',(157.079159972725,-224.431664349587,15.0819971970203));
#85156=CARTESIAN_POINT('Ctrl Pts',(158.893206662794,-222.237877557895,14.9232393317885));
#85157=CARTESIAN_POINT('Ctrl Pts',(161.720190571551,-222.5719851166,14.7644814665567));
#85158=CARTESIAN_POINT('Ctrl Pts',(162.972856136869,-225.128211801113,14.6057236013249));
#85159=CARTESIAN_POINT('Ctrl Pts',(161.504763882629,-227.567099050289,14.4469657360931));
#85160=CARTESIAN_POINT('Ctrl Pts',(158.659511782181,-227.65657734959,14.2882078708613));
#85161=CARTESIAN_POINT('Ctrl Pts',(157.041074445967,-225.314756163012,14.1294500056295));
#85162=CARTESIAN_POINT('Ctrl Pts',(158.130645660447,-222.684870148424,13.9706921403977));
#85163=CARTESIAN_POINT('Ctrl Pts',(160.931049892975,-222.173790882957,13.8119342751659));
#85164=CARTESIAN_POINT('Ctrl Pts',(162.879357300065,-224.24925809027,13.6531764099341));
#85165=CARTESIAN_POINT('Ctrl Pts',(162.192477019363,-227.011804263845,13.4944185447023));
#85166=CARTESIAN_POINT('Ctrl Pts',(159.499041856757,-227.933147254261,13.3356606794706));
#85167=CARTESIAN_POINT('Ctrl Pts',(157.264083567147,-226.170073992921,13.1769028142388));
#85168=CARTESIAN_POINT('Ctrl Pts',(157.533035889297,-223.336149059271,13.018144949007));
#85169=CARTESIAN_POINT('Ctrl Pts',(160.059753668551,-222.024980441147,12.8593870837752));
#85170=CARTESIAN_POINT('Ctrl Pts',(162.531784892697,-223.436549606296,12.7006292185434));
#85171=CARTESIAN_POINT('Ctrl Pts',(162.686726682607,-226.278988510281,12.5418713533116));
#85172=CARTESIAN_POINT('Ctrl Pts',(160.382776318248,-227.950897179953,12.3831134880798));
#85173=CARTESIAN_POINT('Ctrl Pts',(157.728509082481,-226.922144866572,12.224355622848));
#85174=CARTESIAN_POINT('Ctrl Pts',(157.153110245103,-224.134245646892,12.0655977576162));
#85175=CARTESIAN_POINT('Ctrl Pts',(159.183184799456,-222.138684777131,11.9068398923844));
#85176=CARTESIAN_POINT('Ctrl Pts',(161.960808593226,-222.761799486821,11.7480820271526));
#85177=CARTESIAN_POINT('Ctrl Pts',(162.943900439583,-225.433315218158,11.5893241619209));
#85178=CARTESIAN_POINT('Ctrl Pts',(161.232734719399,-227.708260878876,11.4305662966891));
#85179=CARTESIAN_POINT('Ctrl Pts',(158.393370232498,-227.504606289747,11.2718084314573));
#85180=CARTESIAN_POINT('Ctrl Pts',(157.024393245635,-225.008736122732,11.1130505662255));
#85181=CARTESIAN_POINT('Ctrl Pts',(158.378691443354,-222.504870656537,10.9542927009937));
#85182=CARTESIAN_POINT('Ctrl Pts',(161.216811168359,-222.28454746736,10.7955348357619));
#85183=CARTESIAN_POINT('Ctrl Pts',(162.941305359932,-224.549406329273,10.6367769705301));
#85184=CARTESIAN_POINT('Ctrl Pts',(161.973917001759,-227.226648500916,10.4780191052983));
#85185=CARTESIAN_POINT('Ctrl Pts',(159.199999881199,-227.866062052082,10.3192612400665));
#85186=CARTESIAN_POINT('Ctrl Pts',(157.158242837906,-225.882455725887,10.1605033748347));
#85187=CARTESIAN_POINT('Ctrl Pts',(157.717261837613,-223.091225954063,10.0017455096029));
#85188=CARTESIAN_POINT('Ctrl Pts',(160.36544271377,-222.046906114019,9.84298764437113));
#85189=CARTESIAN_POINT('Ctrl Pts',(162.679170432655,-223.705257682298,9.68422977913934));
#85190=CARTESIAN_POINT('Ctrl Pts',(162.540921476931,-226.548557368823,9.52547191390755));
#85191=CARTESIAN_POINT('Ctrl Pts',(160.077221285438,-227.974617412297,9.36671404867575));
#85192=CARTESIAN_POINT('Ctrl Pts',(157.54284817655,-226.678307717011,9.20795618344396));
#85193=CARTESIAN_POINT('Ctrl Pts',(157.257260319857,-223.846010865114,9.04919831821217));
#85194=CARTESIAN_POINT('Ctrl Pts',(159.481827710576,-222.069844824086,8.89044045298037));
#85195=CARTESIAN_POINT('Ctrl Pts',(162.180626360199,-222.975356684828,8.73168258774859));
#85196=CARTESIAN_POINT('Ctrl Pts',(162.883715850719,-225.733822027999,8.57292472251678));
#85197=CARTESIAN_POINT('Ctrl Pts',(160.94762870806,-227.820693480001,8.414166857285));
#85198=CARTESIAN_POINT('Ctrl Pts',(158.144271809049,-227.326066370028,8.2554089920532));
#85199=CARTESIAN_POINT('Ctrl Pts',(157.039277277422,-224.702623409675,8.09665112682141));
#85200=CARTESIAN_POINT('Ctrl Pts',(158.64393606507,-222.351339493094,7.93789326158962));
#85201=CARTESIAN_POINT('Ctrl Pts',(161.48966451264,-222.424109568277,7.77913539635783));
#85202=CARTESIAN_POINT('Ctrl Pts',(162.972052056822,-224.854334465279,7.62037753112604));
#85203=CARTESIAN_POINT('Ctrl Pts',(161.734417675473,-227.417872453929,7.46161966589424));
#85204=CARTESIAN_POINT('Ctrl Pts',(158.909444305736,-227.768573667824,7.30286180066245));
#85205=CARTESIAN_POINT('Ctrl Pts',(157.082547464504,-225.585476369798,7.14410393543066));
#85206=CARTESIAN_POINT('Ctrl Pts',(157.925703069032,-222.866551121156,6.98534607019886));
#85207=CARTESIAN_POINT('Ctrl Pts',(160.667255143213,-222.100158202536,6.82658820496708));
#85208=CARTESIAN_POINT('Ctrl Pts',(162.798135336563,-223.987700382922,6.66783033973528));
#85209=CARTESIAN_POINT('Ctrl Pts',(162.368162179926,-226.80169913305,6.50907247450349));
#85210=CARTESIAN_POINT('Ctrl Pts',(159.770847089346,-227.966782907461,6.3503146092717));
#85211=CARTESIAN_POINT('Ctrl Pts',(157.383252733585,-226.41666708163,6.19155674403991));
#85212=CARTESIAN_POINT('Ctrl Pts',(157.390505373146,-223.5700175984,6.03279887880811));
#85213=CARTESIAN_POINT('Ctrl Pts',(159.785967392588,-222.032087952882,5.87404101357632));
#85214=CARTESIAN_POINT('Ctrl Pts',(162.377312045917,-223.210391296176,5.71528314834452));
#85215=CARTESIAN_POINT('Ctrl Pts',(162.792940808308,-226.026544454835,5.55652528311274));
#85216=CARTESIAN_POINT('Ctrl Pts',(160.652470252765,-227.903204168797,5.39776741788094));
#85217=CARTESIAN_POINT('Ctrl Pts',(157.91485894755,-227.122851541641,5.23900955264915));
#85218=CARTESIAN_POINT('Ctrl Pts',(157.085568651541,-224.399665267055,5.08025168741735));
#85219=CARTESIAN_POINT('Ctrl Pts',(158.923565811034,-222.225905316451,4.92149382218556));
#85220=CARTESIAN_POINT('Ctrl Pts',(161.746715497939,-222.590996711146,4.76273595695377));
#85221=CARTESIAN_POINT('Ctrl Pts',(162.971271229819,-225.16080782106,4.60397809172198));
#85222=CARTESIAN_POINT('Ctrl Pts',(161.476519649008,-227.58344761948,4.44522022649019));
#85223=CARTESIAN_POINT('Ctrl Pts',(158.630457343494,-227.64171625811,4.28646236125839));
#85224=CARTESIAN_POINT('Ctrl Pts',(157.037800423344,-225.282286281269,4.1277044960266));
#85225=CARTESIAN_POINT('Ctrl Pts',(158.156148439294,-222.66450791077,3.96894663079481));
#85226=CARTESIAN_POINT('Ctrl Pts',(160.961989331031,-222.184171808785,3.81018876556301));
#85227=CARTESIAN_POINT('Ctrl Pts',(162.887417624971,-224.280881556065,3.65143090033122));
#85228=CARTESIAN_POINT('Ctrl Pts',(162.170281421805,-227.035728476212,3.49267303509943));
#85229=CARTESIAN_POINT('Ctrl Pts',(159.466903747323,-227.927476772375,3.33391516986764));
#85230=CARTESIAN_POINT('Ctrl Pts',(157.251415741134,-226.139998446992,3.17515730463585));
#85231=CARTESIAN_POINT('Ctrl Pts',(157.55143194305,-223.309193576523,3.01639943940405));
#85232=CARTESIAN_POINT('Ctrl Pts',(160.09237752926,-222.025814701629,2.85764157417226));
#85233=CARTESIAN_POINT('Ctrl Pts',(162.548779214987,-223.464410046505,2.69888370894047));
#85234=CARTESIAN_POINT('Ctrl Pts',(162.672538241262,-226.308377356738,2.54012584370868));
#85235=CARTESIAN_POINT('Ctrl Pts',(160.350390420134,-227.954917553418,2.38136797847688));
#85236=CARTESIAN_POINT('Ctrl Pts',(157.70756520503,-226.897117753222,2.22261011324509));
#85237=CARTESIAN_POINT('Ctrl Pts',(157.162776421762,-224.103074963931,2.0638522480133));
#85238=CARTESIAN_POINT('Ctrl Pts',(159.214614135679,-222.129899791342,1.90509438278151));
#85239=CARTESIAN_POINT('Ctrl Pts',(161.985237812524,-222.783436359779,1.74633651754971));
#85240=CARTESIAN_POINT('Ctrl Pts',(162.93897015616,-225.465579887444,1.58757865231792));
#85241=CARTESIAN_POINT('Ctrl Pts',(161.202960791094,-227.721608115667,1.42882078708613));
#85242=CARTESIAN_POINT('Ctrl Pts',(158.365994157881,-227.4868551559,1.27006292185433));
#85243=CARTESIAN_POINT('Ctrl Pts',(157.024485374886,-224.976060971526,1.11130505662254));
#85244=CARTESIAN_POINT('Ctrl Pts',(158.406134744506,-222.487324103837,0.952547191390749));
#85245=CARTESIAN_POINT('Ctrl Pts',(161.246557418698,-222.29788038346,0.793789326158957));
#85246=CARTESIAN_POINT('Ctrl Pts',(162.945990021977,-224.582055024746,0.635031460927165));
#85247=CARTESIAN_POINT('Ctrl Pts',(161.949545639495,-227.247408636808,0.47627359569537));
#85248=CARTESIAN_POINT('Ctrl Pts',(159.168282701031,-227.85869812666,0.317515730463582));
#85249=CARTESIAN_POINT('Ctrl Pts',(157.149564424984,-225.848042905619,0.158757865231786));
#85250=CARTESIAN_POINT('Ctrl Pts',(157.542565484547,-224.000243484621,0.0529192884105924));
#85251=CARTESIAN_POINT('Ctrl Pts',(158.086534003335,-223.364012796625,-4.44089209850063E-15));
#85252=CARTESIAN_POINT('Ctrl Pts',(158.086534003335,-223.364012796625,-4.44089209850063E-15));
#85253=CARTESIAN_POINT('Ctrl Pts',(158.024938131872,-223.421897790789,-4.02047441971943E-15));
#85254=CARTESIAN_POINT('Ctrl Pts',(157.966714212982,-223.482934468891,-1.25170609456878E-15));
#85255=CARTESIAN_POINT('Ctrl Pts',(157.911858615954,-223.546737772691,-1.38777878078145E-15));
#85256=CARTESIAN_POINT('Ctrl Pts',(157.855548999771,-223.612232266285,-1.52745825104056E-15));
#85257=CARTESIAN_POINT('Ctrl Pts',(157.802788200628,-223.680642427049,-1.1358963542259E-14));
#85258=CARTESIAN_POINT('Ctrl Pts',(157.753597853786,-223.751600310779,-1.22124532708767E-14));
#85259=CARTESIAN_POINT('Ctrl Pts',(157.702709598817,-223.825007454886,-1.30954029899182E-14));
#85260=CARTESIAN_POINT('Ctrl Pts',(157.655641951551,-223.90114175895,-2.81027041762154E-15));
#85261=CARTESIAN_POINT('Ctrl Pts',(157.612453799623,-223.979639850734,-1.49880108324396E-15));
#85262=CARTESIAN_POINT('Ctrl Pts',(157.593558983155,-224.013982765889,-9.25033249453769E-16));
#85263=CARTESIAN_POINT('Ctrl Pts',(157.575407220319,-224.048778631187,-8.43275911610205E-15));
#85264=CARTESIAN_POINT('Ctrl Pts',(157.55800588697,-224.083999106998,-8.38218383591993E-15));
#85265=CARTESIAN_POINT('Ctrl Pts',(157.548477933598,-224.103283781599,-8.35449176763588E-15));
#85266=CARTESIAN_POINT('Ctrl Pts',(157.539174987618,-224.122695774927,-8.94435754255875E-16));
#85267=CARTESIAN_POINT('Ctrl Pts',(157.530098465041,-224.142230564629,-3.88578058618805E-16));
#85268=CARTESIAN_POINT('Ctrl Pts',(157.521442320672,-224.16086060256,9.38508900182872E-17));
#85269=CARTESIAN_POINT('Ctrl Pts',(157.512989615474,-224.179608342932,-5.5821178937832E-15));
#85270=CARTESIAN_POINT('Ctrl Pts',(157.504755700859,-224.198437010398,-5.49560397189452E-15));
#85271=CARTESIAN_POINT('Ctrl Pts',(157.468216216528,-224.281992625442,-5.11168280667383E-15));
#85272=CARTESIAN_POINT('Ctrl Pts',(157.435936147707,-224.367231893099,-3.02367079316581E-15));
#85273=CARTESIAN_POINT('Ctrl Pts',(157.407939191047,-224.453755565247,-3.69149155687865E-15));
#85274=CARTESIAN_POINT('Ctrl Pts',(157.379477689978,-224.541714896589,-4.37039325364763E-15));
#85275=CARTESIAN_POINT('Ctrl Pts',(157.355442125594,-224.631002365215,-7.11283600949192E-15));
#85276=CARTESIAN_POINT('Ctrl Pts',(157.33589650728,-224.721235656857,-7.35522753814166E-15));
#85277=CARTESIAN_POINT('Ctrl Pts',(157.31669447316,-224.809882775465,-7.59335816818749E-15));
#85278=CARTESIAN_POINT('Ctrl Pts',(157.301825663592,-224.899443667177,-6.01491689603108E-15));
#85279=CARTESIAN_POINT('Ctrl Pts',(157.291393417184,-224.989578650944,-6.13398221105399E-15));
#85280=CARTESIAN_POINT('Ctrl Pts',(157.287259487947,-225.025295948072,-6.18116357234791E-15));
#85281=CARTESIAN_POINT('Ctrl Pts',(157.28382270983,-225.061103573716,-5.15113929225242E-15));
#85282=CARTESIAN_POINT('Ctrl Pts',(157.281091552527,-225.096980929019,-5.6621374255883E-15));
#85283=CARTESIAN_POINT('Ctrl Pts',(157.279473342812,-225.118238249062,-5.96490363479611E-15));
#85284=CARTESIAN_POINT('Ctrl Pts',(157.278102868135,-225.139520052234,-6.46012964232343E-15));
#85285=CARTESIAN_POINT('Ctrl Pts',(157.276982094653,-225.160822076977,-6.60582699651968E-15));
#85286=CARTESIAN_POINT('Ctrl Pts',(157.276240093157,-225.174924957255,-6.7022850735275E-15));
#85287=CARTESIAN_POINT('Ctrl Pts',(157.27560761903,-225.18903661353,-1.04645236124941E-14));
#85288=CARTESIAN_POINT('Ctrl Pts',(157.275085584502,-225.203141411304,-1.02418074021671E-14));
#85289=CARTESIAN_POINT('Ctrl Pts',(157.271562563848,-225.298329547766,-8.73877691854704E-15));
#85290=CARTESIAN_POINT('Ctrl Pts',(157.273056291674,-225.393366882897,-1.25249371125912E-14));
#85291=CARTESIAN_POINT('Ctrl Pts',(157.279624839535,-225.487854119313,-1.19904086659517E-14));
#85292=CARTESIAN_POINT('Ctrl Pts',(157.286171652655,-225.582028705859,-1.14576489264445E-14));
#85293=CARTESIAN_POINT('Ctrl Pts',(157.297759397958,-225.675657782649,-1.02581785354216E-14));
#85294=CARTESIAN_POINT('Ctrl Pts',(157.314493581616,-225.768363904367,-1.11854969730985E-14));
#85295=CARTESIAN_POINT('Ctrl Pts',(157.316397869106,-225.778913514163,-1.12910223417952E-14));
#85296=CARTESIAN_POINT('Ctrl Pts',(157.318368855583,-225.789451182139,-9.70347588764154E-15));
#85297=CARTESIAN_POINT('Ctrl Pts',(157.320406739366,-225.799976358203,-9.93649607039515E-15));
#85298=CARTESIAN_POINT('Ctrl Pts',(157.337939942263,-225.890531103766,-1.1971137394992E-14));
#85299=CARTESIAN_POINT('Ctrl Pts',(157.36042066591,-225.980161474788,-5.38012735527091E-15));
#85300=CARTESIAN_POINT('Ctrl Pts',(157.387574007674,-226.068629871038,-4.8017145815038E-15));
#85301=CARTESIAN_POINT('Ctrl Pts',(157.398274256088,-226.103492387221,-4.57378092902809E-15));
#85302=CARTESIAN_POINT('Ctrl Pts',(157.409700687624,-226.138174410619,-6.81791231009982E-15));
#85303=CARTESIAN_POINT('Ctrl Pts',(157.421838645824,-226.172661063201,-7.04991620636974E-15));
#85304=CARTESIAN_POINT('Ctrl Pts',(157.42714896822,-226.187748876204,-7.15141725505753E-15));
#85305=CARTESIAN_POINT('Ctrl Pts',(157.432595494617,-226.20279929086,-9.33337609025355E-15));
#85306=CARTESIAN_POINT('Ctrl Pts',(157.438177066941,-226.217811042138,-9.29811783123569E-15));
#85307=CARTESIAN_POINT('Ctrl Pts',(157.44259780243,-226.229700699347,-9.27019246758084E-15));
#85308=CARTESIAN_POINT('Ctrl Pts',(157.447102851067,-226.241564891189,-9.32321973403198E-15));
#85309=CARTESIAN_POINT('Ctrl Pts',(157.451687905131,-226.253393829545,-9.43689570931383E-15));
#85310=CARTESIAN_POINT('Ctrl Pts',(157.485446240419,-226.34048664493,-1.02738567645768E-14));
#85311=CARTESIAN_POINT('Ctrl Pts',(157.523587548176,-226.425804632643,-1.06218398729921E-14));
#85312=CARTESIAN_POINT('Ctrl Pts',(157.565778560797,-226.509117057952,-9.78384040450919E-15));
#85313=CARTESIAN_POINT('Ctrl Pts',(157.609551906108,-226.595554034339,-8.91441258505656E-15));
#85314=CARTESIAN_POINT('Ctrl Pts',(157.657684534616,-226.679832913129,-6.08329446841785E-15));
#85315=CARTESIAN_POINT('Ctrl Pts',(157.709860342191,-226.761692981327,-5.20417042793042E-15));
#85316=CARTESIAN_POINT('Ctrl Pts',(157.762637853889,-226.844497079773,-4.31490811485777E-15));
#85317=CARTESIAN_POINT('Ctrl Pts',(157.819552746941,-226.924827072195,-8.96093847127932E-15));
#85318=CARTESIAN_POINT('Ctrl Pts',(157.880329760087,-227.002398324715,-7.64666108210577E-15));
#85319=CARTESIAN_POINT('Ctrl Pts',(157.92312880423,-227.057023836714,-6.7211497237137E-15));
#85320=CARTESIAN_POINT('Ctrl Pts',(157.967844154052,-227.110281017477,-8.49846093585579E-15));
#85321=CARTESIAN_POINT('Ctrl Pts',(158.014393105504,-227.162062750717,-9.13158437754191E-15));
#85322=CARTESIAN_POINT('Ctrl Pts',(158.02559966715,-227.174529093515,-9.28400750754482E-15));
#85323=CARTESIAN_POINT('Ctrl Pts',(158.036913147564,-227.186910416437,-1.3469166115988E-14));
#85324=CARTESIAN_POINT('Ctrl Pts',(158.048321150992,-227.199193291615,-1.33087985076941E-14));
#85325=CARTESIAN_POINT('Ctrl Pts',(158.116987457225,-227.273125568526,-1.23435243147714E-14));
#85326=CARTESIAN_POINT('Ctrl Pts',(158.189166708083,-227.343596762759,-3.71230618695111E-15));
#85327=CARTESIAN_POINT('Ctrl Pts',(158.264545772445,-227.410319899525,-7.56339435525888E-15));
#85328=CARTESIAN_POINT('Ctrl Pts',(158.329365760519,-227.467696479694,-1.08750232704468E-14));
#85329=CARTESIAN_POINT('Ctrl Pts',(158.3965529381,-227.522301582086,-9.56933057703736E-15));
#85330=CARTESIAN_POINT('Ctrl Pts',(158.465934417848,-227.573937429872,-6.84868828315643E-15));
#85331=CARTESIAN_POINT('Ctrl Pts',(158.491454071548,-227.592929947167,-5.84799113118415E-15));
#85332=CARTESIAN_POINT('Ctrl Pts',(158.517270804806,-227.611520587321,-1.17738964924128E-14));
#85333=CARTESIAN_POINT('Ctrl Pts',(158.543376723496,-227.629698856678,-1.18516307878735E-14));
#85334=CARTESIAN_POINT('Ctrl Pts',(158.560069303013,-227.641322359009,-1.19013354515399E-14));
#85335=CARTESIAN_POINT('Ctrl Pts',(158.57688116617,-227.652777833288,-1.23844299269826E-14));
#85336=CARTESIAN_POINT('Ctrl Pts',(158.593795463636,-227.664052888908,-1.19002030452009E-14));
#85337=CARTESIAN_POINT('Ctrl Pts',(158.679989147357,-227.721509521675,-9.43262797853806E-15));
#85338=CARTESIAN_POINT('Ctrl Pts',(158.768924488191,-227.774344032196,-5.88836659555711E-15));
#85339=CARTESIAN_POINT('Ctrl Pts',(158.86029512281,-227.822237061513,-2.13370987545147E-15));
#85340=CARTESIAN_POINT('Ctrl Pts',(158.951665757429,-227.870130090831,1.62094684465417E-15));
#85341=CARTESIAN_POINT('Ctrl Pts',(159.045472324464,-227.913082541088,-5.46458148948038E-15));
#85342=CARTESIAN_POINT('Ctrl Pts',(159.141446274327,-227.95073460326,-7.40379979546901E-15));
#85343=CARTESIAN_POINT('Ctrl Pts',(159.162330716372,-227.958927892287,-7.86016396636461E-15));
#85344=CARTESIAN_POINT('Ctrl Pts',(159.183317909858,-227.966870015372,8.49377045481285E-16));
#85345=CARTESIAN_POINT('Ctrl Pts',(159.204403760484,-227.974562200359,8.32667268468867E-16));
#85346=CARTESIAN_POINT('Ctrl Pts',(157.485690666959,-224.998572567547,19.112583302492));
#85347=CARTESIAN_POINT('Ctrl Pts',(157.484001293575,-224.6725707558,19.092036810933));
#85348=CARTESIAN_POINT('Ctrl Pts',(157.542838236001,-224.347153873571,19.071490319374));
#85349=CARTESIAN_POINT('Ctrl Pts',(157.665030280249,-224.047579988685,19.0509438278151));
#85350=CARTESIAN_POINT('Ctrl Pts',(157.979746591422,-223.276001212375,18.9980245394045));
#85351=CARTESIAN_POINT('Ctrl Pts',(158.714738560392,-222.675855870717,18.9451052509939));
#85352=CARTESIAN_POINT('Ctrl Pts',(159.533660666009,-222.521758115913,18.8921859625833));
#85353=CARTESIAN_POINT('Ctrl Pts',(160.352582771625,-222.367660361109,18.8392666741727));
#85354=CARTESIAN_POINT('Ctrl Pts',(161.255435013888,-222.659610193158,18.7863473857621));
#85355=CARTESIAN_POINT('Ctrl Pts',(161.829078591495,-223.264017324161,18.7334280973515));
#85356=CARTESIAN_POINT('Ctrl Pts',(162.402722169101,-223.868424455164,18.6805088089409));
#85357=CARTESIAN_POINT('Ctrl Pts',(162.647157082051,-224.785288885121,18.6275895205303));
#85358=CARTESIAN_POINT('Ctrl Pts',(162.450526850331,-225.595050601476,18.5746702321197));
#85359=CARTESIAN_POINT('Ctrl Pts',(162.253896618611,-226.404812317831,18.5217509437091));
#85360=CARTESIAN_POINT('Ctrl Pts',(161.616201242222,-227.107471320585,18.4688316552985));
#85361=CARTESIAN_POINT('Ctrl Pts',(160.829251591834,-227.381492245887,18.4159123668879));
#85362=CARTESIAN_POINT('Ctrl Pts',(160.042301941446,-227.655513171189,18.3629930784773));
#85363=CARTESIAN_POINT('Ctrl Pts',(159.10609801706,-227.500896019039,18.3100737900667));
#85364=CARTESIAN_POINT('Ctrl Pts',(158.449046003258,-226.988392929152,18.2571545016561));
#85365=CARTESIAN_POINT('Ctrl Pts',(157.850708419101,-226.521687319499,18.2089641019347));
#85366=CARTESIAN_POINT('Ctrl Pts',(157.483861600094,-225.758199612281,18.1607737022134));
#85367=CARTESIAN_POINT('Ctrl Pts',(157.479093605947,-224.998703157778,18.112583302492));
#85368=CARTESIAN_POINT('Origin',(-160.,-225.,22.2084234471774));
#85369=CARTESIAN_POINT('Ctrl Pts',(-163.076377950168,-224.997773694264,
19.7084234471775));
#85370=CARTESIAN_POINT('Ctrl Pts',(-163.077562842917,-224.85366922826,19.7009407276991));
#85371=CARTESIAN_POINT('Ctrl Pts',(-163.002826982104,-223.691638940026,
19.6405387198101));
#85372=CARTESIAN_POINT('Ctrl Pts',(-161.521864797362,-221.70110626648,19.5272174235105));
#85373=CARTESIAN_POINT('Ctrl Pts',(-158.054123026994,-221.932389233715,
19.3684595582787));
#85374=CARTESIAN_POINT('Ctrl Pts',(-156.367330739964,-224.970773973196,
19.2097016930469));
#85375=CARTESIAN_POINT('Ctrl Pts',(-158.005117242933,-228.036087327305,
19.0509438278151));
#85376=CARTESIAN_POINT('Ctrl Pts',(-161.468639631394,-228.322686472282,
18.8921859625833));
#85377=CARTESIAN_POINT('Ctrl Pts',(-162.992852930873,-226.341897473527,
18.7780125023707));
#85378=CARTESIAN_POINT('Ctrl Pts',(-163.077320562719,-225.163035204797,
18.7167583305688));
#85379=CARTESIAN_POINT('Ctrl Pts',(-163.075931333395,-225.0024275328,18.7084234471774));
#85380=CARTESIAN_POINT('Ctrl Pts',(-163.070362267144,-225.003024949566,
19.7915765528225));
#85381=CARTESIAN_POINT('Ctrl Pts',(-163.065080691912,-224.299688720016,
19.7552124583938));
#85382=CARTESIAN_POINT('Ctrl Pts',(-162.477826131062,-222.562575755896,
19.6659290755545));
#85383=CARTESIAN_POINT('Ctrl Pts',(-159.592724505823,-221.390669564417,
19.5237264043046));
#85384=CARTESIAN_POINT('Ctrl Pts',(-156.746988377721,-223.383220985595,
19.3649685390728));
#85385=CARTESIAN_POINT('Ctrl Pts',(-156.877197897433,-226.856577363582,
19.206210673841));
#85386=CARTESIAN_POINT('Ctrl Pts',(-159.865978935642,-228.630249528,19.0474528086092));
#85387=CARTESIAN_POINT('Ctrl Pts',(-162.574488231656,-227.282183302953,
18.9092414349364));
#85388=CARTESIAN_POINT('Ctrl Pts',(-163.066355304625,-225.625342192633,
18.8239493496742));
#85389=CARTESIAN_POINT('Ctrl Pts',(-163.069604917803,-224.99825730896,18.7915765528225));
#85390=CARTESIAN_POINT('Ctrl Pts',(-158.086534003335,-223.364012796625,
20.));
#85391=CARTESIAN_POINT('Ctrl Pts',(-157.542565484547,-224.000243484621,
19.9470807115894));
#85392=CARTESIAN_POINT('Ctrl Pts',(-157.14956575156,-225.848044358444,19.8412421347682));
#85393=CARTESIAN_POINT('Ctrl Pts',(-159.168282289031,-227.858697938457,
19.6824842695364));
#85394=CARTESIAN_POINT('Ctrl Pts',(-161.949545980211,-227.24740909585,19.5237264043046));
#85395=CARTESIAN_POINT('Ctrl Pts',(-162.945990159525,-224.582054828932,
19.3649685390728));
#85396=CARTESIAN_POINT('Ctrl Pts',(-161.246557549164,-222.297880275211,
19.206210673841));
#85397=CARTESIAN_POINT('Ctrl Pts',(-158.406134608902,-222.487323863959,
19.0474528086093));
#85398=CARTESIAN_POINT('Ctrl Pts',(-157.024485159544,-224.976060998054,
18.8886949433774));
#85399=CARTESIAN_POINT('Ctrl Pts',(-158.365994032564,-227.486855326661,
18.7299370781457));
#85400=CARTESIAN_POINT('Ctrl Pts',(-161.202960882393,-227.721608327304,
18.5711792129139));
#85401=CARTESIAN_POINT('Ctrl Pts',(-162.938970375395,-225.465579917995,
18.4124213476821));
#85402=CARTESIAN_POINT('Ctrl Pts',(-161.985237961226,-222.783436196243,
18.2536634824503));
#85403=CARTESIAN_POINT('Ctrl Pts',(-159.21461407685,-222.129899575534,18.0949056172185));
#85404=CARTESIAN_POINT('Ctrl Pts',(-157.16277620961,-224.103074897453,17.9361477519867));
#85405=CARTESIAN_POINT('Ctrl Pts',(-157.707565033574,-226.897117894792,
17.7773898867549));
#85406=CARTESIAN_POINT('Ctrl Pts',(-160.350390446343,-227.954917774566,
17.6186320215231));
#85407=CARTESIAN_POINT('Ctrl Pts',(-162.672538441131,-226.308377454507,
17.4598741562913));
#85408=CARTESIAN_POINT('Ctrl Pts',(-162.548779405603,-223.464409931704,
17.3011162910595));
#85409=CARTESIAN_POINT('Ctrl Pts',(-160.092377536169,-222.025814479178,
17.1423584258277));
#85410=CARTESIAN_POINT('Ctrl Pts',(-157.551431759929,-223.309193450083,
16.9836005605959));
#85411=CARTESIAN_POINT('Ctrl Pts',(-157.251415535576,-226.139998532244,
16.8248426953642));
#85412=CARTESIAN_POINT('Ctrl Pts',(-159.466903707454,-227.927476991314,
16.6660848301324));
#85413=CARTESIAN_POINT('Ctrl Pts',(-162.170281584114,-227.035728628457,
16.5073269649006));
#85414=CARTESIAN_POINT('Ctrl Pts',(-162.887417840912,-224.280881502285,
16.3485690996688));
#85415=CARTESIAN_POINT('Ctrl Pts',(-160.961989402975,-222.184171598198,
16.189811234437));
#85416=CARTESIAN_POINT('Ctrl Pts',(-158.156148301398,-222.664507736106,
16.0310533692052));
#85417=CARTESIAN_POINT('Ctrl Pts',(-157.03780020181,-225.28228630238,15.8722955039734));
#85418=CARTESIAN_POINT('Ctrl Pts',(-158.63045724107,-227.641716455676,15.7135376387416));
#85419=CARTESIAN_POINT('Ctrl Pts',(-161.476519759432,-227.583447812688,
15.5547797735098));
#85420=CARTESIAN_POINT('Ctrl Pts',(-162.971271452032,-225.160807833087,
15.396021908278));
#85421=CARTESIAN_POINT('Ctrl Pts',(-161.746715628571,-222.590996530984,
15.2372640430462));
#85422=CARTESIAN_POINT('Ctrl Pts',(-158.923565730531,-222.225905108985,
15.0785061778144));
#85423=CARTESIAN_POINT('Ctrl Pts',(-157.085568433579,-224.399665222158,
14.9197483125826));
#85424=CARTESIAN_POINT('Ctrl Pts',(-157.914858791609,-227.122851700403,
14.7609904473509));
#85425=CARTESIAN_POINT('Ctrl Pts',(-160.652470301561,-227.903204385919,
14.6022325821191));
#85426=CARTESIAN_POINT('Ctrl Pts',(-162.792941017183,-226.026544531607,
14.4434747168873));
#85427=CARTESIAN_POINT('Ctrl Pts',(-162.377312223709,-223.210391162337,
14.2847168516555));
#85428=CARTESIAN_POINT('Ctrl Pts',(-159.785967376581,-222.032087730921,
14.1259589864237));
#85429=CARTESIAN_POINT('Ctrl Pts',(-157.39050517799,-223.570017491456,13.9672011211919));
#85430=CARTESIAN_POINT('Ctrl Pts',(-157.383252537887,-226.416667187578,
13.8084432559601));
#85431=CARTESIAN_POINT('Ctrl Pts',(-159.770847072208,-227.966783129337,
13.6496853907283));
#85432=CARTESIAN_POINT('Ctrl Pts',(-162.368162357033,-226.801699267793,
13.4909275254965));
#85433=CARTESIAN_POINT('Ctrl Pts',(-162.798135545827,-223.987700307215,
13.3321696602647));
#85434=CARTESIAN_POINT('Ctrl Pts',(-160.667255193115,-222.100157985666,
13.1734117950329));
#85435=CARTESIAN_POINT('Ctrl Pts',(-157.925702913902,-222.866550961602,
13.0146539298011));
#85436=CARTESIAN_POINT('Ctrl Pts',(-157.082547246317,-225.585476413584,
12.8558960645693));
#85437=CARTESIAN_POINT('Ctrl Pts',(-158.909444224176,-227.768573874878,
12.6971381993376));
#85438=CARTESIAN_POINT('Ctrl Pts',(-161.734417805185,-227.417872634754,
12.5383803341058));
#85439=CARTESIAN_POINT('Ctrl Pts',(-162.972052279092,-224.854334454385,
12.379622468874));
#85440=CARTESIAN_POINT('Ctrl Pts',(-161.489664624048,-222.424109375634,
12.2208646036422));
#85441=CARTESIAN_POINT('Ctrl Pts',(-158.643935963655,-222.351339295008,
12.0621067384104));
#85442=CARTESIAN_POINT('Ctrl Pts',(-157.039277055999,-224.702623387435,
11.9033488731786));
#85443=CARTESIAN_POINT('Ctrl Pts',(-158.144271670265,-227.326066543987,
11.7445910079468));
#85444=CARTESIAN_POINT('Ctrl Pts',(-160.94762877893,-227.820693690952,11.585833142715));
#85445=CARTESIAN_POINT('Ctrl Pts',(-162.883716066383,-225.733822082879,
11.4270752774832));
#85446=CARTESIAN_POINT('Ctrl Pts',(-162.180626523281,-222.975356533412,
11.2683174122514));
#85447=CARTESIAN_POINT('Ctrl Pts',(-159.481827671824,-222.069844604949,
11.1095595470196));
#85448=CARTESIAN_POINT('Ctrl Pts',(-157.257260114736,-223.846010778811,
10.9508016817878));
#85449=CARTESIAN_POINT('Ctrl Pts',(-157.542847992787,-226.678307842526,
10.792043816556));
#85450=CARTESIAN_POINT('Ctrl Pts',(-160.077221291214,-227.974617634759,
10.6332859513242));
#85451=CARTESIAN_POINT('Ctrl Pts',(-162.540921666958,-226.548557484635,
10.4745280860925));
#85452=CARTESIAN_POINT('Ctrl Pts',(-162.679170633022,-223.705257585468,
10.3157702208607));
#85453=CARTESIAN_POINT('Ctrl Pts',(-160.3654427411,-222.046905893167,10.1570123556289));
#85454=CARTESIAN_POINT('Ctrl Pts',(-157.717261666894,-223.091225811312,
9.99825449039707));
#85455=CARTESIAN_POINT('Ctrl Pts',(-157.15824262538,-225.882455791883,9.83949662516529));
#85456=CARTESIAN_POINT('Ctrl Pts',(-159.199999821369,-227.866062266425,
9.68073875993349));
#85457=CARTESIAN_POINT('Ctrl Pts',(-161.973917149382,-227.22664866744,9.5219808947017));
#85458=CARTESIAN_POINT('Ctrl Pts',(-162.941305579903,-224.549406295574,
9.36322302946991));
#85459=CARTESIAN_POINT('Ctrl Pts',(-161.216811259361,-222.28454726428,9.20446516423811));
#85460=CARTESIAN_POINT('Ctrl Pts',(-158.378691322102,-222.504870469934,
9.04570729900632));
#85461=CARTESIAN_POINT('Ctrl Pts',(-157.024393023099,-225.008736123386,
8.88694943377453));
#85462=CARTESIAN_POINT('Ctrl Pts',(-158.393370112343,-227.504606477058,
8.72819156854273));
#85463=CARTESIAN_POINT('Ctrl Pts',(-161.232734811591,-227.708261081419,
8.56943370331094));
#85464=CARTESIAN_POINT('Ctrl Pts',(-162.943900659748,-225.433315250564,
8.41067583807915));
#85465=CARTESIAN_POINT('Ctrl Pts',(-161.960808739869,-222.761799319433,
8.25191797284736));
#85466=CARTESIAN_POINT('Ctrl Pts',(-159.183184738369,-222.138684563142,
8.09316010761556));
#85467=CARTESIAN_POINT('Ctrl Pts',(-157.153110032193,-224.134245582145,
7.93440224238378));
#85468=CARTESIAN_POINT('Ctrl Pts',(-157.728508912603,-226.922145010324,
7.77564437715198));
#85469=CARTESIAN_POINT('Ctrl Pts',(-160.382776346874,-227.950897400641,
7.61688651192019));
#85470=CARTESIAN_POINT('Ctrl Pts',(-162.686726883539,-226.278988605933,
7.45812864668839));
#85471=CARTESIAN_POINT('Ctrl Pts',(-162.531785082041,-223.43654948937,7.2993707814566));
#85472=CARTESIAN_POINT('Ctrl Pts',(-160.05975367302,-222.024980218655,7.14061291622481));
#85473=CARTESIAN_POINT('Ctrl Pts',(-157.5330357048,-223.336148934837,6.98185505099302));
#85474=CARTESIAN_POINT('Ctrl Pts',(-157.264083362536,-226.170074080427,
6.82309718576123));
#85475=CARTESIAN_POINT('Ctrl Pts',(-159.499041819292,-227.933147473623,
6.66433932052943));
#85476=CARTESIAN_POINT('Ctrl Pts',(-162.192477183332,-227.011804414302,
6.50558145529764));
#85477=CARTESIAN_POINT('Ctrl Pts',(-162.879357515403,-224.249258034125,
6.34682359006585));
#85478=CARTESIAN_POINT('Ctrl Pts',(-160.931049962606,-222.173790671594,
6.18806572483405));
#85479=CARTESIAN_POINT('Ctrl Pts',(-158.130645520644,-222.684869975283,
6.02930785960226));
#85480=CARTESIAN_POINT('Ctrl Pts',(-157.041074224678,-225.314756186552,
5.87054999437047));
#85481=CARTESIAN_POINT('Ctrl Pts',(-158.65951168193,-227.656577548267,5.71179212913868));
#85482=CARTESIAN_POINT('Ctrl Pts',(-161.504763995166,-227.567099242275,
5.55303426390689));
#85483=CARTESIAN_POINT('Ctrl Pts',(-162.972856359199,-225.128211810702,
5.3942763986751));
#85484=CARTESIAN_POINT('Ctrl Pts',(-161.720190700198,-222.571984935017,
5.2355185334433));
#85485=CARTESIAN_POINT('Ctrl Pts',(-158.89320658002,-222.237877351324,5.07676066821151));
#85486=CARTESIAN_POINT('Ctrl Pts',(-157.079159754285,-224.431664307083,
4.91800280297972));
#85487=CARTESIAN_POINT('Ctrl Pts',(-157.938265806568,-227.145592066649,
4.75924493774793));
#85488=CARTESIAN_POINT('Ctrl Pts',(-160.684270911606,-227.895874051193,
4.60048707251613));
#85489=CARTESIAN_POINT('Ctrl Pts',(-162.804031305248,-225.99585221796,4.44172920728434));
#85490=CARTESIAN_POINT('Ctrl Pts',(-162.357542358599,-223.184426474016,
4.28297134205255));
#85491=CARTESIAN_POINT('Ctrl Pts',(-159.753430738056,-222.034613549646,
4.12421347682075));
#85492=CARTESIAN_POINT('Ctrl Pts',(-157.374979296373,-223.598722188052,
3.96545561158896));
#85493=CARTESIAN_POINT('Ctrl Pts',(-157.398946699372,-226.445280224801,
3.80669774635717));
#85494=CARTESIAN_POINT('Ctrl Pts',(-159.803397980927,-227.969117856745,
3.64793988112538));
#85495=CARTESIAN_POINT('Ctrl Pts',(-162.387779422388,-226.77561894275,3.48918201589358));
#85496=CARTESIAN_POINT('Ctrl Pts',(-162.786865230829,-223.957073642597,
3.3304241506618));
#85497=CARTESIAN_POINT('Ctrl Pts',(-160.635412088667,-222.093014502851,
3.17166628543));
#85498=CARTESIAN_POINT('Ctrl Pts',(-157.902429829893,-222.889428377601,
3.01290842019821));
#85499=CARTESIAN_POINT('Ctrl Pts',(-157.089143704272,-225.617437314398,
2.85415055496641));
#85500=CARTESIAN_POINT('Ctrl Pts',(-158.939873154425,-227.780367653174,
2.69539268973462));
#85501=CARTESIAN_POINT('Ctrl Pts',(-161.760830634549,-227.398705608841,
2.53663482450283));
#85502=CARTESIAN_POINT('Ctrl Pts',(-162.970276023305,-224.821748319362,
2.37787695927104));
#85503=CARTESIAN_POINT('Ctrl Pts',(-161.461324837368,-222.407926890985,
2.21911909403925));
#85504=CARTESIAN_POINT('Ctrl Pts',(-158.614969373296,-222.366370815315,
2.06036122880745));
#85505=CARTESIAN_POINT('Ctrl Pts',(-157.03619356153,-224.735111764472,1.90160336357566));
#85506=CARTESIAN_POINT('Ctrl Pts',(-158.169893955495,-227.346279041844,
1.74284549834387));
#85507=CARTESIAN_POINT('Ctrl Pts',(-160.978505939593,-227.810130534509,
1.58408763311208));
#85508=CARTESIAN_POINT('Ctrl Pts',(-162.89159221018,-225.702153365617,1.42532976788028));
#85509=CARTESIAN_POINT('Ctrl Pts',(-162.158287419518,-222.951559875847,
1.26657190264849));
#85510=CARTESIAN_POINT('Ctrl Pts',(-159.449730484722,-222.075710302932,
1.1078140374167));
#85511=CARTESIAN_POINT('Ctrl Pts',(-157.244754422452,-223.876146484295,
0.949056172184905));
#85512=CARTESIAN_POINT('Ctrl Pts',(-157.561432469829,-226.705183287036,
0.790298306953112));
#85513=CARTESIAN_POINT('Ctrl Pts',(-160.109776483231,-227.973532810194,
0.631540441721317));
#85514=CARTESIAN_POINT('Ctrl Pts',(-162.557883271515,-226.520720191152,
0.472782576489527));
#85515=CARTESIAN_POINT('Ctrl Pts',(-162.66453771979,-223.67569832521,0.314024711257735));
#85516=CARTESIAN_POINT('Ctrl Pts',(-160.333598844781,-222.043602025466,
0.15526684602594));
#85517=CARTESIAN_POINT('Ctrl Pts',(-157.695294647756,-223.115260895132,
-0.00349101920584827));
#85518=CARTESIAN_POINT('Ctrl Pts',(-157.170584060966,-225.915729262672,
-0.162248884437644));
#85519=CARTESIAN_POINT('Ctrl Pts',(-158.541127016969,-227.215894200354,
-0.268087461258838));
#85520=CARTESIAN_POINT('Ctrl Pts',(-159.349800002025,-227.432086802035,
-0.321006749669435));
#85521=CARTESIAN_POINT('Ctrl Pts',(-157.945668449658,-223.243574678773,
20.1070022498898));
#85522=CARTESIAN_POINT('Ctrl Pts',(-157.361654052493,-223.926643402192,
20.0540829614792));
#85523=CARTESIAN_POINT('Ctrl Pts',(-156.9397224623,-225.9104756942,19.948244384658));
#85524=CARTESIAN_POINT('Ctrl Pts',(-159.107052888527,-228.069149584109,
19.7894865194262));
#85525=CARTESIAN_POINT('Ctrl Pts',(-162.09306767038,-227.412858875035,19.6307286541944));
#85526=CARTESIAN_POINT('Ctrl Pts',(-163.162868084542,-224.551286538285,
19.4719707889626));
#85527=CARTESIAN_POINT('Ctrl Pts',(-161.338326631897,-222.098955605634,
19.3132129237308));
#85528=CARTESIAN_POINT('Ctrl Pts',(-158.288797414932,-222.302345653878,
19.1544550584991));
#85529=CARTESIAN_POINT('Ctrl Pts',(-156.805433686351,-224.974298656435,
18.9956971932672));
#85530=CARTESIAN_POINT('Ctrl Pts',(-158.245701769353,-227.669932660209,
18.8369393280355));
#85531=CARTESIAN_POINT('Ctrl Pts',(-161.291520465393,-227.921967708964,
18.6781814628037));
#85532=CARTESIAN_POINT('Ctrl Pts',(-163.155331517893,-225.499854983788,
18.5194235975719));
#85533=CARTESIAN_POINT('Ctrl Pts',(-162.131387223912,-222.620257185996,
18.3606657323401));
#85534=CARTESIAN_POINT('Ctrl Pts',(-159.15679553024,-221.918608501585,18.2019078671083));
#85535=CARTESIAN_POINT('Ctrl Pts',(-156.953905447948,-224.037045058722,
18.0431500018765));
#85536=CARTESIAN_POINT('Ctrl Pts',(-157.538800539521,-227.036779933787,
17.8843921366447));
#85537=CARTESIAN_POINT('Ctrl Pts',(-160.376185492774,-228.172452932812,
17.7256342714129));
#85538=CARTESIAN_POINT('Ctrl Pts',(-162.869285395553,-226.404697595481,
17.5668764061811));
#85539=CARTESIAN_POINT('Ctrl Pts',(-162.736415466445,-223.351362850873,
17.4081185409494));
#85540=CARTESIAN_POINT('Ctrl Pts',(-160.0991781863,-221.806860867848,17.2493606757175));
#85541=CARTESIAN_POINT('Ctrl Pts',(-157.3711730454,-223.184719641178,17.0906028104858));
#85542=CARTESIAN_POINT('Ctrl Pts',(-157.049070224458,-226.223922952493,
16.931844945254));
#85543=CARTESIAN_POINT('Ctrl Pts',(-159.427658220708,-228.14299201378,16.7730870800222));
#85544=CARTESIAN_POINT('Ctrl Pts',(-162.330053389578,-227.185594913451,
16.6143292147904));
#85545=CARTESIAN_POINT('Ctrl Pts',(-163.099983788551,-224.227941431483,
16.4555713495586));
#85546=CARTESIAN_POINT('Ctrl Pts',(-161.032809145849,-221.976875922408,
16.2968134843268));
#85547=CARTESIAN_POINT('Ctrl Pts',(-158.020407613623,-222.492573449615,
16.138055619095));
#85548=CARTESIAN_POINT('Ctrl Pts',(-156.819728955495,-225.303067657444,
15.9792977538632));
#85549=CARTESIAN_POINT('Ctrl Pts',(-158.52963423227,-227.836194356948,15.8205398886314));
#85550=CARTESIAN_POINT('Ctrl Pts',(-161.585218201835,-227.773636092576,
15.6617820233996));
#85551=CARTESIAN_POINT('Ctrl Pts',(-163.190010535425,-225.172646185314,
15.5030241581678));
#85552=CARTESIAN_POINT('Ctrl Pts',(-161.875305352435,-222.413650496059,
15.344266292936));
#85553=CARTESIAN_POINT('Ctrl Pts',(-158.844320784643,-222.021681771096,
15.1855084277042));
#85554=CARTESIAN_POINT('Ctrl Pts',(-156.871013789299,-224.355469772111,
15.0267505624725));
#85555=CARTESIAN_POINT('Ctrl Pts',(-157.761354850944,-227.279131812342,
14.8679926972407));
#85556=CARTESIAN_POINT('Ctrl Pts',(-160.700503864973,-228.116932507544,
14.7092348320089));
#85557=CARTESIAN_POINT('Ctrl Pts',(-162.998551769325,-226.10211669441,14.5504769667771));
#85558=CARTESIAN_POINT('Ctrl Pts',(-162.552325212306,-223.078643725893,
14.3917191015453));
#85559=CARTESIAN_POINT('Ctrl Pts',(-159.770210721352,-221.813595943883,
14.2329612363135));
#85560=CARTESIAN_POINT('Ctrl Pts',(-157.198399369181,-223.464745028728,
14.0742033710817));
#85561=CARTESIAN_POINT('Ctrl Pts',(-157.190612804165,-226.52095940291,13.9154455058499));
#85562=CARTESIAN_POINT('Ctrl Pts',(-159.753977290301,-228.185191791358,
13.7566876406181));
#85563=CARTESIAN_POINT('Ctrl Pts',(-162.542501750679,-226.93433677761,13.5979297753863));
#85564=CARTESIAN_POINT('Ctrl Pts',(-163.004128708817,-223.913176821059,
13.4391719101545));
#85565=CARTESIAN_POINT('Ctrl Pts',(-160.71637719078,-221.886677395137,13.2804140449227));
#85566=CARTESIAN_POINT('Ctrl Pts',(-157.772997295912,-222.709490694757,
13.1216561796909));
#85567=CARTESIAN_POINT('Ctrl Pts',(-156.86777018825,-225.628578020463,12.9628983144592));
#85568=CARTESIAN_POINT('Ctrl Pts',(-158.82915968113,-227.97239076656,12.8041404492274));
#85569=CARTESIAN_POINT('Ctrl Pts',(-161.862102187797,-227.595871599988,
12.6453825839956));
#85570=CARTESIAN_POINT('Ctrl Pts',(-163.190848845418,-224.843610847187,
12.4866247187638));
#85571=CARTESIAN_POINT('Ctrl Pts',(-161.599330765189,-222.234477440891,
12.327866853532));
#85572=CARTESIAN_POINT('Ctrl Pts',(-158.544105231552,-222.15635017194,12.1691089883002));
#85573=CARTESIAN_POINT('Ctrl Pts',(-156.821314532746,-224.680731113806,
12.0103511230684));
#85574=CARTESIAN_POINT('Ctrl Pts',(-158.007656648573,-227.497306927762,
11.8515932578366));
#85575=CARTESIAN_POINT('Ctrl Pts',(-161.017391321278,-228.028347539634,
11.6928353926048));
#85576=CARTESIAN_POINT('Ctrl Pts',(-163.096009496758,-225.78784460232,11.534077527373));
#85577=CARTESIAN_POINT('Ctrl Pts',(-162.341159902552,-222.826306315944,
11.3753196621412));
#85578=CARTESIAN_POINT('Ctrl Pts',(-159.443680857594,-221.854132403737,
11.2165617969094));
#85579=CARTESIAN_POINT('Ctrl Pts',(-157.055345069889,-223.761056391922,
11.0578039316776));
#85580=CARTESIAN_POINT('Ctrl Pts',(-157.361957358426,-226.801861521499,
10.8990460664459));
#85581=CARTESIAN_POINT('Ctrl Pts',(-160.082906168792,-228.193603057457,
10.740288201214));
#85582=CARTESIAN_POINT('Ctrl Pts',(-162.72797925674,-226.662559200816,10.5815303359823));
#85583=CARTESIAN_POINT('Ctrl Pts',(-162.876405836195,-223.609941228966,
10.4227724707505));
#85584=CARTESIAN_POINT('Ctrl Pts',(-160.392345907475,-221.829504989705,
10.2640146055187));
#85585=CARTESIAN_POINT('Ctrl Pts',(-157.549211019663,-222.950705659188,
10.1052567402869));
#85586=CARTESIAN_POINT('Ctrl Pts',(-156.94903811028,-225.947420428797,9.9464988750551));
#85587=CARTESIAN_POINT('Ctrl Pts',(-159.141105402393,-228.077056059227,
9.7877410098233));
#85588=CARTESIAN_POINT('Ctrl Pts',(-162.11923299646,-227.390570105255,9.62898314459151));
#85589=CARTESIAN_POINT('Ctrl Pts',(-163.157838635504,-224.516234484961,
9.47022527935971));
#85590=CARTESIAN_POINT('Ctrl Pts',(-161.306390479514,-222.084641045007,
9.31146741412792));
#85591=CARTESIAN_POINT('Ctrl Pts',(-158.259333808045,-222.321184006019,
9.15270954889613));
#85592=CARTESIAN_POINT('Ctrl Pts',(-156.805334767004,-225.009379259381,
8.99395168366434));
#85593=CARTESIAN_POINT('Ctrl Pts',(-158.275093221573,-227.688990614926,
8.83519381843254));
#85594=CARTESIAN_POINT('Ctrl Pts',(-161.323486291929,-227.907637865433,
8.67643595320076));
#85595=CARTESIAN_POINT('Ctrl Pts',(-163.160624759956,-225.465215055836,
8.51767808796896));
#85596=CARTESIAN_POINT('Ctrl Pts',(-162.10515957196,-222.597027445432,8.35892022273717));
#85597=CARTESIAN_POINT('Ctrl Pts',(-159.12305242649,-221.928040222474,8.20016235750537));
#85598=CARTESIAN_POINT('Ctrl Pts',(-156.943527665811,-224.070510467106,
8.04140449227359));
#85599=CARTESIAN_POINT('Ctrl Pts',(-157.561286265189,-227.063649495691,
7.88264662704179));
#85600=CARTESIAN_POINT('Ctrl Pts',(-160.410955578766,-228.168136586971,
7.72388876181));
#85601=CARTESIAN_POINT('Ctrl Pts',(-162.884518362817,-226.373145198439,
7.56513089657821));
#85602=CARTESIAN_POINT('Ctrl Pts',(-162.718170054648,-223.321451378293,
7.40637303134641));
#85603=CARTESIAN_POINT('Ctrl Pts',(-160.064152619355,-221.805965190726,
7.24761516611462));
#85604=CARTESIAN_POINT('Ctrl Pts',(-157.351422709351,-223.213659535005,
7.08885730088283));
#85605=CARTESIAN_POINT('Ctrl Pts',(-157.062670631596,-226.256212602601,
6.93009943565104));
#85606=CARTESIAN_POINT('Ctrl Pts',(-159.462162276297,-228.149079945696,
6.77134157041924));
#85607=CARTESIAN_POINT('Ctrl Pts',(-162.353882984581,-227.159909446325,
6.61258370518746));
#85608=CARTESIAN_POINT('Ctrl Pts',(-163.091330077941,-224.193989906614,
6.45382583995566));
#85609=CARTESIAN_POINT('Ctrl Pts',(-160.999592005533,-221.965730772674,
6.29506797472387));
#85610=CARTESIAN_POINT('Ctrl Pts',(-157.993027368969,-222.514434716263,
6.13631010949207));
#85611=CARTESIAN_POINT('Ctrl Pts',(-156.823244005403,-225.337927909786,
5.97755224426028));
#85612=CARTESIAN_POINT('Ctrl Pts',(-158.560827603168,-227.852149493561,
5.8187943790285));
#85613=CARTESIAN_POINT('Ctrl Pts',(-161.61554172192,-227.756083972987,5.6600365137967));
#85614=CARTESIAN_POINT('Ctrl Pts',(-163.1917121203,-225.137650508716,5.50127864856491));
#85615=CARTESIAN_POINT('Ctrl Pts',(-161.846827711693,-222.393239304281,
5.34252078333311));
#85616=CARTESIAN_POINT('Ctrl Pts',(-158.811726653968,-222.034535386059,
5.18376291810132));
#85617=CARTESIAN_POINT('Ctrl Pts',(-156.864133315805,-224.389824565903,
5.02500505286953));
#85618=CARTESIAN_POINT('Ctrl Pts',(-157.786485043701,-227.303546279037,
4.86624718763773));
#85619=CARTESIAN_POINT('Ctrl Pts',(-160.734645572559,-228.109062528182,
4.70748932240594));
#85620=CARTESIAN_POINT('Ctrl Pts',(-163.010458502297,-226.069164873794,
4.54873145717415));
#85621=CARTESIAN_POINT('Ctrl Pts',(-162.531099929123,-223.050767568959,
4.38997359194236));
#85622=CARTESIAN_POINT('Ctrl Pts',(-159.735278800335,-221.816307708349,
4.23121572671057));
#85623=CARTESIAN_POINT('Ctrl Pts',(-157.181730503097,-223.495562907887,
4.07245786147877));
#85624=CARTESIAN_POINT('Ctrl Pts',(-157.207462338545,-226.551678874916,
3.91369999624698));
#85625=CARTESIAN_POINT('Ctrl Pts',(-159.788924532055,-228.187698396745,
3.75494213101518));
#85626=CARTESIAN_POINT('Ctrl Pts',(-162.563562985294,-226.906336471008,
3.5961842657834));
#85627=CARTESIAN_POINT('Ctrl Pts',(-162.992028695687,-223.880295482423,
3.4374264005516));
#85628=CARTESIAN_POINT('Ctrl Pts',(-160.682189860438,-221.879008023352,
3.27866853531981));
#85629=CARTESIAN_POINT('Ctrl Pts',(-157.748010893835,-222.734052300533,
3.11991067008802));
#85630=CARTESIAN_POINT('Ctrl Pts',(-156.874852264295,-225.662891819106,
2.96115280485622));
#85631=CARTESIAN_POINT('Ctrl Pts',(-158.861828728588,-227.985052779313,
2.80239493962443));
#85632=CARTESIAN_POINT('Ctrl Pts',(-161.890459477026,-227.575293535821,
2.64363707439264));
#85633=CARTESIAN_POINT('Ctrl Pts',(-163.18894182522,-224.808625785839,2.48487920916085));
#85634=CARTESIAN_POINT('Ctrl Pts',(-161.568904659887,-222.217103633969,
2.32612134392905));
#85635=CARTESIAN_POINT('Ctrl Pts',(-158.513006178533,-222.172488282818,
2.16736347869726));
#85636=CARTESIAN_POINT('Ctrl Pts',(-156.81800403756,-224.71561122042,2.00860561346547));
#85637=CARTESIAN_POINT('Ctrl Pts',(-158.035165195383,-227.519007429433,
1.84984774823368));
#85638=CARTESIAN_POINT('Ctrl Pts',(-161.05054159698,-228.017006744663,1.69108988300188));
#85639=CARTESIAN_POINT('Ctrl Pts',(-163.104465466566,-225.7538444972,1.53233201777009));
#85640=CARTESIAN_POINT('Ctrl Pts',(-162.317176238485,-222.80075779587,1.3735741525383));
#85641=CARTESIAN_POINT('Ctrl Pts',(-159.409220739539,-221.860429922718,
1.21481628730651));
#85642=CARTESIAN_POINT('Ctrl Pts',(-157.04191873346,-223.793410627992,1.05605842207472));
#85643=CARTESIAN_POINT('Ctrl Pts',(-157.381909987635,-226.830715482678,
0.897300556842923));
#85644=CARTESIAN_POINT('Ctrl Pts',(-160.117858009173,-228.192438370269,
0.738542691611127));
#85645=CARTESIAN_POINT('Ctrl Pts',(-162.746189540825,-226.632672581258,
0.579784826379337));
#85646=CARTESIAN_POINT('Ctrl Pts',(-162.86069567705,-223.578205874871,0.421026961147545));
#85647=CARTESIAN_POINT('Ctrl Pts',(-160.358157726966,-221.825957897847,
0.26226909591575));
#85648=CARTESIAN_POINT('Ctrl Pts',(-157.525626832351,-222.976510157985,
0.103511230683962));
#85649=CARTESIAN_POINT('Ctrl Pts',(-156.962288097762,-225.983143426199,
-0.0552466345478338));
#85650=CARTESIAN_POINT('Ctrl Pts',(-158.43372769508,-227.379023915733,-0.161085211369028));
#85651=CARTESIAN_POINT('Ctrl Pts',(-159.301933573839,-227.611132185939,
-0.214004499779625));
#85652=CARTESIAN_POINT('Ctrl Pts',(-157.804802895981,-223.123136560921,
20.2140044997796));
#85653=CARTESIAN_POINT('Ctrl Pts',(-157.180742620438,-223.853043319762,
20.161085211369));
#85654=CARTESIAN_POINT('Ctrl Pts',(-156.729879173041,-225.972907029956,
20.0552466345478));
#85655=CARTESIAN_POINT('Ctrl Pts',(-159.045823488024,-228.27960122976,19.896488769316));
#85656=CARTESIAN_POINT('Ctrl Pts',(-162.236589360548,-227.57830865422,19.7377309040842));
#85657=CARTESIAN_POINT('Ctrl Pts',(-163.37974600956,-224.520518247638,19.5789730388525));
#85658=CARTESIAN_POINT('Ctrl Pts',(-161.430095714629,-221.900030936057,
19.4202151736207));
#85659=CARTESIAN_POINT('Ctrl Pts',(-158.171460220963,-222.117367443797,
19.2614573083889));
#85660=CARTESIAN_POINT('Ctrl Pts',(-156.586382213157,-224.972536314815,
19.1026994431571));
#85661=CARTESIAN_POINT('Ctrl Pts',(-158.125409506143,-227.853009993757,
18.9439415779253));
#85662=CARTESIAN_POINT('Ctrl Pts',(-161.380080048394,-228.122327090623,
18.7851837126935));
#85663=CARTESIAN_POINT('Ctrl Pts',(-163.371692660391,-225.534130049582,
18.6264258474617));
#85664=CARTESIAN_POINT('Ctrl Pts',(-162.277536486599,-222.457078175749,
18.4676679822299));
#85665=CARTESIAN_POINT('Ctrl Pts',(-159.09897698363,-221.707317427635,18.3089101169981));
#85666=CARTESIAN_POINT('Ctrl Pts',(-156.745034686285,-223.971015219991,
18.1501522517663));
#85667=CARTESIAN_POINT('Ctrl Pts',(-157.370036045468,-227.176441972781,
17.9913943865345));
#85668=CARTESIAN_POINT('Ctrl Pts',(-160.401980539204,-228.389988091059,
17.8326365213027));
#85669=CARTESIAN_POINT('Ctrl Pts',(-163.066032349974,-226.501017736455,
17.6738786560709));
#85670=CARTESIAN_POINT('Ctrl Pts',(-162.924051527288,-223.238315770043,
17.5151207908391));
#85671=CARTESIAN_POINT('Ctrl Pts',(-160.10597883643,-221.587907256516,17.3563629256074));
#85672=CARTESIAN_POINT('Ctrl Pts',(-157.190914330871,-223.060245832273,
17.1976050603756));
#85673=CARTESIAN_POINT('Ctrl Pts',(-156.84672491334,-226.307847372741,17.0388471951438));
#85674=CARTESIAN_POINT('Ctrl Pts',(-159.388412733961,-228.358507036245,
16.880089329912));
#85675=CARTESIAN_POINT('Ctrl Pts',(-162.489825195042,-227.335461198446,
16.7213314646802));
#85676=CARTESIAN_POINT('Ctrl Pts',(-163.312549736191,-224.175001360682,
16.5625735994484));
#85677=CARTESIAN_POINT('Ctrl Pts',(-161.103628888722,-221.769580246619,
16.4038157342166));
#85678=CARTESIAN_POINT('Ctrl Pts',(-157.884666925848,-222.320639163124,
16.2450578689848));
#85679=CARTESIAN_POINT('Ctrl Pts',(-156.60165770918,-225.323849012509,16.086300003753));
#85680=CARTESIAN_POINT('Ctrl Pts',(-158.42881122347,-228.03067225822,15.9275421385212));
#85681=CARTESIAN_POINT('Ctrl Pts',(-161.693916644237,-227.963824372464,
15.7687842732894));
#85682=CARTESIAN_POINT('Ctrl Pts',(-163.408749618819,-225.184484537541,
15.6100264080576));
#85683=CARTESIAN_POINT('Ctrl Pts',(-162.003895076299,-222.236304461133,
15.4512685428259));
#85684=CARTESIAN_POINT('Ctrl Pts',(-158.765075838754,-221.817458433208,
15.292510677594));
#85685=CARTESIAN_POINT('Ctrl Pts',(-156.656459145018,-224.311274322064,
15.1337528123623));
#85686=CARTESIAN_POINT('Ctrl Pts',(-157.60785091028,-227.435411924282,14.9749949471305));
#85687=CARTESIAN_POINT('Ctrl Pts',(-160.748537428385,-228.330660629168,
14.8162370818987));
#85688=CARTESIAN_POINT('Ctrl Pts',(-163.204162521467,-226.177688857214,
14.6574792166669));
#85689=CARTESIAN_POINT('Ctrl Pts',(-162.727338200903,-222.94689628945,14.4987213514351));
#85690=CARTESIAN_POINT('Ctrl Pts',(-159.754454066123,-221.595104156844,
14.3399634862033));
#85691=CARTESIAN_POINT('Ctrl Pts',(-157.00629356037,-223.359472566001,14.1812056209715));
#85692=CARTESIAN_POINT('Ctrl Pts',(-156.997973070443,-226.625251618241,
14.0224477557397));
#85693=CARTESIAN_POINT('Ctrl Pts',(-159.737107508394,-228.403600453379,
13.8636898905079));
#85694=CARTESIAN_POINT('Ctrl Pts',(-162.716841144325,-227.066974287427,
13.7049320252761));
#85695=CARTESIAN_POINT('Ctrl Pts',(-163.210121871807,-223.838653334904,
13.5461741600443));
#85696=CARTESIAN_POINT('Ctrl Pts',(-160.765499188446,-221.673196804608,
13.3874162948125));
#85697=CARTESIAN_POINT('Ctrl Pts',(-157.620291677922,-222.552430427911,
13.2286584295807));
#85698=CARTESIAN_POINT('Ctrl Pts',(-156.652993130184,-225.671679627342,
13.069900564349));
#85699=CARTESIAN_POINT('Ctrl Pts',(-158.748875138084,-228.176207658242,
12.9111426991172));
#85700=CARTESIAN_POINT('Ctrl Pts',(-161.98978657041,-227.773870565221,12.7523848338854));
#85701=CARTESIAN_POINT('Ctrl Pts',(-163.409645411744,-224.832887239989,
12.5936269686536));
#85702=CARTESIAN_POINT('Ctrl Pts',(-161.70899690633,-222.044845506148,12.4348691034218));
#85703=CARTESIAN_POINT('Ctrl Pts',(-158.444274499449,-221.961361048871,
12.27611123819));
#85704=CARTESIAN_POINT('Ctrl Pts',(-156.603352009494,-224.658838840176,
12.1173533729582));
#85705=CARTESIAN_POINT('Ctrl Pts',(-157.87104162688,-227.668547311536,11.9585955077264));
#85706=CARTESIAN_POINT('Ctrl Pts',(-161.087153863627,-228.236001388316,
11.7998376424946));
#85707=CARTESIAN_POINT('Ctrl Pts',(-163.308302927133,-225.841867121762,
11.6410797772628));
#85708=CARTESIAN_POINT('Ctrl Pts',(-162.501693281823,-222.677256098477,
11.482321912031));
#85709=CARTESIAN_POINT('Ctrl Pts',(-159.405534043365,-221.638420202526,
11.3235640467992));
#85710=CARTESIAN_POINT('Ctrl Pts',(-156.853430025042,-223.676102005032,
11.1648061815675));
#85711=CARTESIAN_POINT('Ctrl Pts',(-157.181066724065,-226.925415200472,
11.0060483163357));
#85712=CARTESIAN_POINT('Ctrl Pts',(-160.088591046371,-228.412588480155,
10.8472904511039));
#85713=CARTESIAN_POINT('Ctrl Pts',(-162.915036846522,-226.776560916997,
10.6885325858721));
#85714=CARTESIAN_POINT('Ctrl Pts',(-163.073641039367,-223.514624872465,
10.5297747206403));
#85715=CARTESIAN_POINT('Ctrl Pts',(-160.419249073851,-221.612104086242,
10.3710168554085));
#85716=CARTESIAN_POINT('Ctrl Pts',(-157.381160372433,-222.810185507065,
10.2122589901767));
#85717=CARTESIAN_POINT('Ctrl Pts',(-156.739833595181,-226.01238506571,10.0535011249449));
#85718=CARTESIAN_POINT('Ctrl Pts',(-159.082210983416,-228.288049852028,
9.89474325971311));
#85719=CARTESIAN_POINT('Ctrl Pts',(-162.264548843538,-227.554491543069,
9.73598539448133));
#85720=CARTESIAN_POINT('Ctrl Pts',(-163.374371691105,-224.483062674347,
9.57722752924952));
#85721=CARTESIAN_POINT('Ctrl Pts',(-161.395969699666,-221.884734825734,
9.41846966401773));
#85722=CARTESIAN_POINT('Ctrl Pts',(-158.139976293989,-222.137497542104,
9.25971179878595));
#85723=CARTESIAN_POINT('Ctrl Pts',(-156.586276510909,-225.010022395376,
9.10095393355415));
#85724=CARTESIAN_POINT('Ctrl Pts',(-158.156816330804,-227.873374752793,
8.94219606832236));
#85725=CARTESIAN_POINT('Ctrl Pts',(-161.414237772266,-228.107014649447,
8.78343820309056));
#85726=CARTESIAN_POINT('Ctrl Pts',(-163.377348860164,-225.497114861107,
8.62468033785877));
#85727=CARTESIAN_POINT('Ctrl Pts',(-162.249510404051,-222.432255571431,
8.46592247262698));
#85728=CARTESIAN_POINT('Ctrl Pts',(-159.062920114611,-221.717395881806,
8.30716460739519));
#85729=CARTESIAN_POINT('Ctrl Pts',(-156.733945299429,-224.006775352068,
8.1484067421634));
#85730=CARTESIAN_POINT('Ctrl Pts',(-157.394063617775,-227.205153981059,
7.9896488769316));
#85731=CARTESIAN_POINT('Ctrl Pts',(-160.439134810658,-228.385375773301,
7.83089101169981));
#85732=CARTESIAN_POINT('Ctrl Pts',(-163.082309842095,-226.467301790944,
7.67213314646802));
#85733=CARTESIAN_POINT('Ctrl Pts',(-162.904555027255,-223.206353267216,
7.51337528123622));
#85734=CARTESIAN_POINT('Ctrl Pts',(-160.068551565691,-221.586950162798,
7.35461741600443));
#85735=CARTESIAN_POINT('Ctrl Pts',(-157.169809713902,-223.091170135173,
7.19585955077264));
#85736=CARTESIAN_POINT('Ctrl Pts',(-156.861257900655,-226.342351124774,
7.03710168554085));
#85737=CARTESIAN_POINT('Ctrl Pts',(-159.425282733301,-228.365012417769,
6.87834382030906));
#85738=CARTESIAN_POINT('Ctrl Pts',(-162.51528878583,-227.308014478348,6.71958595507726));
#85739=CARTESIAN_POINT('Ctrl Pts',(-163.303302640478,-224.138721779103,
6.56082808984547));
#85740=CARTESIAN_POINT('Ctrl Pts',(-161.06813404846,-221.757670873754,6.40207022461368));
#85741=CARTESIAN_POINT('Ctrl Pts',(-157.855409217295,-222.343999457244,
6.24331235938189));
#85742=CARTESIAN_POINT('Ctrl Pts',(-156.605413786127,-225.36109963302,6.08455449415009));
#85743=CARTESIAN_POINT('Ctrl Pts',(-158.462143524407,-228.047721438856,
5.9257966289183));
#85744=CARTESIAN_POINT('Ctrl Pts',(-161.726319448675,-227.945068703699,
5.76703876368651));
#85745=CARTESIAN_POINT('Ctrl Pts',(-163.410567881401,-225.14708920673,5.60828089845471));
#85746=CARTESIAN_POINT('Ctrl Pts',(-161.973464723187,-222.214493673545,
5.44952303322292));
#85747=CARTESIAN_POINT('Ctrl Pts',(-158.730246727916,-221.831193420794,
5.29076516799113));
#85748=CARTESIAN_POINT('Ctrl Pts',(-156.649106877325,-224.347984824723,
5.13200730275933));
#85749=CARTESIAN_POINT('Ctrl Pts',(-157.634704280835,-227.461500491424,
4.97324943752755));
#85750=CARTESIAN_POINT('Ctrl Pts',(-160.785020233513,-228.322251005172,
4.81449157229575));
#85751=CARTESIAN_POINT('Ctrl Pts',(-163.216885699347,-226.142477529628,
4.65573370706396));
#85752=CARTESIAN_POINT('Ctrl Pts',(-162.704657499646,-222.917108663901,
4.49697584183216));
#85753=CARTESIAN_POINT('Ctrl Pts',(-159.717126862614,-221.598001867052,
4.33821797660038));
#85754=CARTESIAN_POINT('Ctrl Pts',(-156.988481709821,-223.392403627723,
4.17946011136858));
#85755=CARTESIAN_POINT('Ctrl Pts',(-157.015977977717,-226.65807752503,4.02070224613679));
#85756=CARTESIAN_POINT('Ctrl Pts',(-159.774451083183,-228.406278936745,
3.861944380905));
#85757=CARTESIAN_POINT('Ctrl Pts',(-162.7393465482,-227.037053999266,3.70318651567321));
#85758=CARTESIAN_POINT('Ctrl Pts',(-163.197192160546,-223.803517322249,
3.54442865044141));
#85759=CARTESIAN_POINT('Ctrl Pts',(-160.728967632209,-221.665001543853,
3.38567078520962));
#85760=CARTESIAN_POINT('Ctrl Pts',(-157.593591957777,-222.578676223465,
3.22691291997783));
#85761=CARTESIAN_POINT('Ctrl Pts',(-156.660560824318,-225.708346323814,
3.06815505474603));
#85762=CARTESIAN_POINT('Ctrl Pts',(-158.78378430275,-228.189737905452,2.90939718951424));
#85763=CARTESIAN_POINT('Ctrl Pts',(-162.020088319504,-227.751881462801,
2.75063932428245));
#85764=CARTESIAN_POINT('Ctrl Pts',(-163.407607627134,-224.795503252315,
2.59188145905066));
#85765=CARTESIAN_POINT('Ctrl Pts',(-161.676484482407,-222.026280376954,
2.43312359381886));
#85766=CARTESIAN_POINT('Ctrl Pts',(-158.41104298377,-221.978605750321,2.27436572858707));
#85767=CARTESIAN_POINT('Ctrl Pts',(-156.599814513589,-224.696110676368,
2.11560786335528));
#85768=CARTESIAN_POINT('Ctrl Pts',(-157.900436435271,-227.691735817022,
1.95684999812349));
#85769=CARTESIAN_POINT('Ctrl Pts',(-161.122577254367,-228.223882954817,
1.7980921328917));
#85770=CARTESIAN_POINT('Ctrl Pts',(-163.317338722953,-225.805535628783,
1.6393342676599));
#85771=CARTESIAN_POINT('Ctrl Pts',(-162.476065057453,-222.649955715892,
1.48057640242811));
#85772=CARTESIAN_POINT('Ctrl Pts',(-159.368710994356,-221.645149542503,
1.32181853719632));
#85773=CARTESIAN_POINT('Ctrl Pts',(-156.839083044467,-223.710674771688,
1.16306067196453));
#85774=CARTESIAN_POINT('Ctrl Pts',(-157.20238750544,-226.956247678321,1.00430280673273));
#85775=CARTESIAN_POINT('Ctrl Pts',(-160.125939535115,-228.411343930344,
0.845544941500937));
#85776=CARTESIAN_POINT('Ctrl Pts',(-162.934495810134,-226.744624971365,
0.686787076269146));
#85777=CARTESIAN_POINT('Ctrl Pts',(-163.05685363431,-223.480713424532,0.528029211037356));
#85778=CARTESIAN_POINT('Ctrl Pts',(-160.38271660915,-221.608313770228,0.36927134580556));
#85779=CARTESIAN_POINT('Ctrl Pts',(-157.355959016946,-222.837759420837,
0.210513480573772));
#85780=CARTESIAN_POINT('Ctrl Pts',(-156.753992134557,-226.050557589728,
0.0517556153419762));
#85781=CARTESIAN_POINT('Ctrl Pts',(-158.326328373192,-227.542153631111,
-0.0540829614792177));
#85782=CARTESIAN_POINT('Ctrl Pts',(-159.254067145653,-227.790177569842,
-0.107002249889815));
#85783=CARTESIAN_POINT('Ctrl Pts',(-157.663937342304,-223.002698443069,
20.3210067496694));
#85784=CARTESIAN_POINT('Ctrl Pts',(-156.999831188384,-223.779443237332,
20.2680874612588));
#85785=CARTESIAN_POINT('Ctrl Pts',(-156.520035883781,-226.035338365711,
20.1622488844376));
#85786=CARTESIAN_POINT('Ctrl Pts',(-158.984594087522,-228.490052875411,
20.0034910192058));
#85787=CARTESIAN_POINT('Ctrl Pts',(-162.380111050717,-227.743758433405,
19.844733153974));
#85788=CARTESIAN_POINT('Ctrl Pts',(-163.596623934578,-224.489749956991,
19.6859752887423));
#85789=CARTESIAN_POINT('Ctrl Pts',(-161.521864797362,-221.70110626648,19.5272174235105));
#85790=CARTESIAN_POINT('Ctrl Pts',(-158.054123026994,-221.932389233715,
19.3684595582787));
#85791=CARTESIAN_POINT('Ctrl Pts',(-156.367330739964,-224.970773973196,
19.2097016930469));
#85792=CARTESIAN_POINT('Ctrl Pts',(-158.005117242933,-228.036087327305,
19.0509438278151));
#85793=CARTESIAN_POINT('Ctrl Pts',(-161.468639631394,-228.322686472282,
18.8921859625833));
#85794=CARTESIAN_POINT('Ctrl Pts',(-163.58805380289,-225.568405115375,18.7334280973515));
#85795=CARTESIAN_POINT('Ctrl Pts',(-162.423685749286,-222.293899165502,
18.5746702321197));
#85796=CARTESIAN_POINT('Ctrl Pts',(-159.04115843702,-221.496026353686,18.4159123668879));
#85797=CARTESIAN_POINT('Ctrl Pts',(-156.536163924622,-223.90498538126,18.2571545016561));
#85798=CARTESIAN_POINT('Ctrl Pts',(-157.201271551415,-227.316104011775,
18.0983966364243));
#85799=CARTESIAN_POINT('Ctrl Pts',(-160.427775585634,-228.607523249306,
17.9396387711926));
#85800=CARTESIAN_POINT('Ctrl Pts',(-163.262779304396,-226.597337877429,
17.7808809059607));
#85801=CARTESIAN_POINT('Ctrl Pts',(-163.111687588131,-223.125268689213,
17.622123040729));
#85802=CARTESIAN_POINT('Ctrl Pts',(-160.11277948656,-221.368953645186,17.4633651754972));
#85803=CARTESIAN_POINT('Ctrl Pts',(-157.010655616342,-222.935772023368,
17.3046073102654));
#85804=CARTESIAN_POINT('Ctrl Pts',(-156.644379602221,-226.39177179299,17.1458494450336));
#85805=CARTESIAN_POINT('Ctrl Pts',(-159.349167247214,-228.574022058711,
16.9870915798018));
#85806=CARTESIAN_POINT('Ctrl Pts',(-162.649597000506,-227.48532748344,16.82833371457));
#85807=CARTESIAN_POINT('Ctrl Pts',(-163.52511568383,-224.12206128988,16.6695758493382));
#85808=CARTESIAN_POINT('Ctrl Pts',(-161.174448631596,-221.562284570829,
16.5108179841064));
#85809=CARTESIAN_POINT('Ctrl Pts',(-157.748926238073,-222.148704876632,
16.3520601188746));
#85810=CARTESIAN_POINT('Ctrl Pts',(-156.383586462865,-225.344630367573,
16.1933022536428));
#85811=CARTESIAN_POINT('Ctrl Pts',(-158.327988214669,-228.225150159492,
16.034544388411));
#85812=CARTESIAN_POINT('Ctrl Pts',(-161.80261508664,-228.154012652352,15.8757865231792));
#85813=CARTESIAN_POINT('Ctrl Pts',(-163.627488702212,-225.196322889768,
15.7170286579475));
#85814=CARTESIAN_POINT('Ctrl Pts',(-162.132484800163,-222.058958426208,
15.5582707927157));
#85815=CARTESIAN_POINT('Ctrl Pts',(-158.685830892865,-221.613235095319,
15.3995129274839));
#85816=CARTESIAN_POINT('Ctrl Pts',(-156.441904500737,-224.267078872017,
15.2407550622521));
#85817=CARTESIAN_POINT('Ctrl Pts',(-157.454346969616,-227.591692036222,
15.0819971970203));
#85818=CARTESIAN_POINT('Ctrl Pts',(-160.796570991797,-228.544388750793,
14.9232393317885));
#85819=CARTESIAN_POINT('Ctrl Pts',(-163.409773273609,-226.253261020018,
14.7644814665567));
#85820=CARTESIAN_POINT('Ctrl Pts',(-162.902351189501,-222.815148853006,
14.6057236013249));
#85821=CARTESIAN_POINT('Ctrl Pts',(-159.738697410893,-221.376612369806,
14.4469657360931));
#85822=CARTESIAN_POINT('Ctrl Pts',(-156.814187751561,-223.254200103273,
14.2882078708613));
#85823=CARTESIAN_POINT('Ctrl Pts',(-156.805333336721,-226.729543833573,
14.1294500056295));
#85824=CARTESIAN_POINT('Ctrl Pts',(-159.720237726487,-228.622009115399,
13.9706921403977));
#85825=CARTESIAN_POINT('Ctrl Pts',(-162.891180537971,-227.199611797244,
13.8119342751659));
#85826=CARTESIAN_POINT('Ctrl Pts',(-163.416115034797,-223.764129848749,
13.6531764099341));
#85827=CARTESIAN_POINT('Ctrl Pts',(-160.814621186112,-221.459716214079,
13.4944185447024));
#85828=CARTESIAN_POINT('Ctrl Pts',(-157.467586059932,-222.395370161066,
13.3356606794706));
#85829=CARTESIAN_POINT('Ctrl Pts',(-156.438216072117,-225.714781234221,
13.1769028142388));
#85830=CARTESIAN_POINT('Ctrl Pts',(-158.668590595037,-228.380024549925,
13.018144949007));
#85831=CARTESIAN_POINT('Ctrl Pts',(-162.117470953023,-227.951869530454,
12.8593870837752));
#85832=CARTESIAN_POINT('Ctrl Pts',(-163.628441978069,-224.822163632791,
12.7006292185434));
#85833=CARTESIAN_POINT('Ctrl Pts',(-161.818663047472,-221.855213571405,
12.5418713533116));
#85834=CARTESIAN_POINT('Ctrl Pts',(-158.344443767345,-221.766371925803,
12.3831134880798));
#85835=CARTESIAN_POINT('Ctrl Pts',(-156.385389486241,-224.636946566547,
12.224355622848));
#85836=CARTESIAN_POINT('Ctrl Pts',(-157.734426605188,-227.839787695311,
12.0655977576162));
#85837=CARTESIAN_POINT('Ctrl Pts',(-161.156916405975,-228.443655236998,
11.9068398923844));
#85838=CARTESIAN_POINT('Ctrl Pts',(-163.520596357509,-225.895889641203,
11.7480820271526));
#85839=CARTESIAN_POINT('Ctrl Pts',(-162.662226661094,-222.528205881009,
11.5893241619208));
#85840=CARTESIAN_POINT('Ctrl Pts',(-159.367387229136,-221.422708001315,
11.4305662966891));
#85841=CARTESIAN_POINT('Ctrl Pts',(-156.651514980196,-223.591147618143,
11.2718084314573));
#85842=CARTESIAN_POINT('Ctrl Pts',(-157.000176089704,-227.048968879445,
11.1130505662255));
#85843=CARTESIAN_POINT('Ctrl Pts',(-160.09427592395,-228.631573902853,10.9542927009937));
#85844=CARTESIAN_POINT('Ctrl Pts',(-163.102094436304,-226.890562633178,
10.7955348357619));
#85845=CARTESIAN_POINT('Ctrl Pts',(-163.27087624254,-223.419308515963,10.6367769705301));
#85846=CARTESIAN_POINT('Ctrl Pts',(-160.446152240227,-221.39470318278,10.4780191052983));
#85847=CARTESIAN_POINT('Ctrl Pts',(-157.213109725203,-222.669665354942,
10.3192612400665));
#85848=CARTESIAN_POINT('Ctrl Pts',(-156.530629080082,-226.077349702623,
10.1605033748347));
#85849=CARTESIAN_POINT('Ctrl Pts',(-159.02331656444,-228.499043644829,10.0017455096029));
#85850=CARTESIAN_POINT('Ctrl Pts',(-162.409864690616,-227.718412980884,
9.84298764437113));
#85851=CARTESIAN_POINT('Ctrl Pts',(-163.590904746706,-224.449890863733,
9.68422977913934));
#85852=CARTESIAN_POINT('Ctrl Pts',(-161.48554891982,-221.684828606461,9.52547191390754));
#85853=CARTESIAN_POINT('Ctrl Pts',(-158.020618779932,-221.953811078189,
9.36671404867575));
#85854=CARTESIAN_POINT('Ctrl Pts',(-156.367218254814,-225.010665531371,
9.20795618344397));
#85855=CARTESIAN_POINT('Ctrl Pts',(-158.038539440034,-228.057758890661,
9.04919831821217));
#85856=CARTESIAN_POINT('Ctrl Pts',(-161.504989252603,-228.306391433462,
8.89044045298037));
#85857=CARTESIAN_POINT('Ctrl Pts',(-163.594072960372,-225.529014666379,
8.73168258774858));
#85858=CARTESIAN_POINT('Ctrl Pts',(-162.393861236142,-222.267483697429,
8.5729247225168));
#85859=CARTESIAN_POINT('Ctrl Pts',(-159.002787802732,-221.506751541139,
8.41416685728499));
#85860=CARTESIAN_POINT('Ctrl Pts',(-156.524362933047,-223.943040237029,
8.25540899205321));
#85861=CARTESIAN_POINT('Ctrl Pts',(-157.226840970362,-227.346658466427,
8.09665112682141));
#85862=CARTESIAN_POINT('Ctrl Pts',(-160.46731404255,-228.602614959631,7.93789326158962));
#85863=CARTESIAN_POINT('Ctrl Pts',(-163.280101321373,-226.56145838345,7.77913539635782));
#85864=CARTESIAN_POINT('Ctrl Pts',(-163.090939999863,-223.091255156139,
7.62037753112604));
#85865=CARTESIAN_POINT('Ctrl Pts',(-160.072950512026,-221.36793513487,7.46161966589424));
#85866=CARTESIAN_POINT('Ctrl Pts',(-156.988196718452,-222.968680735341,
7.30286180066245));
#85867=CARTESIAN_POINT('Ctrl Pts',(-156.659845169714,-226.428489646948,
7.14410393543065));
#85868=CARTESIAN_POINT('Ctrl Pts',(-159.388403190305,-228.580944889843,
6.98534607019887));
#85869=CARTESIAN_POINT('Ctrl Pts',(-162.676694587079,-227.45611951037,6.82658820496707));
#85870=CARTESIAN_POINT('Ctrl Pts',(-163.515275203016,-224.083453651592,
6.66783033973528));
#85871=CARTESIAN_POINT('Ctrl Pts',(-161.136676091388,-221.549610974834,
6.50907247450348));
#85872=CARTESIAN_POINT('Ctrl Pts',(-157.71779106562,-222.173564198225,6.3503146092717));
#85873=CARTESIAN_POINT('Ctrl Pts',(-156.387583566852,-225.384271356254,
6.1915567440399));
#85874=CARTESIAN_POINT('Ctrl Pts',(-158.363459445645,-228.24329338415,6.03279887880811));
#85875=CARTESIAN_POINT('Ctrl Pts',(-161.837097175429,-228.134053434412,
5.87404101357632));
#85876=CARTESIAN_POINT('Ctrl Pts',(-163.629423642502,-225.156527904744,
5.71528314834452));
#85877=CARTESIAN_POINT('Ctrl Pts',(-162.100101734681,-222.03574804281,5.55652528311273));
#85878=CARTESIAN_POINT('Ctrl Pts',(-158.648766801864,-221.627851455529,
5.39776741788094));
#85879=CARTESIAN_POINT('Ctrl Pts',(-156.434080438846,-224.306145083543,
5.23900955264915));
#85880=CARTESIAN_POINT('Ctrl Pts',(-157.482923517968,-227.619454703812,
5.08025168741736));
#85881=CARTESIAN_POINT('Ctrl Pts',(-160.835394894467,-228.535439482161,
4.92149382218556));
#85882=CARTESIAN_POINT('Ctrl Pts',(-163.423312896397,-226.215790185461,
4.76273595695377));
#85883=CARTESIAN_POINT('Ctrl Pts',(-162.87821507017,-222.783449758844,4.60397809172198));
#85884=CARTESIAN_POINT('Ctrl Pts',(-159.698974924892,-221.379696025755,
4.44522022649019));
#85885=CARTESIAN_POINT('Ctrl Pts',(-156.795232916545,-223.289244347558,
4.28646236125839));
#85886=CARTESIAN_POINT('Ctrl Pts',(-156.82449361689,-226.764476175145,4.1277044960266));
#85887=CARTESIAN_POINT('Ctrl Pts',(-159.759977634311,-228.624859476745,
3.96894663079481));
#85888=CARTESIAN_POINT('Ctrl Pts',(-162.915130111106,-227.167771527524,
3.81018876556301));
#85889=CARTESIAN_POINT('Ctrl Pts',(-163.402355625404,-223.726739162074,
3.65143090033122));
#85890=CARTESIAN_POINT('Ctrl Pts',(-160.77574540398,-221.450995064354,3.49267303509943));
#85891=CARTESIAN_POINT('Ctrl Pts',(-157.439173021718,-222.423300146398,
3.33391516986764));
#85892=CARTESIAN_POINT('Ctrl Pts',(-156.446269384341,-225.753800828521,
3.17515730463584));
#85893=CARTESIAN_POINT('Ctrl Pts',(-158.705739876912,-228.394423031591,
3.01639943940405));
#85894=CARTESIAN_POINT('Ctrl Pts',(-162.149717161981,-227.928469389781,
2.85764157417226));
#85895=CARTESIAN_POINT('Ctrl Pts',(-163.626273429048,-224.782380718792,
2.69888370894047));
#85896=CARTESIAN_POINT('Ctrl Pts',(-161.784064304926,-221.835457119938,
2.54012584370867));
#85897=CARTESIAN_POINT('Ctrl Pts',(-158.309079789007,-221.784723217824,
2.38136797847688));
#85898=CARTESIAN_POINT('Ctrl Pts',(-156.381624989618,-224.676610132315,
2.22261011324509));
#85899=CARTESIAN_POINT('Ctrl Pts',(-157.765707675159,-227.864464204611,
2.0638522480133));
#85900=CARTESIAN_POINT('Ctrl Pts',(-161.194612911753,-228.430759164971,
1.90509438278151));
#85901=CARTESIAN_POINT('Ctrl Pts',(-163.53021197934,-225.857226760367,1.74633651754971));
#85902=CARTESIAN_POINT('Ctrl Pts',(-162.63495387642,-222.499153635915,1.58757865231792));
#85903=CARTESIAN_POINT('Ctrl Pts',(-159.328201249173,-221.429869162289,
1.42882078708612));
#85904=CARTESIAN_POINT('Ctrl Pts',(-156.636247355474,-223.627938915385,
1.27006292185434));
#85905=CARTESIAN_POINT('Ctrl Pts',(-157.022865023245,-227.081779873964,
1.11130505662254));
#85906=CARTESIAN_POINT('Ctrl Pts',(-160.134021061057,-228.63024949042,0.952547191390747));
#85907=CARTESIAN_POINT('Ctrl Pts',(-163.122802079444,-226.856577361471,
0.793789326158957));
#85908=CARTESIAN_POINT('Ctrl Pts',(-163.253011591569,-223.383220974194,
0.635031460927165));
#85909=CARTESIAN_POINT('Ctrl Pts',(-160.407275491335,-221.390669642609,
0.47627359569537));
#85910=CARTESIAN_POINT('Ctrl Pts',(-157.18629120154,-222.69900868369,0.317515730463582));
#85911=CARTESIAN_POINT('Ctrl Pts',(-156.545696171353,-226.117971753255,
0.158757865231786));
#85912=CARTESIAN_POINT('Ctrl Pts',(-158.218929051303,-227.70528334649,0.0529192884105924));
#85913=CARTESIAN_POINT('Ctrl Pts',(-159.206200717467,-227.969222953746,
-4.44089209850063E-15));
#85914=CARTESIAN_POINT('Ctrl Pts',(-159.206200717467,-227.969222953746,
-4.44089209850063E-15));
#85915=CARTESIAN_POINT('Ctrl Pts',(-159.113164853268,-227.935190019033,
-4.15823203790848E-15));
#85916=CARTESIAN_POINT('Ctrl Pts',(-159.022195992629,-227.896385128928,
-5.66635079944646E-15));
#85917=CARTESIAN_POINT('Ctrl Pts',(-158.933501676326,-227.853137676309,
-5.99520433297585E-15));
#85918=CARTESIAN_POINT('Ctrl Pts',(-158.842829036744,-227.808925590939,
-6.33139293179453E-15));
#85919=CARTESIAN_POINT('Ctrl Pts',(-158.754532873528,-227.760069932939,
-5.08640997726718E-15));
#85920=CARTESIAN_POINT('Ctrl Pts',(-158.668863854363,-227.706877060488,
-4.6074255521944E-15));
#85921=CARTESIAN_POINT('Ctrl Pts',(-158.585928616916,-227.655381624328,
-4.14372598595588E-15));
#85922=CARTESIAN_POINT('Ctrl Pts',(-158.505455204851,-227.59982050253,-6.97772062172547E-16));
#85923=CARTESIAN_POINT('Ctrl Pts',(-158.427704734505,-227.540440966992,
1.16573417585641E-15));
#85924=CARTESIAN_POINT('Ctrl Pts',(-158.359673072952,-227.488483873397,
2.79630213413175E-15));
#85925=CARTESIAN_POINT('Ctrl Pts',(-158.29372646032,-227.433602589581,-2.63172470389904E-15));
#85926=CARTESIAN_POINT('Ctrl Pts',(-158.230065068767,-227.375949804433,
-3.1641356201817E-15));
#85927=CARTESIAN_POINT('Ctrl Pts',(-158.216686274063,-227.363833751708,
-3.2760247286858E-15));
#85928=CARTESIAN_POINT('Ctrl Pts',(-158.203406590895,-227.351593348083,
3.2015646022047E-15));
#85929=CARTESIAN_POINT('Ctrl Pts',(-158.190245171691,-227.339246427072,
2.99760216648792E-15));
#85930=CARTESIAN_POINT('Ctrl Pts',(-158.117820261348,-227.271303553023,
1.8752337583938E-15));
#85931=CARTESIAN_POINT('Ctrl Pts',(-158.048861110802,-227.200038557941,
-1.25208198436776E-15));
#85932=CARTESIAN_POINT('Ctrl Pts',(-157.983606937581,-227.125743461044,
-1.36002320516582E-15));
#85933=CARTESIAN_POINT('Ctrl Pts',(-157.918710403508,-227.051855553971,
-1.46737283151989E-15));
#85934=CARTESIAN_POINT('Ctrl Pts',(-157.857477860833,-226.974969868741,
-3.36873373652266E-15));
#85935=CARTESIAN_POINT('Ctrl Pts',(-157.800188235161,-226.895346902578,
-3.80251385934116E-15));
#85936=CARTESIAN_POINT('Ctrl Pts',(-157.744357521391,-226.817751579147,
-4.22524753218019E-15));
#85937=CARTESIAN_POINT('Ctrl Pts',(-157.692271198614,-226.737555871033,
-4.98425732962394E-15));
#85938=CARTESIAN_POINT('Ctrl Pts',(-157.644234215362,-226.654986798192,
-4.69069227904129E-15));
#85939=CARTESIAN_POINT('Ctrl Pts',(-157.623520326731,-226.619382427072,
-4.56410494253316E-15));
#85940=CARTESIAN_POINT('Ctrl Pts',(-157.603559993929,-226.583336637164,
-9.73322648313371E-15));
#85941=CARTESIAN_POINT('Ctrl Pts',(-157.584380642184,-226.546867300965,
-1.06303854607859E-14));
#85942=CARTESIAN_POINT('Ctrl Pts',(-157.571170306177,-226.521747985591,
-1.12483297846706E-14));
#85943=CARTESIAN_POINT('Ctrl Pts',(-157.558330518607,-226.496427729856,
3.35764189332899E-15));
#85944=CARTESIAN_POINT('Ctrl Pts',(-157.545870771917,-226.47091237078,4.05231403988182E-15));
#85945=CARTESIAN_POINT('Ctrl Pts',(-157.539658128808,-226.458189975719,
4.39868947045594E-15));
#85946=CARTESIAN_POINT('Ctrl Pts',(-157.533540525665,-226.445420051201,
-7.52285493344474E-16));
#85947=CARTESIAN_POINT('Ctrl Pts',(-157.527524328383,-226.432614845812,
-1.0547118733939E-15));
#85948=CARTESIAN_POINT('Ctrl Pts',(-157.48732379761,-226.34704982372,-3.0755400524729E-15));
#85949=CARTESIAN_POINT('Ctrl Pts',(-157.451579868608,-226.259774598662,
-4.13920845915888E-15));
#85950=CARTESIAN_POINT('Ctrl Pts',(-157.42054357986,-226.17102724452,-5.19029264012261E-15));
#85951=CARTESIAN_POINT('Ctrl Pts',(-157.390193323743,-226.084241580497,
-6.21814343603167E-15));
#85952=CARTESIAN_POINT('Ctrl Pts',(-157.364344673472,-225.996047472969,
-2.30602227738755E-15));
#85953=CARTESIAN_POINT('Ctrl Pts',(-157.343281522306,-225.906658800827,
-1.83186799063151E-15));
#85954=CARTESIAN_POINT('Ctrl Pts',(-157.33965861153,-225.891283742224,-1.75031235532725E-15));
#85955=CARTESIAN_POINT('Ctrl Pts',(-157.336177403255,-225.875873335079,
-1.11974478500717E-14));
#85956=CARTESIAN_POINT('Ctrl Pts',(-157.332839500122,-225.860428662792,
-1.13520304267922E-14));
#85957=CARTESIAN_POINT('Ctrl Pts',(-157.312711908479,-225.767297123485,
-1.22863078582233E-14));
#85958=CARTESIAN_POINT('Ctrl Pts',(-157.297790949491,-225.672918626754,
-2.72065433198562E-15));
#85959=CARTESIAN_POINT('Ctrl Pts',(-157.287998321733,-225.577701310259,
-2.55351295663786E-15));
#85960=CARTESIAN_POINT('Ctrl Pts',(-157.284735624775,-225.545976909347,
-2.49782497680672E-15));
#85961=CARTESIAN_POINT('Ctrl Pts',(-157.282042626464,-225.514159512456,
-7.4552035416634E-15));
#85962=CARTESIAN_POINT('Ctrl Pts',(-157.27991762978,-225.482264673585,-8.13238365537927E-15));
#85963=CARTESIAN_POINT('Ctrl Pts',(-157.278692828001,-225.463881183537,
-8.52269551529948E-15));
#85964=CARTESIAN_POINT('Ctrl Pts',(-157.277656733797,-225.445471971603,
-5.44258673003032E-15));
#85965=CARTESIAN_POINT('Ctrl Pts',(-157.276809107702,-225.427040064452,
-5.13478148889135E-15));
#85966=CARTESIAN_POINT('Ctrl Pts',(-157.27623458174,-225.41454680917,-4.92614928261313E-15));
#85967=CARTESIAN_POINT('Ctrl Pts',(-157.275746761203,-225.402044751541,
-4.56125519357613E-15));
#85968=CARTESIAN_POINT('Ctrl Pts',(-157.27534569061,-225.389544220778,-4.52415882534751E-15));
#85969=CARTESIAN_POINT('Ctrl Pts',(-157.272356045913,-225.296363254102,
-4.24763653062282E-15));
#85970=CARTESIAN_POINT('Ctrl Pts',(-157.274175073836,-225.203121070918,
-5.75556499322864E-15));
#85971=CARTESIAN_POINT('Ctrl Pts',(-157.280663972965,-225.11019208928,-6.96664947952286E-15));
#85972=CARTESIAN_POINT('Ctrl Pts',(-157.287165723555,-225.017079059002,
-8.18013255502608E-15));
#85973=CARTESIAN_POINT('Ctrl Pts',(-157.298356244342,-224.924279492042,
-6.82012577763791E-15));
#85974=CARTESIAN_POINT('Ctrl Pts',(-157.314146942062,-224.832182066588,
-6.50868248186498E-15));
#85975=CARTESIAN_POINT('Ctrl Pts',(-157.329715012396,-224.741383089712,
-6.20163011344484E-15));
#85976=CARTESIAN_POINT('Ctrl Pts',(-157.349754928696,-224.651265749557,
-6.37045444938708E-15));
#85977=CARTESIAN_POINT('Ctrl Pts',(-157.374224841053,-224.562227675715,
-8.40993941153556E-15));
#85978=CARTESIAN_POINT('Ctrl Pts',(-157.383741679345,-224.527598988116,
-9.20313590120162E-15));
#85979=CARTESIAN_POINT('Ctrl Pts',(-157.393929021839,-224.493133887988,
-9.22030469681423E-15));
#85980=CARTESIAN_POINT('Ctrl Pts',(-157.404785975198,-224.458857230651,
-9.67281810204668E-15));
#85981=CARTESIAN_POINT('Ctrl Pts',(-157.410769888121,-224.439965325527,
-9.92222516164008E-15));
#85982=CARTESIAN_POINT('Ctrl Pts',(-157.416957228107,-224.421130681043,
-1.27377712901384E-14));
#85983=CARTESIAN_POINT('Ctrl Pts',(-157.423347951588,-224.402357585388,
-1.29757316003065E-14));
#85984=CARTESIAN_POINT('Ctrl Pts',(-157.428583915131,-224.38697665947,-1.3170694113126E-14));
#85985=CARTESIAN_POINT('Ctrl Pts',(-157.433956678714,-224.371636528744,
-1.35354925628854E-14));
#85986=CARTESIAN_POINT('Ctrl Pts',(-157.439460724043,-224.356354233907,
-1.27953203588049E-14));
#85987=CARTESIAN_POINT('Ctrl Pts',(-157.471855748141,-224.266407607404,
-8.438907038856E-15));
#85988=CARTESIAN_POINT('Ctrl Pts',(-157.508835731473,-224.178337278242,
-9.18892624322844E-15));
#85989=CARTESIAN_POINT('Ctrl Pts',(-157.550328055791,-224.092586094792,
-7.72298891504875E-15));
#85990=CARTESIAN_POINT('Ctrl Pts',(-157.581447299029,-224.028272707204,
-6.62353591891397E-15));
#85991=CARTESIAN_POINT('Ctrl Pts',(-157.615105879293,-223.965264374664,
-8.64296102576464E-15));
#85992=CARTESIAN_POINT('Ctrl Pts',(-157.651290488186,-223.90376501913,-7.66053886991358E-15));
#85993=CARTESIAN_POINT('Ctrl Pts',(-157.665717481941,-223.879244902832,
-7.26884199267624E-15));
#85994=CARTESIAN_POINT('Ctrl Pts',(-157.680546182159,-223.854964851476,
-4.75898920195301E-15));
#85995=CARTESIAN_POINT('Ctrl Pts',(-157.695776333974,-223.830938597538,
-3.14331893846997E-15));
#85996=CARTESIAN_POINT('Ctrl Pts',(-157.706205612398,-223.814485938704,
-2.03694290071405E-15));
#85997=CARTESIAN_POINT('Ctrl Pts',(-157.716818754359,-223.798159331959,
-6.56110042008239E-15));
#85998=CARTESIAN_POINT('Ctrl Pts',(-157.727611295651,-223.781968701565,
-6.58501031480796E-15));
#85999=CARTESIAN_POINT('Ctrl Pts',(-157.775201002763,-223.710576122415,
-6.69044098737037E-15));
#86000=CARTESIAN_POINT('Ctrl Pts',(-157.826299872079,-223.641787294174,
-3.28198090435521E-15));
#86001=CARTESIAN_POINT('Ctrl Pts',(-157.880874030867,-223.575954690689,
-3.53883589099269E-16));
#86002=CARTESIAN_POINT('Ctrl Pts',(-157.931842788648,-223.514471268944,
2.38077116575345E-15));
#86003=CARTESIAN_POINT('Ctrl Pts',(-157.985843340743,-223.455566244336,
-2.7573366700933E-15));
#86004=CARTESIAN_POINT('Ctrl Pts',(-158.04287080899,-223.399561029707,-6.05418493115906E-16));
#86005=CARTESIAN_POINT('Ctrl Pts',(-158.056034841079,-223.38663297126,-1.05207374013562E-16));
#86006=CARTESIAN_POINT('Ctrl Pts',(-158.069360250185,-223.373859589861,
6.80932906126852E-16));
#86007=CARTESIAN_POINT('Ctrl Pts',(-158.082843652116,-223.361242283932,
8.04911692853238E-16));
#86008=CARTESIAN_POINT('Ctrl Pts',(-162.519491502139,-225.001988389076,
18.3874166975081));
#86009=CARTESIAN_POINT('Ctrl Pts',(-162.520629418137,-225.133541932024,
18.3957515808994));
#86010=CARTESIAN_POINT('Ctrl Pts',(-162.511215066058,-225.264932196066,
18.4040864642908));
#86011=CARTESIAN_POINT('Ctrl Pts',(-162.490680057533,-225.394560699254,
18.4124213476821));
#86012=CARTESIAN_POINT('Ctrl Pts',(-162.360300544394,-226.217589387765,
18.4653406360927));
#86013=CARTESIAN_POINT('Ctrl Pts',(-161.781630713394,-226.969598857535,
18.5182599245033));
#86014=CARTESIAN_POINT('Ctrl Pts',(-161.019467989588,-227.306478092312,
18.5711792129139));
#86015=CARTESIAN_POINT('Ctrl Pts',(-160.257305265783,-227.64335732709,18.6240985013245));
#86016=CARTESIAN_POINT('Ctrl Pts',(-159.311649649173,-227.565106326875,
18.6770177897351));
#86017=CARTESIAN_POINT('Ctrl Pts',(-158.615237028698,-227.107515105334,
18.7299370781457));
#86018=CARTESIAN_POINT('Ctrl Pts',(-157.918824408224,-226.649923883792,
18.7828563665563));
#86019=CARTESIAN_POINT('Ctrl Pts',(-157.471654783884,-225.812992440923,
18.8357756549669));
#86020=CARTESIAN_POINT('Ctrl Pts',(-157.47834487994,-224.97973719714,18.8886949433775));
#86021=CARTESIAN_POINT('Ctrl Pts',(-157.485034975996,-224.146481953356,
18.9416142317881));
#86022=CARTESIAN_POINT('Ctrl Pts',(-157.945584792449,-223.316902908658,
18.9945335201987));
#86023=CARTESIAN_POINT('Ctrl Pts',(-158.649263524052,-222.87053945485,19.0474528086093));
#86024=CARTESIAN_POINT('Ctrl Pts',(-159.352942255656,-222.424176001043,
19.1003720970199));
#86025=CARTESIAN_POINT('Ctrl Pts',(-160.29974990241,-222.361028138127,19.1532913854305));
#86026=CARTESIAN_POINT('Ctrl Pts',(-161.056392494181,-222.710149965623,
19.2062106738411));
#86027=CARTESIAN_POINT('Ctrl Pts',(-161.813035085951,-223.059271793118,
19.2591299622517));
#86028=CARTESIAN_POINT('Ctrl Pts',(-162.379512622738,-223.820663311025,
19.3120492506623));
#86029=CARTESIAN_POINT('Ctrl Pts',(-162.496677361246,-224.645584781132,
19.3649685390729));
#86030=CARTESIAN_POINT('Ctrl Pts',(-162.513244304932,-224.762227618515,
19.3724512585513));
#86031=CARTESIAN_POINT('Ctrl Pts',(-162.520827869545,-224.880140648168,
19.3799339780297));
#86032=CARTESIAN_POINT('Ctrl Pts',(-162.519857325378,-224.99817643576,19.3874166975081));
#86033=CARTESIAN_POINT('Ctrl Pts',(-160.793799282533,-227.969222953746,
20.));
#86034=CARTESIAN_POINT('Ctrl Pts',(-161.781070948697,-227.70528334649,19.9470807115894));
#86035=CARTESIAN_POINT('Ctrl Pts',(-163.454303791657,-226.117971486511,
19.8412421347682));
#86036=CARTESIAN_POINT('Ctrl Pts',(-162.813708830336,-222.699008736782,
19.6824842695364));
#86037=CARTESIAN_POINT('Ctrl Pts',(-159.592724505823,-221.390669564417,
19.5237264043046));
#86038=CARTESIAN_POINT('Ctrl Pts',(-156.746988377721,-223.383220985595,
19.3649685390728));
#86039=CARTESIAN_POINT('Ctrl Pts',(-156.877197897433,-226.856577363582,
19.206210673841));
#86040=CARTESIAN_POINT('Ctrl Pts',(-159.865978935642,-228.630249528,19.0474528086092));
#86041=CARTESIAN_POINT('Ctrl Pts',(-162.977135003112,-227.081779887678,
18.8886949433775));
#86042=CARTESIAN_POINT('Ctrl Pts',(-163.363752671914,-223.627938905832,
18.7299370781457));
#86043=CARTESIAN_POINT('Ctrl Pts',(-160.671798756939,-221.429869131324,
18.5711792129139));
#86044=CARTESIAN_POINT('Ctrl Pts',(-157.365046101209,-222.499153615461,
18.4124213476821));
#86045=CARTESIAN_POINT('Ctrl Pts',(-156.469787991194,-225.857226767288,
18.2536634824503));
#86046=CARTESIAN_POINT('Ctrl Pts',(-158.805387078146,-228.430759193889,
18.0949056172185));
#86047=CARTESIAN_POINT('Ctrl Pts',(-162.234292343626,-227.864464228569,
17.9361477519867));
#86048=CARTESIAN_POINT('Ctrl Pts',(-163.618375040713,-224.676610129639,
17.7773898867549));
#86049=CARTESIAN_POINT('Ctrl Pts',(-161.690920225189,-221.784723190834,
17.6186320215231));
#86050=CARTESIAN_POINT('Ctrl Pts',(-158.215935680102,-221.835457093401,
17.4598741562913));
#86051=CARTESIAN_POINT('Ctrl Pts',(-156.373726540536,-224.782380716962,
17.3011162910595));
#86052=CARTESIAN_POINT('Ctrl Pts',(-157.850282819984,-227.928469414349,
17.1423584258277));
#86053=CARTESIAN_POINT('Ctrl Pts',(-161.294260133946,-228.394423060065,
16.9836005605959));
#86054=CARTESIAN_POINT('Ctrl Pts',(-163.553730645469,-225.753800834845,
16.8248426953641));
#86055=CARTESIAN_POINT('Ctrl Pts',(-162.560826999764,-222.423300124782,
16.6660848301324));
#86056=CARTESIAN_POINT('Ctrl Pts',(-159.224254589513,-221.450995034583,
16.5073269649006));
#86057=CARTESIAN_POINT('Ctrl Pts',(-156.597644346055,-223.726739151393,
16.3485690996688));
#86058=CARTESIAN_POINT('Ctrl Pts',(-157.08486986444,-227.167771545708,16.189811234437));
#86059=CARTESIAN_POINT('Ctrl Pts',(-160.240022367702,-228.624859507152,
16.0310533692052));
#86060=CARTESIAN_POINT('Ctrl Pts',(-163.175506409748,-226.764476189946,
15.8722955039734));
#86061=CARTESIAN_POINT('Ctrl Pts',(-163.204767110338,-223.289244333207,
15.7135376387416));
#86062=CARTESIAN_POINT('Ctrl Pts',(-160.301025077633,-221.379695995386,
15.5547797735098));
#86063=CARTESIAN_POINT('Ctrl Pts',(-157.121784905686,-222.78344974025,15.396021908278));
#86064=CARTESIAN_POINT('Ctrl Pts',(-156.576687074886,-226.21579019566,15.2372640430462));
#86065=CARTESIAN_POINT('Ctrl Pts',(-159.164605098526,-228.535439511819,
15.0785061778144));
#86066=CARTESIAN_POINT('Ctrl Pts',(-162.517076503146,-227.619454725785,
14.9197483125826));
#86067=CARTESIAN_POINT('Ctrl Pts',(-163.565919591067,-224.306145077722,
14.7609904473508));
#86068=CARTESIAN_POINT('Ctrl Pts',(-161.351233209471,-221.627851427242,
14.6022325821191));
#86069=CARTESIAN_POINT('Ctrl Pts',(-157.899898247702,-222.035748017944,
14.4434747168873));
#86070=CARTESIAN_POINT('Ctrl Pts',(-156.370576327052,-225.156527906056,
14.2847168516555));
#86071=CARTESIAN_POINT('Ctrl Pts',(-158.16290280916,-228.134053460702,14.1259589864237));
#86072=CARTESIAN_POINT('Ctrl Pts',(-161.636540568083,-228.243293411356,
13.9672011211919));
#86073=CARTESIAN_POINT('Ctrl Pts',(-163.612416463452,-225.384271359477,
13.8084432559601));
#86074=CARTESIAN_POINT('Ctrl Pts',(-162.282208953524,-222.173564174515,
13.6496853907283));
#86075=CARTESIAN_POINT('Ctrl Pts',(-158.863323899077,-221.54961094589,13.4909275254965));
#86076=CARTESIAN_POINT('Ctrl Pts',(-156.484724767496,-224.083453643903,
13.3321696602647));
#86077=CARTESIAN_POINT('Ctrl Pts',(-157.323305390468,-227.456119530974,
13.1734117950329));
#86078=CARTESIAN_POINT('Ctrl Pts',(-160.611596814825,-228.580944919882,
13.0146539298011));
#86079=CARTESIAN_POINT('Ctrl Pts',(-163.340154858305,-226.428489658931,
12.8558960645694));
#86080=CARTESIAN_POINT('Ctrl Pts',(-163.011803306812,-222.968680718301,
12.6971381993375));
#86081=CARTESIAN_POINT('Ctrl Pts',(-159.927049487362,-221.367935104402,
12.5383803341058));
#86082=CARTESIAN_POINT('Ctrl Pts',(-156.909059974209,-223.091255140127,
12.379622468874));
#86083=CARTESIAN_POINT('Ctrl Pts',(-156.719898651112,-226.561458396548,
12.2208646036422));
#86084=CARTESIAN_POINT('Ctrl Pts',(-159.53268595353,-228.602614989851,12.0621067384104));
#86085=CARTESIAN_POINT('Ctrl Pts',(-162.773159052901,-227.346658486112,
11.9033488731786));
#86086=CARTESIAN_POINT('Ctrl Pts',(-163.475637096109,-223.943040228163,
11.7445910079468));
#86087=CARTESIAN_POINT('Ctrl Pts',(-160.997212205634,-221.506751511835,
11.585833142715));
#86088=CARTESIAN_POINT('Ctrl Pts',(-157.606138743777,-222.267483674507,
11.4270752774832));
#86089=CARTESIAN_POINT('Ctrl Pts',(-156.405927009479,-225.529014670817,
11.2683174122514));
#86090=CARTESIAN_POINT('Ctrl Pts',(-158.495010734773,-228.306391461198,
11.1095595470196));
#86091=CARTESIAN_POINT('Ctrl Pts',(-161.96146057642,-228.057758916311,10.9508016817878));
#86092=CARTESIAN_POINT('Ctrl Pts',(-163.63278177566,-225.01066553146,10.792043816556));
#86093=CARTESIAN_POINT('Ctrl Pts',(-161.979381236672,-221.953811052636,
10.6332859513243));
#86094=CARTESIAN_POINT('Ctrl Pts',(-158.514451067719,-221.684828578651,
10.4745280860924));
#86095=CARTESIAN_POINT('Ctrl Pts',(-156.409095223172,-224.449890859119,
10.3157702208607));
#86096=CARTESIAN_POINT('Ctrl Pts',(-157.590135289169,-227.718413003688,
10.1570123556289));
#86097=CARTESIAN_POINT('Ctrl Pts',(-160.976683443753,-228.499043674182,
9.99825449039708));
#86098=CARTESIAN_POINT('Ctrl Pts',(-163.469370949022,-226.07734971166,9.83949662516527));
#86099=CARTESIAN_POINT('Ctrl Pts',(-162.786890298175,-222.669665335394,
9.6807387599335));
#86100=CARTESIAN_POINT('Ctrl Pts',(-159.553847756031,-221.394703152536,
9.5219808947017));
#86101=CARTESIAN_POINT('Ctrl Pts',(-156.729123730022,-223.419308502703,
9.3632230294699));
#86102=CARTESIAN_POINT('Ctrl Pts',(-156.897905537673,-226.890562649037,
9.20446516423812));
#86103=CARTESIAN_POINT('Ctrl Pts',(-159.905724075259,-228.631573933316,
9.04570729900632));
#86104=CARTESIAN_POINT('Ctrl Pts',(-162.99982393546,-227.048968896633,8.88694943377453));
#86105=CARTESIAN_POINT('Ctrl Pts',(-163.348485047893,-223.591147606325,
8.72819156854274));
#86106=CARTESIAN_POINT('Ctrl Pts',(-160.632612776171,-221.422707971306,
8.56943370331094));
#86107=CARTESIAN_POINT('Ctrl Pts',(-157.337773316573,-222.528205860274,
8.41067583807916));
#86108=CARTESIAN_POINT('Ctrl Pts',(-156.479403612958,-225.895889648718,
8.25191797284736));
#86109=CARTESIAN_POINT('Ctrl Pts',(-158.84308358432,-228.443655265885,8.09316010761556));
#86110=CARTESIAN_POINT('Ctrl Pts',(-162.265573413817,-227.839787719132,
7.93440224238377));
#86111=CARTESIAN_POINT('Ctrl Pts',(-163.61461054408,-224.636946563501,7.77564437715198));
#86112=CARTESIAN_POINT('Ctrl Pts',(-161.655556246542,-221.766371898677,
7.61688651192019));
#86113=CARTESIAN_POINT('Ctrl Pts',(-158.181336937272,-221.855213545024,
7.4581286466884));
#86114=CARTESIAN_POINT('Ctrl Pts',(-156.371557991493,-224.822163631299,
7.29937078145661));
#86115=CARTESIAN_POINT('Ctrl Pts',(-157.882529029215,-227.951869555216,
7.14061291622481));
#86116=CARTESIAN_POINT('Ctrl Pts',(-161.331409416131,-228.380024578279,
6.98185505099302));
#86117=CARTESIAN_POINT('Ctrl Pts',(-163.561783957761,-225.714781240217,
6.82309718576123));
#86118=CARTESIAN_POINT('Ctrl Pts',(-162.532413961312,-222.395370139217,
6.66433932052944));
#86119=CARTESIAN_POINT('Ctrl Pts',(-159.185378807054,-221.459716184381,
6.50558145529764));
#86120=CARTESIAN_POINT('Ctrl Pts',(-156.583884936547,-223.764129838381,
6.34682359006585));
#86121=CARTESIAN_POINT('Ctrl Pts',(-157.108819437776,-227.199611815696,
6.18806572483406));
#86122=CARTESIAN_POINT('Ctrl Pts',(-160.27976227586,-228.622009145783,6.02930785960227));
#86123=CARTESIAN_POINT('Ctrl Pts',(-163.194666690078,-226.729543848082,
5.87054999437047));
#86124=CARTESIAN_POINT('Ctrl Pts',(-163.185812275164,-223.254200088628,
5.71179212913868));
#86125=CARTESIAN_POINT('Ctrl Pts',(-160.261302591299,-221.376612339411,
5.55303426390689));
#86126=CARTESIAN_POINT('Ctrl Pts',(-157.097648786153,-222.815148834678,
5.3942763986751));
#86127=CARTESIAN_POINT('Ctrl Pts',(-156.590226697787,-226.253261030531,
5.2355185334433));
#86128=CARTESIAN_POINT('Ctrl Pts',(-159.203429001521,-228.544388780525,
5.07676066821151));
#86129=CARTESIAN_POINT('Ctrl Pts',(-162.545653051738,-227.591692057962,
4.91800280297972));
#86130=CARTESIAN_POINT('Ctrl Pts',(-163.55809552911,-224.267078865869,4.75924493774792));
#86131=CARTESIAN_POINT('Ctrl Pts',(-161.314169118159,-221.613235066909,
4.60048707251614));
#86132=CARTESIAN_POINT('Ctrl Pts',(-157.867515181948,-222.058958401537,
4.44172920728434));
#86133=CARTESIAN_POINT('Ctrl Pts',(-156.372511267358,-225.196322891415,
4.28297134205255));
#86134=CARTESIAN_POINT('Ctrl Pts',(-158.197384898239,-228.15401267881,4.12421347682076));
#86135=CARTESIAN_POINT('Ctrl Pts',(-161.672011799357,-228.225150186546,
3.96545561158896));
#86136=CARTESIAN_POINT('Ctrl Pts',(-163.616413567471,-225.344630370464,
3.80669774635717));
#86137=CARTESIAN_POINT('Ctrl Pts',(-162.251073780811,-222.148704852714,
3.64793988112538));
#86138=CARTESIAN_POINT('Ctrl Pts',(-158.825551358552,-221.562284541991,
3.48918201589359));
#86139=CARTESIAN_POINT('Ctrl Pts',(-156.474884286599,-224.122061282515,
3.3304241506618));
#86140=CARTESIAN_POINT('Ctrl Pts',(-157.350402977267,-227.485327504289,
3.17166628543));
#86141=CARTESIAN_POINT('Ctrl Pts',(-160.650832758246,-228.574022088692,
3.01290842019821));
#86142=CARTESIAN_POINT('Ctrl Pts',(-163.355620425927,-226.391771804664,
2.85415055496642));
#86143=CARTESIAN_POINT('Ctrl Pts',(-162.989344408734,-222.935772006054,
2.69539268973463));
#86144=CARTESIAN_POINT('Ctrl Pts',(-159.887220512494,-221.368953614723,
2.53663482450283));
#86145=CARTESIAN_POINT('Ctrl Pts',(-156.888312385766,-223.125268673492,
2.37787695927104));
#86146=CARTESIAN_POINT('Ctrl Pts',(-156.737220668234,-226.597337890817,
2.21911909403925));
#86147=CARTESIAN_POINT('Ctrl Pts',(-159.572224410776,-228.60752327959,2.06036122880746));
#86148=CARTESIAN_POINT('Ctrl Pts',(-162.798728472064,-227.316104031162,
1.90160336357566));
#86149=CARTESIAN_POINT('Ctrl Pts',(-163.46383610443,-223.904985372157,1.74284549834387));
#86150=CARTESIAN_POINT('Ctrl Pts',(-160.958841571036,-221.496026324134,
1.58408763311208));
#86151=CARTESIAN_POINT('Ctrl Pts',(-157.576314230351,-222.293899143107,
1.42532976788029));
#86152=CARTESIAN_POINT('Ctrl Pts',(-156.411946167088,-225.568405119559,
1.2665719026485));
#86153=CARTESIAN_POINT('Ctrl Pts',(-158.531360356103,-228.322686501262,
1.1078140374167));
#86154=CARTESIAN_POINT('Ctrl Pts',(-161.994882774227,-228.036087350692,
0.94905617218491));
#86155=CARTESIAN_POINT('Ctrl Pts',(-163.632669289527,-224.970773976824,
0.790298306953122));
#86156=CARTESIAN_POINT('Ctrl Pts',(-161.945876991572,-221.932389200875,
0.631540441721325));
#86157=CARTESIAN_POINT('Ctrl Pts',(-158.478135184779,-221.701106251642,
0.472782576489533));
#86158=CARTESIAN_POINT('Ctrl Pts',(-156.403376046572,-224.489749930199,
0.314024711257741));
#86159=CARTESIAN_POINT('Ctrl Pts',(-157.619888902649,-227.743758496233,
0.155266846025946));
#86160=CARTESIAN_POINT('Ctrl Pts',(-161.015405968821,-228.490052849714,
-0.00349101920584225));
#86161=CARTESIAN_POINT('Ctrl Pts',(-163.47996393464,-226.035338564583,-0.162248884437638));
#86162=CARTESIAN_POINT('Ctrl Pts',(-163.000168811616,-223.779443237332,
-0.268087461258832));
#86163=CARTESIAN_POINT('Ctrl Pts',(-162.336062657696,-223.002698443069,
-0.32100674966943));
#86164=CARTESIAN_POINT('Ctrl Pts',(-160.745932854347,-227.790177569842,
20.1070022498898));
#86165=CARTESIAN_POINT('Ctrl Pts',(-161.673671626808,-227.542153631111,
20.0540829614792));
#86166=CARTESIAN_POINT('Ctrl Pts',(-163.246007830683,-226.050557339068,
19.948244384658));
#86167=CARTESIAN_POINT('Ctrl Pts',(-162.644041013008,-222.837759470728,
19.7894865194262));
#86168=CARTESIAN_POINT('Ctrl Pts',(-159.617283388179,-221.608313696751,
19.6307286541944));
#86169=CARTESIAN_POINT('Ctrl Pts',(-156.943146336833,-223.480713435247,
19.4719707889626));
#86170=CARTESIAN_POINT('Ctrl Pts',(-157.065504168138,-226.744624973348,
19.3132129237308));
#86171=CARTESIAN_POINT('Ctrl Pts',(-159.874060461782,-228.411343965659,
19.1544550584991));
#86172=CARTESIAN_POINT('Ctrl Pts',(-162.797612519329,-226.956247691209,
18.9956971932673));
#86173=CARTESIAN_POINT('Ctrl Pts',(-163.16091698127,-223.710674762712,18.8369393280355));
#86174=CARTESIAN_POINT('Ctrl Pts',(-160.631289011388,-221.645149513406,
18.6781814628037));
#86175=CARTESIAN_POINT('Ctrl Pts',(-157.523934921525,-222.649955696672,
18.5194235975719));
#86176=CARTESIAN_POINT('Ctrl Pts',(-156.682661249357,-225.805535635287,
18.3606657323401));
#86177=CARTESIAN_POINT('Ctrl Pts',(-158.877422736142,-228.223882981991,
18.2019078671083));
#86178=CARTESIAN_POINT('Ctrl Pts',(-162.099563582381,-227.691735839536,
18.0431500018765));
#86179=CARTESIAN_POINT('Ctrl Pts',(-163.400185514913,-224.696110673852,
17.8843921366447));
#86180=CARTESIAN_POINT('Ctrl Pts',(-161.58895702957,-221.978605724959,17.7256342714129));
#86181=CARTESIAN_POINT('Ctrl Pts',(-158.323515503524,-222.026280352017,
17.5668764061811));
#86182=CARTESIAN_POINT('Ctrl Pts',(-156.592392344284,-224.795503250595,
17.4081185409494));
#86183=CARTESIAN_POINT('Ctrl Pts',(-157.979911663549,-227.751881485888,
17.2493606757175));
#86184=CARTESIAN_POINT('Ctrl Pts',(-161.216215707453,-228.189737932209,
17.0906028104858));
#86185=CARTESIAN_POINT('Ctrl Pts',(-163.339439203695,-225.708346329756,
16.931844945254));
#86186=CARTESIAN_POINT('Ctrl Pts',(-162.40640806241,-222.578676203153,16.7730870800222));
#86187=CARTESIAN_POINT('Ctrl Pts',(-159.271032361676,-221.665001515877,
16.6143292147904));
#86188=CARTESIAN_POINT('Ctrl Pts',(-156.802807812634,-223.803517312212,
16.4555713495586));
#86189=CARTESIAN_POINT('Ctrl Pts',(-157.260653428821,-227.037054016354,
16.2968134843268));
#86190=CARTESIAN_POINT('Ctrl Pts',(-160.225548918709,-228.406278965319,
16.138055619095));
#86191=CARTESIAN_POINT('Ctrl Pts',(-162.984022047315,-226.658077538939,
15.9792977538632));
#86192=CARTESIAN_POINT('Ctrl Pts',(-163.011518315441,-223.392403614237,
15.8205398886314));
#86193=CARTESIAN_POINT('Ctrl Pts',(-160.282873139759,-221.598001838514,
15.6617820233996));
#86194=CARTESIAN_POINT('Ctrl Pts',(-157.295342477666,-222.917108646428,
15.5030241581678));
#86195=CARTESIAN_POINT('Ctrl Pts',(-156.783114273668,-226.142477539211,
15.344266292936));
#86196=CARTESIAN_POINT('Ctrl Pts',(-159.214979759902,-228.322251033041,
15.1855084277042));
#86197=CARTESIAN_POINT('Ctrl Pts',(-162.365295739007,-227.461500512073,
15.0267505624725));
#86198=CARTESIAN_POINT('Ctrl Pts',(-163.350893150784,-224.347984819253,
14.8679926972406));
#86199=CARTESIAN_POINT('Ctrl Pts',(-161.269753282735,-221.831193394213,
14.7092348320089));
#86200=CARTESIAN_POINT('Ctrl Pts',(-158.026535260259,-222.214493650178,
14.5504769667771));
#86201=CARTESIAN_POINT('Ctrl Pts',(-156.589432089989,-225.147089207964,
14.3917191015453));
#86202=CARTESIAN_POINT('Ctrl Pts',(-158.273680536844,-227.945068728404,
14.2329612363135));
#86203=CARTESIAN_POINT('Ctrl Pts',(-161.537856488493,-228.047721464422,
14.0742033710817));
#86204=CARTESIAN_POINT('Ctrl Pts',(-163.394586242349,-225.361099636049,
13.9154455058499));
#86205=CARTESIAN_POINT('Ctrl Pts',(-162.144590800695,-222.343999434964,
13.7566876406181));
#86206=CARTESIAN_POINT('Ctrl Pts',(-158.93186594258,-221.757670846556,13.5979297753863));
#86207=CARTESIAN_POINT('Ctrl Pts',(-156.696697331812,-224.138721771878,
13.4391719101545));
#86208=CARTESIAN_POINT('Ctrl Pts',(-157.484711193071,-227.308014497709,
13.2804140449227));
#86209=CARTESIAN_POINT('Ctrl Pts',(-160.57471727152,-228.365012445997,13.1216561796909));
#86210=CARTESIAN_POINT('Ctrl Pts',(-163.138742125675,-226.342351136035,
12.9628983144591));
#86211=CARTESIAN_POINT('Ctrl Pts',(-162.83019030984,-223.09117011916,12.8041404492274));
#86212=CARTESIAN_POINT('Ctrl Pts',(-159.931448433734,-221.586950134167,
12.6453825839956));
#86213=CARTESIAN_POINT('Ctrl Pts',(-157.095444948379,-223.206353252169,
12.4866247187638));
#86214=CARTESIAN_POINT('Ctrl Pts',(-156.917690132049,-226.467301803253,
12.327866853532));
#86215=CARTESIAN_POINT('Ctrl Pts',(-159.560865185658,-228.385375801699,
12.1691089883002));
#86216=CARTESIAN_POINT('Ctrl Pts',(-162.605936404085,-227.205153999557,
12.0103511230684));
#86217=CARTESIAN_POINT('Ctrl Pts',(-163.266054727969,-224.006775343736,
11.8515932578366));
#86218=CARTESIAN_POINT('Ctrl Pts',(-160.93707989325,-221.71739585427,11.6928353926048));
#86219=CARTESIAN_POINT('Ctrl Pts',(-157.750489577079,-222.432255549891,
11.534077527373));
#86220=CARTESIAN_POINT('Ctrl Pts',(-156.622651111505,-225.497114865277,
11.3753196621412));
#86221=CARTESIAN_POINT('Ctrl Pts',(-158.585762215871,-228.107014675511,
11.2165617969094));
#86222=CARTESIAN_POINT('Ctrl Pts',(-161.843183684658,-227.873374776897,
11.0578039316776));
#86223=CARTESIAN_POINT('Ctrl Pts',(-163.413723517728,-225.01002239546,10.8990460664458));
#86224=CARTESIAN_POINT('Ctrl Pts',(-161.860023721614,-222.137497518092,
10.7402882012141));
#86225=CARTESIAN_POINT('Ctrl Pts',(-158.604030288623,-221.884734799601,
10.5815303359823));
#86226=CARTESIAN_POINT('Ctrl Pts',(-156.625628280589,-224.483062670011,
10.4227724707505));
#86227=CARTESIAN_POINT('Ctrl Pts',(-157.735451137466,-227.554491564498,
10.2640146055187));
#86228=CARTESIAN_POINT('Ctrl Pts',(-160.917789024283,-228.28804987961,10.1052567402869));
#86229=CARTESIAN_POINT('Ctrl Pts',(-163.260166432167,-226.012385074202,
9.94649887505509));
#86230=CARTESIAN_POINT('Ctrl Pts',(-162.618839649535,-222.810185488696,
9.78774100982331));
#86231=CARTESIAN_POINT('Ctrl Pts',(-159.580750922632,-221.612104057822,
9.62898314459151));
#86232=CARTESIAN_POINT('Ctrl Pts',(-156.926358934849,-223.514624860004,
9.47022527935972));
#86233=CARTESIAN_POINT('Ctrl Pts',(-157.084963129025,-226.776560931899,
9.31146741412793));
#86234=CARTESIAN_POINT('Ctrl Pts',(-159.911408952885,-228.412588508782,
9.15270954889613));
#86235=CARTESIAN_POINT('Ctrl Pts',(-162.818933299582,-226.925415216624,
8.99395168366434));
#86236=CARTESIAN_POINT('Ctrl Pts',(-163.146570001353,-223.676101993927,
8.83519381843255));
#86237=CARTESIAN_POINT('Ctrl Pts',(-160.594465961621,-221.638420174327,
8.67643595320076));
#86238=CARTESIAN_POINT('Ctrl Pts',(-157.498306697191,-222.677256078992,
8.51767808796897));
#86239=CARTESIAN_POINT('Ctrl Pts',(-156.691697045115,-225.841867128824,
8.35892022273717));
#86240=CARTESIAN_POINT('Ctrl Pts',(-158.912846127253,-228.236001415462,
8.20016235750538));
#86241=CARTESIAN_POINT('Ctrl Pts',(-162.128958390979,-227.668547333921,
8.04140449227359));
#86242=CARTESIAN_POINT('Ctrl Pts',(-163.396648018999,-224.658838837315,
7.88264662704179));
#86243=CARTESIAN_POINT('Ctrl Pts',(-161.555725513602,-221.961361023381,
7.72388876181));
#86244=CARTESIAN_POINT('Ctrl Pts',(-158.291003079333,-222.044845481358,
7.56513089657821));
#86245=CARTESIAN_POINT('Ctrl Pts',(-156.590354559654,-224.832887238587,
7.40637303134642));
#86246=CARTESIAN_POINT('Ctrl Pts',(-158.010213412898,-227.77387058849,7.24761516611462));
#86247=CARTESIAN_POINT('Ctrl Pts',(-161.251124872411,-228.176207684886,
7.08885730088284));
#86248=CARTESIAN_POINT('Ctrl Pts',(-163.347006897893,-225.671679632976,
6.93009943565103));
#86249=CARTESIAN_POINT('Ctrl Pts',(-162.37970834204,-222.552430407379,6.77134157041925));
#86250=CARTESIAN_POINT('Ctrl Pts',(-159.234500805133,-221.673196776701,
6.61258370518745));
#86251=CARTESIAN_POINT('Ctrl Pts',(-156.789878101265,-223.838653325162,
6.45382583995566));
#86252=CARTESIAN_POINT('Ctrl Pts',(-157.283158832885,-227.066974304766,
6.29506797472387));
#86253=CARTESIAN_POINT('Ctrl Pts',(-160.262892493811,-228.40360048193,6.13631010949208));
#86254=CARTESIAN_POINT('Ctrl Pts',(-163.00202695474,-226.625251631875,5.97755224426028));
#86255=CARTESIAN_POINT('Ctrl Pts',(-162.993706464743,-223.359472552239,
5.81879437902849));
#86256=CARTESIAN_POINT('Ctrl Pts',(-160.245545935937,-221.595104128282,
5.6600365137967));
#86257=CARTESIAN_POINT('Ctrl Pts',(-157.272661776218,-222.946896272227,
5.50127864856491));
#86258=CARTESIAN_POINT('Ctrl Pts',(-156.795837451654,-226.177688867093,
5.34252078333311));
#86259=CARTESIAN_POINT('Ctrl Pts',(-159.251462565336,-228.330660657108,
5.18376291810132));
#86260=CARTESIAN_POINT('Ctrl Pts',(-162.392149109786,-227.435411944712,
5.02500505286953));
#86261=CARTESIAN_POINT('Ctrl Pts',(-163.34354088303,-224.311274316287,4.86624718763774));
#86262=CARTESIAN_POINT('Ctrl Pts',(-161.234924171605,-221.817458406511,
4.70748932240595));
#86263=CARTESIAN_POINT('Ctrl Pts',(-157.996104906891,-222.23630443795,4.54873145717415));
#86264=CARTESIAN_POINT('Ctrl Pts',(-156.591250352587,-225.184484539089,
4.38997359194236));
#86265=CARTESIAN_POINT('Ctrl Pts',(-158.306083341553,-227.963824397327,
4.23121572671057));
#86266=CARTESIAN_POINT('Ctrl Pts',(-161.57118878971,-228.030672283643,4.07245786147877));
#86267=CARTESIAN_POINT('Ctrl Pts',(-163.398342319327,-225.323849015226,
3.91369999624698));
#86268=CARTESIAN_POINT('Ctrl Pts',(-162.115333091897,-222.320639140647,
3.75494213101519));
#86269=CARTESIAN_POINT('Ctrl Pts',(-158.89637110202,-221.76958021952,3.5961842657834));
#86270=CARTESIAN_POINT('Ctrl Pts',(-156.687450236022,-224.175001353761,
3.4374264005516));
#86271=CARTESIAN_POINT('Ctrl Pts',(-157.510174784072,-227.335461218037,
3.27866853531981));
#86272=CARTESIAN_POINT('Ctrl Pts',(-160.611587271169,-228.358507064419,
3.11991067008802));
#86273=CARTESIAN_POINT('Ctrl Pts',(-163.153275113112,-226.307847383712,
2.96115280485622));
#86274=CARTESIAN_POINT('Ctrl Pts',(-162.809085692693,-223.060245816003,
2.80239493962444));
#86275=CARTESIAN_POINT('Ctrl Pts',(-159.894021162681,-221.587907227891,
2.64363707439264));
#86276=CARTESIAN_POINT('Ctrl Pts',(-157.075948448183,-223.23831575527,2.48487920916085));
#86277=CARTESIAN_POINT('Ctrl Pts',(-156.933967624306,-226.501017749036,
2.32612134392906));
#86278=CARTESIAN_POINT('Ctrl Pts',(-159.598019457423,-228.389988119517,
2.16736347869727));
#86279=CARTESIAN_POINT('Ctrl Pts',(-162.629963976595,-227.176441990998,
2.00860561346547));
#86280=CARTESIAN_POINT('Ctrl Pts',(-163.254965341015,-223.971015211437,
1.84984774823368));
#86281=CARTESIAN_POINT('Ctrl Pts',(-160.90102302394,-221.707317399865,1.69108988300189));
#86282=CARTESIAN_POINT('Ctrl Pts',(-157.722463494266,-222.457078154705,
1.5323320177701));
#86283=CARTESIAN_POINT('Ctrl Pts',(-156.628307311397,-225.534130053513,
1.37357415253831));
#86284=CARTESIAN_POINT('Ctrl Pts',(-158.619919939858,-228.122327117855,
1.21481628730651));
#86285=CARTESIAN_POINT('Ctrl Pts',(-161.874590509982,-227.853010015733,
1.05605842207472));
#86286=CARTESIAN_POINT('Ctrl Pts',(-163.413617814555,-224.972536318225,
0.897300556842931));
#86287=CARTESIAN_POINT('Ctrl Pts',(-161.828539796483,-222.117367412936,
0.738542691611136));
#86288=CARTESIAN_POINT('Ctrl Pts',(-158.569904268588,-221.900030922114,
0.579784826379343));
#86289=CARTESIAN_POINT('Ctrl Pts',(-156.620253972727,-224.520518222462,
0.421026961147552));
#86290=CARTESIAN_POINT('Ctrl Pts',(-157.76341059563,-227.57830871326,0.262269095915756));
#86291=CARTESIAN_POINT('Ctrl Pts',(-160.954176564921,-228.279601205613,
0.103511230683968));
#86292=CARTESIAN_POINT('Ctrl Pts',(-163.270120656329,-225.972907216835,
-0.055246634547828));
#86293=CARTESIAN_POINT('Ctrl Pts',(-162.819257379562,-223.853043319762,
-0.161085211369022));
#86294=CARTESIAN_POINT('Ctrl Pts',(-162.195197104019,-223.123136560921,
-0.21400449977962));
#86295=CARTESIAN_POINT('Ctrl Pts',(-160.698066426161,-227.611132185939,
20.2140044997796));
#86296=CARTESIAN_POINT('Ctrl Pts',(-161.56627230492,-227.379023915733,20.161085211369));
#86297=CARTESIAN_POINT('Ctrl Pts',(-163.037711869709,-225.983143191625,
20.0552466345478));
#86298=CARTESIAN_POINT('Ctrl Pts',(-162.474373195681,-222.976510204674,
19.896488769316));
#86299=CARTESIAN_POINT('Ctrl Pts',(-159.641842270535,-221.825957829085,
19.7377309040843));
#86300=CARTESIAN_POINT('Ctrl Pts',(-157.139304295944,-223.578205884898,
19.5789730388525));
#86301=CARTESIAN_POINT('Ctrl Pts',(-157.253810438842,-226.632672583114,
19.4202151736207));
#86302=CARTESIAN_POINT('Ctrl Pts',(-159.882141987924,-228.192438403318,
19.2614573083889));
#86303=CARTESIAN_POINT('Ctrl Pts',(-162.618090035545,-226.830715494739,
19.1026994431571));
#86304=CARTESIAN_POINT('Ctrl Pts',(-162.958081290626,-223.793410619591,
18.9439415779253));
#86305=CARTESIAN_POINT('Ctrl Pts',(-160.590779265836,-221.860429895488,
18.7851837126935));
#86306=CARTESIAN_POINT('Ctrl Pts',(-157.682823741842,-222.800757777882,
18.6264258474617));
#86307=CARTESIAN_POINT('Ctrl Pts',(-156.895534507521,-225.753844503286,
18.4676679822299));
#86308=CARTESIAN_POINT('Ctrl Pts',(-158.949458394138,-228.017006770093,
18.3089101169981));
#86309=CARTESIAN_POINT('Ctrl Pts',(-161.964834821137,-227.519007450502,
18.1501522517663));
#86310=CARTESIAN_POINT('Ctrl Pts',(-163.181995989113,-224.715611218066,
17.9913943865345));
#86311=CARTESIAN_POINT('Ctrl Pts',(-161.486993833951,-222.172488259083,
17.8326365213027));
#86312=CARTESIAN_POINT('Ctrl Pts',(-158.431095326946,-222.217103610633,
17.6738786560709));
#86313=CARTESIAN_POINT('Ctrl Pts',(-156.811058148032,-224.808625784229,
17.5151207908392));
#86314=CARTESIAN_POINT('Ctrl Pts',(-158.109540507114,-227.575293557426,
17.3563629256073));
#86315=CARTESIAN_POINT('Ctrl Pts',(-161.138171280961,-227.985052804353,
17.1976050603756));
#86316=CARTESIAN_POINT('Ctrl Pts',(-163.12514776192,-225.662891824667,17.0388471951438));
#86317=CARTESIAN_POINT('Ctrl Pts',(-162.251989125057,-222.734052281524,
16.880089329912));
#86318=CARTESIAN_POINT('Ctrl Pts',(-159.317810133839,-221.879007997171,
16.7213314646802));
#86319=CARTESIAN_POINT('Ctrl Pts',(-157.007971279214,-223.88029547303,16.5625735994484));
#86320=CARTESIAN_POINT('Ctrl Pts',(-157.436436993201,-226.906336486999,
16.4038157342166));
#86321=CARTESIAN_POINT('Ctrl Pts',(-160.211075469716,-228.187698423485,
16.2450578689848));
#86322=CARTESIAN_POINT('Ctrl Pts',(-162.792537684881,-226.551678887932,
16.086300003753));
#86323=CARTESIAN_POINT('Ctrl Pts',(-162.818269520544,-223.495562895267,
15.9275421385212));
#86324=CARTESIAN_POINT('Ctrl Pts',(-160.264721201885,-221.816307681643,
15.7687842732894));
#86325=CARTESIAN_POINT('Ctrl Pts',(-157.468900049645,-223.050767552607,
15.6100264080577));
#86326=CARTESIAN_POINT('Ctrl Pts',(-156.989541472449,-226.069164882762,
15.4512685428258));
#86327=CARTESIAN_POINT('Ctrl Pts',(-159.265354421278,-228.109062554263,
15.2925106775941));
#86328=CARTESIAN_POINT('Ctrl Pts',(-162.213514974867,-227.30354629836,15.1337528123623));
#86329=CARTESIAN_POINT('Ctrl Pts',(-163.135866710501,-224.389824560784,
14.9749949471305));
#86330=CARTESIAN_POINT('Ctrl Pts',(-161.188273356,-222.034535361183,14.8162370818987));
#86331=CARTESIAN_POINT('Ctrl Pts',(-158.153172272815,-222.393239282414,
14.6574792166669));
#86332=CARTESIAN_POINT('Ctrl Pts',(-156.808287852926,-225.13765050987,14.4987213514351));
#86333=CARTESIAN_POINT('Ctrl Pts',(-158.384458264527,-227.756083996107,
14.3399634862033));
#86334=CARTESIAN_POINT('Ctrl Pts',(-161.439172408904,-227.852149517486,
14.1812056209715));
#86335=CARTESIAN_POINT('Ctrl Pts',(-163.176756021246,-225.337927912621,
14.0224477557397));
#86336=CARTESIAN_POINT('Ctrl Pts',(-162.006972647866,-222.514434695413,
13.8636898905079));
#86337=CARTESIAN_POINT('Ctrl Pts',(-159.000407986082,-221.965730747221,
13.7049320252761));
#86338=CARTESIAN_POINT('Ctrl Pts',(-156.908669896127,-224.193989899852,
13.5461741600443));
#86339=CARTESIAN_POINT('Ctrl Pts',(-157.646116995673,-227.159909464444,
13.3874162948125));
#86340=CARTESIAN_POINT('Ctrl Pts',(-160.537837728215,-228.149079972112,
13.2286584295808));
#86341=CARTESIAN_POINT('Ctrl Pts',(-162.937329393044,-226.256212613139,
13.069900564349));
#86342=CARTESIAN_POINT('Ctrl Pts',(-162.648577312867,-223.21365952002,12.9111426991172));
#86343=CARTESIAN_POINT('Ctrl Pts',(-159.935847380107,-221.805965163933,
12.7523848338854));
#86344=CARTESIAN_POINT('Ctrl Pts',(-157.28182992255,-223.321451364212,12.5936269686536));
#86345=CARTESIAN_POINT('Ctrl Pts',(-157.115481612986,-226.373145209957,
12.4348691034218));
#86346=CARTESIAN_POINT('Ctrl Pts',(-159.589044417786,-228.168136613547,
12.27611123819));
#86347=CARTESIAN_POINT('Ctrl Pts',(-162.438713755268,-227.063649513002,
12.1173533729582));
#86348=CARTESIAN_POINT('Ctrl Pts',(-163.056472359829,-224.070510459309,
11.9585955077264));
#86349=CARTESIAN_POINT('Ctrl Pts',(-160.876947580867,-221.928040196705,
11.7998376424946));
#86350=CARTESIAN_POINT('Ctrl Pts',(-157.894840410381,-222.597027425275,
11.6410797772628));
#86351=CARTESIAN_POINT('Ctrl Pts',(-156.839375213531,-225.465215059738,
11.482321912031));
#86352=CARTESIAN_POINT('Ctrl Pts',(-158.676513696969,-227.907637889824,
11.3235640467992));
#86353=CARTESIAN_POINT('Ctrl Pts',(-161.724906792896,-227.688990637483,
11.1648061815674));
#86354=CARTESIAN_POINT('Ctrl Pts',(-163.194665259795,-225.00937925946,11.0060483163357));
#86355=CARTESIAN_POINT('Ctrl Pts',(-161.740666206557,-222.321183983548,
10.8472904511039));
#86356=CARTESIAN_POINT('Ctrl Pts',(-158.693609509527,-222.084641020551,
10.6885325858721));
#86357=CARTESIAN_POINT('Ctrl Pts',(-156.842161338006,-224.516234480902,
10.5297747206403));
#86358=CARTESIAN_POINT('Ctrl Pts',(-157.880766985763,-227.390570125308,
10.3710168554085));
#86359=CARTESIAN_POINT('Ctrl Pts',(-160.858894604812,-228.077056085039,
10.2122589901767));
#86360=CARTESIAN_POINT('Ctrl Pts',(-163.050961915313,-225.947420436744,
10.0535011249449));
#86361=CARTESIAN_POINT('Ctrl Pts',(-162.450789000895,-222.950705641998,
9.89474325971312));
#86362=CARTESIAN_POINT('Ctrl Pts',(-159.607654089233,-221.829504963108,
9.73598539448133));
#86363=CARTESIAN_POINT('Ctrl Pts',(-157.123594139676,-223.609941217306,
9.57722752924952));
#86364=CARTESIAN_POINT('Ctrl Pts',(-157.272020720376,-226.662559214762,
9.41846966401774));
#86365=CARTESIAN_POINT('Ctrl Pts',(-159.917093830512,-228.193603084247,
9.25971179878594));
#86366=CARTESIAN_POINT('Ctrl Pts',(-162.638042663704,-226.801861536614,
9.10095393355416));
#86367=CARTESIAN_POINT('Ctrl Pts',(-162.944654954812,-223.761056381529,
8.94219606832235));
#86368=CARTESIAN_POINT('Ctrl Pts',(-160.556319147072,-221.854132377348,
8.78343820309057));
#86369=CARTESIAN_POINT('Ctrl Pts',(-157.658840077809,-222.82630629771,8.62468033785877));
#86370=CARTESIAN_POINT('Ctrl Pts',(-156.903990477271,-225.787844608929,
8.46592247262698));
#86371=CARTESIAN_POINT('Ctrl Pts',(-158.982608670187,-228.028347565038,
8.30716460739519));
#86372=CARTESIAN_POINT('Ctrl Pts',(-161.99234336814,-227.49730694871,8.1484067421634));
#86373=CARTESIAN_POINT('Ctrl Pts',(-163.178685493918,-224.680731111127,
7.9896488769316));
#86374=CARTESIAN_POINT('Ctrl Pts',(-161.455894780662,-222.156350148086,
7.83089101169981));
#86375=CARTESIAN_POINT('Ctrl Pts',(-158.400669221395,-222.234477417692,
7.67213314646802));
#86376=CARTESIAN_POINT('Ctrl Pts',(-156.809151127816,-224.843610845875,
7.51337528123623));
#86377=CARTESIAN_POINT('Ctrl Pts',(-158.137897796582,-227.595871621763,
7.35461741600443));
#86378=CARTESIAN_POINT('Ctrl Pts',(-161.170840328692,-227.972390791494,
7.19585955077265));
#86379=CARTESIAN_POINT('Ctrl Pts',(-163.132229838025,-225.628578025736,
7.03710168554084));
#86380=CARTESIAN_POINT('Ctrl Pts',(-162.227002722769,-222.709490675542,
6.87834382030906));
#86381=CARTESIAN_POINT('Ctrl Pts',(-159.283622803211,-221.886677369021,
6.71958595507727));
#86382=CARTESIAN_POINT('Ctrl Pts',(-156.995871265982,-223.913176811942,
6.56082808984547));
#86383=CARTESIAN_POINT('Ctrl Pts',(-157.457498227993,-226.934336793837,
6.40207022461368));
#86384=CARTESIAN_POINT('Ctrl Pts',(-160.246022711763,-228.185191818077,
6.24331235938188));
#86385=CARTESIAN_POINT('Ctrl Pts',(-162.809387219402,-226.520959415668,
6.0845544941501));
#86386=CARTESIAN_POINT('Ctrl Pts',(-162.801600654321,-223.46474501585,5.9257966289183));
#86387=CARTESIAN_POINT('Ctrl Pts',(-160.229789280576,-221.813595917153,
5.76703876368651));
#86388=CARTESIAN_POINT('Ctrl Pts',(-157.447674766284,-223.078643709776,
5.60828089845472));
#86389=CARTESIAN_POINT('Ctrl Pts',(-157.001448205521,-226.102116703656,
5.44952303322292));
#86390=CARTESIAN_POINT('Ctrl Pts',(-159.299496129151,-228.11693253369,5.29076516799113));
#86391=CARTESIAN_POINT('Ctrl Pts',(-162.238645167834,-227.279131831461,
5.13200730275934));
#86392=CARTESIAN_POINT('Ctrl Pts',(-163.128986236949,-224.355469766705,
4.97324943752754));
#86393=CARTESIAN_POINT('Ctrl Pts',(-161.155679225052,-222.021681746113,
4.81449157229576));
#86394=CARTESIAN_POINT('Ctrl Pts',(-158.124694631834,-222.413650474363,
4.65573370706396));
#86395=CARTESIAN_POINT('Ctrl Pts',(-156.809989437815,-225.172646186762,
4.49697584183217));
#86396=CARTESIAN_POINT('Ctrl Pts',(-158.414781784868,-227.773636115843,
4.33821797660038));
#86397=CARTESIAN_POINT('Ctrl Pts',(-161.470365780064,-227.83619438074,4.17946011136858));
#86398=CARTESIAN_POINT('Ctrl Pts',(-163.180271071183,-225.303067659987,
4.0207022461368));
#86399=CARTESIAN_POINT('Ctrl Pts',(-161.979592402983,-222.492573428581,
3.861944380905));
#86400=CARTESIAN_POINT('Ctrl Pts',(-158.967190845488,-221.976875897049,
3.70318651567321));
#86401=CARTESIAN_POINT('Ctrl Pts',(-156.900016185444,-224.227941425007,
3.54442865044141));
#86402=CARTESIAN_POINT('Ctrl Pts',(-157.669946590876,-227.185594931785,
3.38567078520963));
#86403=CARTESIAN_POINT('Ctrl Pts',(-160.572341784094,-228.142992040145,
3.22691291997783));
#86404=CARTESIAN_POINT('Ctrl Pts',(-162.950929800296,-226.223922962759,
3.06815505474604));
#86405=CARTESIAN_POINT('Ctrl Pts',(-162.628826976652,-223.184719625952,
2.90939718951425));
#86406=CARTESIAN_POINT('Ctrl Pts',(-159.900821812869,-221.806860841059,
2.75063932428245));
#86407=CARTESIAN_POINT('Ctrl Pts',(-157.2635845106,-223.351362837049,2.59188145905066));
#86408=CARTESIAN_POINT('Ctrl Pts',(-157.130714580378,-226.404697607255,
2.43312359381887));
#86409=CARTESIAN_POINT('Ctrl Pts',(-159.62381450407,-228.172452959444,2.27436572858708));
#86410=CARTESIAN_POINT('Ctrl Pts',(-162.461199481127,-227.036779950835,
2.11560786335528));
#86411=CARTESIAN_POINT('Ctrl Pts',(-163.046094577601,-224.037045050717,
1.95684999812349));
#86412=CARTESIAN_POINT('Ctrl Pts',(-160.843204476844,-221.918608475596,
1.7980921328917));
#86413=CARTESIAN_POINT('Ctrl Pts',(-157.868612758181,-222.620257166302,
1.6393342676599));
#86414=CARTESIAN_POINT('Ctrl Pts',(-156.844668455705,-225.499854987468,
1.48057640242812));
#86415=CARTESIAN_POINT('Ctrl Pts',(-158.708479523612,-227.921967734449,
1.32181853719632));
#86416=CARTESIAN_POINT('Ctrl Pts',(-161.754298245737,-227.669932680775,
1.16306067196453));
#86417=CARTESIAN_POINT('Ctrl Pts',(-163.194566339583,-224.974298659625,
1.00430280673274));
#86418=CARTESIAN_POINT('Ctrl Pts',(-161.711202601395,-222.302345624998,
0.845544941500946));
#86419=CARTESIAN_POINT('Ctrl Pts',(-158.661673352397,-222.098955592586,
0.686787076269153));
#86420=CARTESIAN_POINT('Ctrl Pts',(-156.837131898881,-224.551286514725,
0.528029211037362));
#86421=CARTESIAN_POINT('Ctrl Pts',(-157.90693228861,-227.412858930286,0.369271345805565));
#86422=CARTESIAN_POINT('Ctrl Pts',(-160.89294716102,-228.069149561511,0.210513480573778));
#86423=CARTESIAN_POINT('Ctrl Pts',(-163.060277378019,-225.910475869087,
0.0517556153419819));
#86424=CARTESIAN_POINT('Ctrl Pts',(-162.638345947507,-223.926643402192,
-0.0540829614792118));
#86425=CARTESIAN_POINT('Ctrl Pts',(-162.054331550342,-223.243574678773,
-0.10700224988981));
#86426=CARTESIAN_POINT('Ctrl Pts',(-160.650199997975,-227.432086802035,
20.3210067496694));
#86427=CARTESIAN_POINT('Ctrl Pts',(-161.458872983031,-227.215894200354,
20.2680874612588));
#86428=CARTESIAN_POINT('Ctrl Pts',(-162.829415908735,-225.915729044181,
20.1622488844376));
#86429=CARTESIAN_POINT('Ctrl Pts',(-162.304705378354,-223.11526093862,20.0034910192058));
#86430=CARTESIAN_POINT('Ctrl Pts',(-159.666401152891,-222.043601961419,
19.8447331539741));
#86431=CARTESIAN_POINT('Ctrl Pts',(-157.335462255055,-223.675698334549,
19.6859752887423));
#86432=CARTESIAN_POINT('Ctrl Pts',(-157.442116709546,-226.52072019288,19.5272174235105));
#86433=CARTESIAN_POINT('Ctrl Pts',(-159.890223514064,-227.973532840977,
19.3684595582787));
#86434=CARTESIAN_POINT('Ctrl Pts',(-162.438567551761,-226.705183298269,
19.2097016930469));
#86435=CARTESIAN_POINT('Ctrl Pts',(-162.755245599982,-223.876146476471,
19.0509438278151));
#86436=CARTESIAN_POINT('Ctrl Pts',(-160.550269520285,-222.075710277569,
18.8921859625833));
#86437=CARTESIAN_POINT('Ctrl Pts',(-157.841712562158,-222.951559859093,
18.7334280973515));
#86438=CARTESIAN_POINT('Ctrl Pts',(-157.108407765684,-225.702153371286,
18.5746702321197));
#86439=CARTESIAN_POINT('Ctrl Pts',(-159.021494052134,-227.810130558195,
18.4159123668879));
#86440=CARTESIAN_POINT('Ctrl Pts',(-161.830106059892,-227.346279061469,
18.2571545016561));
#86441=CARTESIAN_POINT('Ctrl Pts',(-162.963806463313,-224.735111762279,
18.0983966364243));
#86442=CARTESIAN_POINT('Ctrl Pts',(-161.385030638332,-222.366370793208,
17.9396387711925));
#86443=CARTESIAN_POINT('Ctrl Pts',(-158.538675150368,-222.407926869249,
17.7808809059607));
#86444=CARTESIAN_POINT('Ctrl Pts',(-157.029723951781,-224.821748317863,
17.622123040729));
#86445=CARTESIAN_POINT('Ctrl Pts',(-158.239169350678,-227.398705628965,
17.4633651754972));
#86446=CARTESIAN_POINT('Ctrl Pts',(-161.060126854468,-227.780367676496,
17.3046073102654));
#86447=CARTESIAN_POINT('Ctrl Pts',(-162.910856320146,-225.617437319578,
17.1458494450336));
#86448=CARTESIAN_POINT('Ctrl Pts',(-162.097570187703,-222.889428359895,
16.9870915798018));
#86449=CARTESIAN_POINT('Ctrl Pts',(-159.364587906002,-222.093014478465,
16.82833371457));
#86450=CARTESIAN_POINT('Ctrl Pts',(-157.213134745793,-223.957073633848,
16.6695758493382));
#86451=CARTESIAN_POINT('Ctrl Pts',(-157.612220557582,-226.775618957645,
16.5108179841064));
#86452=CARTESIAN_POINT('Ctrl Pts',(-160.196602020722,-227.969117881651,
16.3520601188746));
#86453=CARTESIAN_POINT('Ctrl Pts',(-162.601053322447,-226.445280236925,
16.1933022536428));
#86454=CARTESIAN_POINT('Ctrl Pts',(-162.625020725647,-223.598722176297,
16.0345443884111));
#86455=CARTESIAN_POINT('Ctrl Pts',(-160.246569264012,-222.034613524771,
15.8757865231792));
#86456=CARTESIAN_POINT('Ctrl Pts',(-157.642457621625,-223.184426458786,
15.7170286579475));
#86457=CARTESIAN_POINT('Ctrl Pts',(-157.19596867123,-225.995852226314,15.5582707927157));
#86458=CARTESIAN_POINT('Ctrl Pts',(-159.315729082654,-227.895874075485,
15.3995129274839));
#86459=CARTESIAN_POINT('Ctrl Pts',(-162.061734210728,-227.145592084648,
15.2407550622521));
#86460=CARTESIAN_POINT('Ctrl Pts',(-162.920840270217,-224.431664302315,
15.0819971970203));
#86461=CARTESIAN_POINT('Ctrl Pts',(-161.106793429264,-222.237877328154,
14.9232393317885));
#86462=CARTESIAN_POINT('Ctrl Pts',(-158.279809285372,-222.571984914649,
14.7644814665567));
#86463=CARTESIAN_POINT('Ctrl Pts',(-157.027143615862,-225.128211811777,
14.6057236013249));
#86464=CARTESIAN_POINT('Ctrl Pts',(-158.495235992211,-227.567099263809,
14.4469657360931));
#86465=CARTESIAN_POINT('Ctrl Pts',(-161.340488329315,-227.656577570551,
14.2882078708613));
#86466=CARTESIAN_POINT('Ctrl Pts',(-162.958925800143,-225.314756189193,
14.1294500056295));
#86467=CARTESIAN_POINT('Ctrl Pts',(-161.869354495037,-222.684869955862,
13.9706921403977));
#86468=CARTESIAN_POINT('Ctrl Pts',(-159.068950029584,-222.173790647886,
13.811934275166));
#86469=CARTESIAN_POINT('Ctrl Pts',(-157.120642460443,-224.249258027827,
13.6531764099341));
#86470=CARTESIAN_POINT('Ctrl Pts',(-157.807522798276,-227.011804431178,
13.4944185447024));
#86471=CARTESIAN_POINT('Ctrl Pts',(-160.50095818491,-227.933147498227,13.3356606794706));
#86472=CARTESIAN_POINT('Ctrl Pts',(-162.735916660414,-226.170074090242,
13.1769028142388));
#86473=CARTESIAN_POINT('Ctrl Pts',(-162.466964315894,-223.336148920879,
13.018144949007));
#86474=CARTESIAN_POINT('Ctrl Pts',(-159.940246326479,-222.024980193698,
12.8593870837752));
#86475=CARTESIAN_POINT('Ctrl Pts',(-157.468214896721,-223.436549476255,
12.7006292185434));
#86476=CARTESIAN_POINT('Ctrl Pts',(-157.313273093923,-226.278988616662,
12.5418713533116));
#86477=CARTESIAN_POINT('Ctrl Pts',(-159.617223649915,-227.950897425395,
12.3831134880798));
#86478=CARTESIAN_POINT('Ctrl Pts',(-162.271491106452,-226.922145026448,
12.224355622848));
#86479=CARTESIAN_POINT('Ctrl Pts',(-162.846889991688,-224.134245574882,
12.0655977576162));
#86480=CARTESIAN_POINT('Ctrl Pts',(-160.816815268483,-222.13868453914,11.9068398923844));
#86481=CARTESIAN_POINT('Ctrl Pts',(-158.039191243683,-222.761799300658,
11.7480820271526));
#86482=CARTESIAN_POINT('Ctrl Pts',(-157.056099315557,-225.433315254199,
11.5893241619208));
#86483=CARTESIAN_POINT('Ctrl Pts',(-158.767265178067,-227.708261104137,
11.4305662966891));
#86484=CARTESIAN_POINT('Ctrl Pts',(-161.606629901135,-227.504606498068,
11.2718084314573));
#86485=CARTESIAN_POINT('Ctrl Pts',(-162.975607001862,-225.008736123459,
11.1130505662255));
#86486=CARTESIAN_POINT('Ctrl Pts',(-161.621308691499,-222.504870449003,
10.9542927009937));
#86487=CARTESIAN_POINT('Ctrl Pts',(-158.783188730432,-222.284547241501,
10.7955348357619));
#86488=CARTESIAN_POINT('Ctrl Pts',(-157.058694395424,-224.549406291795,
10.6367769705301));
#86489=CARTESIAN_POINT('Ctrl Pts',(-158.026082834059,-227.226648686118,
10.4780191052983));
#86490=CARTESIAN_POINT('Ctrl Pts',(-160.800000185342,-227.866062290468,
10.3192612400665));
#86491=CARTESIAN_POINT('Ctrl Pts',(-162.841757398458,-225.882455799286,
10.1605033748347));
#86492=CARTESIAN_POINT('Ctrl Pts',(-162.282738352255,-223.0912257953,10.0017455096029));
#86493=CARTESIAN_POINT('Ctrl Pts',(-159.634557255835,-222.046905868394,
9.84298764437113));
#86494=CARTESIAN_POINT('Ctrl Pts',(-157.320829344503,-223.705257574607,
9.68422977913933));
#86495=CARTESIAN_POINT('Ctrl Pts',(-157.459078311727,-226.548557497625,
9.52547191390755));
#86496=CARTESIAN_POINT('Ctrl Pts',(-159.922778708139,-227.974617659712,
9.36671404867574));
#86497=CARTESIAN_POINT('Ctrl Pts',(-162.457152027825,-226.678307856605,
9.20795618344397));
#86498=CARTESIAN_POINT('Ctrl Pts',(-162.742739908271,-223.846010769131,
9.04919831821216));
#86499=CARTESIAN_POINT('Ctrl Pts',(-160.518172332523,-222.069844580369,
8.89044045298038));
#86500=CARTESIAN_POINT('Ctrl Pts',(-157.819373458426,-222.975356516428,
8.73168258774858));
#86501=CARTESIAN_POINT('Ctrl Pts',(-157.116283909427,-225.733822089035,
8.57292472251679));
#86502=CARTESIAN_POINT('Ctrl Pts',(-159.05237121312,-227.820693714614,8.414166857285));
#86503=CARTESIAN_POINT('Ctrl Pts',(-161.855728345302,-227.3260665635,8.2554089920532));
#86504=CARTESIAN_POINT('Ctrl Pts',(-162.960722968838,-224.70262338494,8.09665112682141));
#86505=CARTESIAN_POINT('Ctrl Pts',(-161.356064047721,-222.35133927279,7.93789326158962));
#86506=CARTESIAN_POINT('Ctrl Pts',(-158.510335363456,-222.424109354026,
7.77913539635782));
#86507=CARTESIAN_POINT('Ctrl Pts',(-157.027947695977,-224.854334453163,
7.62037753112604));
#86508=CARTESIAN_POINT('Ctrl Pts',(-158.265582180266,-227.417872655037,
7.46161966589424));
#86509=CARTESIAN_POINT('Ctrl Pts',(-161.090555784972,-227.768573898102,
7.30286180066245));
#86510=CARTESIAN_POINT('Ctrl Pts',(-162.917452778156,-225.585476418495,
7.14410393543066));
#86511=CARTESIAN_POINT('Ctrl Pts',(-162.074297103498,-222.866550943705,
6.98534607019887));
#86512=CARTESIAN_POINT('Ctrl Pts',(-159.332744801288,-222.10015796134,6.82658820496707));
#86513=CARTESIAN_POINT('Ctrl Pts',(-157.2018644307,-223.987700298723,6.66783033973528));
#86514=CARTESIAN_POINT('Ctrl Pts',(-157.631837623101,-226.801699282907,
6.50907247450349));
#86515=CARTESIAN_POINT('Ctrl Pts',(-160.229152929714,-227.966783154224,
6.3503146092717));
#86516=CARTESIAN_POINT('Ctrl Pts',(-162.616747484064,-226.416667199462,
6.1915567440399));
#86517=CARTESIAN_POINT('Ctrl Pts',(-162.6094948439,-223.570017479461,6.03279887880812));
#86518=CARTESIAN_POINT('Ctrl Pts',(-160.214032625214,-222.032087706024,
5.87404101357632));
#86519=CARTESIAN_POINT('Ctrl Pts',(-157.622687756349,-223.210391147325,
5.71528314834453));
#86520=CARTESIAN_POINT('Ctrl Pts',(-157.207058959388,-226.026544540218,
5.55652528311273));
#86521=CARTESIAN_POINT('Ctrl Pts',(-159.347529692965,-227.903204410272,
5.39776741788094));
#86522=CARTESIAN_POINT('Ctrl Pts',(-162.085141225883,-227.122851718211,
5.23900955264915));
#86523=CARTESIAN_POINT('Ctrl Pts',(-162.914431590869,-224.399665217122,
5.08025168741736));
#86524=CARTESIAN_POINT('Ctrl Pts',(-161.076434278499,-222.225905085714,
4.92149382218557));
#86525=CARTESIAN_POINT('Ctrl Pts',(-158.253284356777,-222.590996510776,
4.76273595695377));
#86526=CARTESIAN_POINT('Ctrl Pts',(-157.028728523044,-225.160807834436,
4.60397809172198));
#86527=CARTESIAN_POINT('Ctrl Pts',(-158.523480228182,-227.583447834359,
4.44522022649019));
#86528=CARTESIAN_POINT('Ctrl Pts',(-161.369542770418,-227.641716477836,
4.2864623612584));
#86529=CARTESIAN_POINT('Ctrl Pts',(-162.962199823039,-225.282286304748,
4.1277044960266));
#86530=CARTESIAN_POINT('Ctrl Pts',(-161.843851714069,-222.664507716515,
3.96894663079481));
#86531=CARTESIAN_POINT('Ctrl Pts',(-159.038010588956,-222.184171574577,
3.81018876556302));
#86532=CARTESIAN_POINT('Ctrl Pts',(-157.112582134867,-224.280881496252,
3.65143090033122));
#86533=CARTESIAN_POINT('Ctrl Pts',(-157.829718397681,-227.035728645533,
3.49267303509944));
#86534=CARTESIAN_POINT('Ctrl Pts',(-160.533096297017,-227.927477015872,
3.33391516986764));
#86535=CARTESIAN_POINT('Ctrl Pts',(-162.748584487481,-226.139998541806,
3.17515730463585));
#86536=CARTESIAN_POINT('Ctrl Pts',(-162.448568260611,-223.309193435901,
3.01639943940406));
#86537=CARTESIAN_POINT('Ctrl Pts',(-159.907622463056,-222.025814454227,
2.85764157417227));
#86538=CARTESIAN_POINT('Ctrl Pts',(-157.451220573017,-223.464409918827,
2.69888370894047));
#86539=CARTESIAN_POINT('Ctrl Pts',(-157.32746153645,-226.308377465473,2.54012584370868));
#86540=CARTESIAN_POINT('Ctrl Pts',(-159.649609550717,-227.954917799371,
2.38136797847689));
#86541=CARTESIAN_POINT('Ctrl Pts',(-162.292434985658,-226.897117910672,
2.22261011324509));
#86542=CARTESIAN_POINT('Ctrl Pts',(-162.837223814186,-224.103074889997,
2.06385224801331));
#86543=CARTESIAN_POINT('Ctrl Pts',(-160.785385929749,-222.129899551328,
1.90509438278151));
#86544=CARTESIAN_POINT('Ctrl Pts',(-158.014762022095,-222.783436177899,
1.74633651754972));
#86545=CARTESIAN_POINT('Ctrl Pts',(-157.061029600014,-225.465579921422,
1.58757865231793));
#86546=CARTESIAN_POINT('Ctrl Pts',(-158.797039107366,-227.721608351042,
1.42882078708613));
#86547=CARTESIAN_POINT('Ctrl Pts',(-161.634005981492,-227.486855345816,
1.27006292185434));
#86548=CARTESIAN_POINT('Ctrl Pts',(-162.975514864611,-224.976061001026,
1.11130505662255));
#86549=CARTESIAN_POINT('Ctrl Pts',(-161.593865406306,-222.487323837059,
0.952547191390755));
#86550=CARTESIAN_POINT('Ctrl Pts',(-158.753442436207,-222.297880263058,
0.793789326158963));
#86551=CARTESIAN_POINT('Ctrl Pts',(-157.054009825035,-224.582054806988,
0.635031460927172));
#86552=CARTESIAN_POINT('Ctrl Pts',(-158.050453981591,-227.247409147313,
0.476273595695376));
#86553=CARTESIAN_POINT('Ctrl Pts',(-160.83171775712,-227.858697917409,0.317515730463588));
#86554=CARTESIAN_POINT('Ctrl Pts',(-162.850434099709,-225.84804452134,0.158757865231792));
#86555=CARTESIAN_POINT('Ctrl Pts',(-162.457434515453,-224.000243484622,
0.0529192884105984));
#86556=CARTESIAN_POINT('Ctrl Pts',(-161.913465996665,-223.364012796625,
0.));
#86557=CARTESIAN_POINT('Ctrl Pts',(-161.913465996665,-223.364012796625,
0.));
#86558=CARTESIAN_POINT('Ctrl Pts',(-161.975061821414,-223.421897746888,
-3.51911852623003E-16));
#86559=CARTESIAN_POINT('Ctrl Pts',(-162.033285691278,-223.482934384445,
4.3246434463342E-16));
#86560=CARTESIAN_POINT('Ctrl Pts',(-162.08814123845,-223.546737650339,6.66133814775094E-16));
#86561=CARTESIAN_POINT('Ctrl Pts',(-162.144450808367,-223.612232110736,
9.059970199533E-16));
#86562=CARTESIAN_POINT('Ctrl Pts',(-162.197211559747,-223.680642241593,
-9.91859996330672E-16));
#86563=CARTESIAN_POINT('Ctrl Pts',(-162.246401858891,-223.751600097819,
-1.38777878078145E-15));
#86564=CARTESIAN_POINT('Ctrl Pts',(-162.297290107341,-223.82500727525,-1.79736387824417E-15));
#86565=CARTESIAN_POINT('Ctrl Pts',(-162.344357741728,-223.901141619796,
4.27848227219236E-15));
#86566=CARTESIAN_POINT('Ctrl Pts',(-162.387545875999,-223.979639757331,
4.9960036108132E-15));
#86567=CARTESIAN_POINT('Ctrl Pts',(-162.406440684742,-224.013982692503,
5.30991919645982E-15));
#86568=CARTESIAN_POINT('Ctrl Pts',(-162.424592438936,-224.048778578827,
5.06079435892012E-15));
#86569=CARTESIAN_POINT('Ctrl Pts',(-162.441993762856,-224.083999076523,
5.27355936696949E-15));
#86570=CARTESIAN_POINT('Ctrl Pts',(-162.451521735226,-224.103283812009,
5.39005734880947E-15));
#86571=CARTESIAN_POINT('Ctrl Pts',(-162.460824698828,-224.122695867125,
-1.80422085998584E-15));
#86572=CARTESIAN_POINT('Ctrl Pts',(-162.469901237658,-224.142230719459,
-2.16493489801906E-15));
#86573=CARTESIAN_POINT('Ctrl Pts',(-162.478557397273,-224.160860816575,
-2.50894249247741E-15));
#86574=CARTESIAN_POINT('Ctrl Pts',(-162.487010116501,-224.17960861694,1.52748735518423E-15));
#86575=CARTESIAN_POINT('Ctrl Pts',(-162.495244043881,-224.198437344968,
1.49880108324396E-15));
#86576=CARTESIAN_POINT('Ctrl Pts',(-162.531783468902,-224.281992963608,
1.37150097062534E-15));
#86577=CARTESIAN_POINT('Ctrl Pts',(-162.564063480614,-224.367232235573,
-3.46659333174283E-15));
#86578=CARTESIAN_POINT('Ctrl Pts',(-162.592060384007,-224.45375591163,-1.30451205393456E-15));
#86579=CARTESIAN_POINT('Ctrl Pts',(-162.620521837946,-224.541715268642,
8.93444478518701E-16));
#86580=CARTESIAN_POINT('Ctrl Pts',(-162.644557356984,-224.631002763181,
4.3432970000933E-16));
#86581=CARTESIAN_POINT('Ctrl Pts',(-162.664102933426,-224.721236079534,
1.02695629777827E-15));
#86582=CARTESIAN_POINT('Ctrl Pts',(-162.683304934146,-224.809883258132,
1.60916559670726E-15));
#86583=CARTESIAN_POINT('Ctrl Pts',(-162.698173710175,-224.899444209412,
4.52079509896306E-15));
#86584=CARTESIAN_POINT('Ctrl Pts',(-162.708605924403,-224.989579250553,
5.16253706450698E-15));
#86585=CARTESIAN_POINT('Ctrl Pts',(-162.712739843743,-225.025296595084,
5.41683681955754E-15));
#86586=CARTESIAN_POINT('Ctrl Pts',(-162.716176611214,-225.061104267913,
1.34242000952038E-14));
#86587=CARTESIAN_POINT('Ctrl Pts',(-162.718907757196,-225.096981670027,
1.38500322321988E-14));
#86588=CARTESIAN_POINT('Ctrl Pts',(-162.720525958649,-225.118238997391,
1.41023373770799E-14));
#86589=CARTESIAN_POINT('Ctrl Pts',(-162.721896425303,-225.139520807707,
3.52876023556576E-15));
#86590=CARTESIAN_POINT('Ctrl Pts',(-162.723017191021,-225.160822839396,
3.3584246494911E-15));
#86591=CARTESIAN_POINT('Ctrl Pts',(-162.723759187735,-225.174925731069,
3.24565492153553E-15));
#86592=CARTESIAN_POINT('Ctrl Pts',(-162.72439165709,-225.189037398679,3.64992830526776E-15));
#86593=CARTESIAN_POINT('Ctrl Pts',(-162.724913686862,-225.203142207687,
3.69149155687865E-15));
#86594=CARTESIAN_POINT('Ctrl Pts',(-162.728436673681,-225.298330372776,
3.97198664573279E-15));
#86595=CARTESIAN_POINT('Ctrl Pts',(-162.726942917764,-225.39336773222,1.17756522009375E-14));
#86596=CARTESIAN_POINT('Ctrl Pts',(-162.720374349249,-225.487854987023,
1.06303854607859E-14));
#86597=CARTESIAN_POINT('Ctrl Pts',(-162.71382751348,-225.58202962157,9.48890794684939E-15));
#86598=CARTESIAN_POINT('Ctrl Pts',(-162.702239749738,-225.675658740134,
2.24970435481665E-15));
#86599=CARTESIAN_POINT('Ctrl Pts',(-162.685505553451,-225.768364895442,
2.91433543964104E-15));
#86600=CARTESIAN_POINT('Ctrl Pts',(-162.683601264249,-225.778914510579,
2.9899679812951E-15));
#86601=CARTESIAN_POINT('Ctrl Pts',(-162.681630276117,-225.789452183786,
5.32923785720578E-15));
#86602=CARTESIAN_POINT('Ctrl Pts',(-162.679592390737,-225.799977364968,
5.38458166943201E-15));
#86603=CARTESIAN_POINT('Ctrl Pts',(-162.662059174472,-225.890532152657,
5.863838114987E-15));
#86604=CARTESIAN_POINT('Ctrl Pts',(-162.63957844198,-225.980162557517,1.21988532545923E-14));
#86605=CARTESIAN_POINT('Ctrl Pts',(-162.612425094939,-226.068630980284,
1.37667655053519E-14));
#86606=CARTESIAN_POINT('Ctrl Pts',(-162.60172483783,-226.10349352847,1.43846290851872E-14));
#86607=CARTESIAN_POINT('Ctrl Pts',(-162.590298397256,-226.138175582511,
9.10155007490613E-15));
#86608=CARTESIAN_POINT('Ctrl Pts',(-162.578160429641,-226.172662264402,
9.74220704108575E-15));
#86609=CARTESIAN_POINT('Ctrl Pts',(-162.572850001538,-226.187750378864,
1.00224980144874E-14));
#86610=CARTESIAN_POINT('Ctrl Pts',(-162.567403364151,-226.202801093293,
1.26710079476777E-14));
#86611=CARTESIAN_POINT('Ctrl Pts',(-162.561821675617,-226.217813142587,
1.301736496373E-14));
#86612=CARTESIAN_POINT('Ctrl Pts',(-162.557400927301,-226.229702822785,
1.32916828849232E-14));
#86613=CARTESIAN_POINT('Ctrl Pts',(-162.552895865822,-226.241567036791,
-2.18922818415383E-15));
#86614=CARTESIAN_POINT('Ctrl Pts',(-162.548310798671,-226.253395997137,
-1.85962356624714E-15));
#86615=CARTESIAN_POINT('Ctrl Pts',(-162.514552420086,-226.340488837539,
5.67149501155898E-16));
#86616=CARTESIAN_POINT('Ctrl Pts',(-162.476411071193,-226.425806841494,
7.30675670375641E-15));
#86617=CARTESIAN_POINT('Ctrl Pts',(-162.434220018652,-226.509119275137,
8.24340595784179E-15));
#86618=CARTESIAN_POINT('Ctrl Pts',(-162.390446644469,-226.595556235402,
9.21518304820882E-15));
#86619=CARTESIAN_POINT('Ctrl Pts',(-162.342313990897,-226.679835090795,
1.02191638285051E-14));
#86620=CARTESIAN_POINT('Ctrl Pts',(-162.290138160741,-226.761695129367,
1.04777297948999E-14));
#86621=CARTESIAN_POINT('Ctrl Pts',(-162.237360636907,-226.844499181049,
1.07392775539542E-14));
#86622=CARTESIAN_POINT('Ctrl Pts',(-162.18044573594,-226.924829121338,9.48127483138641E-15));
#86623=CARTESIAN_POINT('Ctrl Pts',(-162.119668717606,-227.002400317474,
1.01307850997046E-14));
#86624=CARTESIAN_POINT('Ctrl Pts',(-162.076869286147,-227.057026279444,
1.05881729573591E-14));
#86625=CARTESIAN_POINT('Ctrl Pts',(-162.032153516023,-227.110283883549,
1.04004194029648E-14));
#86626=CARTESIAN_POINT('Ctrl Pts',(-161.985604112955,-227.162066010945,
1.1518563880486E-14));
#86627=CARTESIAN_POINT('Ctrl Pts',(-161.974398233174,-227.174531569172,
1.17877358089457E-14));
#86628=CARTESIAN_POINT('Ctrl Pts',(-161.963085448517,-227.186912117143,
1.11605785323705E-14));
#86629=CARTESIAN_POINT('Ctrl Pts',(-161.951678152587,-227.199194229367,
1.11993747609063E-14));
#86630=CARTESIAN_POINT('Ctrl Pts',(-161.883011874223,-227.273126469054,
1.14329088643908E-14));
#86631=CARTESIAN_POINT('Ctrl Pts',(-161.810832651604,-227.343597623949,
1.49981926778286E-14));
#86632=CARTESIAN_POINT('Ctrl Pts',(-161.735453614524,-227.410320720505,
1.35447209004269E-14));
#86633=CARTESIAN_POINT('Ctrl Pts',(-161.670633677549,-227.467697241631,
1.2294851538123E-14));
#86634=CARTESIAN_POINT('Ctrl Pts',(-161.603446552378,-227.522302286696,
8.96312012513312E-15));
#86635=CARTESIAN_POINT('Ctrl Pts',(-161.534065125301,-227.573938079886,
7.79931674799172E-15));
#86636=CARTESIAN_POINT('Ctrl Pts',(-161.508545380815,-227.592930659083,
7.37124880434049E-15));
#86637=CARTESIAN_POINT('Ctrl Pts',(-161.482728554244,-227.611521358039,
6.88696359544211E-15));
#86638=CARTESIAN_POINT('Ctrl Pts',(-161.456622539761,-227.629699683014,
6.67521593555875E-15));
#86639=CARTESIAN_POINT('Ctrl Pts',(-161.439930141174,-227.64132305227,6.53982275476302E-15));
#86640=CARTESIAN_POINT('Ctrl Pts',(-161.423118461496,-227.652778396977,
1.59935197070125E-14));
#86641=CARTESIAN_POINT('Ctrl Pts',(-161.406204349576,-227.664053326898,
1.52794443764037E-14));
#86642=CARTESIAN_POINT('Ctrl Pts',(-161.320010703824,-227.721509924092,
1.16405447178875E-14));
#86643=CARTESIAN_POINT('Ctrl Pts',(-161.23107539812,-227.774344401213,5.94975413786717E-15));
#86644=CARTESIAN_POINT('Ctrl Pts',(-161.139704794375,-227.822237400702,
6.55031584528842E-15));
#86645=CARTESIAN_POINT('Ctrl Pts',(-161.04833419063,-227.87013040019,7.15087755270967E-15));
#86646=CARTESIAN_POINT('Ctrl Pts',(-160.954527650215,-227.913082824186,
1.10522651367167E-15));
#86647=CARTESIAN_POINT('Ctrl Pts',(-160.858553721283,-227.95073486507,-2.17837900495788E-15));
#86648=CARTESIAN_POINT('Ctrl Pts',(-160.837669284134,-227.95892814933,-2.89637846893106E-15));
#86649=CARTESIAN_POINT('Ctrl Pts',(-160.816682095278,-227.966870267892,
8.4228218624679E-16));
#86650=CARTESIAN_POINT('Ctrl Pts',(-160.795596249024,-227.974562448592,
6.93889390390723E-16));
#86651=CARTESIAN_POINT('Ctrl Pts',(-162.514309543052,-224.998572563953,
19.1125833024919));
#86652=CARTESIAN_POINT('Ctrl Pts',(-162.515998915399,-224.67257072807,19.092036810933));
#86653=CARTESIAN_POINT('Ctrl Pts',(-162.457161966883,-224.347153821985,
19.071490319374));
#86654=CARTESIAN_POINT('Ctrl Pts',(-162.334969911996,-224.04757991362,19.0509438278151));
#86655=CARTESIAN_POINT('Ctrl Pts',(-162.020253573416,-223.276001076837,
18.9980245394045));
#86656=CARTESIAN_POINT('Ctrl Pts',(-161.28526154685,-222.675855677203,18.9451052509939));
#86657=CARTESIAN_POINT('Ctrl Pts',(-160.46633937388,-222.52175790764,18.8921859625832));
#86658=CARTESIAN_POINT('Ctrl Pts',(-159.647417200909,-222.367660138077,
18.8392666741726));
#86659=CARTESIAN_POINT('Ctrl Pts',(-158.744564881534,-222.659609998585,
18.7863473857621));
#86660=CARTESIAN_POINT('Ctrl Pts',(-158.170921255767,-223.264017180871,
18.7334280973515));
#86661=CARTESIAN_POINT('Ctrl Pts',(-157.59727763,-223.868424363157,18.6805088089409));
#86662=CARTESIAN_POINT('Ctrl Pts',(-157.352842697842,-224.785288867222,
18.6275895205303));
#86663=CARTESIAN_POINT('Ctrl Pts',(-157.549472946172,-225.595050650405,
18.5746702321197));
#86664=CARTESIAN_POINT('Ctrl Pts',(-157.746103194501,-226.404812433589,
18.5217509437091));
#86665=CARTESIAN_POINT('Ctrl Pts',(-158.383798623317,-227.107471495892,
18.4688316552985));
#86666=CARTESIAN_POINT('Ctrl Pts',(-159.170748339018,-227.381492444256,
18.4159123668879));
#86667=CARTESIAN_POINT('Ctrl Pts',(-159.95769805472,-227.65551339262,18.3629930784773));
#86668=CARTESIAN_POINT('Ctrl Pts',(-160.893902057306,-227.500896227044,
18.3100737900667));
#86669=CARTESIAN_POINT('Ctrl Pts',(-161.550954125836,-226.988393094392,
18.2571545016561));
#86670=CARTESIAN_POINT('Ctrl Pts',(-162.14929175983,-226.521687445794,18.2089641019347));
#86671=CARTESIAN_POINT('Ctrl Pts',(-162.51613860921,-225.7581996753,18.1607737022133));
#86672=CARTESIAN_POINT('Ctrl Pts',(-162.520906603697,-224.998703157721,
18.112583302492));
#86673=CARTESIAN_POINT('Origin',(-160.,225.,22.2084234471774));
#86674=CARTESIAN_POINT('Ctrl Pts',(-163.076377868511,225.002226294578,19.7084234471774));
#86675=CARTESIAN_POINT('Ctrl Pts',(-163.077562763763,225.146330752986,19.7009407276991));
#86676=CARTESIAN_POINT('Ctrl Pts',(-163.00282692276,226.308360985244,19.6405387198101));
#86677=CARTESIAN_POINT('Ctrl Pts',(-161.521864740257,228.298893686106,19.5272174235105));
#86678=CARTESIAN_POINT('Ctrl Pts',(-158.054123086354,228.067610661284,19.3684595582787));
#86679=CARTESIAN_POINT('Ctrl Pts',(-156.367330834239,225.02922603841,19.2097016930469));
#86680=CARTESIAN_POINT('Ctrl Pts',(-158.005117297794,221.963912747455,19.0509438278151));
#86681=CARTESIAN_POINT('Ctrl Pts',(-161.468639591425,221.677313620367,18.8921859625833));
#86682=CARTESIAN_POINT('Ctrl Pts',(-162.992852850625,223.658102562111,18.7780125023707));
#86683=CARTESIAN_POINT('Ctrl Pts',(-163.077320480262,224.836964798983,18.7167583305688));
#86684=CARTESIAN_POINT('Ctrl Pts',(-163.07593125098,224.997572466666,18.7084234471774));
#86685=CARTESIAN_POINT('Ctrl Pts',(-163.070362295124,224.996974657089,19.7915765528225));
#86686=CARTESIAN_POINT('Ctrl Pts',(-163.065080696031,225.700310975174,19.7552124583938));
#86687=CARTESIAN_POINT('Ctrl Pts',(-162.477826045596,227.437424363323,19.6659290755545));
#86688=CARTESIAN_POINT('Ctrl Pts',(-159.59272451442,228.609330199079,19.5237264043046));
#86689=CARTESIAN_POINT('Ctrl Pts',(-156.746988470599,226.616779048904,19.3649685390728));
#86690=CARTESIAN_POINT('Ctrl Pts',(-156.877197967362,223.143422642792,19.2062106738411));
#86691=CARTESIAN_POINT('Ctrl Pts',(-159.865978945628,221.369750585662,19.0474528086092));
#86692=CARTESIAN_POINT('Ctrl Pts',(-162.574488163549,222.717816747864,18.9092414349364));
#86693=CARTESIAN_POINT('Ctrl Pts',(-163.066355225813,224.374657820191,18.8239493496742));
#86694=CARTESIAN_POINT('Ctrl Pts',(-163.069604839599,225.001742689702,18.7915765528225));
#86695=CARTESIAN_POINT('Ctrl Pts',(-158.086534003335,226.635987203375,20.));
#86696=CARTESIAN_POINT('Ctrl Pts',(-157.542565484547,225.999756515379,19.9470807115894));
#86697=CARTESIAN_POINT('Ctrl Pts',(-157.149565275988,224.151956162406,19.8412421347682));
#86698=CARTESIAN_POINT('Ctrl Pts',(-159.168282436654,222.141301994169,19.6824842695364));
#86699=CARTESIAN_POINT('Ctrl Pts',(-161.94954585807,222.752591068708,19.5237264043046));
#86700=CARTESIAN_POINT('Ctrl Pts',(-162.945990110181,225.417945100886,19.3649685390728));
#86701=CARTESIAN_POINT('Ctrl Pts',(-161.24655750239,227.702119685951,19.206210673841));
#86702=CARTESIAN_POINT('Ctrl Pts',(-158.406134657523,227.512676050035,19.0474528086092));
#86703=CARTESIAN_POINT('Ctrl Pts',(-157.024485236765,225.023939011451,18.8886949433775));
#86704=CARTESIAN_POINT('Ctrl Pts',(-158.3659940775,222.513144734576,18.7299370781456));
#86705=CARTESIAN_POINT('Ctrl Pts',(-161.202960849655,222.278391748584,18.5711792129139));
#86706=CARTESIAN_POINT('Ctrl Pts',(-162.938970296779,224.534420092962,18.4124213476821));
#86707=CARTESIAN_POINT('Ctrl Pts',(-161.985237907903,227.216563745114,18.2536634824503));
#86708=CARTESIAN_POINT('Ctrl Pts',(-159.214614097946,227.87010034708,18.0949056172185));
#86709=CARTESIAN_POINT('Ctrl Pts',(-157.162776285685,225.896925078708,17.9361477519867));
#86710=CARTESIAN_POINT('Ctrl Pts',(-157.707565095056,223.102882155973,17.7773898867549));
#86711=CARTESIAN_POINT('Ctrl Pts',(-160.350390436945,222.045082304735,17.6186320215231));
#86712=CARTESIAN_POINT('Ctrl Pts',(-162.67253836946,223.691622580552,17.4598741562913));
#86713=CARTESIAN_POINT('Ctrl Pts',(-162.54877933725,226.535590027129,17.3011162910595));
#86714=CARTESIAN_POINT('Ctrl Pts',(-160.092377533692,227.974185441053,17.1423584258277));
#86715=CARTESIAN_POINT('Ctrl Pts',(-157.551431825594,226.690806504577,16.9836005605959));
#86716=CARTESIAN_POINT('Ctrl Pts',(-157.251415609286,223.860001498326,16.8248426953641));
#86717=CARTESIAN_POINT('Ctrl Pts',(-159.466903721751,222.072523087195,16.6660848301324));
#86718=CARTESIAN_POINT('Ctrl Pts',(-162.170281525912,222.964271426136,16.5073269649006));
#86719=CARTESIAN_POINT('Ctrl Pts',(-162.887417763478,225.71911847843,16.3485690996688));
#86720=CARTESIAN_POINT('Ctrl Pts',(-160.961989377177,227.815828326288,16.189811234437));
#86721=CARTESIAN_POINT('Ctrl Pts',(-158.156148350846,227.335492201262,16.0310533692052));
#86722=CARTESIAN_POINT('Ctrl Pts',(-157.037800281249,224.71771370519,15.8722955039734));
#86723=CARTESIAN_POINT('Ctrl Pts',(-158.630457277798,222.358283615169,15.7135376387416));
#86724=CARTESIAN_POINT('Ctrl Pts',(-161.476519719835,222.416552256594,15.5547797735098));
#86725=CARTESIAN_POINT('Ctrl Pts',(-162.971271372349,224.839192171226,15.396021908278));
#86726=CARTESIAN_POINT('Ctrl Pts',(-161.746715581728,227.409003404412,15.2372640430462));
#86727=CARTESIAN_POINT('Ctrl Pts',(-158.923565759399,227.77409481662,15.0785061778144));
#86728=CARTESIAN_POINT('Ctrl Pts',(-157.085568511738,225.600334761742,14.9197483125827));
#86729=CARTESIAN_POINT('Ctrl Pts',(-157.914858847527,222.877148356527,14.7609904473508));
#86730=CARTESIAN_POINT('Ctrl Pts',(-160.652470284063,222.096795691938,14.6022325821191));
#86731=CARTESIAN_POINT('Ctrl Pts',(-162.792940942283,223.973455495923,14.4434747168873));
#86732=CARTESIAN_POINT('Ctrl Pts',(-162.377312159954,226.78960878967,14.2847168516555));
#86733=CARTESIAN_POINT('Ctrl Pts',(-159.785967382321,227.967912189486,14.1259589864237));
#86734=CARTESIAN_POINT('Ctrl Pts',(-157.390505247971,226.429982470195,13.9672011211919));
#86735=CARTESIAN_POINT('Ctrl Pts',(-157.383252608062,223.583332850414,13.8084432559601));
#86736=CARTESIAN_POINT('Ctrl Pts',(-159.770847078353,222.033216950225,13.6496853907283));
#86737=CARTESIAN_POINT('Ctrl Pts',(-162.368162293525,223.198300780524,13.4909275254965));
#86738=CARTESIAN_POINT('Ctrl Pts',(-162.798135470788,226.012299665637,13.3321696602647));
#86739=CARTESIAN_POINT('Ctrl Pts',(-160.66725517522,227.899841936567,13.1734117950329));
#86740=CARTESIAN_POINT('Ctrl Pts',(-157.92570296953,227.133448981184,13.0146539298011));
#86741=CARTESIAN_POINT('Ctrl Pts',(-157.082547324556,224.414523602118,12.8558960645693));
#86742=CARTESIAN_POINT('Ctrl Pts',(-158.909444253422,222.231426199369,12.6971381993375));
#86743=CARTESIAN_POINT('Ctrl Pts',(-161.734417758671,222.582127430087,12.5383803341058));
#86744=CARTESIAN_POINT('Ctrl Pts',(-162.972052199389,225.145665541708,12.379622468874));
#86745=CARTESIAN_POINT('Ctrl Pts',(-161.489664584098,227.575890555287,12.2208646036422));
#86746=CARTESIAN_POINT('Ctrl Pts',(-158.643936000021,227.648660633961,12.0621067384104));
#86747=CARTESIAN_POINT('Ctrl Pts',(-157.039277135399,225.29737660459,11.9033488731786));
#86748=CARTESIAN_POINT('Ctrl Pts',(-158.144271720032,222.673933518393,11.7445910079468));
#86749=CARTESIAN_POINT('Ctrl Pts',(-160.947628753517,222.179306384692,11.585833142715));
#86750=CARTESIAN_POINT('Ctrl Pts',(-162.883715989048,224.2661779368,11.4270752774832));
#86751=CARTESIAN_POINT('Ctrl Pts',(-162.180626464802,227.024643412292,11.2683174122514));
#86752=CARTESIAN_POINT('Ctrl Pts',(-159.48182768572,227.930155316471,11.1095595470196));
#86753=CARTESIAN_POINT('Ctrl Pts',(-157.25726018829,226.153989190242,10.9508016817878));
#86754=CARTESIAN_POINT('Ctrl Pts',(-157.542848058682,223.321692202482,10.792043816556));
#86755=CARTESIAN_POINT('Ctrl Pts',(-160.077221289143,222.025382445013,10.6332859513242));
#86756=CARTESIAN_POINT('Ctrl Pts',(-162.540921598817,223.451442556894,10.4745280860925));
#86757=CARTESIAN_POINT('Ctrl Pts',(-162.679170561173,226.29474237981,10.3157702208607));
#86758=CARTESIAN_POINT('Ctrl Pts',(-160.3654427313,227.953094027638,10.1570123556289));
#86759=CARTESIAN_POINT('Ctrl Pts',(-157.717261728112,226.9087741375,9.99825449039708));
#86760=CARTESIAN_POINT('Ctrl Pts',(-157.158242701589,224.117544231782,9.83949662516528));
#86761=CARTESIAN_POINT('Ctrl Pts',(-159.199999842823,222.133937810436,9.6807387599335));
#86762=CARTESIAN_POINT('Ctrl Pts',(-161.973917096446,222.773351392274,9.5219808947017));
#86763=CARTESIAN_POINT('Ctrl Pts',(-162.941305501024,225.450593692342,9.36322302946991));
#86764=CARTESIAN_POINT('Ctrl Pts',(-161.216811226729,227.715452662898,9.20446516423812));
#86765=CARTESIAN_POINT('Ctrl Pts',(-158.378691365582,227.495129463153,9.04570729900632));
#86766=CARTESIAN_POINT('Ctrl Pts',(-157.024393102897,224.991263876849,8.88694943377453));
#86767=CARTESIAN_POINT('Ctrl Pts',(-158.393370155429,222.495393590109,8.72819156854274));
#86768=CARTESIAN_POINT('Ctrl Pts',(-161.232734778532,222.291738991211,8.56943370331094));
#86769=CARTESIAN_POINT('Ctrl Pts',(-162.943900580799,224.566684761056,8.41067583807915));
#86770=CARTESIAN_POINT('Ctrl Pts',(-161.960808687285,227.238200620543,8.25191797284736));
#86771=CARTESIAN_POINT('Ctrl Pts',(-159.183184760274,227.861315360124,8.09316010761557));
#86772=CARTESIAN_POINT('Ctrl Pts',(-157.15311010854,225.865754394638,7.93440224238377));
#86773=CARTESIAN_POINT('Ctrl Pts',(-157.728508973519,223.077855041224,7.77564437715198));
#86774=CARTESIAN_POINT('Ctrl Pts',(-160.382776336609,222.049102678496,7.6168865119202));
#86775=CARTESIAN_POINT('Ctrl Pts',(-162.686726811487,223.721011428366,7.4581286466884));
#86776=CARTESIAN_POINT('Ctrl Pts',(-162.531785014145,226.563450468702,7.29937078145661));
#86777=CARTESIAN_POINT('Ctrl Pts',(-160.059753671418,227.975019701562,7.14061291622482));
#86778=CARTESIAN_POINT('Ctrl Pts',(-157.533035770958,226.663851020543,6.98185505099302));
#86779=CARTESIAN_POINT('Ctrl Pts',(-157.264083435908,223.829925950952,6.82309718576123));
#86780=CARTESIAN_POINT('Ctrl Pts',(-159.499041832727,222.066852605038,6.66433932052944));
#86781=CARTESIAN_POINT('Ctrl Pts',(-162.192477124534,222.98819563965,6.50558145529764));
#86782=CARTESIAN_POINT('Ctrl Pts',(-162.879357438186,225.750741945742,6.34682359006585));
#86783=CARTESIAN_POINT('Ctrl Pts',(-160.931049937637,227.826209252613,6.18806572483406));
#86784=CARTESIAN_POINT('Ctrl Pts',(-158.130645570776,227.315129962631,6.02930785960227));
#86785=CARTESIAN_POINT('Ctrl Pts',(-157.04107430403,224.685243821889,5.87054999437047));
#86786=CARTESIAN_POINT('Ctrl Pts',(-158.659511717879,222.343422522977,5.71179212913868));
#86787=CARTESIAN_POINT('Ctrl Pts',(-161.504763954812,222.432900826569,5.55303426390689));
#86788=CARTESIAN_POINT('Ctrl Pts',(-162.972856279474,224.871788192736,5.39427639867509));
#86789=CARTESIAN_POINT('Ctrl Pts',(-161.720190654067,227.42801499987,5.23551853344331));
#86790=CARTESIAN_POINT('Ctrl Pts',(-158.893206609702,227.762122574602,5.07676066821151));
#86791=CARTESIAN_POINT('Ctrl Pts',(-157.079159832615,225.568335677676,4.91800280297972));
#86792=CARTESIAN_POINT('Ctrl Pts',(-157.938265861858,222.854407990891,4.75924493774793));
#86793=CARTESIAN_POINT('Ctrl Pts',(-160.684270893255,222.104126026468,4.60048707251613));
#86794=CARTESIAN_POINT('Ctrl Pts',(-162.80403123005,224.004147808747,4.44172920728434));
#86795=CARTESIAN_POINT('Ctrl Pts',(-162.357542295375,226.815573477294,4.28297134205255));
#86796=CARTESIAN_POINT('Ctrl Pts',(-159.753430744669,227.965386370829,4.12421347682076));
#86797=CARTESIAN_POINT('Ctrl Pts',(-157.37497936677,226.401277774369,3.96545561158896));
#86798=CARTESIAN_POINT('Ctrl Pts',(-157.398946769126,223.554719813958,3.80669774635717));
#86799=CARTESIAN_POINT('Ctrl Pts',(-159.803397986199,222.03088222288,3.64793988112538));
#86800=CARTESIAN_POINT('Ctrl Pts',(-162.387779358353,223.224381104868,3.48918201589359));
#86801=CARTESIAN_POINT('Ctrl Pts',(-162.786865156092,226.042926329434,3.3304241506618));
#86802=CARTESIAN_POINT('Ctrl Pts',(-160.635412071627,227.906985419191,3.17166628543));
#86803=CARTESIAN_POINT('Ctrl Pts',(-157.902429886146,227.110571565798,3.01290842019822));
#86804=CARTESIAN_POINT('Ctrl Pts',(-157.089143782333,224.382562702162,2.85415055496642));
#86805=CARTESIAN_POINT('Ctrl Pts',(-158.939873182857,222.219632421386,2.69539268973463));
#86806=CARTESIAN_POINT('Ctrl Pts',(-161.760830587323,222.601294455492,2.53663482450283));
#86807=CARTESIAN_POINT('Ctrl Pts',(-162.970275943658,225.178251675845,2.37787695927104));
#86808=CARTESIAN_POINT('Ctrl Pts',(-161.461324798163,227.592073039525,2.21911909403925));
#86809=CARTESIAN_POINT('Ctrl Pts',(-158.61496941047,227.633629114009,2.06036122880746));
#86810=CARTESIAN_POINT('Ctrl Pts',(-157.036193640954,225.264888228518,1.90160336357567));
#86811=CARTESIAN_POINT('Ctrl Pts',(-158.169894004685,222.653721020893,1.74284549834387));
#86812=CARTESIAN_POINT('Ctrl Pts',(-160.978505913143,222.189869541214,1.58408763311208));
#86813=CARTESIAN_POINT('Ctrl Pts',(-162.891592133019,224.297846652507,1.42532976788028));
#86814=CARTESIAN_POINT('Ctrl Pts',(-162.158287360937,227.048440070593,1.2665719026485));
#86815=CARTESIAN_POINT('Ctrl Pts',(-159.449730500729,227.924289615984,1.1078140374167));
#86816=CARTESIAN_POINT('Ctrl Pts',(-157.244754494171,226.123853490694,0.94905617218491));
#86817=CARTESIAN_POINT('Ctrl Pts',(-157.561432538852,223.294816748872,0.790298306953121));
#86818=CARTESIAN_POINT('Ctrl Pts',(-160.109776474582,222.026467288224,0.631540441721325));
#86819=CARTESIAN_POINT('Ctrl Pts',(-162.557883210969,223.479279814359,0.472782576489533));
#86820=CARTESIAN_POINT('Ctrl Pts',(-162.664537639372,226.324301704676,0.314024711257741));
#86821=CARTESIAN_POINT('Ctrl Pts',(-160.333598837337,227.956397769736,0.155266846025946));
#86822=CARTESIAN_POINT('Ctrl Pts',(-157.69529473125,226.88473924401,-0.00349101920584214));
#86823=CARTESIAN_POINT('Ctrl Pts',(-157.170583964077,224.084270038712,-0.162248884437638));
#86824=CARTESIAN_POINT('Ctrl Pts',(-158.541127016969,222.784105799646,-0.268087461258832));
#86825=CARTESIAN_POINT('Ctrl Pts',(-159.349800002025,222.567913197965,-0.32100674966943));
#86826=CARTESIAN_POINT('Ctrl Pts',(-157.945668449658,226.756425321227,20.1070022498898));
#86827=CARTESIAN_POINT('Ctrl Pts',(-157.361654052493,226.073356597808,20.0540829614792));
#86828=CARTESIAN_POINT('Ctrl Pts',(-156.939721951717,224.089524864994,19.948244384658));
#86829=CARTESIAN_POINT('Ctrl Pts',(-159.107053047018,221.930850343558,19.7894865194262));
#86830=CARTESIAN_POINT('Ctrl Pts',(-162.093067539247,222.587141301637,19.6307286541944));
#86831=CARTESIAN_POINT('Ctrl Pts',(-163.162868031566,225.448713386366,19.4719707889626));
#86832=CARTESIAN_POINT('Ctrl Pts',(-161.338326581679,227.90104435267,19.3132129237309));
#86833=CARTESIAN_POINT('Ctrl Pts',(-158.288797467133,227.697654253785,19.1544550584991));
#86834=CARTESIAN_POINT('Ctrl Pts',(-156.805433769257,225.025701353771,18.9956971932673));
#86835=CARTESIAN_POINT('Ctrl Pts',(-158.245701817598,222.330067405536,18.8369393280355));
#86836=CARTESIAN_POINT('Ctrl Pts',(-161.291520430245,222.078032372512,18.6781814628037));
#86837=CARTESIAN_POINT('Ctrl Pts',(-163.155331433491,224.500145027974,18.5194235975719));
#86838=CARTESIAN_POINT('Ctrl Pts',(-162.131387166664,227.379742751044,18.3606657323401));
#86839=CARTESIAN_POINT('Ctrl Pts',(-159.156795552889,228.081391415333,18.2019078671083));
#86840=CARTESIAN_POINT('Ctrl Pts',(-156.953905529623,225.962954915685,18.0431500018765));
#86841=CARTESIAN_POINT('Ctrl Pts',(-157.538800605529,222.963220120716,17.8843921366447));
#86842=CARTESIAN_POINT('Ctrl Pts',(-160.376185482683,221.827547152327,17.7256342714129));
#86843=CARTESIAN_POINT('Ctrl Pts',(-162.869285318606,223.595302442159,17.5668764061811));
#86844=CARTESIAN_POINT('Ctrl Pts',(-162.736415393061,226.648637104929,17.4081185409493));
#86845=CARTESIAN_POINT('Ctrl Pts',(-160.09917818364,228.193139046512,17.2493606757176));
#86846=CARTESIAN_POINT('Ctrl Pts',(-157.3711731159,226.815280310145,17.0906028104857));
#86847=CARTESIAN_POINT('Ctrl Pts',(-157.049070303595,223.776077080328,16.931844945254));
#86848=CARTESIAN_POINT('Ctrl Pts',(-159.427658236056,221.857008070509,16.7730870800222));
#86849=CARTESIAN_POINT('Ctrl Pts',(-162.330053327091,222.814405145161,16.6143292147904));
#86850=CARTESIAN_POINT('Ctrl Pts',(-163.099983705417,225.772058547812,16.4555713495586));
#86851=CARTESIAN_POINT('Ctrl Pts',(-161.032809118151,228.023123996518,16.2968134843268));
#86852=CARTESIAN_POINT('Ctrl Pts',(-158.020407666711,227.507426483142,16.138055619095));
#86853=CARTESIAN_POINT('Ctrl Pts',(-156.819729040783,224.696932350683,15.9792977538632));
#86854=CARTESIAN_POINT('Ctrl Pts',(-158.529634271702,222.163805719112,15.8205398886314));
#86855=CARTESIAN_POINT('Ctrl Pts',(-161.585218159323,222.226363981806,15.6617820233996));
#86856=CARTESIAN_POINT('Ctrl Pts',(-163.190010449876,224.827353819316,15.5030241581678));
#86857=CARTESIAN_POINT('Ctrl Pts',(-161.875305302144,227.586349434581,15.3442662929361));
#86858=CARTESIAN_POINT('Ctrl Pts',(-158.844320815635,227.978318149032,15.1855084277042));
#86859=CARTESIAN_POINT('Ctrl Pts',(-156.871013873211,225.644530210604,15.0267505624725));
#86860=CARTESIAN_POINT('Ctrl Pts',(-157.76135491098,222.720868248779,14.8679926972406));
#86861=CARTESIAN_POINT('Ctrl Pts',(-160.700503846187,221.883067576046,14.7092348320089));
#86862=CARTESIAN_POINT('Ctrl Pts',(-162.998551688911,223.897883335145,14.5504769667771));
#86863=CARTESIAN_POINT('Ctrl Pts',(-162.552325143858,226.92135622258,14.3917191015453));
#86864=CARTESIAN_POINT('Ctrl Pts',(-159.770210727515,228.186403970666,14.2329612363135));
#86865=CARTESIAN_POINT('Ctrl Pts',(-157.198399444313,226.535254930099,14.0742033710817));
#86866=CARTESIAN_POINT('Ctrl Pts',(-157.190612879506,223.479040637879,13.9154455058499));
#86867=CARTESIAN_POINT('Ctrl Pts',(-159.753977296899,221.814808294061,13.7566876406181));
#86868=CARTESIAN_POINT('Ctrl Pts',(-162.542501682495,223.065663274264,13.5979297753863));
#86869=CARTESIAN_POINT('Ctrl Pts',(-163.004128628254,226.086823149794,13.4391719101545));
#86870=CARTESIAN_POINT('Ctrl Pts',(-160.716377171569,228.113322521371,13.2804140449227));
#86871=CARTESIAN_POINT('Ctrl Pts',(-157.772997355635,227.290509243817,13.1216561796909));
#86872=CARTESIAN_POINT('Ctrl Pts',(-156.867770272249,224.371421996394,12.9628983144592));
#86873=CARTESIAN_POINT('Ctrl Pts',(-158.829159712529,222.027609313153,12.8041404492274));
#86874=CARTESIAN_POINT('Ctrl Pts',(-161.86210213786,222.404128469628,12.6453825839956));
#86875=CARTESIAN_POINT('Ctrl Pts',(-163.190848759847,225.156389148619,12.4866247187638));
#86876=CARTESIAN_POINT('Ctrl Pts',(-161.599330722299,227.765522484944,12.327866853532));
#86877=CARTESIAN_POINT('Ctrl Pts',(-158.544105270595,227.8436497518,12.1691089883002));
#86878=CARTESIAN_POINT('Ctrl Pts',(-156.821314617991,225.319268877632,12.0103511230684));
#86879=CARTESIAN_POINT('Ctrl Pts',(-158.007656702003,222.50269313921,11.8515932578366));
#86880=CARTESIAN_POINT('Ctrl Pts',(-161.017391293994,221.971652541579,11.6928353926048));
#86881=CARTESIAN_POINT('Ctrl Pts',(-163.09600941373,224.212155418808,11.534077527373));
#86882=CARTESIAN_POINT('Ctrl Pts',(-162.341159839768,227.173693625762,11.3753196621412));
#86883=CARTESIAN_POINT('Ctrl Pts',(-159.443680872514,228.145867511898,11.2165617969094));
#86884=CARTESIAN_POINT('Ctrl Pts',(-157.055345148858,226.238943574853,11.0578039316776));
#86885=CARTESIAN_POINT('Ctrl Pts',(-157.361957429172,223.198138526823,10.8990460664458));
#86886=CARTESIAN_POINT('Ctrl Pts',(-160.082906166569,221.806397028188,10.7402882012141));
#86887=CARTESIAN_POINT('Ctrl Pts',(-162.727979183582,223.33744084377,10.5815303359823));
#86888=CARTESIAN_POINT('Ctrl Pts',(-162.876405759056,226.390058733755,10.4227724707505));
#86889=CARTESIAN_POINT('Ctrl Pts',(-160.392345896954,228.17049492527,10.2640146055187));
#86890=CARTESIAN_POINT('Ctrl Pts',(-157.549211085388,227.049294285855,10.1052567402869));
#86891=CARTESIAN_POINT('Ctrl Pts',(-156.9490381921,224.052579596611,9.94649887505509));
#86892=CARTESIAN_POINT('Ctrl Pts',(-159.141105425426,221.922944023293,9.7877410098233));
#86893=CARTESIAN_POINT('Ctrl Pts',(-162.119232939627,222.609429958855,9.62898314459152));
#86894=CARTESIAN_POINT('Ctrl Pts',(-163.157838550818,225.483765502066,9.47022527935971));
#86895=CARTESIAN_POINT('Ctrl Pts',(-161.306390444479,227.91535887681,9.31146741412793));
#86896=CARTESIAN_POINT('Ctrl Pts',(-158.259333854726,227.678815922141,9.15270954889614));
#86897=CARTESIAN_POINT('Ctrl Pts',(-156.805334852677,224.990620740871,8.99395168366434));
#86898=CARTESIAN_POINT('Ctrl Pts',(-158.275093267831,222.311009457187,8.83519381843255));
#86899=CARTESIAN_POINT('Ctrl Pts',(-161.323486256436,222.092362212543,8.67643595320076));
#86900=CARTESIAN_POINT('Ctrl Pts',(-163.160624675195,224.53478495664,8.51767808796896));
#86901=CARTESIAN_POINT('Ctrl Pts',(-162.105159515504,227.402972490126,8.35892022273717));
#86902=CARTESIAN_POINT('Ctrl Pts',(-159.123052450008,228.071959695143,8.20016235750538));
#86903=CARTESIAN_POINT('Ctrl Pts',(-156.943527747778,225.929489507967,8.04140449227359));
#86904=CARTESIAN_POINT('Ctrl Pts',(-157.56128633059,222.936350559651,7.88264662704179));
#86905=CARTESIAN_POINT('Ctrl Pts',(-160.410955567745,221.831863497991,7.72388876181));
#86906=CARTESIAN_POINT('Ctrl Pts',(-162.884518285461,223.626854838386,7.56513089657821));
#86907=CARTESIAN_POINT('Ctrl Pts',(-162.718169981753,226.678548576692,7.40637303134641));
#86908=CARTESIAN_POINT('Ctrl Pts',(-160.064152617635,228.194034723617,7.24761516611462));
#86909=CARTESIAN_POINT('Ctrl Pts',(-157.35142278038,226.78634041709,7.08885730088283));
#86910=CARTESIAN_POINT('Ctrl Pts',(-157.062670710368,223.743787431088,6.93009943565105));
#86911=CARTESIAN_POINT('Ctrl Pts',(-159.46216229072,221.850920138755,6.77134157041924));
#86912=CARTESIAN_POINT('Ctrl Pts',(-162.353882921455,222.840090611599,6.61258370518746));
#86913=CARTESIAN_POINT('Ctrl Pts',(-163.091329995038,225.806010071771,6.45382583995566));
#86914=CARTESIAN_POINT('Ctrl Pts',(-160.999591978726,228.034269145954,6.29506797472387));
#86915=CARTESIAN_POINT('Ctrl Pts',(-157.993027422792,227.48556521708,6.13631010949207));
#86916=CARTESIAN_POINT('Ctrl Pts',(-156.823244090596,224.662072099277,5.97755224426028));
#86917=CARTESIAN_POINT('Ctrl Pts',(-158.560827641764,222.147850582927,5.81879437902849));
#86918=CARTESIAN_POINT('Ctrl Pts',(-161.615541678595,222.243916100925,5.6600365137967));
#86919=CARTESIAN_POINT('Ctrl Pts',(-163.191712034706,224.862349494975,5.50127864856491));
#86920=CARTESIAN_POINT('Ctrl Pts',(-161.846827662165,227.606760625812,5.34252078333311));
#86921=CARTESIAN_POINT('Ctrl Pts',(-158.811726685835,227.965464534414,5.18376291810132));
#86922=CARTESIAN_POINT('Ctrl Pts',(-156.864133399902,225.610175417734,5.02500505286953));
#86923=CARTESIAN_POINT('Ctrl Pts',(-157.786485103062,222.696453782739,4.86624718763774));
#86924=CARTESIAN_POINT('Ctrl Pts',(-160.734645552858,221.890937555196,4.70748932240594));
#86925=CARTESIAN_POINT('Ctrl Pts',(-163.010458421564,223.930835154879,4.54873145717415));
#86926=CARTESIAN_POINT('Ctrl Pts',(-162.531099861244,226.949232378767,4.38997359194236));
#86927=CARTESIAN_POINT('Ctrl Pts',(-159.735278807435,228.183692206272,4.23121572671057));
#86928=CARTESIAN_POINT('Ctrl Pts',(-157.181730578677,226.504437051767,4.07245786147877));
#86929=CARTESIAN_POINT('Ctrl Pts',(-157.207462413434,223.448321166697,3.91369999624699));
#86930=CARTESIAN_POINT('Ctrl Pts',(-159.788924537715,221.812301688742,3.75494213101519));
#86931=CARTESIAN_POINT('Ctrl Pts',(-162.563562916545,223.093663580116,3.5961842657834));
#86932=CARTESIAN_POINT('Ctrl Pts',(-162.992028615448,226.119704487549,3.4374264005516));
#86933=CARTESIAN_POINT('Ctrl Pts',(-160.682189842143,228.120991892951,3.27866853531981));
#86934=CARTESIAN_POINT('Ctrl Pts',(-157.748010954229,227.265947638699,3.11991067008802));
#86935=CARTESIAN_POINT('Ctrl Pts',(-156.874852348103,224.337108198673,2.96115280485623));
#86936=CARTESIAN_POINT('Ctrl Pts',(-158.861828759113,222.014947300736,2.80239493962444));
#86937=CARTESIAN_POINT('Ctrl Pts',(-161.890459426324,222.424706533249,2.64363707439264));
#86938=CARTESIAN_POINT('Ctrl Pts',(-163.188941739709,225.191374209016,2.48487920916085));
#86939=CARTESIAN_POINT('Ctrl Pts',(-161.568904617796,227.782896291425,2.32612134392906));
#86940=CARTESIAN_POINT('Ctrl Pts',(-158.513006218444,227.827511641304,2.16736347869727));
#86941=CARTESIAN_POINT('Ctrl Pts',(-156.81800412283,225.284388772055,2.00860561346547));
#86942=CARTESIAN_POINT('Ctrl Pts',(-158.035165248194,222.480992637923,1.84984774823368));
#86943=CARTESIAN_POINT('Ctrl Pts',(-161.050541568583,221.982993336634,1.69108988300189));
#86944=CARTESIAN_POINT('Ctrl Pts',(-163.104465383725,224.246155522258,1.5323320177701));
#86945=CARTESIAN_POINT('Ctrl Pts',(-162.317176175592,227.199242146627,1.37357415253831));
#86946=CARTESIAN_POINT('Ctrl Pts',(-159.409220756724,228.139569990229,1.21481628730651));
#86947=CARTESIAN_POINT('Ctrl Pts',(-157.041918810458,226.206589345156,1.05605842207472));
#86948=CARTESIAN_POINT('Ctrl Pts',(-157.381910061739,223.169284555873,0.897300556842932));
#86949=CARTESIAN_POINT('Ctrl Pts',(-160.117857999888,221.807561735395,0.738542691611135));
#86950=CARTESIAN_POINT('Ctrl Pts',(-162.746189475821,223.367327424658,0.579784826379343));
#86951=CARTESIAN_POINT('Ctrl Pts',(-162.860695590711,226.421794157215,0.421026961147551));
#86952=CARTESIAN_POINT('Ctrl Pts',(-160.358157718974,228.174041882278,0.262269095915756));
#86953=CARTESIAN_POINT('Ctrl Pts',(-157.525626921991,227.023489991401,0.103511230683968));
#86954=CARTESIAN_POINT('Ctrl Pts',(-156.96228799374,224.016855823753,-0.055246634547828));
#86955=CARTESIAN_POINT('Ctrl Pts',(-158.43372769508,222.620976084267,-0.161085211369022));
#86956=CARTESIAN_POINT('Ctrl Pts',(-159.301933573839,222.388867814061,-0.21400449977962));
#86957=CARTESIAN_POINT('Ctrl Pts',(-157.804802895981,226.876863439079,20.2140044997796));
#86958=CARTESIAN_POINT('Ctrl Pts',(-157.180742620438,226.146956680238,20.161085211369));
#86959=CARTESIAN_POINT('Ctrl Pts',(-156.729878627447,224.027093567582,20.0552466345478));
#86960=CARTESIAN_POINT('Ctrl Pts',(-159.045823657383,221.720398692947,19.896488769316));
#86961=CARTESIAN_POINT('Ctrl Pts',(-162.236589220423,222.421691534567,19.7377309040842));
#86962=CARTESIAN_POINT('Ctrl Pts',(-163.379745952951,225.479481671847,19.5789730388525));
#86963=CARTESIAN_POINT('Ctrl Pts',(-161.430095660968,228.099969019388,19.4202151736207));
#86964=CARTESIAN_POINT('Ctrl Pts',(-158.171460276744,227.882632457535,19.2614573083889));
#86965=CARTESIAN_POINT('Ctrl Pts',(-156.586382301748,225.02746369609,19.1026994431571));
#86966=CARTESIAN_POINT('Ctrl Pts',(-158.125409557696,222.146990076495,18.9439415779253));
#86967=CARTESIAN_POINT('Ctrl Pts',(-161.380080010835,221.877672996439,18.7851837126935));
#86968=CARTESIAN_POINT('Ctrl Pts',(-163.371692570201,224.465869962988,18.6264258474617));
#86969=CARTESIAN_POINT('Ctrl Pts',(-162.277536425426,227.542921756974,18.4676679822299));
#86970=CARTESIAN_POINT('Ctrl Pts',(-159.098977007832,228.292682483585,18.3089101169981));
#86971=CARTESIAN_POINT('Ctrl Pts',(-156.745034773561,226.028984752661,18.1501522517663));
#86972=CARTESIAN_POINT('Ctrl Pts',(-157.370036116003,222.823558085459,17.9913943865345));
#86973=CARTESIAN_POINT('Ctrl Pts',(-160.401980528422,221.610011999918,17.8326365213027));
#86974=CARTESIAN_POINT('Ctrl Pts',(-163.066032267751,223.498982303766,17.6738786560709));
#86975=CARTESIAN_POINT('Ctrl Pts',(-162.924051448872,226.761684182729,17.5151207908392));
#86976=CARTESIAN_POINT('Ctrl Pts',(-160.105978833588,228.412092651971,17.3563629256073));
#86977=CARTESIAN_POINT('Ctrl Pts',(-157.190914406205,226.939754115711,17.1976050603756));
#86978=CARTESIAN_POINT('Ctrl Pts',(-156.846724997903,223.69215266233,17.0388471951438));
#86979=CARTESIAN_POINT('Ctrl Pts',(-159.388412750362,221.641493053823,16.880089329912));
#86980=CARTESIAN_POINT('Ctrl Pts',(-162.489825128271,222.664538864185,16.7213314646802));
#86981=CARTESIAN_POINT('Ctrl Pts',(-163.312549647356,225.824998617194,16.5625735994484));
#86982=CARTESIAN_POINT('Ctrl Pts',(-161.103628859126,228.230419666749,16.4038157342166));
#86983=CARTESIAN_POINT('Ctrl Pts',(-157.884666982576,227.679360765022,16.2450578689848));
#86984=CARTESIAN_POINT('Ctrl Pts',(-156.601657800316,224.676150996176,16.086300003753));
#86985=CARTESIAN_POINT('Ctrl Pts',(-158.428811265605,221.969327823056,15.9275421385212));
#86986=CARTESIAN_POINT('Ctrl Pts',(-161.69391659881,222.036175707019,15.7687842732894));
#86987=CARTESIAN_POINT('Ctrl Pts',(-163.408749527404,224.815515467406,15.6100264080576));
#86988=CARTESIAN_POINT('Ctrl Pts',(-162.00389502256,227.763695464751,15.4512685428258));
#86989=CARTESIAN_POINT('Ctrl Pts',(-158.765075871872,228.182541481444,15.2925106775941));
#86990=CARTESIAN_POINT('Ctrl Pts',(-156.656459234684,225.688725659466,15.1337528123623));
#86991=CARTESIAN_POINT('Ctrl Pts',(-157.607850974432,222.56458814103,14.9749949471305));
#86992=CARTESIAN_POINT('Ctrl Pts',(-160.748537408311,221.669339460152,14.8162370818987));
#86993=CARTESIAN_POINT('Ctrl Pts',(-163.204162435539,223.822311174369,14.6574792166669));
#86994=CARTESIAN_POINT('Ctrl Pts',(-162.727338127762,227.053103655491,14.4987213514351));
#86995=CARTESIAN_POINT('Ctrl Pts',(-159.754454072708,228.404895751845,14.3399634862033));
#86996=CARTESIAN_POINT('Ctrl Pts',(-157.006293640655,226.640527390004,14.1812056209715));
#86997=CARTESIAN_POINT('Ctrl Pts',(-156.99797315095,223.374748425344,14.0224477557397));
#86998=CARTESIAN_POINT('Ctrl Pts',(-159.737107515444,221.596399637898,13.8636898905079));
#86999=CARTESIAN_POINT('Ctrl Pts',(-162.716841071466,222.933025768004,13.7049320252761));
#87000=CARTESIAN_POINT('Ctrl Pts',(-163.210121785719,226.161346633951,13.5461741600443));
#87001=CARTESIAN_POINT('Ctrl Pts',(-160.765499167917,228.326803106175,13.3874162948126));
#87002=CARTESIAN_POINT('Ctrl Pts',(-157.62029174174,227.447569506451,13.2286584295807));
#87003=CARTESIAN_POINT('Ctrl Pts',(-156.652993219943,224.328320390671,13.069900564349));
#87004=CARTESIAN_POINT('Ctrl Pts',(-158.748875171636,221.823792426936,12.9111426991172));
#87005=CARTESIAN_POINT('Ctrl Pts',(-161.989786517048,222.226129509168,12.7523848338854));
#87006=CARTESIAN_POINT('Ctrl Pts',(-163.409645320305,225.167112755529,12.5936269686536));
#87007=CARTESIAN_POINT('Ctrl Pts',(-161.708996860499,227.955154414602,12.4348691034218));
#87008=CARTESIAN_POINT('Ctrl Pts',(-158.444274541169,228.038638869639,12.27611123819));
#87009=CARTESIAN_POINT('Ctrl Pts',(-156.603352100584,225.341161150675,12.1173533729582));
#87010=CARTESIAN_POINT('Ctrl Pts',(-157.871041683974,222.331452760028,11.9585955077264));
#87011=CARTESIAN_POINT('Ctrl Pts',(-161.087153834472,221.763998698466,11.7998376424946));
#87012=CARTESIAN_POINT('Ctrl Pts',(-163.308302838412,224.158132900815,11.6410797772628));
#87013=CARTESIAN_POINT('Ctrl Pts',(-162.501693214734,227.322743839232,11.482321912031));
#87014=CARTESIAN_POINT('Ctrl Pts',(-159.405534059307,228.361579707324,11.3235640467992));
#87015=CARTESIAN_POINT('Ctrl Pts',(-156.853430109426,226.323897959464,11.1648061815675));
#87016=CARTESIAN_POINT('Ctrl Pts',(-157.181066799662,223.074584851163,11.0060483163356));
#87017=CARTESIAN_POINT('Ctrl Pts',(-160.088591043995,221.587411611363,10.8472904511039));
#87018=CARTESIAN_POINT('Ctrl Pts',(-162.915036768348,223.223439130646,10.6885325858721));
#87019=CARTESIAN_POINT('Ctrl Pts',(-163.073640956939,226.485375087701,10.5297747206403));
#87020=CARTESIAN_POINT('Ctrl Pts',(-160.419249062608,228.387895822902,10.3710168554085));
#87021=CARTESIAN_POINT('Ctrl Pts',(-157.381160442664,227.189814434209,10.2122589901767));
#87022=CARTESIAN_POINT('Ctrl Pts',(-156.739833682611,223.98761496144,10.0535011249449));
#87023=CARTESIAN_POINT('Ctrl Pts',(-159.082211008029,221.71195023615,9.89474325971311));
#87024=CARTESIAN_POINT('Ctrl Pts',(-162.264548782808,222.445508525436,9.73598539448133));
#87025=CARTESIAN_POINT('Ctrl Pts',(-163.374371600612,225.51693731179,9.57722752924952));
#87026=CARTESIAN_POINT('Ctrl Pts',(-161.39596966223,228.115265090722,9.41846966401774));
#87027=CARTESIAN_POINT('Ctrl Pts',(-158.13997634387,227.86250238113,9.25971179878594));
#87028=CARTESIAN_POINT('Ctrl Pts',(-156.586276602457,224.989977604893,9.10095393355415));
#87029=CARTESIAN_POINT('Ctrl Pts',(-158.156816380233,222.126625324264,8.94219606832236));
#87030=CARTESIAN_POINT('Ctrl Pts',(-161.414237734339,221.892985433876,8.78343820309056));
#87031=CARTESIAN_POINT('Ctrl Pts',(-163.377348769591,224.502885152224,8.62468033785878));
#87032=CARTESIAN_POINT('Ctrl Pts',(-162.249510343725,227.567744359708,8.46592247262697));
#87033=CARTESIAN_POINT('Ctrl Pts',(-159.062920139741,228.282604030162,8.30716460739519));
#87034=CARTESIAN_POINT('Ctrl Pts',(-156.733945387017,225.993224621296,8.14840674216339));
#87035=CARTESIAN_POINT('Ctrl Pts',(-157.39406368766,222.794846078078,7.98964887693161));
#87036=CARTESIAN_POINT('Ctrl Pts',(-160.439134798881,221.614624317487,7.83089101169981));
#87037=CARTESIAN_POINT('Ctrl Pts',(-163.082309759434,223.532698248405,7.67213314646802));
#87038=CARTESIAN_POINT('Ctrl Pts',(-162.904554949362,226.793646684682,7.51337528123623));
#87039=CARTESIAN_POINT('Ctrl Pts',(-160.068551563853,228.413049745672,7.35461741600443));
#87040=CARTESIAN_POINT('Ctrl Pts',(-157.169809789801,226.908829813637,7.19585955077264));
#87041=CARTESIAN_POINT('Ctrl Pts',(-156.861257984829,223.657648911225,7.03710168554085));
#87042=CARTESIAN_POINT('Ctrl Pts',(-159.425282748714,221.634987672473,6.87834382030905));
#87043=CARTESIAN_POINT('Ctrl Pts',(-162.515288718375,222.691985583548,6.71958595507727));
#87044=CARTESIAN_POINT('Ctrl Pts',(-163.303302551891,225.861278197799,6.56082808984547));
#87045=CARTESIAN_POINT('Ctrl Pts',(-161.068134019816,228.242329039294,6.40207022461368));
#87046=CARTESIAN_POINT('Ctrl Pts',(-157.855409274808,227.656000471528,6.24331235938189));
#87047=CARTESIAN_POINT('Ctrl Pts',(-156.605413877162,224.638900376664,6.08455449415009));
#87048=CARTESIAN_POINT('Ctrl Pts',(-158.462143565649,221.952278642878,5.92579662891831));
#87049=CARTESIAN_POINT('Ctrl Pts',(-161.726319402379,222.05493137528,5.7670387636865));
#87050=CARTESIAN_POINT('Ctrl Pts',(-163.410567789938,224.852910797215,5.60828089845472));
#87051=CARTESIAN_POINT('Ctrl Pts',(-161.973464670263,227.785506251754,5.44952303322292));
#87052=CARTESIAN_POINT('Ctrl Pts',(-158.730246761968,228.168806494225,5.29076516799113));
#87053=CARTESIAN_POINT('Ctrl Pts',(-156.649106967188,225.652015157792,5.13200730275933));
#87054=CARTESIAN_POINT('Ctrl Pts',(-157.634704344266,222.538499574588,4.97324943752755));
#87055=CARTESIAN_POINT('Ctrl Pts',(-160.78502021246,221.677749083923,4.81449157229575));
#87056=CARTESIAN_POINT('Ctrl Pts',(-163.216885613078,223.857522501011,4.65573370706397));
#87057=CARTESIAN_POINT('Ctrl Pts',(-162.704657427114,227.08289128024,4.49697584183217));
#87058=CARTESIAN_POINT('Ctrl Pts',(-159.7171268702,228.401998041715,4.33821797660038));
#87059=CARTESIAN_POINT('Ctrl Pts',(-156.988481790584,226.607596329165,4.17946011136858));
#87060=CARTESIAN_POINT('Ctrl Pts',(-157.015978057742,223.341922519436,4.02070224613679));
#87061=CARTESIAN_POINT('Ctrl Pts',(-159.774451089232,221.593721154604,3.861944380905));
#87062=CARTESIAN_POINT('Ctrl Pts',(-162.739346474737,222.962946055363,3.70318651567321));
#87063=CARTESIAN_POINT('Ctrl Pts',(-163.197192074805,226.196482645664,3.54442865044142));
#87064=CARTESIAN_POINT('Ctrl Pts',(-160.728967612659,228.33499836671,3.38567078520962));
#87065=CARTESIAN_POINT('Ctrl Pts',(-157.593592022312,227.4213237116,3.22691291997783));
#87066=CARTESIAN_POINT('Ctrl Pts',(-156.660560913873,224.291653695184,3.06815505474604));
#87067=CARTESIAN_POINT('Ctrl Pts',(-158.783784335368,221.810262180086,2.90939718951425));
#87068=CARTESIAN_POINT('Ctrl Pts',(-162.020088265325,222.248118611005,2.75063932428246));
#87069=CARTESIAN_POINT('Ctrl Pts',(-163.407607535759,225.204496742187,2.59188145905066));
#87070=CARTESIAN_POINT('Ctrl Pts',(-161.676484437429,227.973719543325,2.43312359381887));
#87071=CARTESIAN_POINT('Ctrl Pts',(-158.411043026418,228.021394168598,2.27436572858708));
#87072=CARTESIAN_POINT('Ctrl Pts',(-156.599814604706,225.303889315591,2.11560786335528));
#87073=CARTESIAN_POINT('Ctrl Pts',(-157.900436491704,222.308264254952,1.95684999812349));
#87074=CARTESIAN_POINT('Ctrl Pts',(-161.122577224023,221.776117132055,1.7980921328917));
#87075=CARTESIAN_POINT('Ctrl Pts',(-163.317338634431,224.194464392009,1.6393342676599));
#87076=CARTESIAN_POINT('Ctrl Pts',(-162.476064990247,227.350044222662,1.48057640242812));
#87077=CARTESIAN_POINT('Ctrl Pts',(-159.36871101272,228.354850364474,1.32181853719632));
#87078=CARTESIAN_POINT('Ctrl Pts',(-156.839083126746,226.289325199618,1.16306067196453));
#87079=CARTESIAN_POINT('Ctrl Pts',(-157.202387584625,223.043752362873,1.00430280673274));
#87080=CARTESIAN_POINT('Ctrl Pts',(-160.125939525193,221.588656182565,0.845544941500944));
#87081=CARTESIAN_POINT('Ctrl Pts',(-162.934495740674,223.255375034957,0.686787076269154));
#87082=CARTESIAN_POINT('Ctrl Pts',(-163.056853542051,226.519286609754,0.528029211037361));
#87083=CARTESIAN_POINT('Ctrl Pts',(-160.38271660061,228.39168599482,0.369271345805566));
#87084=CARTESIAN_POINT('Ctrl Pts',(-157.355959112733,227.162240738792,0.210513480573778));
#87085=CARTESIAN_POINT('Ctrl Pts',(-156.753992023402,223.949441608794,0.0517556153419821));
#87086=CARTESIAN_POINT('Ctrl Pts',(-158.326328373191,222.457846368889,-0.0540829614792118));
#87087=CARTESIAN_POINT('Ctrl Pts',(-159.254067145653,222.209822430158,-0.10700224988981));
#87088=CARTESIAN_POINT('Ctrl Pts',(-157.663937342304,226.997301556931,20.3210067496694));
#87089=CARTESIAN_POINT('Ctrl Pts',(-156.999831188384,226.220556762668,20.2680874612588));
#87090=CARTESIAN_POINT('Ctrl Pts',(-156.520035303177,223.96466227017,20.1622488844377));
#87091=CARTESIAN_POINT('Ctrl Pts',(-158.984594267748,221.509947042336,20.0034910192058));
#87092=CARTESIAN_POINT('Ctrl Pts',(-162.3801109016,222.256241767497,19.8447331539741));
#87093=CARTESIAN_POINT('Ctrl Pts',(-163.596623874336,225.510249957328,19.6859752887423));
#87094=CARTESIAN_POINT('Ctrl Pts',(-161.521864740257,228.298893686106,19.5272174235105));
#87095=CARTESIAN_POINT('Ctrl Pts',(-158.054123086354,228.067610661284,19.3684595582787));
#87096=CARTESIAN_POINT('Ctrl Pts',(-156.367330834239,225.02922603841,19.2097016930469));
#87097=CARTESIAN_POINT('Ctrl Pts',(-158.005117297794,221.963912747455,19.0509438278151));
#87098=CARTESIAN_POINT('Ctrl Pts',(-161.468639591425,221.677313620367,18.8921859625833));
#87099=CARTESIAN_POINT('Ctrl Pts',(-163.588053706912,224.431594898001,18.7334280973515));
#87100=CARTESIAN_POINT('Ctrl Pts',(-162.423685684187,227.706100762903,18.5746702321197));
#87101=CARTESIAN_POINT('Ctrl Pts',(-159.041158462775,228.503973551838,18.4159123668879));
#87102=CARTESIAN_POINT('Ctrl Pts',(-156.536164017499,226.095014589637,18.2571545016561));
#87103=CARTESIAN_POINT('Ctrl Pts',(-157.201271626476,222.683896050202,18.0983966364243));
#87104=CARTESIAN_POINT('Ctrl Pts',(-160.427775574161,221.392476847509,17.9396387711926));
#87105=CARTESIAN_POINT('Ctrl Pts',(-163.262779216896,223.402662165373,17.7808809059608));
#87106=CARTESIAN_POINT('Ctrl Pts',(-163.111687504683,226.874731260529,17.622123040729));
#87107=CARTESIAN_POINT('Ctrl Pts',(-160.112779483536,228.631046257429,17.4633651754972));
#87108=CARTESIAN_POINT('Ctrl Pts',(-157.01065569651,227.064227921279,17.3046073102654));
#87109=CARTESIAN_POINT('Ctrl Pts',(-156.644379692211,223.608228244332,17.1458494450336));
#87110=CARTESIAN_POINT('Ctrl Pts',(-159.349167264668,221.425978037138,16.9870915798018));
#87111=CARTESIAN_POINT('Ctrl Pts',(-162.64959692945,222.514672583209,16.82833371457));
#87112=CARTESIAN_POINT('Ctrl Pts',(-163.525115589295,225.877938686576,16.6695758493382));
#87113=CARTESIAN_POINT('Ctrl Pts',(-161.1744486001,228.437715336979,16.5108179841064));
#87114=CARTESIAN_POINT('Ctrl Pts',(-157.748926298441,227.851295046903,16.3520601188746));
#87115=CARTESIAN_POINT('Ctrl Pts',(-156.383586559849,224.655369641669,16.1933022536428));
#87116=CARTESIAN_POINT('Ctrl Pts',(-158.327988259509,221.774849926999,16.034544388411));
#87117=CARTESIAN_POINT('Ctrl Pts',(-161.802615038297,221.845987432231,15.8757865231792));
#87118=CARTESIAN_POINT('Ctrl Pts',(-163.627488604931,224.803677115496,15.7170286579474));
#87119=CARTESIAN_POINT('Ctrl Pts',(-162.132484742975,227.94104149492,15.5582707927157));
#87120=CARTESIAN_POINT('Ctrl Pts',(-158.685830928108,228.386764813856,15.3995129274839));
#87121=CARTESIAN_POINT('Ctrl Pts',(-156.441904596157,225.732921108328,15.2407550622521));
#87122=CARTESIAN_POINT('Ctrl Pts',(-157.454347037885,222.408308033282,15.0819971970203));
#87123=CARTESIAN_POINT('Ctrl Pts',(-160.796570970435,221.455611344259,14.9232393317885));
#87124=CARTESIAN_POINT('Ctrl Pts',(-163.409773182167,223.746739013592,14.7644814665567));
#87125=CARTESIAN_POINT('Ctrl Pts',(-162.902351111666,227.184851088401,14.6057236013249));
#87126=CARTESIAN_POINT('Ctrl Pts',(-159.738697417901,228.623387533023,14.4469657360931));
#87127=CARTESIAN_POINT('Ctrl Pts',(-156.814187836997,226.745799849908,14.2882078708613));
#87128=CARTESIAN_POINT('Ctrl Pts',(-156.805333422394,223.270456212809,14.1294500056295));
#87129=CARTESIAN_POINT('Ctrl Pts',(-159.720237733989,221.377990981734,13.9706921403977));
#87130=CARTESIAN_POINT('Ctrl Pts',(-162.891180460436,222.800388261744,13.8119342751659));
#87131=CARTESIAN_POINT('Ctrl Pts',(-163.416114943184,226.235870118108,13.6531764099341));
#87132=CARTESIAN_POINT('Ctrl Pts',(-160.814621164266,228.540283690979,13.4944185447024));
#87133=CARTESIAN_POINT('Ctrl Pts',(-157.467586127845,227.604629769084,13.3356606794706));
#87134=CARTESIAN_POINT('Ctrl Pts',(-156.438216167636,224.285218784948,13.1769028142388));
#87135=CARTESIAN_POINT('Ctrl Pts',(-158.668590630742,221.61997554072,13.018144949007));
#87136=CARTESIAN_POINT('Ctrl Pts',(-162.117470896237,222.048130548708,12.8593870837752));
#87137=CARTESIAN_POINT('Ctrl Pts',(-163.628441880763,225.17783636244,12.7006292185434));
#87138=CARTESIAN_POINT('Ctrl Pts',(-161.8186629987,228.14478634426,12.5418713533116));
#87139=CARTESIAN_POINT('Ctrl Pts',(-158.344443811744,228.233627987479,12.3831134880798));
#87140=CARTESIAN_POINT('Ctrl Pts',(-156.385389583177,225.363053423717,12.224355622848));
#87141=CARTESIAN_POINT('Ctrl Pts',(-157.734426665945,222.160212380846,12.0655977576162));
#87142=CARTESIAN_POINT('Ctrl Pts',(-161.156916374949,221.556344855353,11.9068398923844));
#87143=CARTESIAN_POINT('Ctrl Pts',(-163.520596263094,224.104110382822,11.7480820271526));
#87144=CARTESIAN_POINT('Ctrl Pts',(-162.6622265897,227.471794052703,11.5893241619208));
#87145=CARTESIAN_POINT('Ctrl Pts',(-159.367387246101,228.577291902751,11.4305662966891));
#87146=CARTESIAN_POINT('Ctrl Pts',(-156.651515069994,226.408852344075,11.2718084314573));
#87147=CARTESIAN_POINT('Ctrl Pts',(-157.000176170152,222.951031175503,11.1130505662255));
#87148=CARTESIAN_POINT('Ctrl Pts',(-160.094275921422,221.368426194538,10.9542927009937));
#87149=CARTESIAN_POINT('Ctrl Pts',(-163.102094353113,223.109437417523,10.7955348357619));
#87150=CARTESIAN_POINT('Ctrl Pts',(-163.270876154823,226.580691441646,10.6367769705301));
#87151=CARTESIAN_POINT('Ctrl Pts',(-160.446152228262,228.605296720535,10.4780191052983));
#87152=CARTESIAN_POINT('Ctrl Pts',(-157.213109799941,227.330334582564,10.3192612400665));
#87153=CARTESIAN_POINT('Ctrl Pts',(-156.530629173122,223.922650326269,10.1605033748347));
#87154=CARTESIAN_POINT('Ctrl Pts',(-159.023316590632,221.500956449007,10.0017455096029));
#87155=CARTESIAN_POINT('Ctrl Pts',(-162.409864625989,222.281587092017,9.84298764437113));
#87156=CARTESIAN_POINT('Ctrl Pts',(-163.590904650406,225.550109121514,9.68422977913934));
#87157=CARTESIAN_POINT('Ctrl Pts',(-161.485548879981,228.315171304634,9.52547191390754));
#87158=CARTESIAN_POINT('Ctrl Pts',(-158.020618833015,228.046188840119,9.36671404867576));
#87159=CARTESIAN_POINT('Ctrl Pts',(-156.367218352237,224.989334468915,9.20795618344395));
#87160=CARTESIAN_POINT('Ctrl Pts',(-158.038539492636,221.942241191341,9.04919831821217));
#87161=CARTESIAN_POINT('Ctrl Pts',(-161.504989212242,221.693608655208,8.89044045298038));
#87162=CARTESIAN_POINT('Ctrl Pts',(-163.594072863987,224.470985347808,8.73168258774859));
#87163=CARTESIAN_POINT('Ctrl Pts',(-162.393861171944,227.732516229291,8.57292472251679));
#87164=CARTESIAN_POINT('Ctrl Pts',(-159.002787829475,228.493248365181,8.414166857285));
#87165=CARTESIAN_POINT('Ctrl Pts',(-156.524363026255,226.056959734625,8.2554089920532));
#87166=CARTESIAN_POINT('Ctrl Pts',(-157.226841044731,222.653341596505,8.09665112682142));
#87167=CARTESIAN_POINT('Ctrl Pts',(-160.467314030017,221.397385136983,7.93789326158962));
#87168=CARTESIAN_POINT('Ctrl Pts',(-163.280101233408,223.438541658425,7.77913539635783));
#87169=CARTESIAN_POINT('Ctrl Pts',(-163.090939916971,226.908744792673,7.62037753112604));
#87170=CARTESIAN_POINT('Ctrl Pts',(-160.07295051007,228.632064767727,7.46161966589424));
#87171=CARTESIAN_POINT('Ctrl Pts',(-156.988196799222,227.031319210184,7.30286180066245));
#87172=CARTESIAN_POINT('Ctrl Pts',(-156.65984525929,223.571510391361,7.14410393543066));
#87173=CARTESIAN_POINT('Ctrl Pts',(-159.388403206707,221.41905520619,6.98534607019887));
#87174=CARTESIAN_POINT('Ctrl Pts',(-162.676694515296,222.543880555497,6.82658820496707));
#87175=CARTESIAN_POINT('Ctrl Pts',(-163.515275108744,225.916546323828,6.66783033973529));
#87176=CARTESIAN_POINT('Ctrl Pts',(-161.136676060905,228.450388932634,6.50907247450349));
#87177=CARTESIAN_POINT('Ctrl Pts',(-157.717791126824,227.826435725977,6.3503146092717));
#87178=CARTESIAN_POINT('Ctrl Pts',(-156.387583663728,224.615728654052,6.1915567440399));
#87179=CARTESIAN_POINT('Ctrl Pts',(-158.363459489534,221.756706702828,6.03279887880811));
#87180=CARTESIAN_POINT('Ctrl Pts',(-161.837097126162,221.865946649636,5.87404101357632));
#87181=CARTESIAN_POINT('Ctrl Pts',(-163.62942354517,224.843472099454,5.71528314834452));
#87182=CARTESIAN_POINT('Ctrl Pts',(-162.100101678361,227.964251877696,5.55652528311274));
#87183=CARTESIAN_POINT('Ctrl Pts',(-158.648766838101,228.372148454037,5.39776741788094));
#87184=CARTESIAN_POINT('Ctrl Pts',(-156.434080534475,225.69385489785,5.23900955264915));
#87185=CARTESIAN_POINT('Ctrl Pts',(-157.48292358547,222.380545366436,5.08025168741736));
#87186=CARTESIAN_POINT('Ctrl Pts',(-160.835394872063,221.464560612651,4.92149382218557));
#87187=CARTESIAN_POINT('Ctrl Pts',(-163.423312804591,223.784209847143,4.76273595695377));
#87188=CARTESIAN_POINT('Ctrl Pts',(-162.878214992983,227.216550181714,4.60397809172198));
#87189=CARTESIAN_POINT('Ctrl Pts',(-159.698974932965,228.620303877157,4.44522022649019));
#87190=CARTESIAN_POINT('Ctrl Pts',(-156.79523300249,226.710755606563,4.28646236125839));
#87191=CARTESIAN_POINT('Ctrl Pts',(-156.82449370205,223.235523872175,4.1277044960266));
#87192=CARTESIAN_POINT('Ctrl Pts',(-159.759977640748,221.375140620465,3.96894663079481));
#87193=CARTESIAN_POINT('Ctrl Pts',(-162.915130032929,222.832228530611,3.81018876556302));
#87194=CARTESIAN_POINT('Ctrl Pts',(-163.402355534161,226.273260803779,3.65143090033122));
#87195=CARTESIAN_POINT('Ctrl Pts',(-160.775745383176,228.54900484047,3.49267303509943));
#87196=CARTESIAN_POINT('Ctrl Pts',(-157.439173090395,227.576699784501,3.33391516986764));
#87197=CARTESIAN_POINT('Ctrl Pts',(-156.446269479642,224.246199191696,3.17515730463585));
#87198=CARTESIAN_POINT('Ctrl Pts',(-158.705739911624,221.605577059435,3.01639943940406));
#87199=CARTESIAN_POINT('Ctrl Pts',(-162.149717104325,222.071530688761,2.85764157417226));
#87200=CARTESIAN_POINT('Ctrl Pts',(-163.62627333181,225.217619275357,2.69888370894047));
#87201=CARTESIAN_POINT('Ctrl Pts',(-161.784064257062,228.164542795226,2.54012584370868));
#87202=CARTESIAN_POINT('Ctrl Pts',(-158.309079834391,228.215276695892,2.38136797847689));
#87203=CARTESIAN_POINT('Ctrl Pts',(-156.381625086582,225.323389859127,2.22261011324509));
#87204=CARTESIAN_POINT('Ctrl Pts',(-157.765707735213,222.135535871982,2.0638522480133));
#87205=CARTESIAN_POINT('Ctrl Pts',(-161.194612879462,221.569240927476,1.90509438278151));
#87206=CARTESIAN_POINT('Ctrl Pts',(-163.530211885137,224.14277326176,1.74633651754971));
#87207=CARTESIAN_POINT('Ctrl Pts',(-162.634953804902,227.500846298696,1.58757865231793));
#87208=CARTESIAN_POINT('Ctrl Pts',(-159.328201268715,228.570130738719,1.42882078708613));
#87209=CARTESIAN_POINT('Ctrl Pts',(-156.636247443033,226.37206105408,1.27006292185434));
#87210=CARTESIAN_POINT('Ctrl Pts',(-157.022865107512,222.918220169874,1.11130505662255));
#87211=CARTESIAN_POINT('Ctrl Pts',(-160.134021050498,221.369750629735,0.952547191390755));
#87212=CARTESIAN_POINT('Ctrl Pts',(-163.122802005527,223.143422645256,0.793789326158964));
#87213=CARTESIAN_POINT('Ctrl Pts',(-163.25301149339,226.616779062293,0.635031460927171));
#87214=CARTESIAN_POINT('Ctrl Pts',(-160.407275482247,228.609330107362,0.476273595695376));
#87215=CARTESIAN_POINT('Ctrl Pts',(-157.186291303474,227.300991486183,0.317515730463588));
#87216=CARTESIAN_POINT('Ctrl Pts',(-156.545696053065,223.882027393836,0.158757865231792));
#87217=CARTESIAN_POINT('Ctrl Pts',(-158.218929051303,222.29471665351,0.0529192884105984));
#87218=CARTESIAN_POINT('Ctrl Pts',(-159.206200717467,222.030777046254,0.));
#87219=CARTESIAN_POINT('Ctrl Pts',(-159.206200717467,222.030777046254,0.));
#87220=CARTESIAN_POINT('Ctrl Pts',(-159.113164836944,222.064809986938,4.63034655208678E-16));
#87221=CARTESIAN_POINT('Ctrl Pts',(-159.022195960155,222.103614880716,2.71860146874827E-18));
#87222=CARTESIAN_POINT('Ctrl Pts',(-158.933501628106,222.146862335309,5.55111512312578E-17));
#87223=CARTESIAN_POINT('Ctrl Pts',(-158.842828980427,222.191074418795,1.09481232003075E-16));
#87224=CARTESIAN_POINT('Ctrl Pts',(-158.754532809116,222.239930072316,3.09433814103877E-15));
#87225=CARTESIAN_POINT('Ctrl Pts',(-158.668863782053,222.29312293841,2.55351295663786E-15));
#87226=CARTESIAN_POINT('Ctrl Pts',(-158.585928546965,222.344618362203,2.02994609300867E-15));
#87227=CARTESIAN_POINT('Ctrl Pts',(-158.50545513685,222.400179468892,-1.45413356794216E-15));
#87228=CARTESIAN_POINT('Ctrl Pts',(-158.427704668138,222.459558987316,-2.4980018054066E-15));
#87229=CARTESIAN_POINT('Ctrl Pts',(-158.359673008016,222.511516065936,-3.41138651318799E-15));
#87230=CARTESIAN_POINT('Ctrl Pts',(-158.293726396571,222.566397333241,3.31443200639852E-15));
#87231=CARTESIAN_POINT('Ctrl Pts',(-158.230065006024,222.624050100838,4.49640324973188E-15));
#87232=CARTESIAN_POINT('Ctrl Pts',(-158.216686222763,222.636166139703,4.74480085697196E-15));
#87233=CARTESIAN_POINT('Ctrl Pts',(-158.203406550876,222.648406529201,-1.97156843780396E-16));
#87234=CARTESIAN_POINT('Ctrl Pts',(-158.19024514275,222.660753435868,0.));
#87235=CARTESIAN_POINT('Ctrl Pts',(-158.117820229753,222.72869629065,1.08491941895841E-15));
#87236=CARTESIAN_POINT('Ctrl Pts',(-158.048861076532,222.799961265629,3.84701060022766E-15));
#87237=CARTESIAN_POINT('Ctrl Pts',(-157.983606900735,222.874256342348,3.85802501057242E-15));
#87238=CARTESIAN_POINT('Ctrl Pts',(-157.91871036732,222.94814422569,3.86897905359346E-15));
#87239=CARTESIAN_POINT('Ctrl Pts',(-157.857477825039,223.025029886816,6.98233960792838E-15));
#87240=CARTESIAN_POINT('Ctrl Pts',(-157.800188199579,223.104652829295,6.9111383282916E-15));
#87241=CARTESIAN_POINT('Ctrl Pts',(-157.744357483621,223.182248132977,6.84175022551745E-15));
#87242=CARTESIAN_POINT('Ctrl Pts',(-157.692271158803,223.262443821962,-5.23084561579274E-16));
#87243=CARTESIAN_POINT('Ctrl Pts',(-157.644234173771,223.345012877019,-4.16333634234434E-16));
#87244=CARTESIAN_POINT('Ctrl Pts',(-157.623520285302,223.380617238873,-3.70301877629731E-16));
#87245=CARTESIAN_POINT('Ctrl Pts',(-157.603559952642,223.416663019726,-2.91706587269718E-15));
#87246=CARTESIAN_POINT('Ctrl Pts',(-157.584380601027,223.453132347144,-3.46944695195361E-15));
#87247=CARTESIAN_POINT('Ctrl Pts',(-157.571170272066,223.478251643241,-3.84991527617551E-15));
#87248=CARTESIAN_POINT('Ctrl Pts',(-157.558330491145,223.503571879617,3.30872527225209E-15));
#87249=CARTESIAN_POINT('Ctrl Pts',(-157.545870750695,223.529087219283,3.52495810318487E-15));
#87250=CARTESIAN_POINT('Ctrl Pts',(-157.539658105459,223.541809615391,3.6327755872119E-15));
#87251=CARTESIAN_POINT('Ctrl Pts',(-157.533540500235,223.554579541051,5.24877045946864E-16));
#87252=CARTESIAN_POINT('Ctrl Pts',(-157.527524300936,223.567384747645,2.4980018054066E-16));
#87253=CARTESIAN_POINT('Ctrl Pts',(-157.487323769582,223.652949750335,-1.58827658575181E-15));
#87254=CARTESIAN_POINT('Ctrl Pts',(-157.451579839888,223.7402249579,-8.46591886096976E-15));
#87255=CARTESIAN_POINT('Ctrl Pts',(-157.420543550398,223.828972297192,-5.57887069874141E-15));
#87256=CARTESIAN_POINT('Ctrl Pts',(-157.390193293269,223.915757947517,-2.75563842743794E-15));
#87257=CARTESIAN_POINT('Ctrl Pts',(-157.364344642025,224.003952043901,3.01207522017872E-16));
#87258=CARTESIAN_POINT('Ctrl Pts',(-157.343281489985,224.093340708165,7.21644966006352E-16));
#87259=CARTESIAN_POINT('Ctrl Pts',(-157.339658573778,224.108715787825,7.93961285378772E-16));
#87260=CARTESIAN_POINT('Ctrl Pts',(-157.336177360488,224.124126216227,3.93408136349463E-15));
#87261=CARTESIAN_POINT('Ctrl Pts',(-157.332839452763,224.139570909969,3.99680288865056E-15));
#87262=CARTESIAN_POINT('Ctrl Pts',(-157.312711861727,224.232702447729,4.37608524451406E-15));
#87263=CARTESIAN_POINT('Ctrl Pts',(-157.29779090409,224.327080946637,-3.10799959844018E-16));
#87264=CARTESIAN_POINT('Ctrl Pts',(-157.28799827831,224.422298268421,-1.4432899320127E-15));
#87265=CARTESIAN_POINT('Ctrl Pts',(-157.284735582254,224.454022668725,-1.82061166869276E-15));
#87266=CARTESIAN_POINT('Ctrl Pts',(-157.282042584831,224.48584006534,8.80200877206319E-15));
#87267=CARTESIAN_POINT('Ctrl Pts',(-157.279917589015,224.517734904248,9.15933995315754E-15));
#87268=CARTESIAN_POINT('Ctrl Pts',(-157.278692787876,224.536118392216,9.36529783516321E-15));
#87269=CARTESIAN_POINT('Ctrl Pts',(-157.277656694263,224.554527602168,6.51887382620648E-15));
#87270=CARTESIAN_POINT('Ctrl Pts',(-157.276809068708,224.572959507432,6.77236045021345E-15));
#87271=CARTESIAN_POINT('Ctrl Pts',(-157.276234543042,224.585452762959,6.94417519866532E-15));
#87272=CARTESIAN_POINT('Ctrl Pts',(-157.275746722798,224.597954820887,4.16905420329119E-15));
#87273=CARTESIAN_POINT('Ctrl Pts',(-157.275345652497,224.610455351992,4.16333634234434E-15));
#87274=CARTESIAN_POINT('Ctrl Pts',(-157.272356009785,224.703636327093,4.12071448459771E-15));
#87275=CARTESIAN_POINT('Ctrl Pts',(-157.274175040167,224.796878521229,3.65420848031107E-15));
#87276=CARTESIAN_POINT('Ctrl Pts',(-157.28066394211,224.889807515738,4.37150315946155E-15));
#87277=CARTESIAN_POINT('Ctrl Pts',(-157.287165695516,224.982920558858,5.09021846185362E-15));
#87278=CARTESIAN_POINT('Ctrl Pts',(-157.29835621947,225.075720140589,3.27636343276335E-15));
#87279=CARTESIAN_POINT('Ctrl Pts',(-157.314146920592,225.16781758215,2.5951463200613E-15));
#87280=CARTESIAN_POINT('Ctrl Pts',(-157.329714993719,225.258616571636,1.92353346735484E-15));
#87281=CARTESIAN_POINT('Ctrl Pts',(-157.349754912718,225.34873392575,5.78387140447215E-15));
#87282=CARTESIAN_POINT('Ctrl Pts',(-157.374224827573,225.437772014373,5.70377078901174E-15));
#87283=CARTESIAN_POINT('Ctrl Pts',(-157.383741664711,225.472400699991,5.67261806467303E-15));
#87284=CARTESIAN_POINT('Ctrl Pts',(-157.393929005722,225.506865798334,1.39646007254645E-15));
#87285=CARTESIAN_POINT('Ctrl Pts',(-157.404785957261,225.541142454069,2.4980018054066E-16));
#87286=CARTESIAN_POINT('Ctrl Pts',(-157.410770219746,225.560035465086,-3.82229330717133E-16));
#87287=CARTESIAN_POINT('Ctrl Pts',(-157.416957933028,225.578871208808,4.76239706612756E-15));
#87288=CARTESIAN_POINT('Ctrl Pts',(-157.423349053532,225.597645396291,4.94049245958195E-15));
#87289=CARTESIAN_POINT('Ctrl Pts',(-157.428584730572,225.613025419601,5.08639018779692E-15));
#87290=CARTESIAN_POINT('Ctrl Pts',(-157.433957191302,225.628364651371,1.41988730813603E-15));
#87291=CARTESIAN_POINT('Ctrl Pts',(-157.439460918369,225.64364605392,1.66533453693773E-15));
#87292=CARTESIAN_POINT('Ctrl Pts',(-157.471855948626,225.733592646819,3.1100410614556E-15));
#87293=CARTESIAN_POINT('Ctrl Pts',(-157.508835933315,225.821662943619,3.31193101344564E-15));
#87294=CARTESIAN_POINT('Ctrl Pts',(-157.550328254259,225.907414095892,3.49026363366534E-15));
#87295=CARTESIAN_POINT('Ctrl Pts',(-157.581447494966,225.971727460097,3.62401309883011E-15));
#87296=CARTESIAN_POINT('Ctrl Pts',(-157.615106070035,226.034735769921,1.73102608059913E-15));
#87297=CARTESIAN_POINT('Ctrl Pts',(-157.651290671058,226.096235103398,7.49400541621981E-16));
#87298=CARTESIAN_POINT('Ctrl Pts',(-157.665717951457,226.120755703417,3.58013418418384E-16));
#87299=CARTESIAN_POINT('Ctrl Pts',(-157.680546954031,226.145036228956,4.50893100540133E-15));
#87300=CARTESIAN_POINT('Ctrl Pts',(-157.695777423898,226.169062946708,4.2257863874795E-15));
#87301=CARTESIAN_POINT('Ctrl Pts',(-157.706206438561,226.185515163475,4.03190403206177E-15));
#87302=CARTESIAN_POINT('Ctrl Pts',(-157.716819306202,226.201841333482,9.48857707092389E-15));
#87303=CARTESIAN_POINT('Ctrl Pts',(-157.727611563923,226.218031534773,9.45771239102555E-15));
#87304=CARTESIAN_POINT('Ctrl Pts',(-157.775201280265,226.28942411146,9.32161099321723E-15));
#87305=CARTESIAN_POINT('Ctrl Pts',(-157.826300157625,226.358212936193,2.36509029748788E-15));
#87306=CARTESIAN_POINT('Ctrl Pts',(-157.880874323238,226.424045534683,1.60982338570648E-15));
#87307=CARTESIAN_POINT('Ctrl Pts',(-157.931843006989,226.48552885477,9.04453730645144E-16));
#87308=CARTESIAN_POINT('Ctrl Pts',(-157.985843474429,226.544433784549,2.05927059619376E-15));
#87309=CARTESIAN_POINT('Ctrl Pts',(-158.042870847355,226.600438912347,4.47124975933022E-16));
#87310=CARTESIAN_POINT('Ctrl Pts',(-158.056034879742,226.613366972652,7.5849346180632E-17));
#87311=CARTESIAN_POINT('Ctrl Pts',(-158.069360289123,226.626140355812,9.46940075139361E-16));
#87312=CARTESIAN_POINT('Ctrl Pts',(-158.082843691308,226.638757663408,7.49400541621981E-16));
#87313=CARTESIAN_POINT('Ctrl Pts',(-162.519491434632,224.998011610487,18.387416697508));
#87314=CARTESIAN_POINT('Ctrl Pts',(-162.520629350597,224.866458071072,18.3957515808994));
#87315=CARTESIAN_POINT('Ctrl Pts',(-162.511214998764,224.735067810581,18.4040864642907));
#87316=CARTESIAN_POINT('Ctrl Pts',(-162.490679990779,224.605439310924,18.4124213476821));
#87317=CARTESIAN_POINT('Ctrl Pts',(-162.360300481071,223.782410644836,18.4653406360927));
#87318=CARTESIAN_POINT('Ctrl Pts',(-161.781630665363,223.03040119671,18.5182599245033));
#87319=CARTESIAN_POINT('Ctrl Pts',(-161.01946796215,222.693521970312,18.5711792129139));
#87320=CARTESIAN_POINT('Ctrl Pts',(-160.257305258936,222.356642743915,18.6240985013245));
#87321=CARTESIAN_POINT('Ctrl Pts',(-159.311649668218,222.434893739245,18.6770177897351));
#87322=CARTESIAN_POINT('Ctrl Pts',(-158.61523706607,222.892484949723,18.7299370781457));
#87323=CARTESIAN_POINT('Ctrl Pts',(-157.918824463922,223.350076160201,18.7828563665563));
#87324=CARTESIAN_POINT('Ctrl Pts',(-157.471654850343,224.187007585826,18.8357756549669));
#87325=CARTESIAN_POINT('Ctrl Pts',(-157.478344947014,225.020262805069,18.8886949433775));
#87326=CARTESIAN_POINT('Ctrl Pts',(-157.485035043684,225.853518024313,18.9416142317881));
#87327=CARTESIAN_POINT('Ctrl Pts',(-157.945584850604,226.683097037174,18.9945335201987));
#87328=CARTESIAN_POINT('Ctrl Pts',(-158.649263561541,227.129460482924,19.0474528086093));
#87329=CARTESIAN_POINT('Ctrl Pts',(-159.352942272479,227.575823928674,19.1003720970199));
#87330=CARTESIAN_POINT('Ctrl Pts',(-160.299749887435,227.638971807313,19.1532913854305));
#87331=CARTESIAN_POINT('Ctrl Pts',(-161.056392462878,227.289849982455,19.2062106738411));
#87332=CARTESIAN_POINT('Ctrl Pts',(-161.813035038321,226.940728157596,19.2591299622517));
#87333=CARTESIAN_POINT('Ctrl Pts',(-162.379512574251,226.179336629241,19.3120492506623));
#87334=CARTESIAN_POINT('Ctrl Pts',(-162.496677300197,225.354415193034,19.3649685390729));
#87335=CARTESIAN_POINT('Ctrl Pts',(-162.513244242107,225.237772360444,19.3724512585512));
#87336=CARTESIAN_POINT('Ctrl Pts',(-162.520827804709,225.119859336471,19.3799339780296));
#87337=CARTESIAN_POINT('Ctrl Pts',(-162.519857258493,225.0018235551,19.387416697508));
#87338=CARTESIAN_POINT('Ctrl Pts',(-160.793799282533,222.030777046254,20.));
#87339=CARTESIAN_POINT('Ctrl Pts',(-161.781070948697,222.29471665351,19.9470807115894));
#87340=CARTESIAN_POINT('Ctrl Pts',(-163.454303903543,223.882027706698,19.8412421347682));
#87341=CARTESIAN_POINT('Ctrl Pts',(-162.813708733919,227.30099142385,19.6824842695364));
#87342=CARTESIAN_POINT('Ctrl Pts',(-159.59272451442,228.609330199079,19.5237264043046));
#87343=CARTESIAN_POINT('Ctrl Pts',(-156.746988470599,226.616779048904,19.3649685390728));
#87344=CARTESIAN_POINT('Ctrl Pts',(-156.877197967362,223.143422642792,19.2062106738411));
#87345=CARTESIAN_POINT('Ctrl Pts',(-159.865978945628,221.369750585662,19.0474528086092));
#87346=CARTESIAN_POINT('Ctrl Pts',(-162.977134923396,222.918220153796,18.8886949433775));
#87347=CARTESIAN_POINT('Ctrl Pts',(-163.363752589082,226.372061065279,18.7299370781457));
#87348=CARTESIAN_POINT('Ctrl Pts',(-160.671798738453,228.570130775029,18.5711792129139));
#87349=CARTESIAN_POINT('Ctrl Pts',(-157.365046168866,227.50084632268,18.4124213476821));
#87350=CARTESIAN_POINT('Ctrl Pts',(-156.469788080311,224.142773253644,18.2536634824503));
#87351=CARTESIAN_POINT('Ctrl Pts',(-158.805387108694,221.569240893567,18.0949056172185));
#87352=CARTESIAN_POINT('Ctrl Pts',(-162.234292286814,222.135535843889,17.9361477519867));
#87353=CARTESIAN_POINT('Ctrl Pts',(-163.618374948983,225.323389862265,17.7773898867549));
#87354=CARTESIAN_POINT('Ctrl Pts',(-161.690920182255,228.21527672754,17.6186320215231));
#87355=CARTESIAN_POINT('Ctrl Pts',(-158.215935725382,228.164542826343,17.4598741562913));
#87356=CARTESIAN_POINT('Ctrl Pts',(-156.373726632524,225.217619277503,17.3011162910595));
#87357=CARTESIAN_POINT('Ctrl Pts',(-157.850282874527,222.071530659953,17.1423584258277));
#87358=CARTESIAN_POINT('Ctrl Pts',(-161.294260101108,221.605577026048,16.9836005605959));
#87359=CARTESIAN_POINT('Ctrl Pts',(-163.553730555313,224.24619918428,16.8248426953642));
#87360=CARTESIAN_POINT('Ctrl Pts',(-162.560826934795,227.576699809846,16.6660848301323));
#87361=CARTESIAN_POINT('Ctrl Pts',(-159.224254609194,228.54900487538,16.5073269649006));
#87362=CARTESIAN_POINT('Ctrl Pts',(-156.597644432372,226.273260816304,16.3485690996688));
#87363=CARTESIAN_POINT('Ctrl Pts',(-157.084869938397,222.832228509288,16.189811234437));
#87364=CARTESIAN_POINT('Ctrl Pts',(-160.240022361613,221.37514058481,16.0310533692052));
#87365=CARTESIAN_POINT('Ctrl Pts',(-163.175506329186,223.235523854818,15.8722955039734));
#87366=CARTESIAN_POINT('Ctrl Pts',(-163.204767029033,226.710755623391,15.7135376387416));
#87367=CARTESIAN_POINT('Ctrl Pts',(-160.301025069996,228.620303912768,15.5547797735098));
#87368=CARTESIAN_POINT('Ctrl Pts',(-157.121784978706,227.216550203517,15.396021908278));
#87369=CARTESIAN_POINT('Ctrl Pts',(-156.576687161735,223.784209835184,15.2372640430462));
#87370=CARTESIAN_POINT('Ctrl Pts',(-159.164605119719,221.464560577875,15.0785061778144));
#87371=CARTESIAN_POINT('Ctrl Pts',(-162.517076439288,222.38054534067,14.9197483125826));
#87372=CARTESIAN_POINT('Ctrl Pts',(-163.565919500601,225.693854904675,14.7609904473509));
#87373=CARTESIAN_POINT('Ctrl Pts',(-161.35123317519,228.372148487207,14.602232582119));
#87374=CARTESIAN_POINT('Ctrl Pts',(-157.899898300982,227.964251906854,14.4434747168873));
#87375=CARTESIAN_POINT('Ctrl Pts',(-156.37057641913,224.843472097915,14.2847168516555));
#87376=CARTESIAN_POINT('Ctrl Pts',(-158.162902855767,221.865946618808,14.1259589864237));
#87377=CARTESIAN_POINT('Ctrl Pts',(-161.636540526564,221.756706670925,13.9672011211919));
#87378=CARTESIAN_POINT('Ctrl Pts',(-163.612416371805,224.615728650272,13.8084432559601));
#87379=CARTESIAN_POINT('Ctrl Pts',(-162.282208895625,227.826435753778,13.6496853907283));
#87380=CARTESIAN_POINT('Ctrl Pts',(-158.863323927915,228.450388966574,13.4909275254965));
#87381=CARTESIAN_POINT('Ctrl Pts',(-156.484724856678,225.916546332844,13.3321696602647));
#87382=CARTESIAN_POINT('Ctrl Pts',(-157.323305458375,222.543880531338,13.1734117950329));
#87383=CARTESIAN_POINT('Ctrl Pts',(-160.611596799308,221.419055170966,13.0146539298011));
#87384=CARTESIAN_POINT('Ctrl Pts',(-163.340154773566,223.57151037731,12.8558960645693));
#87385=CARTESIAN_POINT('Ctrl Pts',(-163.011803230403,227.031319230165,12.6971381993375));
#87386=CARTESIAN_POINT('Ctrl Pts',(-159.927049489213,228.632064803453,12.5383803341058));
#87387=CARTESIAN_POINT('Ctrl Pts',(-156.909060052626,226.908744811449,12.379622468874));
#87388=CARTESIAN_POINT('Ctrl Pts',(-156.719898734327,223.438541643066,12.2208646036422));
#87389=CARTESIAN_POINT('Ctrl Pts',(-159.532685965386,221.397385101546,12.0621067384104));
#87390=CARTESIAN_POINT('Ctrl Pts',(-162.773158982547,222.653341573422,11.9033488731786));
#87391=CARTESIAN_POINT('Ctrl Pts',(-163.475637007933,226.056959745022,11.7445910079468));
#87392=CARTESIAN_POINT('Ctrl Pts',(-160.997212180335,228.493248399541,11.585833142715));
#87393=CARTESIAN_POINT('Ctrl Pts',(-157.606138804509,227.732516256169,11.4270752774832));
#87394=CARTESIAN_POINT('Ctrl Pts',(-156.40592710066,224.470985342605,11.2683174122514));
#87395=CARTESIAN_POINT('Ctrl Pts',(-158.495010772954,221.693608622685,11.1095595470196));
#87396=CARTESIAN_POINT('Ctrl Pts',(-161.961460526658,221.942241161264,10.9508016817878));
#87397=CARTESIAN_POINT('Ctrl Pts',(-163.632781683497,224.98933446881,10.792043816556));
#87398=CARTESIAN_POINT('Ctrl Pts',(-161.979381186455,228.046188870082,10.6332859513243));
#87399=CARTESIAN_POINT('Ctrl Pts',(-158.514451105407,228.315171337243,10.4745280860925));
#87400=CARTESIAN_POINT('Ctrl Pts',(-156.409095314272,225.550109126926,10.3157702208607));
#87401=CARTESIAN_POINT('Ctrl Pts',(-157.590135350307,222.281587065278,10.1570123556289));
#87402=CARTESIAN_POINT('Ctrl Pts',(-160.976683418975,221.500956414589,9.99825449039708));
#87403=CARTESIAN_POINT('Ctrl Pts',(-163.469370861004,223.922650315672,9.83949662516528));
#87404=CARTESIAN_POINT('Ctrl Pts',(-162.786890227472,227.330334605486,9.68073875993349));
#87405=CARTESIAN_POINT('Ctrl Pts',(-159.55384776735,228.605296755998,9.52198089470171));
#87406=CARTESIAN_POINT('Ctrl Pts',(-156.729123813004,226.580691457195,9.36322302946991));
#87407=CARTESIAN_POINT('Ctrl Pts',(-156.897905616373,223.109437398927,9.20446516423812));
#87408=CARTESIAN_POINT('Ctrl Pts',(-159.90572407765,221.368426158816,9.04570729900633));
#87409=CARTESIAN_POINT('Ctrl Pts',(-162.999823859355,222.951031155348,8.88694943377453));
#87410=CARTESIAN_POINT('Ctrl Pts',(-163.348484962943,226.408852357933,8.72819156854274));
#87411=CARTESIAN_POINT('Ctrl Pts',(-160.632612760122,228.577291937938,8.56943370331094));
#87412=CARTESIAN_POINT('Ctrl Pts',(-157.337773384114,227.471794077016,8.41067583807916));
#87413=CARTESIAN_POINT('Ctrl Pts',(-156.479403702276,224.10411037401,8.25191797284736));
#87414=CARTESIAN_POINT('Ctrl Pts',(-158.843083613671,221.55634482148,8.09316010761557));
#87415=CARTESIAN_POINT('Ctrl Pts',(-162.26557335634,222.160212352913,7.93440224238377));
#87416=CARTESIAN_POINT('Ctrl Pts',(-163.614610452378,225.363053427288,7.77564437715199));
#87417=CARTESIAN_POINT('Ctrl Pts',(-161.655556204541,228.233628019286,7.61688651192019));
#87418=CARTESIAN_POINT('Ctrl Pts',(-158.181336983412,228.144786375193,7.45812864668841));
#87419=CARTESIAN_POINT('Ctrl Pts',(-156.371558083546,225.177836364189,7.2993707814566));
#87420=CARTESIAN_POINT('Ctrl Pts',(-157.882529082935,222.048130519673,7.14061291622482));
#87421=CARTESIAN_POINT('Ctrl Pts',(-161.331409382354,221.619975507472,6.98185505099302));
#87422=CARTESIAN_POINT('Ctrl Pts',(-163.561783867399,224.285218777917,6.82309718576123));
#87423=CARTESIAN_POINT('Ctrl Pts',(-162.532413897065,227.604629794704,6.66433932052944));
#87424=CARTESIAN_POINT('Ctrl Pts',(-159.185378827721,228.540283725802,6.50558145529764));
#87425=CARTESIAN_POINT('Ctrl Pts',(-156.583885023213,226.235870130265,6.34682359006585));
#87426=CARTESIAN_POINT('Ctrl Pts',(-157.108819511125,222.800388240108,6.18806572483406));
#87427=CARTESIAN_POINT('Ctrl Pts',(-160.279762268762,221.377990946107,6.02930785960227));
#87428=CARTESIAN_POINT('Ctrl Pts',(-163.19466660903,223.270456195797,5.87054999437048));
#87429=CARTESIAN_POINT('Ctrl Pts',(-163.18581219434,226.745799867081,5.71179212913868));
#87430=CARTESIAN_POINT('Ctrl Pts',(-160.26130258467,228.623387568664,5.5530342639069));
#87431=CARTESIAN_POINT('Ctrl Pts',(-157.097648859785,227.184851109893,5.39427639867509));
#87432=CARTESIAN_POINT('Ctrl Pts',(-156.590226784293,223.746739001265,5.23551853344331));
#87433=CARTESIAN_POINT('Ctrl Pts',(-159.203429021729,221.455611309395,5.07676066821151));
#87434=CARTESIAN_POINT('Ctrl Pts',(-162.545652987155,222.408308007789,4.91800280297972));
#87435=CARTESIAN_POINT('Ctrl Pts',(-163.558095438842,225.732921115537,4.75924493774792));
#87436=CARTESIAN_POINT('Ctrl Pts',(-161.314169084819,228.386764847169,4.60048707251614));
#87437=CARTESIAN_POINT('Ctrl Pts',(-157.867515236049,227.941041523849,4.44172920728434));
#87438=CARTESIAN_POINT('Ctrl Pts',(-156.372511359387,224.803677113565,4.28297134205255));
#87439=CARTESIAN_POINT('Ctrl Pts',(-158.197384943971,221.845987401207,4.12421347682076));
#87440=CARTESIAN_POINT('Ctrl Pts',(-161.672011756938,221.774849895275,3.96545561158897));
#87441=CARTESIAN_POINT('Ctrl Pts',(-163.616413475723,224.655369638279,3.80669774635717));
#87442=CARTESIAN_POINT('Ctrl Pts',(-162.251073723701,227.851295074949,3.64793988112539));
#87443=CARTESIAN_POINT('Ctrl Pts',(-158.825551388348,228.437715370794,3.48918201589359));
#87444=CARTESIAN_POINT('Ctrl Pts',(-156.474884376031,225.877938695212,3.3304241506618));
#87445=CARTESIAN_POINT('Ctrl Pts',(-157.350403044487,222.514672558763,3.17166628543001));
#87446=CARTESIAN_POINT('Ctrl Pts',(-160.650832741734,221.425978001981,3.01290842019821));
#87447=CARTESIAN_POINT('Ctrl Pts',(-163.355620340796,223.608228230643,2.85415055496642));
#87448=CARTESIAN_POINT('Ctrl Pts',(-162.989344332895,227.064227941581,2.69539268973463));
#87449=CARTESIAN_POINT('Ctrl Pts',(-159.887220515355,228.631046293149,2.53663482450283));
#87450=CARTESIAN_POINT('Ctrl Pts',(-156.88831246471,226.874731278963,2.37787695927104));
#87451=CARTESIAN_POINT('Ctrl Pts',(-156.73722075101,223.402662149674,2.21911909403925));
#87452=CARTESIAN_POINT('Ctrl Pts',(-159.572224421631,221.392476811998,2.06036122880746));
#87453=CARTESIAN_POINT('Ctrl Pts',(-162.798728401055,222.68389602747,1.90160336357567));
#87454=CARTESIAN_POINT('Ctrl Pts',(-163.463836016567,226.095014600311,1.74284549834387));
#87455=CARTESIAN_POINT('Ctrl Pts',(-160.958841546672,228.50397358649,1.58408763311208));
#87456=CARTESIAN_POINT('Ctrl Pts',(-157.576314291936,227.706100789163,1.42532976788028));
#87457=CARTESIAN_POINT('Ctrl Pts',(-156.411946257884,224.431594893095,1.2665719026485));
#87458=CARTESIAN_POINT('Ctrl Pts',(-158.531360393914,221.677313586384,1.1078140374167));
#87459=CARTESIAN_POINT('Ctrl Pts',(-161.994882722329,221.963912720035,0.949056172184911));
#87460=CARTESIAN_POINT('Ctrl Pts',(-163.632669200339,225.029226034151,0.79029830695312));
#87461=CARTESIAN_POINT('Ctrl Pts',(-161.945876935419,228.067610699799,0.631540441721325));
#87462=CARTESIAN_POINT('Ctrl Pts',(-158.478135238796,228.298893703494,0.472782576489533));
#87463=CARTESIAN_POINT('Ctrl Pts',(-156.403376103572,225.51024998876,0.314024711257742));
#87464=CARTESIAN_POINT('Ctrl Pts',(-157.6198890437,222.256241693801,0.155266846025946));
#87465=CARTESIAN_POINT('Ctrl Pts',(-161.015405798375,221.509947072523,-0.00349101920584216));
#87466=CARTESIAN_POINT('Ctrl Pts',(-163.479964483845,223.964662036918,-0.162248884437638));
#87467=CARTESIAN_POINT('Ctrl Pts',(-163.000168811616,226.220556762668,-0.268087461258832));
#87468=CARTESIAN_POINT('Ctrl Pts',(-162.336062657696,226.997301556931,-0.32100674966943));
#87469=CARTESIAN_POINT('Ctrl Pts',(-160.745932854347,222.209822430158,20.1070022498898));
#87470=CARTESIAN_POINT('Ctrl Pts',(-161.673671626808,222.457846368889,20.0540829614792));
#87471=CARTESIAN_POINT('Ctrl Pts',(-163.246007935822,223.949441902791,19.948244384658));
#87472=CARTESIAN_POINT('Ctrl Pts',(-162.644040922406,227.162240680218,19.7894865194262));
#87473=CARTESIAN_POINT('Ctrl Pts',(-159.617283396257,228.391686081006,19.6307286541944));
#87474=CARTESIAN_POINT('Ctrl Pts',(-156.94314642411,226.519286597172,19.4719707889626));
#87475=CARTESIAN_POINT('Ctrl Pts',(-157.065504233849,223.255375032642,19.3132129237309));
#87476=CARTESIAN_POINT('Ctrl Pts',(-159.874060471167,221.588656141149,19.154455058499));
#87477=CARTESIAN_POINT('Ctrl Pts',(-162.797612444419,223.043752347765,18.9956971932673));
#87478=CARTESIAN_POINT('Ctrl Pts',(-163.160916903433,226.289325210142,18.8369393280355));
#87479=CARTESIAN_POINT('Ctrl Pts',(-160.631288994016,228.354850398594,18.6781814628037));
#87480=CARTESIAN_POINT('Ctrl Pts',(-157.523934985103,227.350044245199,18.5194235975719));
#87481=CARTESIAN_POINT('Ctrl Pts',(-156.6826613331,224.194464384383,18.3606657323401));
#87482=CARTESIAN_POINT('Ctrl Pts',(-158.877422764847,221.776117100191,18.2019078671083));
#87483=CARTESIAN_POINT('Ctrl Pts',(-162.099563528995,222.308264228553,18.0431500018765));
#87484=CARTESIAN_POINT('Ctrl Pts',(-163.400185428714,225.30388931854,17.8843921366447));
#87485=CARTESIAN_POINT('Ctrl Pts',(-161.588956989225,228.021394198337,17.7256342714129));
#87486=CARTESIAN_POINT('Ctrl Pts',(-158.323515546074,227.973719572567,17.5668764061811));
#87487=CARTESIAN_POINT('Ctrl Pts',(-156.592392430726,225.204496744203,17.4081185409493));
#87488=CARTESIAN_POINT('Ctrl Pts',(-157.979911714803,222.248118583934,17.2493606757176));
#87489=CARTESIAN_POINT('Ctrl Pts',(-161.216215676596,221.810262148711,17.0906028104857));
#87490=CARTESIAN_POINT('Ctrl Pts',(-163.339439118975,224.291653688216,16.931844945254));
#87491=CARTESIAN_POINT('Ctrl Pts',(-162.406408001359,227.421323735417,16.7730870800222));
#87492=CARTESIAN_POINT('Ctrl Pts',(-159.27103238017,228.334998399515,16.6143292147904));
#87493=CARTESIAN_POINT('Ctrl Pts',(-156.802807893747,226.196482657433,16.4555713495586));
#87494=CARTESIAN_POINT('Ctrl Pts',(-157.260653498318,222.962946035326,16.2968134843268));
#87495=CARTESIAN_POINT('Ctrl Pts',(-160.225548912986,221.593721121098,16.138055619095));
#87496=CARTESIAN_POINT('Ctrl Pts',(-162.98402197161,223.341922503126,15.9792977538632));
#87497=CARTESIAN_POINT('Ctrl Pts',(-163.011518239039,226.607596344978,15.8205398886314));
#87498=CARTESIAN_POINT('Ctrl Pts',(-160.282873132583,228.401998075178,15.6617820233996));
#87499=CARTESIAN_POINT('Ctrl Pts',(-157.295342546282,227.082891300729,15.5030241581678));
#87500=CARTESIAN_POINT('Ctrl Pts',(-156.78311435528,223.857522489773,15.344266292936));
#87501=CARTESIAN_POINT('Ctrl Pts',(-159.214979779818,221.677749051244,15.1855084277043));
#87502=CARTESIAN_POINT('Ctrl Pts',(-162.365295678999,222.538499550375,15.0267505624724));
#87503=CARTESIAN_POINT('Ctrl Pts',(-163.350893065773,225.652015164205,14.8679926972407));
#87504=CARTESIAN_POINT('Ctrl Pts',(-161.269753250522,228.168806525395,14.7092348320089));
#87505=CARTESIAN_POINT('Ctrl Pts',(-158.026535310325,227.785506279153,14.5504769667771));
#87506=CARTESIAN_POINT('Ctrl Pts',(-156.589432176514,224.852910795768,14.3917191015453));
#87507=CARTESIAN_POINT('Ctrl Pts',(-158.27368058064,222.054931346312,14.2329612363135));
#87508=CARTESIAN_POINT('Ctrl Pts',(-161.537856449478,221.952278612899,14.0742033710817));
#87509=CARTESIAN_POINT('Ctrl Pts',(-163.394586156228,224.638900373112,13.9154455058499));
#87510=CARTESIAN_POINT('Ctrl Pts',(-162.144590746287,227.656000497653,13.7566876406181));
#87511=CARTESIAN_POINT('Ctrl Pts',(-158.931865969678,228.242329071187,13.5979297753863));
#87512=CARTESIAN_POINT('Ctrl Pts',(-156.696697415616,225.861278206272,13.4391719101545));
#87513=CARTESIAN_POINT('Ctrl Pts',(-157.484711256883,222.691985560846,13.2804140449227));
#87514=CARTESIAN_POINT('Ctrl Pts',(-160.574717256939,221.634987639373,13.1216561796909));
#87515=CARTESIAN_POINT('Ctrl Pts',(-163.138742046045,223.65764889802,12.9628983144591));
#87516=CARTESIAN_POINT('Ctrl Pts',(-162.830190238038,226.908829832413,12.8041404492274));
#87517=CARTESIAN_POINT('Ctrl Pts',(-159.931448435473,228.413049779244,12.6453825839956));
#87518=CARTESIAN_POINT('Ctrl Pts',(-157.095445022068,226.793646702326,12.4866247187638));
#87519=CARTESIAN_POINT('Ctrl Pts',(-156.917690210247,223.532698233973,12.327866853532));
#87520=CARTESIAN_POINT('Ctrl Pts',(-159.560865196799,221.614624284187,12.1691089883002));
#87521=CARTESIAN_POINT('Ctrl Pts',(-162.605936337972,222.794846056387,12.0103511230684));
#87522=CARTESIAN_POINT('Ctrl Pts',(-163.266054645109,225.993224631066,11.8515932578366));
#87523=CARTESIAN_POINT('Ctrl Pts',(-160.937079869477,228.282604062451,11.6928353926048));
#87524=CARTESIAN_POINT('Ctrl Pts',(-157.750489634149,227.567744384966,11.534077527373));
#87525=CARTESIAN_POINT('Ctrl Pts',(-156.622651197188,224.502885147334,11.3753196621412));
#87526=CARTESIAN_POINT('Ctrl Pts',(-158.58576225175,221.892985403314,11.2165617969094));
#87527=CARTESIAN_POINT('Ctrl Pts',(-161.843183637897,222.126625296,11.0578039316776));
#87528=CARTESIAN_POINT('Ctrl Pts',(-163.413723431122,224.989977604794,10.8990460664458));
#87529=CARTESIAN_POINT('Ctrl Pts',(-161.860023674426,227.862502409287,10.7402882012141));
#87530=CARTESIAN_POINT('Ctrl Pts',(-158.604030324039,228.115265121365,10.5815303359823));
#87531=CARTESIAN_POINT('Ctrl Pts',(-156.625628366196,225.516937316875,10.4227724707505));
#87532=CARTESIAN_POINT('Ctrl Pts',(-157.735451194917,222.445508500309,10.2640146055187));
#87533=CARTESIAN_POINT('Ctrl Pts',(-160.917789000998,221.711950203807,10.1052567402869));
#87534=CARTESIAN_POINT('Ctrl Pts',(-163.260166349457,223.987614951482,9.9464988750551));
#87535=CARTESIAN_POINT('Ctrl Pts',(-162.618839583096,227.189814455749,9.78774100982331));
#87536=CARTESIAN_POINT('Ctrl Pts',(-159.580750933268,228.387895856227,9.62898314459151));
#87537=CARTESIAN_POINT('Ctrl Pts',(-156.926359012827,226.485375102312,9.47022527935972));
#87538=CARTESIAN_POINT('Ctrl Pts',(-157.084963202979,223.223439113172,9.31146741412793));
#87539=CARTESIAN_POINT('Ctrl Pts',(-159.911408955133,221.587411577795,9.15270954889613));
#87540=CARTESIAN_POINT('Ctrl Pts',(-162.818933228066,223.074584832224,8.99395168366434));
#87541=CARTESIAN_POINT('Ctrl Pts',(-163.146569921525,226.323897972486,8.83519381843255));
#87542=CARTESIAN_POINT('Ctrl Pts',(-160.59446594654,228.36157974039,8.67643595320076));
#87543=CARTESIAN_POINT('Ctrl Pts',(-157.498306760659,227.32274386208,8.51767808796897));
#87544=CARTESIAN_POINT('Ctrl Pts',(-156.691697129046,224.158132892534,8.35892022273717));
#87545=CARTESIAN_POINT('Ctrl Pts',(-158.912846154834,221.763998666635,8.20016235750538));
#87546=CARTESIAN_POINT('Ctrl Pts',(-162.128958336967,222.331452733779,8.04140449227358));
#87547=CARTESIAN_POINT('Ctrl Pts',(-163.396647932827,225.34116115403,7.8826466270418));
#87548=CARTESIAN_POINT('Ctrl Pts',(-161.555725474133,228.038638899528,7.72388876181));
#87549=CARTESIAN_POINT('Ctrl Pts',(-158.291003122691,227.95515444367,7.56513089657821));
#87550=CARTESIAN_POINT('Ctrl Pts',(-156.590354646156,225.167112757173,7.40637303134641));
#87551=CARTESIAN_POINT('Ctrl Pts',(-158.010213463379,222.226129481883,7.24761516611463));
#87552=CARTESIAN_POINT('Ctrl Pts',(-161.251124840671,221.823792395694,7.08885730088283));
#87553=CARTESIAN_POINT('Ctrl Pts',(-163.34700681298,224.328320384064,6.93009943565104));
#87554=CARTESIAN_POINT('Ctrl Pts',(-162.379708281668,227.447569530526,6.77134157041925));
#87555=CARTESIAN_POINT('Ctrl Pts',(-159.234500824553,228.326803138899,6.61258370518746));
#87556=CARTESIAN_POINT('Ctrl Pts',(-156.789878182705,226.161346645375,6.45382583995566));
#87557=CARTESIAN_POINT('Ctrl Pts',(-157.28315890181,222.933025747673,6.29506797472387));
#87558=CARTESIAN_POINT('Ctrl Pts',(-160.262892487142,221.596399604419,6.13631010949208));
#87559=CARTESIAN_POINT('Ctrl Pts',(-163.002026878579,223.374748409357,5.97755224426028));
#87560=CARTESIAN_POINT('Ctrl Pts',(-162.993706388793,226.640527406141,5.8187943790285));
#87561=CARTESIAN_POINT('Ctrl Pts',(-160.245545929708,228.404895785336,5.6600365137967));
#87562=CARTESIAN_POINT('Ctrl Pts',(-157.27266184541,227.053103675686,5.50127864856491));
#87563=CARTESIAN_POINT('Ctrl Pts',(-156.795837532943,223.822311162785,5.34252078333311));
#87564=CARTESIAN_POINT('Ctrl Pts',(-159.251462584326,221.669339427391,5.18376291810132));
#87565=CARTESIAN_POINT('Ctrl Pts',(-162.392149049098,222.564588117074,5.02500505286953));
#87566=CARTESIAN_POINT('Ctrl Pts',(-163.343540798205,225.68872566624,4.86624718763774));
#87567=CARTESIAN_POINT('Ctrl Pts',(-161.234924140276,228.182541512748,4.70748932240595));
#87568=CARTESIAN_POINT('Ctrl Pts',(-157.99610495773,227.763695491936,4.54873145717415));
#87569=CARTESIAN_POINT('Ctrl Pts',(-156.591250439066,224.815515465591,4.38997359194236));
#87570=CARTESIAN_POINT('Ctrl Pts',(-158.306083384528,222.036175677865,4.23121572671057));
#87571=CARTESIAN_POINT('Ctrl Pts',(-161.571188749849,221.969327793245,4.07245786147877));
#87572=CARTESIAN_POINT('Ctrl Pts',(-163.398342233112,224.67615099299,3.91369999624699));
#87573=CARTESIAN_POINT('Ctrl Pts',(-162.115333038231,227.679360791378,3.75494213101519));
#87574=CARTESIAN_POINT('Ctrl Pts',(-158.896371130019,228.230419698525,3.5961842657834));
#87575=CARTESIAN_POINT('Ctrl Pts',(-156.687450320061,225.824998625309,3.4374264005516));
#87576=CARTESIAN_POINT('Ctrl Pts',(-157.510174847238,222.664538841213,3.27866853531982));
#87577=CARTESIAN_POINT('Ctrl Pts',(-160.611587255653,221.641493020787,3.11991067008802));
#87578=CARTESIAN_POINT('Ctrl Pts',(-163.153275033114,223.692152649466,2.96115280485623));
#87579=CARTESIAN_POINT('Ctrl Pts',(-162.809085621427,226.93975413479,2.80239493962444));
#87580=CARTESIAN_POINT('Ctrl Pts',(-159.89402116537,228.412092685536,2.64363707439264));
#87581=CARTESIAN_POINT('Ctrl Pts',(-157.075948522366,226.761684200052,2.48487920916085));
#87582=CARTESIAN_POINT('Ctrl Pts',(-156.933967702091,223.498982289014,2.32612134392906));
#87583=CARTESIAN_POINT('Ctrl Pts',(-159.598019467623,221.610011966548,2.16736347869727));
#87584=CARTESIAN_POINT('Ctrl Pts',(-162.629963909868,222.823558064097,2.00860561346547));
#87585=CARTESIAN_POINT('Ctrl Pts',(-163.254965258451,226.028984762691,1.84984774823368));
#87586=CARTESIAN_POINT('Ctrl Pts',(-160.901023001045,228.292682516148,1.69108988300189));
#87587=CARTESIAN_POINT('Ctrl Pts',(-157.722463552137,227.54292178165,1.5323320177701));
#87588=CARTESIAN_POINT('Ctrl Pts',(-156.628307396718,224.465869958378,1.37357415253831));
#87589=CARTESIAN_POINT('Ctrl Pts',(-158.619919975389,221.877672964505,1.21481628730651));
#87590=CARTESIAN_POINT('Ctrl Pts',(-161.874590461213,222.146990050728,1.05605842207472));
#87591=CARTESIAN_POINT('Ctrl Pts',(-163.413617730746,225.027463692089,0.897300556842931));
#87592=CARTESIAN_POINT('Ctrl Pts',(-161.828539743717,227.882632493727,0.738542691611135));
#87593=CARTESIAN_POINT('Ctrl Pts',(-158.569904319348,228.099969035727,0.579784826379343));
#87594=CARTESIAN_POINT('Ctrl Pts',(-156.620254026289,225.479481701384,0.421026961147552));
#87595=CARTESIAN_POINT('Ctrl Pts',(-157.763410728175,222.421691465315,0.262269095915756));
#87596=CARTESIAN_POINT('Ctrl Pts',(-160.954176404753,221.720398721314,0.103511230683968));
#87597=CARTESIAN_POINT('Ctrl Pts',(-163.270121172418,224.027093348395,-0.055246634547828));
#87598=CARTESIAN_POINT('Ctrl Pts',(-162.819257379562,226.146956680238,-0.161085211369022));
#87599=CARTESIAN_POINT('Ctrl Pts',(-162.195197104019,226.876863439079,-0.21400449977962));
#87600=CARTESIAN_POINT('Ctrl Pts',(-160.698066426161,222.388867814061,20.2140044997796));
#87601=CARTESIAN_POINT('Ctrl Pts',(-161.56627230492,222.620976084267,20.161085211369));
#87602=CARTESIAN_POINT('Ctrl Pts',(-163.037711968101,224.016856098884,20.0552466345478));
#87603=CARTESIAN_POINT('Ctrl Pts',(-162.474373110892,227.023489936586,19.896488769316));
#87604=CARTESIAN_POINT('Ctrl Pts',(-159.641842278095,228.174041962934,19.7377309040842));
#87605=CARTESIAN_POINT('Ctrl Pts',(-157.139304377621,226.421794145441,19.5789730388524));
#87606=CARTESIAN_POINT('Ctrl Pts',(-157.253810500337,223.367327422492,19.4202151736207));
#87607=CARTESIAN_POINT('Ctrl Pts',(-159.882141996706,221.807561696636,19.2614573083889));
#87608=CARTESIAN_POINT('Ctrl Pts',(-162.618089965442,223.169284541734,19.1026994431571));
#87609=CARTESIAN_POINT('Ctrl Pts',(-162.958081217784,226.206589355004,18.9439415779253));
#87610=CARTESIAN_POINT('Ctrl Pts',(-160.590779249579,228.139570022159,18.7851837126935));
#87611=CARTESIAN_POINT('Ctrl Pts',(-157.68282380134,227.199242167719,18.6264258474617));
#87612=CARTESIAN_POINT('Ctrl Pts',(-156.89553458589,224.246155515121,18.4676679822299));
#87613=CARTESIAN_POINT('Ctrl Pts',(-158.949458421001,221.982993306815,18.3089101169981));
#87614=CARTESIAN_POINT('Ctrl Pts',(-161.964834771176,222.480992613217,18.1501522517663));
#87615=CARTESIAN_POINT('Ctrl Pts',(-163.181995908446,225.284388774815,17.9913943865345));
#87616=CARTESIAN_POINT('Ctrl Pts',(-161.486993796195,227.827511669135,17.8326365213027));
#87617=CARTESIAN_POINT('Ctrl Pts',(-158.431095366766,227.78289631879,17.673878656071));
#87618=CARTESIAN_POINT('Ctrl Pts',(-156.811058228927,225.191374210904,17.5151207908391));
#87619=CARTESIAN_POINT('Ctrl Pts',(-158.109540555079,222.424706507915,17.3563629256074));
#87620=CARTESIAN_POINT('Ctrl Pts',(-161.138171252083,222.014947271375,17.1976050603756));
#87621=CARTESIAN_POINT('Ctrl Pts',(-163.125147682637,224.337108192152,17.0388471951438));
#87622=CARTESIAN_POINT('Ctrl Pts',(-162.251989067923,227.265947660988,16.880089329912));
#87623=CARTESIAN_POINT('Ctrl Pts',(-159.317810151146,228.12099192365,16.7213314646802));
#87624=CARTESIAN_POINT('Ctrl Pts',(-157.007971355121,226.119704498563,16.5625735994484));
#87625=CARTESIAN_POINT('Ctrl Pts',(-157.436437058239,223.093663561365,16.4038157342166));
#87626=CARTESIAN_POINT('Ctrl Pts',(-160.211075464361,221.812301657386,16.2450578689848));
#87627=CARTESIAN_POINT('Ctrl Pts',(-162.792537614034,223.448321151434,16.086300003753));
#87628=CARTESIAN_POINT('Ctrl Pts',(-162.818269449045,226.504437066565,15.9275421385212));
#87629=CARTESIAN_POINT('Ctrl Pts',(-160.26472119517,228.183692237588,15.7687842732894));
#87630=CARTESIAN_POINT('Ctrl Pts',(-157.468900113859,226.949232397941,15.6100264080576));
#87631=CARTESIAN_POINT('Ctrl Pts',(-156.989541548824,223.930835144362,15.4512685428259));
#87632=CARTESIAN_POINT('Ctrl Pts',(-159.265354439916,221.890937524614,15.292510677594));
#87633=CARTESIAN_POINT('Ctrl Pts',(-162.21351491871,222.69645376008,15.1337528123623));
#87634=CARTESIAN_POINT('Ctrl Pts',(-163.135866630944,225.610175423736,14.9749949471305));
#87635=CARTESIAN_POINT('Ctrl Pts',(-161.188273325853,227.965464563583,14.8162370818987));
#87636=CARTESIAN_POINT('Ctrl Pts',(-158.153172319669,227.606760651453,14.6574792166669));
#87637=CARTESIAN_POINT('Ctrl Pts',(-156.808287933899,224.862349493622,14.4987213514351));
#87638=CARTESIAN_POINT('Ctrl Pts',(-158.384458305513,222.243916073815,14.3399634862033));
#87639=CARTESIAN_POINT('Ctrl Pts',(-161.439172372392,222.147850554872,14.1812056209715));
#87640=CARTESIAN_POINT('Ctrl Pts',(-163.176755940652,224.662072095952,14.0224477557397));
#87641=CARTESIAN_POINT('Ctrl Pts',(-162.00697259695,227.485565241528,13.8636898905079));
#87642=CARTESIAN_POINT('Ctrl Pts',(-159.000408011441,228.0342691758,13.7049320252761));
#87643=CARTESIAN_POINT('Ctrl Pts',(-156.908669974554,225.806010079699,13.5461741600444));
#87644=CARTESIAN_POINT('Ctrl Pts',(-157.646117055391,222.840090590353,13.3874162948125));
#87645=CARTESIAN_POINT('Ctrl Pts',(-160.53783771457,221.85092010778,13.2286584295808));
#87646=CARTESIAN_POINT('Ctrl Pts',(-162.937329318524,223.743787418731,13.069900564349));
#87647=CARTESIAN_POINT('Ctrl Pts',(-162.648577245673,226.786340434661,12.9111426991172));
#87648=CARTESIAN_POINT('Ctrl Pts',(-159.935847381734,228.194034755035,12.7523848338854));
#87649=CARTESIAN_POINT('Ctrl Pts',(-157.28182999151,226.678548593203,12.5936269686536));
#87650=CARTESIAN_POINT('Ctrl Pts',(-157.115481686166,223.626854824879,12.4348691034218));
#87651=CARTESIAN_POINT('Ctrl Pts',(-159.589044428212,221.831863466828,12.27611123819));
#87652=CARTESIAN_POINT('Ctrl Pts',(-162.438713693398,222.936350539352,12.1173533729582));
#87653=CARTESIAN_POINT('Ctrl Pts',(-163.056472282286,225.92948951711,11.9585955077264));
#87654=CARTESIAN_POINT('Ctrl Pts',(-160.876947558619,228.07195972536,11.7998376424946));
#87655=CARTESIAN_POINT('Ctrl Pts',(-157.894840463788,227.402972513763,11.6410797772628));
#87656=CARTESIAN_POINT('Ctrl Pts',(-156.839375293716,224.534784952064,11.482321912031));
#87657=CARTESIAN_POINT('Ctrl Pts',(-158.676513730546,222.092362183943,11.3235640467992));
#87658=CARTESIAN_POINT('Ctrl Pts',(-161.724906749135,222.311009430736,11.1648061815675));
#87659=CARTESIAN_POINT('Ctrl Pts',(-163.194665178747,224.990620740778,11.0060483163357));
#87660=CARTESIAN_POINT('Ctrl Pts',(-161.740666162396,227.678815948491,10.8472904511039));
#87661=CARTESIAN_POINT('Ctrl Pts',(-158.693609542671,227.915358905487,10.6885325858721));
#87662=CARTESIAN_POINT('Ctrl Pts',(-156.84216141812,225.483765506824,10.5297747206403));
#87663=CARTESIAN_POINT('Ctrl Pts',(-157.880767039527,222.60942993534,10.3710168554085));
#87664=CARTESIAN_POINT('Ctrl Pts',(-160.858894583022,221.922943993026,10.2122589901767));
#87665=CARTESIAN_POINT('Ctrl Pts',(-163.05096183791,224.052579587292,10.0535011249449));
#87666=CARTESIAN_POINT('Ctrl Pts',(-162.450788938719,227.049294306012,9.89474325971312));
#87667=CARTESIAN_POINT('Ctrl Pts',(-159.607654099187,228.170494956457,9.73598539448132));
#87668=CARTESIAN_POINT('Ctrl Pts',(-157.123594212651,226.390058747429,9.57722752924954));
#87669=CARTESIAN_POINT('Ctrl Pts',(-157.272020789584,223.337440827417,9.41846966401773));
#87670=CARTESIAN_POINT('Ctrl Pts',(-159.917093832615,221.806396996775,9.25971179878595));
#87671=CARTESIAN_POINT('Ctrl Pts',(-162.638042596777,223.198138509099,9.10095393355415));
#87672=CARTESIAN_POINT('Ctrl Pts',(-162.944654880107,226.238943587039,8.94219606832235));
#87673=CARTESIAN_POINT('Ctrl Pts',(-160.556319132959,228.145867542842,8.78343820309057));
#87674=CARTESIAN_POINT('Ctrl Pts',(-157.658840137204,227.173693647144,8.62468033785877));
#87675=CARTESIAN_POINT('Ctrl Pts',(-156.903990555816,224.212155411058,8.46592247262698));
#87676=CARTESIAN_POINT('Ctrl Pts',(-158.982608695998,221.971652511791,8.30716460739519));
#87677=CARTESIAN_POINT('Ctrl Pts',(-161.992343317594,222.502693114646,8.1484067421634));
#87678=CARTESIAN_POINT('Ctrl Pts',(-163.178685413276,225.319268880773,7.98964887693161));
#87679=CARTESIAN_POINT('Ctrl Pts',(-161.455894743725,227.843649779771,7.83089101169981));
#87680=CARTESIAN_POINT('Ctrl Pts',(-158.40066926197,227.765522512147,7.67213314646803));
#87681=CARTESIAN_POINT('Ctrl Pts',(-156.809151208767,225.156389150158,7.51337528123622));
#87682=CARTESIAN_POINT('Ctrl Pts',(-158.137897843824,222.404128444094,7.35461741600444));
#87683=CARTESIAN_POINT('Ctrl Pts',(-161.170840298987,222.027609283915,7.19585955077264));
#87684=CARTESIAN_POINT('Ctrl Pts',(-163.13222975856,224.371421990211,7.03710168554085));
#87685=CARTESIAN_POINT('Ctrl Pts',(-162.227002666271,227.290509266348,6.87834382030905));
#87686=CARTESIAN_POINT('Ctrl Pts',(-159.283622821385,228.113322551995,6.71958595507727));
#87687=CARTESIAN_POINT('Ctrl Pts',(-156.995871342197,226.086823160485,6.56082808984547));
#87688=CARTESIAN_POINT('Ctrl Pts',(-157.457498292496,223.065663255237,6.40207022461368));
#87689=CARTESIAN_POINT('Ctrl Pts',(-160.246022705521,221.814808262731,6.24331235938189));
#87690=CARTESIAN_POINT('Ctrl Pts',(-162.809387148128,223.479040622918,6.08455449415009));
#87691=CARTESIAN_POINT('Ctrl Pts',(-162.801600583245,226.535254945201,5.9257966289183));
#87692=CARTESIAN_POINT('Ctrl Pts',(-160.229789274746,228.186404002008,5.76703876368651));
#87693=CARTESIAN_POINT('Ctrl Pts',(-157.447674831036,226.92135624148,5.60828089845472));
#87694=CARTESIAN_POINT('Ctrl Pts',(-157.001448281594,223.897883324305,5.44952303322293));
#87695=CARTESIAN_POINT('Ctrl Pts',(-159.299496146922,221.883067545386,5.29076516799113));
#87696=CARTESIAN_POINT('Ctrl Pts',(-162.23864511104,222.72086822636,5.13200730275934));
#87697=CARTESIAN_POINT('Ctrl Pts',(-163.128986157567,225.644530216944,4.97324943752755));
#87698=CARTESIAN_POINT('Ctrl Pts',(-161.155679195733,227.978318178328,4.81449157229575));
#87699=CARTESIAN_POINT('Ctrl Pts',(-158.12469467941,227.586349460022,4.65573370706397));
#87700=CARTESIAN_POINT('Ctrl Pts',(-156.809989518745,224.827353817618,4.49697584183217));
#87701=CARTESIAN_POINT('Ctrl Pts',(-158.414781825084,222.226363954524,4.33821797660038));
#87702=CARTESIAN_POINT('Ctrl Pts',(-161.470365742761,222.163805691214,4.17946011136859));
#87703=CARTESIAN_POINT('Ctrl Pts',(-163.1802709905,224.696932347702,4.02070224613679));
#87704=CARTESIAN_POINT('Ctrl Pts',(-161.979592352761,227.507426507806,3.861944380905));
#87705=CARTESIAN_POINT('Ctrl Pts',(-158.96719087169,228.023124026255,3.70318651567321));
#87706=CARTESIAN_POINT('Ctrl Pts',(-156.900016264091,225.772058555407,3.54442865044142));
#87707=CARTESIAN_POINT('Ctrl Pts',(-157.669946649989,222.814405123663,3.38567078520962));
#87708=CARTESIAN_POINT('Ctrl Pts',(-160.572341769573,221.857008039592,3.22691291997783));
#87709=CARTESIAN_POINT('Ctrl Pts',(-162.950929725432,223.77607706829,3.06815505474604));
#87710=CARTESIAN_POINT('Ctrl Pts',(-162.628826909959,226.815280327998,2.90939718951425));
#87711=CARTESIAN_POINT('Ctrl Pts',(-159.900821815385,228.193139077924,2.75063932428246));
#87712=CARTESIAN_POINT('Ctrl Pts',(-157.263584580022,226.64863712114,2.59188145905066));
#87713=CARTESIAN_POINT('Ctrl Pts',(-157.130714653171,223.595302428353,2.43312359381887));
#87714=CARTESIAN_POINT('Ctrl Pts',(-159.623814513615,221.827547121098,2.27436572858708));
#87715=CARTESIAN_POINT('Ctrl Pts',(-162.461199418682,222.963220100725,2.11560786335528));
#87716=CARTESIAN_POINT('Ctrl Pts',(-163.046094500334,225.962954925072,1.95684999812349));
#87717=CARTESIAN_POINT('Ctrl Pts',(-160.843204455419,228.081391445806,1.7980921328917));
#87718=CARTESIAN_POINT('Ctrl Pts',(-157.868612812338,227.379742774137,1.63933426765991));
#87719=CARTESIAN_POINT('Ctrl Pts',(-156.844668535551,224.50014502366,1.48057640242812));
#87720=CARTESIAN_POINT('Ctrl Pts',(-158.708479556863,222.078032342627,1.32181853719632));
#87721=CARTESIAN_POINT('Ctrl Pts',(-161.754298200098,222.330067381422,1.16306067196453));
#87722=CARTESIAN_POINT('Ctrl Pts',(-163.194566261152,225.025701350026,1.00430280673274));
#87723=CARTESIAN_POINT('Ctrl Pts',(-161.711202552014,227.697654287655,0.845544941500945));
#87724=CARTESIAN_POINT('Ctrl Pts',(-158.6616733999,227.90104436796,0.686787076269153));
#87725=CARTESIAN_POINT('Ctrl Pts',(-156.837131949006,225.448713414009,0.528029211037362));
#87726=CARTESIAN_POINT('Ctrl Pts',(-157.90693241265,222.587141236829,0.369271345805566));
#87727=CARTESIAN_POINT('Ctrl Pts',(-160.89294701113,221.930850370105,0.210513480573778));
#87728=CARTESIAN_POINT('Ctrl Pts',(-163.06027786099,224.089524659872,0.051755615341982));
#87729=CARTESIAN_POINT('Ctrl Pts',(-162.638345947507,226.073356597808,-0.0540829614792118));
#87730=CARTESIAN_POINT('Ctrl Pts',(-162.054331550342,226.756425321227,-0.10700224988981));
#87731=CARTESIAN_POINT('Ctrl Pts',(-160.650199997975,222.567913197965,20.3210067496694));
#87732=CARTESIAN_POINT('Ctrl Pts',(-161.458872983031,222.784105799646,20.2680874612588));
#87733=CARTESIAN_POINT('Ctrl Pts',(-162.82941600038,224.084270294977,20.1622488844376));
#87734=CARTESIAN_POINT('Ctrl Pts',(-162.304705299379,226.884739192954,20.0034910192058));
#87735=CARTESIAN_POINT('Ctrl Pts',(-159.666401159932,227.956397844861,19.8447331539741));
#87736=CARTESIAN_POINT('Ctrl Pts',(-157.335462331131,226.324301693709,19.6859752887422));
#87737=CARTESIAN_POINT('Ctrl Pts',(-157.442116766824,223.479279812341,19.5272174235105));
#87738=CARTESIAN_POINT('Ctrl Pts',(-159.890223522245,222.026467252124,19.3684595582787));
#87739=CARTESIAN_POINT('Ctrl Pts',(-162.438567486465,223.294816735702,19.2097016930469));
#87740=CARTESIAN_POINT('Ctrl Pts',(-162.755245532134,226.123853499867,19.0509438278151));
#87741=CARTESIAN_POINT('Ctrl Pts',(-160.550269505142,227.924289645724,18.8921859625833));
#87742=CARTESIAN_POINT('Ctrl Pts',(-157.841712617577,227.048440090238,18.7334280973515));
#87743=CARTESIAN_POINT('Ctrl Pts',(-157.10840783868,224.29784664586,18.5746702321197));
#87744=CARTESIAN_POINT('Ctrl Pts',(-159.021494077155,222.189869513439,18.4159123668879));
#87745=CARTESIAN_POINT('Ctrl Pts',(-161.830106013357,222.653720997882,18.2571545016561));
#87746=CARTESIAN_POINT('Ctrl Pts',(-162.963806388178,225.264888231089,18.0983966364243));
#87747=CARTESIAN_POINT('Ctrl Pts',(-161.385030603165,227.633629139932,17.9396387711925));
#87748=CARTESIAN_POINT('Ctrl Pts',(-158.538675187457,227.592073065013,17.7808809059608));
#87749=CARTESIAN_POINT('Ctrl Pts',(-157.029724027129,225.178251677604,17.622123040729));
#87750=CARTESIAN_POINT('Ctrl Pts',(-158.239169395355,222.601294431896,17.4633651754972));
#87751=CARTESIAN_POINT('Ctrl Pts',(-161.060126827571,222.219632394038,17.3046073102654));
#87752=CARTESIAN_POINT('Ctrl Pts',(-162.910856246299,224.382562696088,17.1458494450336));
#87753=CARTESIAN_POINT('Ctrl Pts',(-162.097570134487,227.110571586559,16.9870915798018));
#87754=CARTESIAN_POINT('Ctrl Pts',(-159.364587922123,227.906985447785,16.82833371457));
#87755=CARTESIAN_POINT('Ctrl Pts',(-157.213134816495,226.042926339693,16.6695758493382));
#87756=CARTESIAN_POINT('Ctrl Pts',(-157.61222061816,223.224381087403,16.5108179841064));
#87757=CARTESIAN_POINT('Ctrl Pts',(-160.196602015734,222.030882193675,16.3520601188746));
#87758=CARTESIAN_POINT('Ctrl Pts',(-162.601053256459,223.554719799741,16.1933022536428));
#87759=CARTESIAN_POINT('Ctrl Pts',(-162.62502065905,226.401277788152,16.034544388411));
#87760=CARTESIAN_POINT('Ctrl Pts',(-160.246569257757,227.965386399998,15.8757865231792));
#87761=CARTESIAN_POINT('Ctrl Pts',(-157.642457681435,226.815573495153,15.7170286579474));
#87762=CARTESIAN_POINT('Ctrl Pts',(-157.195968742368,224.004147798951,15.5582707927157));
#87763=CARTESIAN_POINT('Ctrl Pts',(-159.315729100014,222.104125997983,15.3995129274839));
#87764=CARTESIAN_POINT('Ctrl Pts',(-162.061734158422,222.854407969786,15.2407550622521));
#87765=CARTESIAN_POINT('Ctrl Pts',(-162.920840196116,225.568335683266,15.0819971970203));
#87766=CARTESIAN_POINT('Ctrl Pts',(-161.106793401185,227.762122601771,14.9232393317885));
#87767=CARTESIAN_POINT('Ctrl Pts',(-158.279809329013,227.428015023753,14.7644814665567));
#87768=CARTESIAN_POINT('Ctrl Pts',(-157.027143691284,224.871788191475,14.6057236013249));
#87769=CARTESIAN_POINT('Ctrl Pts',(-158.495236030387,222.432900801318,14.4469657360931));
#87770=CARTESIAN_POINT('Ctrl Pts',(-161.340488295306,222.343422496845,14.2882078708613));
#87771=CARTESIAN_POINT('Ctrl Pts',(-162.958925725075,224.685243818793,14.1294500056295));
#87772=CARTESIAN_POINT('Ctrl Pts',(-161.869354447612,227.315129985403,13.9706921403977));
#87773=CARTESIAN_POINT('Ctrl Pts',(-159.068950053205,227.826209280413,13.8119342751659));
#87774=CARTESIAN_POINT('Ctrl Pts',(-157.120642533492,225.750741953127,13.6531764099342));
#87775=CARTESIAN_POINT('Ctrl Pts',(-157.807522853899,222.988195619861,13.4944185447023));
#87776=CARTESIAN_POINT('Ctrl Pts',(-160.500958172201,222.066852576186,13.3356606794706));
#87777=CARTESIAN_POINT('Ctrl Pts',(-162.735916591004,223.829925939442,13.1769028142388));
#87778=CARTESIAN_POINT('Ctrl Pts',(-162.466964253308,226.663851036909,13.018144949007));
#87779=CARTESIAN_POINT('Ctrl Pts',(-159.940246327995,227.975019730826,12.8593870837752));
#87780=CARTESIAN_POINT('Ctrl Pts',(-157.468214960952,226.563450484081,12.7006292185434));
#87781=CARTESIAN_POINT('Ctrl Pts',(-157.313273162085,223.721011415786,12.5418713533116));
#87782=CARTESIAN_POINT('Ctrl Pts',(-159.617223659625,222.049102649469,12.3831134880798));
#87783=CARTESIAN_POINT('Ctrl Pts',(-162.271491048824,223.077855022317,12.224355622848));
#87784=CARTESIAN_POINT('Ctrl Pts',(-162.846889919463,225.865754403154,12.0655977576162));
#87785=CARTESIAN_POINT('Ctrl Pts',(-160.816815247761,227.861315388269,11.9068398923844));
#87786=CARTESIAN_POINT('Ctrl Pts',(-158.039191293428,227.238200642559,11.7480820271526));
#87787=CARTESIAN_POINT('Ctrl Pts',(-157.056099390243,224.566684756794,11.5893241619209));
#87788=CARTESIAN_POINT('Ctrl Pts',(-158.767265209342,222.291738964571,11.4305662966891));
#87789=CARTESIAN_POINT('Ctrl Pts',(-161.606629860374,222.495393565473,11.2718084314573));
#87790=CARTESIAN_POINT('Ctrl Pts',(-162.975606926372,224.991263876762,11.1130505662255));
#87791=CARTESIAN_POINT('Ctrl Pts',(-161.621308650367,227.495129487696,10.9542927009937));
#87792=CARTESIAN_POINT('Ctrl Pts',(-158.783188761302,227.715452689608,10.7955348357619));
#87793=CARTESIAN_POINT('Ctrl Pts',(-157.058694470044,225.450593696774,10.6367769705301));
#87794=CARTESIAN_POINT('Ctrl Pts',(-158.026082884138,222.773351370371,10.4780191052983));
#87795=CARTESIAN_POINT('Ctrl Pts',(-160.800000165046,222.133937782244,10.3192612400665));
#87796=CARTESIAN_POINT('Ctrl Pts',(-162.841757326363,224.117544223102,10.1605033748347));
#87797=CARTESIAN_POINT('Ctrl Pts',(-162.282738294342,226.908774156275,10.0017455096029));
#87798=CARTESIAN_POINT('Ctrl Pts',(-159.634557265106,227.953094056686,9.84298764437113));
#87799=CARTESIAN_POINT('Ctrl Pts',(-157.320829412474,226.294742392546,9.68422977913935));
#87800=CARTESIAN_POINT('Ctrl Pts',(-157.45907837619,223.451442541662,9.52547191390754));
#87801=CARTESIAN_POINT('Ctrl Pts',(-159.922778710098,222.025382415754,9.36671404867576));
#87802=CARTESIAN_POINT('Ctrl Pts',(-162.457151965487,223.321692185974,9.20795618344396));
#87803=CARTESIAN_POINT('Ctrl Pts',(-162.742739838688,226.153989201593,9.04919831821217));
#87804=CARTESIAN_POINT('Ctrl Pts',(-160.518172319377,227.930155345293,8.89044045298038));
#87805=CARTESIAN_POINT('Ctrl Pts',(-157.819373513749,227.024643432207,8.73168258774858));
#87806=CARTESIAN_POINT('Ctrl Pts',(-157.116283982586,224.266177929582,8.5729247225168));
#87807=CARTESIAN_POINT('Ctrl Pts',(-159.052371237161,222.179306356947,8.41416685728499));
#87808=CARTESIAN_POINT('Ctrl Pts',(-161.855728298222,222.673933495512,8.25540899205321));
#87809=CARTESIAN_POINT('Ctrl Pts',(-162.960722893725,225.297376607515,8.09665112682141));
#87810=CARTESIAN_POINT('Ctrl Pts',(-161.356064013318,227.648660660014,7.93789326158962));
#87811=CARTESIAN_POINT('Ctrl Pts',(-158.510335401249,227.575890580624,7.77913539635783));
#87812=CARTESIAN_POINT('Ctrl Pts',(-157.027947771377,225.145665543142,7.62037753112604));
#87813=CARTESIAN_POINT('Ctrl Pts',(-158.265582224268,222.582127406304,7.46161966589425));
#87814=CARTESIAN_POINT('Ctrl Pts',(-161.090555757304,222.231426172136,7.30286180066245));
#87815=CARTESIAN_POINT('Ctrl Pts',(-162.917452704141,224.414523596358,7.14410393543066));
#87816=CARTESIAN_POINT('Ctrl Pts',(-162.074297050874,227.133449002169,6.98534607019887));
#87817=CARTESIAN_POINT('Ctrl Pts',(-159.332744818217,227.899841965091,6.82658820496707));
#87818=CARTESIAN_POINT('Ctrl Pts',(-157.201864501689,226.012299675595,6.66783033973529));
#87819=CARTESIAN_POINT('Ctrl Pts',(-157.631837683181,223.198300762802,6.50907247450349));
#87820=CARTESIAN_POINT('Ctrl Pts',(-160.229152923901,222.033216921042,6.3503146092717));
#87821=CARTESIAN_POINT('Ctrl Pts',(-162.616747417678,223.583332836479,6.1915567440399));
#87822=CARTESIAN_POINT('Ctrl Pts',(-162.609494777697,226.429982484261,6.03279887880811));
#87823=CARTESIAN_POINT('Ctrl Pts',(-160.214032619784,227.96791221868,5.87404101357632));
#87824=CARTESIAN_POINT('Ctrl Pts',(-157.622687816661,226.789608807273,5.71528314834453));
#87825=CARTESIAN_POINT('Ctrl Pts',(-157.207059030245,223.973455485825,5.55652528311273));
#87826=CARTESIAN_POINT('Ctrl Pts',(-159.347529709518,222.096795663381,5.39776741788095));
#87827=CARTESIAN_POINT('Ctrl Pts',(-162.085141172983,222.877148335646,5.23900955264915));
#87828=CARTESIAN_POINT('Ctrl Pts',(-162.91443151693,225.600334767647,5.08025168741736));
#87829=CARTESIAN_POINT('Ctrl Pts',(-161.07643425119,227.774094843907,4.92149382218557));
#87830=CARTESIAN_POINT('Ctrl Pts',(-158.253284401091,227.409003428108,4.76273595695378));
#87831=CARTESIAN_POINT('Ctrl Pts',(-157.028728598424,224.839192169644,4.60397809172198));
#87832=CARTESIAN_POINT('Ctrl Pts',(-158.523480265641,222.416552231182,4.44522022649019));
#87833=CARTESIAN_POINT('Ctrl Pts',(-161.369542735673,222.358283589184,4.28646236125839));
#87834=CARTESIAN_POINT('Ctrl Pts',(-162.962199747888,224.717713702413,4.12770449602661));
#87835=CARTESIAN_POINT('Ctrl Pts',(-161.843851667291,227.335492224234,3.96894663079481));
#87836=CARTESIAN_POINT('Ctrl Pts',(-159.038010613361,227.815828353986,3.81018876556302));
#87837=CARTESIAN_POINT('Ctrl Pts',(-157.112582208121,225.719118485504,3.65143090033122));
#87838=CARTESIAN_POINT('Ctrl Pts',(-157.82971845274,222.964271406113,3.49267303509944));
#87839=CARTESIAN_POINT('Ctrl Pts',(-160.533096283493,222.072523058399,3.33391516986764));
#87840=CARTESIAN_POINT('Ctrl Pts',(-162.74858441775,223.860001487113,3.17515730463585));
#87841=CARTESIAN_POINT('Ctrl Pts',(-162.448568198491,226.690806521207,3.01639943940406));
#87842=CARTESIAN_POINT('Ctrl Pts',(-159.9076224654,227.974185470311,2.85764157417226));
#87843=CARTESIAN_POINT('Ctrl Pts',(-157.451220637679,226.535590042229,2.69888370894047));
#87844=CARTESIAN_POINT('Ctrl Pts',(-157.327461604252,223.691622567693,2.54012584370868));
#87845=CARTESIAN_POINT('Ctrl Pts',(-159.649609559608,222.045082275649,2.38136797847689));
#87846=CARTESIAN_POINT('Ctrl Pts',(-162.292434927495,223.102882137353,2.2226101132451));
#87847=CARTESIAN_POINT('Ctrl Pts',(-162.837223742218,225.896925087452,2.0638522480133));
#87848=CARTESIAN_POINT('Ctrl Pts',(-160.785385909792,227.870100375464,1.90509438278151));
#87849=CARTESIAN_POINT('Ctrl Pts',(-158.014762072539,227.216563766624,1.74633651754972));
#87850=CARTESIAN_POINT('Ctrl Pts',(-157.061029674385,224.534420088943,1.58757865231793));
#87851=CARTESIAN_POINT('Ctrl Pts',(-158.797039138337,222.278391720749,1.42882078708613));
#87852=CARTESIAN_POINT('Ctrl Pts',(-161.634005938982,222.513144712115,1.27006292185434));
#87853=CARTESIAN_POINT('Ctrl Pts',(-162.975514791558,225.023939007964,1.11130505662255));
#87854=CARTESIAN_POINT('Ctrl Pts',(-161.593865360312,227.512676081583,0.952547191390756));
#87855=CARTESIAN_POINT('Ctrl Pts',(-158.753442480452,227.702119700194,0.793789326158963));
#87856=CARTESIAN_POINT('Ctrl Pts',(-157.054009871723,225.417945126632,0.635031460927172));
#87857=CARTESIAN_POINT('Ctrl Pts',(-158.050454097125,222.752591008343,0.476273595695375));
#87858=CARTESIAN_POINT('Ctrl Pts',(-160.831717617507,222.141302018896,0.317515730463588));
#87859=CARTESIAN_POINT('Ctrl Pts',(-162.850434549562,224.151955971349,0.158757865231792));
#87860=CARTESIAN_POINT('Ctrl Pts',(-162.457434515453,225.999756515378,0.0529192884105984));
#87861=CARTESIAN_POINT('Ctrl Pts',(-161.913465996665,226.635987203375,0.));
#87862=CARTESIAN_POINT('Ctrl Pts',(-161.913465996665,226.635987203375,0.));
#87863=CARTESIAN_POINT('Ctrl Pts',(-161.975061835647,226.578102239736,-1.1918084162755E-16));
#87864=CARTESIAN_POINT('Ctrl Pts',(-162.03328572045,226.517065589828,-7.91451747642661E-15));
#87865=CARTESIAN_POINT('Ctrl Pts',(-162.088141282815,226.453262312389,-5.71764857681956E-15));
#87866=CARTESIAN_POINT('Ctrl Pts',(-162.144450866834,226.387767841878,-3.46254866446102E-15));
#87867=CARTESIAN_POINT('Ctrl Pts',(-162.197211632774,226.319357701911,2.40033719953046E-15));
#87868=CARTESIAN_POINT('Ctrl Pts',(-162.246401946459,226.248399837308,1.66533453693773E-15));
#87869=CARTESIAN_POINT('Ctrl Pts',(-162.297290196901,226.174992670038,9.0496126895645E-16));
#87870=CARTESIAN_POINT('Ctrl Pts',(-162.344357835219,226.098858337835,3.49623503131884E-15));
#87871=CARTESIAN_POINT('Ctrl Pts',(-162.387545974877,226.02036021425,4.05231403988182E-15));
#87872=CARTESIAN_POINT('Ctrl Pts',(-162.406440785977,225.986017285181,4.29559860612813E-15));
#87873=CARTESIAN_POINT('Ctrl Pts',(-162.424592542808,225.951221405267,1.66664251847669E-15));
#87874=CARTESIAN_POINT('Ctrl Pts',(-162.441993869605,225.916000914244,1.66533453693773E-15));
#87875=CARTESIAN_POINT('Ctrl Pts',(-162.451521836186,225.896716197316,1.66461836141054E-15));
#87876=CARTESIAN_POINT('Ctrl Pts',(-162.460824794419,225.877304161032,1.76785945204013E-15));
#87877=CARTESIAN_POINT('Ctrl Pts',(-162.469901328297,225.857769327789,1.60982338570648E-15));
#87878=CARTESIAN_POINT('Ctrl Pts',(-162.478557483357,225.83913924852,1.45910674500921E-15));
#87879=CARTESIAN_POINT('Ctrl Pts',(-162.487010198395,225.820391466247,1.64355834195759E-15));
#87880=CARTESIAN_POINT('Ctrl Pts',(-162.495244121967,225.801562756482,1.55431223447522E-15));
#87881=CARTESIAN_POINT('Ctrl Pts',(-162.531783565047,225.718007138947,1.15826737976362E-15));
#87882=CARTESIAN_POINT('Ctrl Pts',(-162.564063594148,225.632767868306,-2.35018207924615E-16));
#87883=CARTESIAN_POINT('Ctrl Pts',(-162.592060513761,225.546244193452,1.60982338570648E-15));
#87884=CARTESIAN_POINT('Ctrl Pts',(-162.620521982054,225.458284844261,3.48527615872856E-15));
#87885=CARTESIAN_POINT('Ctrl Pts',(-162.644557514902,225.368997357617,3.19370643993033E-15));
#87886=CARTESIAN_POINT('Ctrl Pts',(-162.664103104093,225.278764048794,1.74860126378462E-15));
#87887=CARTESIAN_POINT('Ctrl Pts',(-162.68330511497,225.190116888533,3.28898586209486E-16));
#87888=CARTESIAN_POINT('Ctrl Pts',(-162.698173901202,225.100555955463,9.49040340436925E-15));
#87889=CARTESIAN_POINT('Ctrl Pts',(-162.708606125223,225.010420931865,9.54791801177635E-15));
#87890=CARTESIAN_POINT('Ctrl Pts',(-162.712740047564,224.974703601891,9.57070902163041E-15));
#87891=CARTESIAN_POINT('Ctrl Pts',(-162.716176818268,224.938895943555,8.03528719691709E-15));
#87892=CARTESIAN_POINT('Ctrl Pts',(-162.718907967693,224.90301855582,8.40993941153556E-15));
#87893=CARTESIAN_POINT('Ctrl Pts',(-162.720526171663,224.881761230701,8.63192056555412E-15));
#87894=CARTESIAN_POINT('Ctrl Pts',(-162.721896640762,224.860479422577,7.91625006826265E-15));
#87895=CARTESIAN_POINT('Ctrl Pts',(-162.723017408846,224.839177393018,8.07687250414801E-15));
#87896=CARTESIAN_POINT('Ctrl Pts',(-162.723759407018,224.825074504822,8.18321167943288E-15));
#87897=CARTESIAN_POINT('Ctrl Pts',(-162.724391877827,224.810962840671,-1.70682398921736E-15));
#87898=CARTESIAN_POINT('Ctrl Pts',(-162.72491390905,224.796858035091,-1.2490009027033E-15));
#87899=CARTESIAN_POINT('Ctrl Pts',(-162.728436906185,224.701669878708,1.84067908658679E-15));
#87900=CARTESIAN_POINT('Ctrl Pts',(-162.726943158831,224.606632526655,3.561771636142E-15));
#87901=CARTESIAN_POINT('Ctrl Pts',(-162.720374596608,224.512145277437,4.24660306919122E-15));
#87902=CARTESIAN_POINT('Ctrl Pts',(-162.713827767741,224.417970657526,4.92916860522656E-15));
#87903=CARTESIAN_POINT('Ctrl Pts',(-162.702240009616,224.324341551697,7.98702549658127E-15));
#87904=CARTESIAN_POINT('Ctrl Pts',(-162.685505817175,224.23163540663,7.88258347483861E-15));
#87905=CARTESIAN_POINT('Ctrl Pts',(-162.683601528504,224.221085793176,7.87069836240063E-15));
#87906=CARTESIAN_POINT('Ctrl Pts',(-162.681630540887,224.210548121617,1.13803607953457E-14));
#87907=CARTESIAN_POINT('Ctrl Pts',(-162.679592656004,224.20002294205,1.14908083048704E-14));
#87908=CARTESIAN_POINT('Ctrl Pts',(-162.662059443819,224.109468167218,1.24420909448365E-14));
#87909=CARTESIAN_POINT('Ctrl Pts',(-162.639578714029,224.019837772689,9.58219353840262E-15));
#87910=CARTESIAN_POINT('Ctrl Pts',(-162.612425368603,223.931369358019,1.01585406753202E-14));
#87911=CARTESIAN_POINT('Ctrl Pts',(-162.60172511415,223.896506819604,1.03856604250736E-14));
#87912=CARTESIAN_POINT('Ctrl Pts',(-162.590298676337,223.86182477492,8.90058523051191E-15));
#87913=CARTESIAN_POINT('Ctrl Pts',(-162.578160711599,223.827338101979,8.90953977261688E-15));
#87914=CARTESIAN_POINT('Ctrl Pts',(-162.572850315517,223.812250078835,8.91345741172205E-15));
#87915=CARTESIAN_POINT('Ctrl Pts',(-162.56740371175,223.797199455213,5.91681775914833E-15));
#87916=CARTESIAN_POINT('Ctrl Pts',(-162.561822058418,223.782187496193,5.82867087928207E-15));
#87917=CARTESIAN_POINT('Ctrl Pts',(-162.55740131404,223.770297823102,5.75885736698703E-15));
#87918=CARTESIAN_POINT('Ctrl Pts',(-162.552896256506,223.758433615952,6.99654648590045E-15));
#87919=CARTESIAN_POINT('Ctrl Pts',(-162.548311193376,223.746604662409,7.105427357601E-15));
#87920=CARTESIAN_POINT('Ctrl Pts',(-162.514552827935,223.659511829625,7.9070826788108E-15));
#87921=CARTESIAN_POINT('Ctrl Pts',(-162.476411491524,223.574193830615,9.12682322584472E-15));
#87922=CARTESIAN_POINT('Ctrl Pts',(-162.434220451094,223.490881399508,8.42381719934338E-15));
#87923=CARTESIAN_POINT('Ctrl Pts',(-162.390447085663,223.404444434346,7.69444576443903E-15));
#87924=CARTESIAN_POINT('Ctrl Pts',(-162.342314439683,223.320165571839,1.09227548171616E-14));
#87925=CARTESIAN_POINT('Ctrl Pts',(-162.290138616362,223.238305524255,9.53404022396853E-15));
#87926=CARTESIAN_POINT('Ctrl Pts',(-162.237361096172,223.155501458327,8.12931083370241E-15));
#87927=CARTESIAN_POINT('Ctrl Pts',(-162.180446197562,223.075171502158,1.26107348299605E-14));
#87928=CARTESIAN_POINT('Ctrl Pts',(-162.119669180754,222.997600288849,1.22402088464924E-14));
#87929=CARTESIAN_POINT('Ctrl Pts',(-162.076869866936,222.94297446356,1.19792836040716E-14));
#87930=CARTESIAN_POINT('Ctrl Pts',(-162.032154224472,222.889716988046,9.06583501434719E-15));
#87931=CARTESIAN_POINT('Ctrl Pts',(-161.985604958578,222.837934980372,8.52096171399808E-15));
#87932=CARTESIAN_POINT('Ctrl Pts',(-161.9743988715,222.825469183633,8.38979106001418E-15));
#87933=CARTESIAN_POINT('Ctrl Pts',(-161.963085875323,222.813088400073,5.60125771483385E-15));
#87934=CARTESIAN_POINT('Ctrl Pts',(-161.951678364305,222.800806055908,5.71764857681956E-15));
#87935=CARTESIAN_POINT('Ctrl Pts',(-161.883012077408,222.726873804882,6.41825086494875E-15));
#87936=CARTESIAN_POINT('Ctrl Pts',(-161.810832846144,222.656402638005,1.24845656601378E-14));
#87937=CARTESIAN_POINT('Ctrl Pts',(-161.73545380071,222.589679529204,1.12479470182336E-14));
#87938=CARTESIAN_POINT('Ctrl Pts',(-161.670633848202,222.532302990158,1.01845538540404E-14));
#87939=CARTESIAN_POINT('Ctrl Pts',(-161.603446707105,222.477697927691,1.0704076426586E-14));
#87940=CARTESIAN_POINT('Ctrl Pts',(-161.534065264026,222.426062117926,1.09842690498851E-14));
#87941=CARTESIAN_POINT('Ctrl Pts',(-161.508545546914,222.407069557385,1.10873288331103E-14));
#87942=CARTESIAN_POINT('Ctrl Pts',(-161.482728748481,222.38847887615,5.71429167113529E-15));
#87943=CARTESIAN_POINT('Ctrl Pts',(-161.456622762885,222.370300567934,5.88418203051333E-15));
#87944=CARTESIAN_POINT('Ctrl Pts',(-161.439930310342,222.358677158962,5.99281178329901E-15));
#87945=CARTESIAN_POINT('Ctrl Pts',(-161.423118575947,222.347221775582,1.01871413174874E-14));
#87946=CARTESIAN_POINT('Ctrl Pts',(-161.406204408697,222.335946808143,9.91567938868343E-15));
#87947=CARTESIAN_POINT('Ctrl Pts',(-161.320010751063,222.278490199795,8.53232446466678E-15));
#87948=CARTESIAN_POINT('Ctrl Pts',(-161.231075434318,222.225655712217,6.65843379994348E-15));
#87949=CARTESIAN_POINT('Ctrl Pts',(-161.139704820809,222.177762703399,5.31519273039294E-15));
#87950=CARTESIAN_POINT('Ctrl Pts',(-161.0483342073,222.129869694581,3.97195166084239E-15));
#87951=CARTESIAN_POINT('Ctrl Pts',(-160.954527658396,222.086917262382,1.53223770557588E-16));
#87952=CARTESIAN_POINT('Ctrl Pts',(-160.858553722692,222.049265214854,1.94115556961805E-15));
#87953=CARTESIAN_POINT('Ctrl Pts',(-160.837669284051,222.04107192914,2.34062737524038E-15));
#87954=CARTESIAN_POINT('Ctrl Pts',(-160.816682093783,222.033129809198,7.10494195145333E-16));
#87955=CARTESIAN_POINT('Ctrl Pts',(-160.795596246196,222.025437627191,7.49400541621981E-16));
#87956=CARTESIAN_POINT('Ctrl Pts',(-162.514309478995,225.001427434952,19.112583302492));
#87957=CARTESIAN_POINT('Ctrl Pts',(-162.515998851658,225.327429263472,19.092036810933));
#87958=CARTESIAN_POINT('Ctrl Pts',(-162.457161905,225.65284616228,19.071490319374));
#87959=CARTESIAN_POINT('Ctrl Pts',(-162.334969853357,225.952420063482,19.050943827815));
#87960=CARTESIAN_POINT('Ctrl Pts',(-162.020253523137,226.723998881819,18.9980245394044));
#87961=CARTESIAN_POINT('Ctrl Pts',(-161.28526151414,227.324144263772,18.9451052509938));
#87962=CARTESIAN_POINT('Ctrl Pts',(-160.466339361713,227.478242028834,18.8921859625833));
#87963=CARTESIAN_POINT('Ctrl Pts',(-159.647417209287,227.632339793896,18.8392666741727));
#87964=CARTESIAN_POINT('Ctrl Pts',(-158.744564913432,227.340389942067,18.7863473857621));
#87965=CARTESIAN_POINT('Ctrl Pts',(-158.170921302355,226.735982775423,18.7334280973515));
#87966=CARTESIAN_POINT('Ctrl Pts',(-157.597277691277,226.131575608779,18.6805088089409));
#87967=CARTESIAN_POINT('Ctrl Pts',(-157.352842764978,225.214711127319,18.6275895205303));
#87968=CARTESIAN_POINT('Ctrl Pts',(-157.549473008242,224.404949364519,18.5746702321197));
#87969=CARTESIAN_POINT('Ctrl Pts',(-157.746103251505,223.595187601719,18.5217509437091));
#87970=CARTESIAN_POINT('Ctrl Pts',(-158.38379866433,222.892528557579,18.4688316552985));
#87971=CARTESIAN_POINT('Ctrl Pts',(-159.170748360109,222.61850761625,18.4159123668879));
#87972=CARTESIAN_POINT('Ctrl Pts',(-159.957698055889,222.34448667492,18.3629930784773));
#87973=CARTESIAN_POINT('Ctrl Pts',(-160.893902034623,222.499103836401,18.3100737900667));
#87974=CARTESIAN_POINT('Ctrl Pts',(-161.55095408646,223.011606956009,18.2571545016561));
#87975=CARTESIAN_POINT('Ctrl Pts',(-162.149291705253,223.478312592728,18.2089641019347));
#87976=CARTESIAN_POINT('Ctrl Pts',(-162.516138545369,224.241800343922,18.1607737022133));
#87977=CARTESIAN_POINT('Ctrl Pts',(-162.520906539752,225.001296842262,18.1125833024919));
#87978=CARTESIAN_POINT('Origin',(160.,225.,22.2084234471774));
#87979=CARTESIAN_POINT('Ctrl Pts',(156.923621908153,225.002226325067,19.7084234471775));
#87980=CARTESIAN_POINT('Ctrl Pts',(156.922437019742,225.146330804243,19.7009407276991));
#87981=CARTESIAN_POINT('Ctrl Pts',(156.9971729149,226.308361189561,19.6405387198101));
#87982=CARTESIAN_POINT('Ctrl Pts',(158.478135103599,228.298893815846,19.5272174235105));
#87983=CARTESIAN_POINT('Ctrl Pts',(161.945877075973,228.067610948411,19.3684595582787));
#87984=CARTESIAN_POINT('Ctrl Pts',(163.632669423604,225.029226006693,19.2097016930469));
#87985=CARTESIAN_POINT('Ctrl Pts',(161.994882852242,221.963912542979,19.0509438278151));
#87986=CARTESIAN_POINT('Ctrl Pts',(158.531360299265,221.677313366987,18.8921859625833));
#87987=CARTESIAN_POINT('Ctrl Pts',(157.007146929903,223.658102464642,18.7780125023707));
#87988=CARTESIAN_POINT('Ctrl Pts',(156.922679294227,224.836964788643,18.7167583305688));
#87989=CARTESIAN_POINT('Ctrl Pts',(156.924068523622,224.997572468126,18.7084234471774));
#87990=CARTESIAN_POINT('Ctrl Pts',(156.929637674279,224.99697422706,19.7915765528225));
#87991=CARTESIAN_POINT('Ctrl Pts',(156.934919299465,225.700310641978,19.7552124583938));
#87992=CARTESIAN_POINT('Ctrl Pts',(157.522174047868,227.437424493836,19.6659290755545));
#87993=CARTESIAN_POINT('Ctrl Pts',(160.40727547618,228.609329940462,19.5237264043046));
#87994=CARTESIAN_POINT('Ctrl Pts',(163.25301142787,226.616779086673,19.3649685390728));
#87995=CARTESIAN_POINT('Ctrl Pts',(163.122801956202,223.143422649729,19.2062106738411));
#87996=CARTESIAN_POINT('Ctrl Pts',(160.13402104345,221.369750709928,19.0474528086092));
#87997=CARTESIAN_POINT('Ctrl Pts',(157.425511910903,222.717816803407,18.9092414349364));
#87998=CARTESIAN_POINT('Ctrl Pts',(156.933644860339,224.374657834208,18.8239493496742));
#87999=CARTESIAN_POINT('Ctrl Pts',(156.930395245889,225.001742688239,18.7915765528225));
#88000=CARTESIAN_POINT('Ctrl Pts',(161.913465996665,226.635987203375,20.));
#88001=CARTESIAN_POINT('Ctrl Pts',(162.457434515453,225.999756515379,19.9470807115894));
#88002=CARTESIAN_POINT('Ctrl Pts',(162.85043342369,224.151954738239,19.8412421347682));
#88003=CARTESIAN_POINT('Ctrl Pts',(160.831717966777,222.141302178128,19.6824842695364));
#88004=CARTESIAN_POINT('Ctrl Pts',(158.050453807979,222.752590618786,19.5237264043046));
#88005=CARTESIAN_POINT('Ctrl Pts',(157.054009754812,225.417945292734,19.3649685390728));
#88006=CARTESIAN_POINT('Ctrl Pts',(158.753442369712,227.702119792221,19.206210673841));
#88007=CARTESIAN_POINT('Ctrl Pts',(161.593865475439,227.512676285221,19.0474528086092));
#88008=CARTESIAN_POINT('Ctrl Pts',(162.975514974434,225.023938985472,18.8886949433775));
#88009=CARTESIAN_POINT('Ctrl Pts',(161.634006045394,222.51314456709,18.7299370781457));
#88010=CARTESIAN_POINT('Ctrl Pts',(158.79703906081,222.278391541041,18.5711792129139));
#88011=CARTESIAN_POINT('Ctrl Pts',(157.061029488215,224.534420062994,18.4124213476821));
#88012=CARTESIAN_POINT('Ctrl Pts',(158.014761946265,227.216563905499,18.2536634824503));
#88013=CARTESIAN_POINT('Ctrl Pts',(160.785385959748,227.870100558722,18.0949056172185));
#88014=CARTESIAN_POINT('Ctrl Pts',(162.837223922373,225.896925143905,17.9361477519867));
#88015=CARTESIAN_POINT('Ctrl Pts',(162.292435073093,223.102882017134,17.7773898867549));
#88016=CARTESIAN_POINT('Ctrl Pts',(159.649609537352,222.045082087855,17.6186320215231));
#88017=CARTESIAN_POINT('Ctrl Pts',(157.327461434526,223.691622484669,17.4598741562913));
#88018=CARTESIAN_POINT('Ctrl Pts',(157.451220475812,226.535590139715,17.3011162910595));
#88019=CARTESIAN_POINT('Ctrl Pts',(159.907622459533,227.974185659212,17.1423584258277));
#88020=CARTESIAN_POINT('Ctrl Pts',(162.448568353993,226.690806628577,16.983600560596));
#88021=CARTESIAN_POINT('Ctrl Pts',(162.748584592305,223.86000141472,16.8248426953641));
#88022=CARTESIAN_POINT('Ctrl Pts',(160.533096317349,222.07252287248,16.6660848301324));
#88023=CARTESIAN_POINT('Ctrl Pts',(157.829718314911,222.96427127683,16.5073269649006));
#88024=CARTESIAN_POINT('Ctrl Pts',(157.112582024748,225.719118531172,16.3485690996688));
#88025=CARTESIAN_POINT('Ctrl Pts',(159.038010552267,227.815828532812,16.189811234437));
#88026=CARTESIAN_POINT('Ctrl Pts',(161.843851784389,227.335492372555,16.0310533692052));
#88027=CARTESIAN_POINT('Ctrl Pts',(162.96219993601,224.717713684486,15.8722955039734));
#88028=CARTESIAN_POINT('Ctrl Pts',(161.369542822649,222.358283421415,15.7135376387416));
#88029=CARTESIAN_POINT('Ctrl Pts',(158.523480171871,222.416552067114,15.5547797735098));
#88030=CARTESIAN_POINT('Ctrl Pts',(157.028728409726,224.839192159431,15.396021908278));
#88031=CARTESIAN_POINT('Ctrl Pts',(158.253284290161,227.409003581098,15.2372640430462));
#88032=CARTESIAN_POINT('Ctrl Pts',(161.076434319551,227.774095020083,15.0785061778144));
#88033=CARTESIAN_POINT('Ctrl Pts',(162.914431702018,225.600334805773,14.9197483125826));
#88034=CARTESIAN_POINT('Ctrl Pts',(162.085141305405,222.877148200829,14.7609904473508));
#88035=CARTESIAN_POINT('Ctrl Pts',(159.347529668082,222.096795479006,14.6022325821191));
#88036=CARTESIAN_POINT('Ctrl Pts',(157.207058852872,223.973455420632,14.4434747168873));
#88037=CARTESIAN_POINT('Ctrl Pts',(157.622687665684,226.789608920927,14.2847168516555));
#88038=CARTESIAN_POINT('Ctrl Pts',(160.214032633376,227.967912407165,14.1259589864237));
#88039=CARTESIAN_POINT('Ctrl Pts',(162.609494943419,226.429982575076,13.9672011211919));
#88040=CARTESIAN_POINT('Ctrl Pts',(162.616747583861,223.58333274651,13.8084432559601));
#88041=CARTESIAN_POINT('Ctrl Pts',(160.229152938454,222.03321673263,13.6496853907283));
#88042=CARTESIAN_POINT('Ctrl Pts',(157.631837532785,223.19830064838,13.4909275254965));
#88043=CARTESIAN_POINT('Ctrl Pts',(157.201864323986,226.012299739883,13.3321696602647));
#88044=CARTESIAN_POINT('Ctrl Pts',(159.33274477584,227.899842149253,13.1734117950329));
#88045=CARTESIAN_POINT('Ctrl Pts',(162.074297182607,227.133449137659,13.0146539298011));
#88046=CARTESIAN_POINT('Ctrl Pts',(162.917452889421,224.414523559176,12.8558960645693));
#88047=CARTESIAN_POINT('Ctrl Pts',(161.090555826563,222.231425996311,12.6971381993376));
#88048=CARTESIAN_POINT('Ctrl Pts',(158.26558211412,222.582127252751,12.5383803341057));
#88049=CARTESIAN_POINT('Ctrl Pts',(157.02794758263,225.145665552392,12.379622468874));
#88050=CARTESIAN_POINT('Ctrl Pts',(158.510335306644,227.575890744212,12.2208646036422));
#88051=CARTESIAN_POINT('Ctrl Pts',(161.356064099438,227.648660828224,12.0621067384104));
#88052=CARTESIAN_POINT('Ctrl Pts',(162.960723081753,225.297376626401,11.9033488731786));
#88053=CARTESIAN_POINT('Ctrl Pts',(161.855728416075,222.67393334779,11.7445910079468));
#88054=CARTESIAN_POINT('Ctrl Pts',(159.05237117698,222.179306177811,11.585833142715));
#88055=CARTESIAN_POINT('Ctrl Pts',(157.116283799449,224.266177882979,11.4270752774832));
#88056=CARTESIAN_POINT('Ctrl Pts',(157.819373375262,227.024643560787,11.2683174122514));
#88057=CARTESIAN_POINT('Ctrl Pts',(160.518172352285,227.93015553138,11.1095595470196));
#88058=CARTESIAN_POINT('Ctrl Pts',(162.742740012873,226.15398927488,10.9508016817878));
#88059=CARTESIAN_POINT('Ctrl Pts',(162.457152121535,223.321692079389,10.792043816556));
#88060=CARTESIAN_POINT('Ctrl Pts',(159.922778705194,222.025382226843,10.6332859513242));
#88061=CARTESIAN_POINT('Ctrl Pts',(157.459078214822,223.451442443317,10.4745280860925));
#88062=CARTESIAN_POINT('Ctrl Pts',(157.320829242326,226.294742474771,10.3157702208606));
#88063=CARTESIAN_POINT('Ctrl Pts',(159.634557241897,227.95309424423,10.1570123556289));
#88064=CARTESIAN_POINT('Ctrl Pts',(162.282738439313,226.908774277497,9.99825449039706));
#88065=CARTESIAN_POINT('Ctrl Pts',(162.841757506836,224.117544167059,9.83949662516529));
#88066=CARTESIAN_POINT('Ctrl Pts',(160.800000215852,222.133937600228,9.68073875993349));
#88067=CARTESIAN_POINT('Ctrl Pts',(158.026082758779,222.773351228962,9.52198089470171));
#88068=CARTESIAN_POINT('Ctrl Pts',(157.058694283249,225.45059372539,9.3632230294699));
#88069=CARTESIAN_POINT('Ctrl Pts',(158.783188684025,227.715452862059,9.20446516423811));
#88070=CARTESIAN_POINT('Ctrl Pts',(161.621308753332,227.495129646155,9.04570729900632));
#88071=CARTESIAN_POINT('Ctrl Pts',(162.975607115345,224.991263876208,8.88694943377453));
#88072=CARTESIAN_POINT('Ctrl Pts',(161.606629962408,222.495393406412,8.72819156854274));
#88073=CARTESIAN_POINT('Ctrl Pts',(158.767265131054,222.291738792576,8.56943370331094));
#88074=CARTESIAN_POINT('Ctrl Pts',(157.056099203283,224.566684729275,8.41067583807915));
#88075=CARTESIAN_POINT('Ctrl Pts',(158.039191168902,227.238200784702,8.25191797284736));
#88076=CARTESIAN_POINT('Ctrl Pts',(160.816815299634,227.861315569984,8.09316010761556));
#88077=CARTESIAN_POINT('Ctrl Pts',(162.846890100262,225.865754458136,7.93440224238378));
#88078=CARTESIAN_POINT('Ctrl Pts',(162.271491193081,223.077854900246,7.77564437715198));
#88079=CARTESIAN_POINT('Ctrl Pts',(159.617223635317,222.049102462065,7.61688651192019));
#88080=CARTESIAN_POINT('Ctrl Pts',(157.313272991458,223.72101133456,7.4581286466884));
#88081=CARTESIAN_POINT('Ctrl Pts',(157.468214800164,226.563450583371,7.2993707814566));
#88082=CARTESIAN_POINT('Ctrl Pts',(159.9402463242,227.975019919762,7.14061291622481));
#88083=CARTESIAN_POINT('Ctrl Pts',(162.466964409978,226.663851142576,6.98185505099302));
#88084=CARTESIAN_POINT('Ctrl Pts',(162.735916764755,223.829925865134,6.82309718576123));
#88085=CARTESIAN_POINT('Ctrl Pts',(160.500958204016,222.066852389909,6.66433932052943));
#88086=CARTESIAN_POINT('Ctrl Pts',(157.807522714661,222.988195492096,6.50558145529764));
#88087=CARTESIAN_POINT('Ctrl Pts',(157.120642350631,225.750742000804,6.34682359006585));
#88088=CARTESIAN_POINT('Ctrl Pts',(159.068949994076,227.826209459899,6.18806572483406));
#88089=CARTESIAN_POINT('Ctrl Pts',(161.86935456633,227.315130132432,6.02930785960226));
#88090=CARTESIAN_POINT('Ctrl Pts',(162.958925912989,224.685243798804,5.87054999437047));
#88091=CARTESIAN_POINT('Ctrl Pts',(161.340488380438,222.343422328133,5.71179212913868));
#88092=CARTESIAN_POINT('Ctrl Pts',(158.495235934823,222.432900638288,5.55303426390689));
#88093=CARTESIAN_POINT('Ctrl Pts',(157.027143502485,224.871788183333,5.39427639867509));
#88094=CARTESIAN_POINT('Ctrl Pts',(158.279809219768,227.42801517795,5.2355185334433));
#88095=CARTESIAN_POINT('Ctrl Pts',(161.106793471474,227.762122777187,5.07676066821151));
#88096=CARTESIAN_POINT('Ctrl Pts',(162.920840381611,225.56833571936,4.91800280297972));
#88097=CARTESIAN_POINT('Ctrl Pts',(162.061734289357,222.854407833525,4.75924493774793));
#88098=CARTESIAN_POINT('Ctrl Pts',(159.315729056558,222.104125814073,4.60048707251613));
#88099=CARTESIAN_POINT('Ctrl Pts',(157.195968564291,224.004147735707,4.44172920728434));
#88100=CARTESIAN_POINT('Ctrl Pts',(157.642457531714,226.815573610455,4.28297134205255));
#88101=CARTESIAN_POINT('Ctrl Pts',(160.246569273415,227.965386588322,4.12421347682076));
#88102=CARTESIAN_POINT('Ctrl Pts',(162.625020825759,226.401277877144,3.96545561158896));
#88103=CARTESIAN_POINT('Ctrl Pts',(162.601053421645,223.554719707956,3.80669774635717));
#88104=CARTESIAN_POINT('Ctrl Pts',(160.196602028221,222.030882005113,3.64793988112538));
#88105=CARTESIAN_POINT('Ctrl Pts',(157.612220466518,223.224380974637,3.48918201589359));
#88106=CARTESIAN_POINT('Ctrl Pts',(157.213134639509,226.042926405927,3.33042415066179));
#88107=CARTESIAN_POINT('Ctrl Pts',(159.364587881769,227.9069856324,3.17166628543));
#88108=CARTESIAN_POINT('Ctrl Pts',(162.0975702677,227.110571720598,3.01290842019821));
#88109=CARTESIAN_POINT('Ctrl Pts',(162.910856431158,224.382562656872,2.85415055496641));
#88110=CARTESIAN_POINT('Ctrl Pts',(161.060126894903,222.219632217471,2.69539268973462));
#88111=CARTESIAN_POINT('Ctrl Pts',(158.239169283519,222.601294279545,2.53663482450283));
#88112=CARTESIAN_POINT('Ctrl Pts',(157.029723838513,225.178251688952,2.37787695927104));
#88113=CARTESIAN_POINT('Ctrl Pts',(158.538675094614,227.592073229572,2.21911909403925));
#88114=CARTESIAN_POINT('Ctrl Pts',(161.385030691198,227.6336293073,2.06036122880745));
#88115=CARTESIAN_POINT('Ctrl Pts',(162.963806576262,225.26488824769,1.90160336357566));
#88116=CARTESIAN_POINT('Ctrl Pts',(161.830106129847,222.653720849312,1.74284549834387));
#88117=CARTESIAN_POINT('Ctrl Pts',(159.02149401452,222.189869334119,1.58408763311208));
#88118=CARTESIAN_POINT('Ctrl Pts',(157.108407655953,224.297846602939,1.42532976788028));
#88119=CARTESIAN_POINT('Ctrl Pts',(157.841712478851,227.048440217077,1.26657190264849));
#88120=CARTESIAN_POINT('Ctrl Pts',(160.550269543046,227.924289837736,1.1078140374167));
#88121=CARTESIAN_POINT('Ctrl Pts',(162.755245701977,226.123853559107,0.949056172184904));
#88122=CARTESIAN_POINT('Ctrl Pts',(162.438567649914,223.29481665065,0.790298306953114));
#88123=CARTESIAN_POINT('Ctrl Pts',(159.890223501773,222.026467019093,0.631540441721318));
#88124=CARTESIAN_POINT('Ctrl Pts',(157.442116623435,223.479279799228,0.472782576489526));
#88125=CARTESIAN_POINT('Ctrl Pts',(157.335462140697,226.324301623048,0.314024711257735));
#88126=CARTESIAN_POINT('Ctrl Pts',(159.666401142308,227.95639832968,0.15526684602594));
#88127=CARTESIAN_POINT('Ctrl Pts',(162.304705497016,226.88473886389,-0.00349101920584817));
#88128=CARTESIAN_POINT('Ctrl Pts',(162.829415771032,224.084271948927,-0.162248884437644));
#88129=CARTESIAN_POINT('Ctrl Pts',(161.458872983031,222.784105799646,-0.268087461258838));
#88130=CARTESIAN_POINT('Ctrl Pts',(160.650199997975,222.567913197965,-0.321006749669435));
#88131=CARTESIAN_POINT('Ctrl Pts',(162.054331550342,226.756425321227,20.1070022498898));
#88132=CARTESIAN_POINT('Ctrl Pts',(162.638345947507,226.073356597808,20.0540829614792));
#88133=CARTESIAN_POINT('Ctrl Pts',(163.060276652233,224.089523335983,19.948244384658));
#88134=CARTESIAN_POINT('Ctrl Pts',(160.892947386112,221.93085054106,19.7894865194262));
#88135=CARTESIAN_POINT('Ctrl Pts',(157.906932102218,222.587140818593,19.6307286541944));
#88136=CARTESIAN_POINT('Ctrl Pts',(156.837131823488,225.448713592338,19.4719707889627));
#88137=CARTESIAN_POINT('Ctrl Pts',(158.661673281008,227.901044466763,19.3132129237308));
#88138=CARTESIAN_POINT('Ctrl Pts',(161.711202675617,227.697654506284,19.1544550584991));
#88139=CARTESIAN_POINT('Ctrl Pts',(163.194566457491,225.025701325879,18.9956971932673));
#88140=CARTESIAN_POINT('Ctrl Pts',(161.754298314344,222.33006722572,18.8369393280355));
#88141=CARTESIAN_POINT('Ctrl Pts',(158.708479473629,222.07803214969,18.6781814628037));
#88142=CARTESIAN_POINT('Ctrl Pts',(156.844668335675,224.500144995801,18.5194235975719));
#88143=CARTESIAN_POINT('Ctrl Pts',(157.868612676768,227.379742923236,18.3606657323401));
#88144=CARTESIAN_POINT('Ctrl Pts',(160.843204509053,228.081391642555,18.2019078671083));
#88145=CARTESIAN_POINT('Ctrl Pts',(163.046094693752,225.96295498568,18.0431500018765));
#88146=CARTESIAN_POINT('Ctrl Pts',(162.461199574998,222.963219971656,17.8843921366447));
#88147=CARTESIAN_POINT('Ctrl Pts',(159.623814489722,221.82754691948,17.7256342714129));
#88148=CARTESIAN_POINT('Ctrl Pts',(157.130714470951,223.595302339218,17.5668764061811));
#88149=CARTESIAN_POINT('Ctrl Pts',(157.26358440624,226.648637225804,17.4081185409493));
#88150=CARTESIAN_POINT('Ctrl Pts',(159.900821809086,228.193139280731,17.2493606757175));
#88151=CARTESIAN_POINT('Ctrl Pts',(162.628827076909,226.815280443273,17.0906028104858));
#88152=CARTESIAN_POINT('Ctrl Pts',(162.950929912838,223.776076990567,16.9318449452539));
#88153=CARTESIAN_POINT('Ctrl Pts',(160.572341805922,221.857007839987,16.7730870800222));
#88154=CARTESIAN_POINT('Ctrl Pts',(157.669946502014,222.814404984862,16.6143292147904));
#88155=CARTESIAN_POINT('Ctrl Pts',(156.900016067218,225.772058604437,16.4555713495586));
#88156=CARTESIAN_POINT('Ctrl Pts',(158.967190806099,228.023124218246,16.2968134843268));
#88157=CARTESIAN_POINT('Ctrl Pts',(161.97959247848,227.507426667046,16.138055619095));
#88158=CARTESIAN_POINT('Ctrl Pts',(163.180271192471,224.696932328455,15.9792977538632));
#88159=CARTESIAN_POINT('Ctrl Pts',(161.470365836141,222.163805511095,15.8205398886314));
#88160=CARTESIAN_POINT('Ctrl Pts',(158.414781724411,222.226363778377,15.6617820233996));
#88161=CARTESIAN_POINT('Ctrl Pts',(156.809989316156,224.827353806653,15.5030241581678));
#88162=CARTESIAN_POINT('Ctrl Pts',(158.124694560314,227.586349624274,15.344266292936));
#88163=CARTESIAN_POINT('Ctrl Pts',(161.155679269127,227.978318367473,15.1855084277042));
#88164=CARTESIAN_POINT('Ctrl Pts',(163.128986356281,225.644530257876,15.0267505624725));
#88165=CARTESIAN_POINT('Ctrl Pts',(162.238645253212,222.720868081619,14.8679926972407));
#88166=CARTESIAN_POINT('Ctrl Pts',(159.299496102435,221.883067347437,14.7092348320089));
#88167=CARTESIAN_POINT('Ctrl Pts',(157.001448091164,223.897883254312,14.5504769667771));
#88168=CARTESIAN_POINT('Ctrl Pts',(157.447674668944,226.9213563635,14.3917191015453));
#88169=CARTESIAN_POINT('Ctrl Pts',(160.229789289339,228.186404204368,14.2329612363135));
#88170=CARTESIAN_POINT('Ctrl Pts',(162.801600761167,226.535255042701,14.0742033710817));
#88171=CARTESIAN_POINT('Ctrl Pts',(162.809387326546,223.479040526326,13.9154455058499));
#88172=CARTESIAN_POINT('Ctrl Pts',(160.246022721146,221.814808060447,13.7566876406181));
#88173=CARTESIAN_POINT('Ctrl Pts',(157.457498131028,223.065663132392,13.5979297753863));
#88174=CARTESIAN_POINT('Ctrl Pts',(156.995871151412,226.086823229506,13.4391719101545));
#88175=CARTESIAN_POINT('Ctrl Pts',(159.283622775889,228.113322749714,13.2804140449227));
#88176=CARTESIAN_POINT('Ctrl Pts',(162.227002807702,227.290509411812,13.1216561796909));
#88177=CARTESIAN_POINT('Ctrl Pts',(163.132229957481,224.371421950292,12.9628983144592));
#88178=CARTESIAN_POINT('Ctrl Pts',(161.170840373345,222.027609095146,12.8041404492274));
#88179=CARTESIAN_POINT('Ctrl Pts',(158.137897725566,222.404128279236,12.6453825839956));
#88180=CARTESIAN_POINT('Ctrl Pts',(156.809151006124,225.156389160089,12.4866247187638));
#88181=CARTESIAN_POINT('Ctrl Pts',(158.4006691604,227.765522687778,12.327866853532));
#88182=CARTESIAN_POINT('Ctrl Pts',(161.455894836186,227.843649960364,12.1691089883002));
#88183=CARTESIAN_POINT('Ctrl Pts',(163.178685615146,225.319268901049,12.0103511230684));
#88184=CARTESIAN_POINT('Ctrl Pts',(161.992343444123,222.502692956048,11.8515932578366));
#88185=CARTESIAN_POINT('Ctrl Pts',(158.982608631386,221.971652319468,11.6928353926048));
#88186=CARTESIAN_POINT('Ctrl Pts',(156.903990359196,224.212155361024,11.534077527373));
#88187=CARTESIAN_POINT('Ctrl Pts',(157.658839988522,227.173693785189,11.3753196621412));
#88188=CARTESIAN_POINT('Ctrl Pts',(160.556319168289,228.145867742628,11.2165617969094));
#88189=CARTESIAN_POINT('Ctrl Pts',(162.944655067114,226.238943665722,11.0578039316776));
#88190=CARTESIAN_POINT('Ctrl Pts',(162.638042764312,223.198138394667,10.8990460664458));
#88191=CARTESIAN_POINT('Ctrl Pts',(159.917093827351,221.806396793957,10.740288201214));
#88192=CARTESIAN_POINT('Ctrl Pts',(157.272020616337,223.337440721832,10.5815303359823));
#88193=CARTESIAN_POINT('Ctrl Pts',(157.123594029977,226.390058835707,10.4227724707505));
#88194=CARTESIAN_POINT('Ctrl Pts',(159.60765407427,228.170495157807,10.2640146055187));
#88195=CARTESIAN_POINT('Ctrl Pts',(162.450789094363,227.049294436158,10.1052567402869));
#88196=CARTESIAN_POINT('Ctrl Pts',(163.050962031669,224.052579527124,9.94649887505509));
#88197=CARTESIAN_POINT('Ctrl Pts',(160.858894637569,221.92294379761,9.78774100982331));
#88198=CARTESIAN_POINT('Ctrl Pts',(157.88076690494,222.609429783521,9.62898314459151));
#88199=CARTESIAN_POINT('Ctrl Pts',(156.842161217574,225.483765537547,9.47022527935972));
#88200=CARTESIAN_POINT('Ctrl Pts',(158.693609459705,227.915359090634,9.31146741412792));
#88201=CARTESIAN_POINT('Ctrl Pts',(161.740666272941,227.678816118616,9.15270954889613));
#88202=CARTESIAN_POINT('Ctrl Pts',(163.194665381632,224.990620740183,8.99395168366434));
#88203=CARTESIAN_POINT('Ctrl Pts',(161.72490685868,222.311009259966,8.83519381843255));
#88204=CARTESIAN_POINT('Ctrl Pts',(158.676513646495,222.092361999286,8.67643595320076));
#88205=CARTESIAN_POINT('Ctrl Pts',(156.839375092992,224.534784922519,8.51767808796896));
#88206=CARTESIAN_POINT('Ctrl Pts',(157.894840330095,227.402972666369,8.35892022273717));
#88207=CARTESIAN_POINT('Ctrl Pts',(160.876947614311,228.071959920453,8.20016235750538));
#88208=CARTESIAN_POINT('Ctrl Pts',(163.056472476395,225.92948957614,8.04140449227359));
#88209=CARTESIAN_POINT('Ctrl Pts',(162.438713848275,222.936350408295,7.88264662704179));
#88210=CARTESIAN_POINT('Ctrl Pts',(159.589044402114,221.831863265628,7.72388876181));
#88211=CARTESIAN_POINT('Ctrl Pts',(157.115481502978,223.626854737674,7.56513089657821));
#88212=CARTESIAN_POINT('Ctrl Pts',(157.281829818885,226.678548699803,7.40637303134641));
#88213=CARTESIAN_POINT('Ctrl Pts',(159.93584737766,228.19403495788,7.24761516611462));
#88214=CARTESIAN_POINT('Ctrl Pts',(162.648577413877,226.786340548107,7.08885730088283));
#88215=CARTESIAN_POINT('Ctrl Pts',(162.937329505067,223.743787338953,6.93009943565104));
#88216=CARTESIAN_POINT('Ctrl Pts',(160.537837748727,221.85091990779,6.77134157041924));
#88217=CARTESIAN_POINT('Ctrl Pts',(157.646116905902,222.840090453183,6.61258370518745));
#88218=CARTESIAN_POINT('Ctrl Pts',(156.908669778231,225.806010130887,6.45382583995566));
#88219=CARTESIAN_POINT('Ctrl Pts',(159.000407947959,228.034269368499,6.29506797472387));
#88220=CARTESIAN_POINT('Ctrl Pts',(162.006972724407,227.485565399381,6.13631010949207));
#88221=CARTESIAN_POINT('Ctrl Pts',(163.1767561424,224.662072074492,5.97755224426028));
#88222=CARTESIAN_POINT('Ctrl Pts',(161.439172463791,222.147850373739,5.81879437902849));
#88223=CARTESIAN_POINT('Ctrl Pts',(158.384458202915,222.243915898783,5.6600365137967));
#88224=CARTESIAN_POINT('Ctrl Pts',(156.808287731201,224.86234948488,5.50127864856491));
#88225=CARTESIAN_POINT('Ctrl Pts',(158.153172202382,227.606760817002,5.34252078333311));
#88226=CARTESIAN_POINT('Ctrl Pts',(161.188273401317,227.965464751912,5.18376291810132));
#88227=CARTESIAN_POINT('Ctrl Pts',(163.135866830095,225.610175462486,5.02500505286953));
#88228=CARTESIAN_POINT('Ctrl Pts',(162.213515059285,222.696453613788,4.86624718763774));
#88229=CARTESIAN_POINT('Ctrl Pts',(159.265354393261,221.890937327165,4.70748932240594));
#88230=CARTESIAN_POINT('Ctrl Pts',(156.989541357638,223.930835076462,4.54873145717415));
#88231=CARTESIAN_POINT('Ctrl Pts',(157.468899953115,226.949232521731,4.38997359194236));
#88232=CARTESIAN_POINT('Ctrl Pts',(160.264721211981,228.183692439776,4.23121572671057));
#88233=CARTESIAN_POINT('Ctrl Pts',(162.818269628026,226.504437162108,4.07245786147877));
#88234=CARTESIAN_POINT('Ctrl Pts',(162.792537791381,223.448321052891,3.91369999624698));
#88235=CARTESIAN_POINT('Ctrl Pts',(160.211075477766,221.812301454944,3.75494213101519));
#88236=CARTESIAN_POINT('Ctrl Pts',(157.436436895433,223.093663440297,3.5961842657834));
#88237=CARTESIAN_POINT('Ctrl Pts',(157.007971165105,226.119704569673,3.4374264005516));
#88238=CARTESIAN_POINT('Ctrl Pts',(159.317810107821,228.120992121855,3.27866853531981));
#88239=CARTESIAN_POINT('Ctrl Pts',(162.251989210943,227.265947804894,3.11991067008802));
#88240=CARTESIAN_POINT('Ctrl Pts',(163.125147881105,224.33710815005,2.96115280485623));
#88241=CARTESIAN_POINT('Ctrl Pts',(161.138171324371,222.014947081809,2.80239493962443));
#88242=CARTESIAN_POINT('Ctrl Pts',(158.10954043501,222.424706344349,2.64363707439264));
#88243=CARTESIAN_POINT('Ctrl Pts',(156.811058026427,225.191374223088,2.48487920916085));
#88244=CARTESIAN_POINT('Ctrl Pts',(158.431095267087,227.782896495463,2.32612134392906));
#88245=CARTESIAN_POINT('Ctrl Pts',(161.486993890709,227.827511848824,2.16736347869726));
#88246=CARTESIAN_POINT('Ctrl Pts',(163.181996110377,225.284388792637,2.00860561346547));
#88247=CARTESIAN_POINT('Ctrl Pts',(161.964834896241,222.480992453711,1.84984774823368));
#88248=CARTESIAN_POINT('Ctrl Pts',(158.949458353755,221.982993114294,1.69108988300189));
#88249=CARTESIAN_POINT('Ctrl Pts',(156.895534389711,224.246155469041,1.53233201777009));
#88250=CARTESIAN_POINT('Ctrl Pts',(157.682823652402,227.199242303896,1.3735741525383));
#88251=CARTESIAN_POINT('Ctrl Pts',(160.590779290273,228.139570228306,1.21481628730651));
#88252=CARTESIAN_POINT('Ctrl Pts',(162.95808140013,226.206589418606,1.05605842207471));
#88253=CARTESIAN_POINT('Ctrl Pts',(162.618090140923,223.169284450419,0.897300556842924));
#88254=CARTESIAN_POINT('Ctrl Pts',(159.882141974727,221.80756144645,0.738542691611128));
#88255=CARTESIAN_POINT('Ctrl Pts',(157.253810346392,223.367327408414,0.579784826379337));
#88256=CARTESIAN_POINT('Ctrl Pts',(157.139304173167,226.421794069577,0.421026961147545));
#88257=CARTESIAN_POINT('Ctrl Pts',(159.641842259173,228.174042483444,0.26226909591575));
#88258=CARTESIAN_POINT('Ctrl Pts',(162.474373323079,227.023489583297,0.103511230683962));
#88259=CARTESIAN_POINT('Ctrl Pts',(163.037711721868,224.016857874595,-0.0552466345478338));
#88260=CARTESIAN_POINT('Ctrl Pts',(161.56627230492,222.620976084267,-0.161085211369028));
#88261=CARTESIAN_POINT('Ctrl Pts',(160.698066426161,222.388867814061,-0.214004499779625));
#88262=CARTESIAN_POINT('Ctrl Pts',(162.195197104019,226.876863439079,20.2140044997796));
#88263=CARTESIAN_POINT('Ctrl Pts',(162.819257379562,226.146956680238,20.161085211369));
#88264=CARTESIAN_POINT('Ctrl Pts',(163.270119880776,224.027091933727,20.0552466345478));
#88265=CARTESIAN_POINT('Ctrl Pts',(160.954176805447,221.720398903991,19.8964887693161));
#88266=CARTESIAN_POINT('Ctrl Pts',(157.763410396457,222.4216910184,19.7377309040842));
#88267=CARTESIAN_POINT('Ctrl Pts',(156.620253892164,225.479481891942,19.5789730388525));
#88268=CARTESIAN_POINT('Ctrl Pts',(158.569904192303,228.099969141304,19.4202151736207));
#88269=CARTESIAN_POINT('Ctrl Pts',(161.828539875795,227.882632727348,19.2614573083889));
#88270=CARTESIAN_POINT('Ctrl Pts',(163.413617940547,225.027463666286,19.1026994431571));
#88271=CARTESIAN_POINT('Ctrl Pts',(161.874590583293,222.146989884349,18.9439415779253));
#88272=CARTESIAN_POINT('Ctrl Pts',(158.619919886447,221.877672758339,18.7851837126935));
#88273=CARTESIAN_POINT('Ctrl Pts',(156.628307183136,224.465869928608,18.6264258474617));
#88274=CARTESIAN_POINT('Ctrl Pts',(157.722463407271,227.542921940972,18.4676679822299));
#88275=CARTESIAN_POINT('Ctrl Pts',(160.901023058357,228.292682726388,18.3089101169981));
#88276=CARTESIAN_POINT('Ctrl Pts',(163.254965465131,226.028984827456,18.1501522517663));
#88277=CARTESIAN_POINT('Ctrl Pts',(162.629964076903,222.823557926178,17.9913943865345));
#88278=CARTESIAN_POINT('Ctrl Pts',(159.598019442091,221.610011751104,17.8326365213027));
#88279=CARTESIAN_POINT('Ctrl Pts',(156.933967507375,223.498982193766,17.673878656071));
#88280=CARTESIAN_POINT('Ctrl Pts',(157.075948336667,226.761684311892,17.5151207908391));
#88281=CARTESIAN_POINT('Ctrl Pts',(159.894021158639,228.41209290225,17.3563629256074));
#88282=CARTESIAN_POINT('Ctrl Pts',(162.809085799825,226.939754257969,17.1976050603756));
#88283=CARTESIAN_POINT('Ctrl Pts',(163.15327523337,223.692152566413,17.0388471951438));
#88284=CARTESIAN_POINT('Ctrl Pts',(160.611587294494,221.641492807494,16.880089329912));
#88285=CARTESIAN_POINT('Ctrl Pts',(157.510174689116,222.664538692895,16.7213314646802));
#88286=CARTESIAN_POINT('Ctrl Pts',(156.687450109689,225.824998677702,16.5625735994484));
#88287=CARTESIAN_POINT('Ctrl Pts',(158.89637105993,228.230419903681,16.4038157342166));
#88288=CARTESIAN_POINT('Ctrl Pts',(162.11533317257,227.679360961537,16.2450578689848));
#88289=CARTESIAN_POINT('Ctrl Pts',(163.398342448932,224.676150972424,16.086300003753));
#88290=CARTESIAN_POINT('Ctrl Pts',(161.571188849632,221.969327600774,15.9275421385212));
#88291=CARTESIAN_POINT('Ctrl Pts',(158.306083276952,222.03617548964,15.7687842732894));
#88292=CARTESIAN_POINT('Ctrl Pts',(156.591250222585,224.815515453875,15.6100264080576));
#88293=CARTESIAN_POINT('Ctrl Pts',(157.996104830467,227.763695667451,15.4512685428258));
#88294=CARTESIAN_POINT('Ctrl Pts',(161.234924218702,228.182541714864,15.2925106775941));
#88295=CARTESIAN_POINT('Ctrl Pts',(163.343541010544,225.68872570998,15.1337528123623));
#88296=CARTESIAN_POINT('Ctrl Pts',(162.392149201018,222.564587962408,14.9749949471305));
#88297=CARTESIAN_POINT('Ctrl Pts',(159.251462536788,221.669339215869,14.8162370818987));
#88298=CARTESIAN_POINT('Ctrl Pts',(156.795837329455,223.822311087992,14.6574792166669));
#88299=CARTESIAN_POINT('Ctrl Pts',(157.272661672204,227.053103806073,14.4987213514351));
#88300=CARTESIAN_POINT('Ctrl Pts',(160.245545945302,228.404896001573,14.3399634862033));
#88301=CARTESIAN_POINT('Ctrl Pts',(162.993706578915,226.640527510327,14.1812056209715));
#88302=CARTESIAN_POINT('Ctrl Pts',(163.00202706923,223.374748306142,14.0224477557397));
#88303=CARTESIAN_POINT('Ctrl Pts',(160.262892503838,221.596399388265,13.8636898905079));
#88304=CARTESIAN_POINT('Ctrl Pts',(157.283158729271,222.933025616404,13.7049320252761));
#88305=CARTESIAN_POINT('Ctrl Pts',(156.789877978838,226.161346719129,13.5461741600443));
#88306=CARTESIAN_POINT('Ctrl Pts',(159.234500775938,228.326803350176,13.3874162948126));
#88307=CARTESIAN_POINT('Ctrl Pts',(162.379708432797,227.447569685965,13.2286584295807));
#88308=CARTESIAN_POINT('Ctrl Pts',(163.34700702554,224.328320341408,13.069900564349));
#88309=CARTESIAN_POINT('Ctrl Pts',(161.251124920127,221.823792193981,12.9111426991172));
#88310=CARTESIAN_POINT('Ctrl Pts',(158.010213337013,222.226129305721,12.7523848338854));
#88311=CARTESIAN_POINT('Ctrl Pts',(156.590354429619,225.167112767786,12.5936269686536));
#88312=CARTESIAN_POINT('Ctrl Pts',(158.291003014156,227.955154631344,12.4348691034218));
#88313=CARTESIAN_POINT('Ctrl Pts',(161.555725572934,228.038639092505,12.27611123819));
#88314=CARTESIAN_POINT('Ctrl Pts',(163.396648148539,225.341161175697,12.1173533729582));
#88315=CARTESIAN_POINT('Ctrl Pts',(162.128958472172,222.331452564307,11.9585955077264));
#88316=CARTESIAN_POINT('Ctrl Pts',(158.912846085792,221.763998461125,11.7998376424946));
#88317=CARTESIAN_POINT('Ctrl Pts',(156.691696918944,224.158132839069,11.6410797772628));
#88318=CARTESIAN_POINT('Ctrl Pts',(157.498306601782,227.322744009591,11.482321912031));
#88319=CARTESIAN_POINT('Ctrl Pts',(160.594465984293,228.361579953876,11.3235640467992));
#88320=CARTESIAN_POINT('Ctrl Pts',(163.146570121355,226.323898056563,11.1648061815674));
#88321=CARTESIAN_POINT('Ctrl Pts',(162.818933407089,223.074584709946,11.0060483163357));
#88322=CARTESIAN_POINT('Ctrl Pts',(159.911408949507,221.58741136107,10.8472904511039));
#88323=CARTESIAN_POINT('Ctrl Pts',(157.084963017852,223.223439000347,10.6885325858721));
#88324=CARTESIAN_POINT('Ctrl Pts',(156.926358817628,226.485375196644,10.5297747206403));
#88325=CARTESIAN_POINT('Ctrl Pts',(159.580750906643,228.387896071384,10.3710168554085));
#88326=CARTESIAN_POINT('Ctrl Pts',(162.618839749411,227.189814594819,10.2122589901767));
#88327=CARTESIAN_POINT('Ctrl Pts',(163.260166556502,223.987614887188,10.0535011249449));
#88328=CARTESIAN_POINT('Ctrl Pts',(160.917789059285,221.711949994992,9.89474325971312));
#88329=CARTESIAN_POINT('Ctrl Pts',(157.735451051101,222.445508338079,9.73598539448132));
#88330=CARTESIAN_POINT('Ctrl Pts',(156.625628151898,225.516937349704,9.57722752924952));
#88331=CARTESIAN_POINT('Ctrl Pts',(158.604030235384,228.115265319207,9.41846966401773));
#88332=CARTESIAN_POINT('Ctrl Pts',(161.860023792551,227.862502591077,9.25971179878595));
#88333=CARTESIAN_POINT('Ctrl Pts',(163.413723647919,224.989977604158,9.10095393355415));
#88334=CARTESIAN_POINT('Ctrl Pts',(161.843183754953,222.126625113519,8.94219606832236));
#88335=CARTESIAN_POINT('Ctrl Pts',(158.585762161935,221.892985205995,8.78343820309056));
#88336=CARTESIAN_POINT('Ctrl Pts',(156.622650982701,224.502885115764,8.62468033785877));
#88337=CARTESIAN_POINT('Ctrl Pts',(157.750489491288,227.567744548037,8.46592247262698));
#88338=CARTESIAN_POINT('Ctrl Pts',(160.937079928988,228.282604270921,8.30716460739519));
#88339=CARTESIAN_POINT('Ctrl Pts',(163.266054852528,225.993224694143,8.1484067421634));
#88340=CARTESIAN_POINT('Ctrl Pts',(162.605936503469,222.794845916344,7.9896488769316));
#88341=CARTESIAN_POINT('Ctrl Pts',(159.560865168911,221.614624069191,7.83089101169982));
#88342=CARTESIAN_POINT('Ctrl Pts',(156.917690014497,223.532698140788,7.67213314646801));
#88343=CARTESIAN_POINT('Ctrl Pts',(157.095444837606,226.793646816236,7.51337528123623));
#88344=CARTESIAN_POINT('Ctrl Pts',(159.93144843112,228.413049995998,7.35461741600443));
#88345=CARTESIAN_POINT('Ctrl Pts',(162.830190417776,226.908829953638,7.19585955077264));
#88346=CARTESIAN_POINT('Ctrl Pts',(163.138742245379,223.657648812771,7.03710168554085));
#88347=CARTESIAN_POINT('Ctrl Pts',(160.574717293439,221.63498742567,6.87834382030906));
#88348=CARTESIAN_POINT('Ctrl Pts',(157.484711097144,222.691985414269,6.71958595507726));
#88349=CARTESIAN_POINT('Ctrl Pts',(156.696697205832,225.861278260969,6.56082808984547));
#88350=CARTESIAN_POINT('Ctrl Pts',(158.931865901843,228.242329277099,6.40207022461368));
#88351=CARTESIAN_POINT('Ctrl Pts',(162.144590882485,227.65600066633,6.24331235938188));
#88352=CARTESIAN_POINT('Ctrl Pts',(163.39458637181,224.63890035018,6.08455449415009));
#88353=CARTESIAN_POINT('Ctrl Pts',(161.537856547144,221.952278419346,5.92579662891829));
#88354=CARTESIAN_POINT('Ctrl Pts',(158.273680471006,222.054931159278,5.76703876368651));
#88355=CARTESIAN_POINT('Ctrl Pts',(156.589431959918,224.852910786426,5.60828089845471));
#88356=CARTESIAN_POINT('Ctrl Pts',(158.026535184995,227.785506456054,5.44952303322292));
#88357=CARTESIAN_POINT('Ctrl Pts',(161.269753331161,228.168806726638,5.29076516799113));
#88358=CARTESIAN_POINT('Ctrl Pts',(163.350893278579,225.652015205613,5.13200730275933));
#88359=CARTESIAN_POINT('Ctrl Pts',(162.365295829214,222.538499394052,4.97324943752755));
#88360=CARTESIAN_POINT('Ctrl Pts',(159.214979729963,221.677748840256,4.81449157229575));
#88361=CARTESIAN_POINT('Ctrl Pts',(156.783114150984,223.857522417217,4.65573370706396));
#88362=CARTESIAN_POINT('Ctrl Pts',(157.295342374516,227.082891433008,4.49697584183217));
#88363=CARTESIAN_POINT('Ctrl Pts',(160.282873150547,228.40199829123,4.33821797660038));
#88364=CARTESIAN_POINT('Ctrl Pts',(163.011518430293,226.607596447073,4.17946011136858));
#88365=CARTESIAN_POINT('Ctrl Pts',(162.984022161118,223.341922397826,4.02070224613679));
#88366=CARTESIAN_POINT('Ctrl Pts',(160.225548927311,221.593720904774,3.861944380905));
#88367=CARTESIAN_POINT('Ctrl Pts',(157.260653324349,222.962945905958,3.7031865156732));
#88368=CARTESIAN_POINT('Ctrl Pts',(156.802807690702,226.196482733419,3.54442865044142));
#88369=CARTESIAN_POINT('Ctrl Pts',(159.271032333874,228.334998611311,3.38567078520962));
#88370=CARTESIAN_POINT('Ctrl Pts',(162.406408154186,227.421323889191,3.22691291997783));
#88371=CARTESIAN_POINT('Ctrl Pts',(163.339439331051,224.291653643227,3.06815505474604));
#88372=CARTESIAN_POINT('Ctrl Pts',(161.216215753841,221.810261946147,2.90939718951424));
#88373=CARTESIAN_POINT('Ctrl Pts',(157.979911586501,222.248118409152,2.75063932428245));
#88374=CARTESIAN_POINT('Ctrl Pts',(156.59239221434,225.204496757223,2.59188145905066));
#88375=CARTESIAN_POINT('Ctrl Pts',(158.323515439561,227.973719761354,2.43312359381887));
#88376=CARTESIAN_POINT('Ctrl Pts',(161.58895709022,228.021394390348,2.27436572858707));
#88377=CARTESIAN_POINT('Ctrl Pts',(163.400185644492,225.303889337585,2.11560786335528));
#88378=CARTESIAN_POINT('Ctrl Pts',(162.099563662636,222.308264058109,1.95684999812349));
#88379=CARTESIAN_POINT('Ctrl Pts',(158.87742269299,221.776116894469,1.7980921328917));
#88380=CARTESIAN_POINT('Ctrl Pts',(156.682661123469,224.194464335143,1.6393342676599));
#88381=CARTESIAN_POINT('Ctrl Pts',(157.523934825953,227.350044390714,1.48057640242811));
#88382=CARTESIAN_POINT('Ctrl Pts',(160.6312890375,228.354850618877,1.32181853719632));
#88383=CARTESIAN_POINT('Ctrl Pts',(163.160917098283,226.289325278104,1.16306067196453));
#88384=CARTESIAN_POINT('Ctrl Pts',(162.797612631933,223.043752250189,1.00430280673273));
#88385=CARTESIAN_POINT('Ctrl Pts',(159.874060447681,221.588655873807,0.845544941500939));
#88386=CARTESIAN_POINT('Ctrl Pts',(157.065504069348,223.255375017599,0.686787076269146));
#88387=CARTESIAN_POINT('Ctrl Pts',(156.943146205637,226.519286516107,0.528029211037356));
#88388=CARTESIAN_POINT('Ctrl Pts',(159.617283376038,228.391686637208,0.36927134580556));
#88389=CARTESIAN_POINT('Ctrl Pts',(162.644041149142,227.162240302705,0.210513480573772));
#88390=CARTESIAN_POINT('Ctrl Pts',(163.246007672705,223.949443800262,0.0517556153419762));
#88391=CARTESIAN_POINT('Ctrl Pts',(161.673671626809,222.457846368889,-0.0540829614792177));
#88392=CARTESIAN_POINT('Ctrl Pts',(160.745932854347,222.209822430158,-0.107002249889815));
#88393=CARTESIAN_POINT('Ctrl Pts',(162.336062657696,226.997301556931,20.3210067496694));
#88394=CARTESIAN_POINT('Ctrl Pts',(163.000168811616,226.220556762668,20.2680874612588));
#88395=CARTESIAN_POINT('Ctrl Pts',(163.479963109319,223.96466053147,20.1622488844376));
#88396=CARTESIAN_POINT('Ctrl Pts',(161.015406224782,221.509947266923,20.0034910192059));
#88397=CARTESIAN_POINT('Ctrl Pts',(157.619888690695,222.256241218208,19.844733153974));
#88398=CARTESIAN_POINT('Ctrl Pts',(156.40337596084,225.510250191546,19.6859752887423));
#88399=CARTESIAN_POINT('Ctrl Pts',(158.478135103599,228.298893815846,19.5272174235105));
#88400=CARTESIAN_POINT('Ctrl Pts',(161.945877075973,228.067610948411,19.3684595582787));
#88401=CARTESIAN_POINT('Ctrl Pts',(163.632669423604,225.029226006693,19.2097016930469));
#88402=CARTESIAN_POINT('Ctrl Pts',(161.994882852242,221.963912542979,19.0509438278151));
#88403=CARTESIAN_POINT('Ctrl Pts',(158.531360299265,221.677313366987,18.8921859625833));
#88404=CARTESIAN_POINT('Ctrl Pts',(156.411946030597,224.431594861414,18.7334280973515));
#88405=CARTESIAN_POINT('Ctrl Pts',(157.576314137774,227.706100958709,18.5746702321197));
#88406=CARTESIAN_POINT('Ctrl Pts',(160.958841607661,228.503973810221,18.4159123668879));
#88407=CARTESIAN_POINT('Ctrl Pts',(163.46383623651,226.095014669232,18.2571545016561));
#88408=CARTESIAN_POINT('Ctrl Pts',(162.798728578809,222.6838958807,18.0983966364243));
#88409=CARTESIAN_POINT('Ctrl Pts',(159.57222439446,221.39247658273,17.9396387711925));
#88410=CARTESIAN_POINT('Ctrl Pts',(156.7372205438,223.402662048314,17.7808809059608));
#88411=CARTESIAN_POINT('Ctrl Pts',(156.888312267094,226.87473139798,17.622123040729));
#88412=CARTESIAN_POINT('Ctrl Pts',(159.887220508192,228.631046523769,17.4633651754972));
#88413=CARTESIAN_POINT('Ctrl Pts',(162.98934452274,227.064228072664,17.3046073102654));
#88414=CARTESIAN_POINT('Ctrl Pts',(163.355620553903,223.60822814226,17.1458494450336));
#88415=CARTESIAN_POINT('Ctrl Pts',(160.650832783067,221.425977775001,16.9870915798018));
#88416=CARTESIAN_POINT('Ctrl Pts',(157.350402876218,222.514672400928,16.82833371457));
#88417=CARTESIAN_POINT('Ctrl Pts',(156.47488415216,225.877938750967,16.6695758493382));
#88418=CARTESIAN_POINT('Ctrl Pts',(158.825551313761,228.437715589115,16.5108179841064));
#88419=CARTESIAN_POINT('Ctrl Pts',(162.251073866661,227.851295256028,16.3520601188746));
#88420=CARTESIAN_POINT('Ctrl Pts',(163.616413705393,224.655369616393,16.1933022536428));
#88421=CARTESIAN_POINT('Ctrl Pts',(161.672011863123,221.774849690454,16.034544388411));
#88422=CARTESIAN_POINT('Ctrl Pts',(158.197384829492,221.845987200903,15.8757865231793));
#88423=CARTESIAN_POINT('Ctrl Pts',(156.372511129014,224.803677101097,15.7170286579474));
#88424=CARTESIAN_POINT('Ctrl Pts',(157.86751510062,227.941041710627,15.5582707927157));
#88425=CARTESIAN_POINT('Ctrl Pts',(161.314169168278,228.386765062254,15.3995129274839));
#88426=CARTESIAN_POINT('Ctrl Pts',(163.558095664808,225.732921162083,15.2407550622521));
#88427=CARTESIAN_POINT('Ctrl Pts',(162.545653148823,222.408307843197,15.0819971970203));
#88428=CARTESIAN_POINT('Ctrl Pts',(159.203428971142,221.4556110843,14.9232393317885));
#88429=CARTESIAN_POINT('Ctrl Pts',(156.590226567747,223.746738921673,14.7644814665567));
#88430=CARTESIAN_POINT('Ctrl Pts',(157.097648675464,227.184851248647,14.6057236013249));
#88431=CARTESIAN_POINT('Ctrl Pts',(160.261302601264,228.623387798777,14.4469657360931));
#88432=CARTESIAN_POINT('Ctrl Pts',(163.185812396663,226.745799977952,14.2882078708613));
#88433=CARTESIAN_POINT('Ctrl Pts',(163.194666811915,223.270456085958,14.1294500056295));
#88434=CARTESIAN_POINT('Ctrl Pts',(160.27976228653,221.377990716082,13.9706921403978));
#88435=CARTESIAN_POINT('Ctrl Pts',(157.108819327513,222.800388100416,13.8119342751659));
#88436=CARTESIAN_POINT('Ctrl Pts',(156.583884806264,226.235870208751,13.6531764099342));
#88437=CARTESIAN_POINT('Ctrl Pts',(159.185378775986,228.540283950637,13.4944185447024));
#88438=CARTESIAN_POINT('Ctrl Pts',(162.532414057892,227.604629960118,13.3356606794706));
#88439=CARTESIAN_POINT('Ctrl Pts',(163.561784093599,224.285218732523,13.1769028142388));
#88440=CARTESIAN_POINT('Ctrl Pts',(161.331409466909,221.619975292816,13.018144949007));
#88441=CARTESIAN_POINT('Ctrl Pts',(157.882528948459,222.048130332206,12.8593870837752));
#88442=CARTESIAN_POINT('Ctrl Pts',(156.371557853113,225.177836375483,12.7006292185434));
#88443=CARTESIAN_POINT('Ctrl Pts',(158.181336867912,228.14478657491,12.5418713533116));
#88444=CARTESIAN_POINT('Ctrl Pts',(161.655556309681,228.233628224646,12.3831134880798));
#88445=CARTESIAN_POINT('Ctrl Pts',(163.614610681933,225.363053450345,12.224355622848));
#88446=CARTESIAN_POINT('Ctrl Pts',(162.265573500221,222.160212172565,12.0655977576162));
#88447=CARTESIAN_POINT('Ctrl Pts',(158.843083540198,221.556344602782,11.9068398923844));
#88448=CARTESIAN_POINT('Ctrl Pts',(156.479403478692,224.104110317114,11.7480820271526));
#88449=CARTESIAN_POINT('Ctrl Pts',(157.337773215042,227.471794233994,11.5893241619208));
#88450=CARTESIAN_POINT('Ctrl Pts',(160.632612800297,228.577292165123,11.4305662966891));
#88451=CARTESIAN_POINT('Ctrl Pts',(163.348485175597,226.408852447405,11.2718084314573));
#88452=CARTESIAN_POINT('Ctrl Pts',(162.999824049866,222.951031025224,11.1130505662255));
#88453=CARTESIAN_POINT('Ctrl Pts',(159.905724071664,221.368425928184,10.9542927009937));
#88454=CARTESIAN_POINT('Ctrl Pts',(156.897905419367,223.109437278862,10.7955348357619));
#88455=CARTESIAN_POINT('Ctrl Pts',(156.729123605279,226.580691557581,10.6367769705301));
#88456=CARTESIAN_POINT('Ctrl Pts',(159.553847739015,228.605296984961,10.4780191052983));
#88457=CARTESIAN_POINT('Ctrl Pts',(162.786890404461,227.33033475348,10.3192612400665));
#88458=CARTESIAN_POINT('Ctrl Pts',(163.469371081335,223.922650247252,10.1605033748347));
#88459=CARTESIAN_POINT('Ctrl Pts',(160.976683481002,221.500956192374,10.0017455096029));
#88460=CARTESIAN_POINT('Ctrl Pts',(157.590135197262,222.281586892638,9.84298764437113));
#88461=CARTESIAN_POINT('Ctrl Pts',(156.409095086223,225.550109161861,9.68422977913934));
#88462=CARTESIAN_POINT('Ctrl Pts',(158.514451011063,228.315171547782,9.52547191390754));
#88463=CARTESIAN_POINT('Ctrl Pts',(161.979381312161,228.046189063538,9.36671404867575));
#88464=CARTESIAN_POINT('Ctrl Pts',(163.632781914206,224.989334468133,9.20795618344396));
#88465=CARTESIAN_POINT('Ctrl Pts',(161.961460651225,221.942240967073,9.04919831821217));
#88466=CARTESIAN_POINT('Ctrl Pts',(158.495010677376,221.693608412704,8.89044045298037));
#88467=CARTESIAN_POINT('Ctrl Pts',(156.40592687241,224.470985309008,8.73168258774858));
#88468=CARTESIAN_POINT('Ctrl Pts',(157.606138652481,227.732516429704,8.57292472251679));
#88469=CARTESIAN_POINT('Ctrl Pts',(160.997212243665,228.493248621389,8.414166857285));
#88470=CARTESIAN_POINT('Ctrl Pts',(163.475637228661,226.056959812147,8.2554089920532));
#88471=CARTESIAN_POINT('Ctrl Pts',(162.773159158663,222.653341424392,8.09665112682142));
#88472=CARTESIAN_POINT('Ctrl Pts',(159.532685935708,221.397384872754,7.93789326158962));
#88473=CARTESIAN_POINT('Ctrl Pts',(156.719898526016,223.438541543901,7.77913539635783));
#88474=CARTESIAN_POINT('Ctrl Pts',(156.909059856328,226.908744932668,7.62037753112604));
#88475=CARTESIAN_POINT('Ctrl Pts',(159.927049484579,228.632065034116,7.46161966589424));
#88476=CARTESIAN_POINT('Ctrl Pts',(163.011803421676,227.031319359169,7.30286180066245));
#88477=CARTESIAN_POINT('Ctrl Pts',(163.34015498569,223.57151028659,7.14410393543066));
#88478=CARTESIAN_POINT('Ctrl Pts',(160.61159683815,221.41905494355,6.98534607019886));
#88479=CARTESIAN_POINT('Ctrl Pts',(157.323305288385,222.543880375355,6.82658820496707));
#88480=CARTESIAN_POINT('Ctrl Pts',(156.484724633432,225.916546391051,6.66783033973528));
#88481=CARTESIAN_POINT('Ctrl Pts',(158.863323855727,228.450389185699,6.50907247450349));
#88482=CARTESIAN_POINT('Ctrl Pts',(162.282209040562,227.826435933279,6.35031460927169));
#88483=CARTESIAN_POINT('Ctrl Pts',(163.612416601221,224.615728625868,6.1915567440399));
#88484=CARTESIAN_POINT('Ctrl Pts',(161.636540630497,221.756706464952,6.03279887880811));
#88485=CARTESIAN_POINT('Ctrl Pts',(158.162902739098,221.865946419773,5.87404101357632));
#88486=CARTESIAN_POINT('Ctrl Pts',(156.370576188634,224.843472087974,5.71528314834453));
#88487=CARTESIAN_POINT('Ctrl Pts',(157.899898167609,227.964252095106,5.55652528311273));
#88488=CARTESIAN_POINT('Ctrl Pts',(161.351233261004,228.372148701364,5.39776741788094));
#88489=CARTESIAN_POINT('Ctrl Pts',(163.565919727063,225.69385494874,5.23900955264914));
#88490=CARTESIAN_POINT('Ctrl Pts',(162.517076599142,222.380545174315,5.08025168741736));
#88491=CARTESIAN_POINT('Ctrl Pts',(159.164605066666,221.464560353348,4.92149382218556));
#88492=CARTESIAN_POINT('Ctrl Pts',(156.57668694433,223.784209757972,4.76273595695378));
#88493=CARTESIAN_POINT('Ctrl Pts',(157.121784795917,227.216550344284,4.60397809172198));
#88494=CARTESIAN_POINT('Ctrl Pts',(160.301025089113,228.620304142684,4.44522022649019));
#88495=CARTESIAN_POINT('Ctrl Pts',(163.20476723256,226.710755732037,4.28646236125839));
#88496=CARTESIAN_POINT('Ctrl Pts',(163.175506530854,223.235523742761,4.1277044960266));
#88497=CARTESIAN_POINT('Ctrl Pts',(160.240022376856,221.375140354604,3.96894663079481));
#88498=CARTESIAN_POINT('Ctrl Pts',(157.084869753264,222.832228371618,3.81018876556302));
#88499=CARTESIAN_POINT('Ctrl Pts',(156.597644216298,226.273260897166,3.65143090033123));
#88500=CARTESIAN_POINT('Ctrl Pts',(159.224254559927,228.549005100767,3.49267303509943));
#88501=CARTESIAN_POINT('Ctrl Pts',(162.560827097429,227.576699973488,3.33391516986764));
#88502=CARTESIAN_POINT('Ctrl Pts',(163.553730780998,224.246199136404,3.17515730463585));
#88503=CARTESIAN_POINT('Ctrl Pts',(161.29426018331,221.605576810485,3.01639943940405));
#88504=CARTESIAN_POINT('Ctrl Pts',(157.850282737992,222.071530473955,2.85764157417226));
#88505=CARTESIAN_POINT('Ctrl Pts',(156.373726402253,225.217619291359,2.69888370894047));
#88506=CARTESIAN_POINT('Ctrl Pts',(158.215935612034,228.164543027245,2.54012584370868));
#88507=CARTESIAN_POINT('Ctrl Pts',(161.69092028973,228.215276931872,2.38136797847688));
#88508=CARTESIAN_POINT('Ctrl Pts',(163.618375178607,225.323389882532,2.22261011324509));
#88509=CARTESIAN_POINT('Ctrl Pts',(162.23429242903,222.135535662507,2.0638522480133));
#88510=CARTESIAN_POINT('Ctrl Pts',(158.805387032225,221.569240674643,1.90509438278151));
#88511=CARTESIAN_POINT('Ctrl Pts',(156.469787857227,224.142773201245,1.74633651754971));
#88512=CARTESIAN_POINT('Ctrl Pts',(157.365045999503,227.500846477532,1.58757865231792));
#88513=CARTESIAN_POINT('Ctrl Pts',(160.671798784727,228.570131009447,1.42882078708613));
#88514=CARTESIAN_POINT('Ctrl Pts',(163.363752796435,226.372061137603,1.27006292185433));
#88515=CARTESIAN_POINT('Ctrl Pts',(162.977135122943,222.918220049959,1.11130505662254));
#88516=CARTESIAN_POINT('Ctrl Pts',(159.865978920635,221.369750301164,0.952547191390749));
#88517=CARTESIAN_POINT('Ctrl Pts',(156.877197792305,223.143422626784,0.793789326158956));
#88518=CARTESIAN_POINT('Ctrl Pts',(156.746988238107,226.616778962636,0.635031460927165));
#88519=CARTESIAN_POINT('Ctrl Pts',(159.592724492903,228.609330790972,0.47627359569537));
#88520=CARTESIAN_POINT('Ctrl Pts',(162.813708975205,227.300991022112,0.317515730463582));
#88521=CARTESIAN_POINT('Ctrl Pts',(163.454303623542,223.882029725929,0.158757865231786));
#88522=CARTESIAN_POINT('Ctrl Pts',(161.781070948697,222.29471665351,0.0529192884105924));
#88523=CARTESIAN_POINT('Ctrl Pts',(160.793799282533,222.030777046254,-4.44089209850063E-15));
#88524=CARTESIAN_POINT('Ctrl Pts',(160.793799282533,222.030777046254,-4.44089209850063E-15));
#88525=CARTESIAN_POINT('Ctrl Pts',(160.886835118416,222.064809970609,-5.00621204762829E-15));
#88526=CARTESIAN_POINT('Ctrl Pts',(160.977803951042,222.103614854342,-3.61054845394339E-15));
#88527=CARTESIAN_POINT('Ctrl Pts',(161.066498240031,222.146862303535,-3.38618022510673E-15));
#88528=CARTESIAN_POINT('Ctrl Pts',(161.157170865599,222.191074392185,-3.15680743645755E-15));
#88529=CARTESIAN_POINT('Ctrl Pts',(161.245467014803,222.239930057968,-6.14220668071666E-15));
#88530=CARTESIAN_POINT('Ctrl Pts',(161.331136020296,222.293122941464,-6.10622663543836E-15));
#88531=CARTESIAN_POINT('Ctrl Pts',(161.414071261832,222.344618399072,-6.07139474112087E-15));
#88532=CARTESIAN_POINT('Ctrl Pts',(161.494544677277,222.400179547073,-6.69073627993026E-15));
#88533=CARTESIAN_POINT('Ctrl Pts',(161.572295150453,222.459559112292,-6.43929354282591E-15));
#88534=CARTESIAN_POINT('Ctrl Pts',(161.640326814483,222.511516231859,-6.2192811478596E-15));
#88535=CARTESIAN_POINT('Ctrl Pts',(161.706273429172,222.56639754431,-2.90661151556184E-15));
#88536=CARTESIAN_POINT('Ctrl Pts',(161.769934822469,222.624050359897,-2.1094237467878E-15));
#88537=CARTESIAN_POINT('Ctrl Pts',(161.783313637273,222.63616643689,-1.94189006632134E-15));
#88538=CARTESIAN_POINT('Ctrl Pts',(161.796593340256,222.64840686525,-6.04831299584486E-15));
#88539=CARTESIAN_POINT('Ctrl Pts',(161.809754778918,222.660753811381,-5.88418203051333E-15));
#88540=CARTESIAN_POINT('Ctrl Pts',(161.882179684673,222.728696718903,-4.9810003950793E-15));
#88541=CARTESIAN_POINT('Ctrl Pts',(161.951138830584,222.799961748911,-2.73633371429518E-15));
#88542=CARTESIAN_POINT('Ctrl Pts',(162.016392999341,222.874256880864,-3.24740234702858E-15));
#88543=CARTESIAN_POINT('Ctrl Pts',(162.081289534507,222.948144829102,-3.75567000453203E-15));
#88544=CARTESIAN_POINT('Ctrl Pts',(162.142522077819,223.025030556139,-1.03735117717522E-14));
#88545=CARTESIAN_POINT('Ctrl Pts',(162.199811703815,223.104653563377,-1.15740750317173E-14));
#88546=CARTESIAN_POINT('Ctrl Pts',(162.255642413703,223.182248921006,-1.27440651984299E-14));
#88547=CARTESIAN_POINT('Ctrl Pts',(162.307728732862,223.262444662234,-8.20072163964933E-15));
#88548=CARTESIAN_POINT('Ctrl Pts',(162.355765712955,223.34501376585,-9.57567358739198E-15));
#88549=CARTESIAN_POINT('Ctrl Pts',(162.376479601884,223.380618153094,-1.01685626880933E-14));
#88550=CARTESIAN_POINT('Ctrl Pts',(162.396439934948,223.416663958761,-2.61105265973387E-15));
#88551=CARTESIAN_POINT('Ctrl Pts',(162.415619286929,223.453133310247,-2.55351295663786E-15));
#88552=CARTESIAN_POINT('Ctrl Pts',(162.428829636786,223.478252662175,-2.51388077254134E-15));
#88553=CARTESIAN_POINT('Ctrl Pts',(162.441669437427,223.503572954656,-7.17365798022769E-15));
#88554=CARTESIAN_POINT('Ctrl Pts',(162.45412919638,223.529088350617,-7.57727214306669E-15));
#88555=CARTESIAN_POINT('Ctrl Pts',(162.460341835531,223.541810743441,-7.77852075142854E-15));
#88556=CARTESIAN_POINT('Ctrl Pts',(162.466459434798,223.554580665549,4.45523880766167E-15));
#88557=CARTESIAN_POINT('Ctrl Pts',(162.472475628322,223.567385868417,4.13558076672871E-15));
#88558=CARTESIAN_POINT('Ctrl Pts',(162.512676157777,223.652950924293,1.99960850495947E-15));
#88559=CARTESIAN_POINT('Ctrl Pts',(162.548420085257,223.74022617982,-7.11576176770946E-15));
#88560=CARTESIAN_POINT('Ctrl Pts',(162.57945637239,223.828973559839,-6.57807142090405E-15));
#88561=CARTESIAN_POINT('Ctrl Pts',(162.609806626417,223.915759247713,-6.05226630304389E-15));
#88562=CARTESIAN_POINT('Ctrl Pts',(162.635655274658,224.003953374654,-8.47510144726437E-15));
#88563=CARTESIAN_POINT('Ctrl Pts',(162.656718423957,224.093342060539,-8.60422844084496E-15));
#88564=CARTESIAN_POINT('Ctrl Pts',(162.660341324486,224.108717079385,-8.62643852191117E-15));
#88565=CARTESIAN_POINT('Ctrl Pts',(162.663822523297,224.124127446413,-7.27321386741096E-15));
#88566=CARTESIAN_POINT('Ctrl Pts',(162.66716041776,224.139572078222,-7.41073868937292E-15));
#88567=CARTESIAN_POINT('Ctrl Pts',(162.687288010448,224.232703620192,-8.24215987393993E-15));
#88568=CARTESIAN_POINT('Ctrl Pts',(162.702208971776,224.327082113126,-4.25211970581271E-15));
#88569=CARTESIAN_POINT('Ctrl Pts',(162.712001602964,224.422299420426,-4.49640324973188E-15));
#88570=CARTESIAN_POINT('Ctrl Pts',(162.715264301484,224.454023822342,-4.57779338298299E-15));
#88571=CARTESIAN_POINT('Ctrl Pts',(162.71795730133,224.485841219662,-6.6124359778604E-15));
#88572=CARTESIAN_POINT('Ctrl Pts',(162.720082299518,224.51773605842,-6.77236045021345E-15));
#88573=CARTESIAN_POINT('Ctrl Pts',(162.721307102418,224.536119552202,-6.86453744993252E-15));
#88574=CARTESIAN_POINT('Ctrl Pts',(162.722343197653,224.554528767701,-5.15903927657121E-15));
#88575=CARTESIAN_POINT('Ctrl Pts',(162.723190824689,224.572960678251,-5.16253706450698E-15));
#88576=CARTESIAN_POINT('Ctrl Pts',(162.723765351252,224.585453935017,-5.16490788562594E-15));
#88577=CARTESIAN_POINT('Ctrl Pts',(162.72425317236,224.597955994038,-6.09967805737917E-15));
#88578=CARTESIAN_POINT('Ctrl Pts',(162.724654243491,224.610456526116,-6.16173778666962E-15));
#88579=CARTESIAN_POINT('Ctrl Pts',(162.727643891428,224.703637478209,-6.62434086836518E-15));
#88580=CARTESIAN_POINT('Ctrl Pts',(162.725824867569,224.796879642422,-1.66933774719167E-14));
#88581=CARTESIAN_POINT('Ctrl Pts',(162.71933597312,224.889808601752,-1.62370117351429E-14));
#88582=CARTESIAN_POINT('Ctrl Pts',(162.712834227217,224.982921609736,-1.57797421520312E-14));
#88583=CARTESIAN_POINT('Ctrl Pts',(162.701643711728,225.075721151049,-6.75753491926581E-15));
#88584=CARTESIAN_POINT('Ctrl Pts',(162.685853019716,225.167818548531,-6.63358257213531E-15));
#88585=CARTESIAN_POINT('Ctrl Pts',(162.670284954048,225.258617503434,-6.5113777771573E-15));
#88586=CARTESIAN_POINT('Ctrl Pts',(162.650245042262,225.34873481927,-7.10343674945186E-15));
#88587=CARTESIAN_POINT('Ctrl Pts',(162.625775134076,225.437772867359,-5.16253706450698E-15));
#88588=CARTESIAN_POINT('Ctrl Pts',(162.616258293167,225.472401560365,-4.40768202457879E-15));
#88589=CARTESIAN_POINT('Ctrl Pts',(162.606070947409,225.506866665537,-1.0540714498591E-14));
#88590=CARTESIAN_POINT('Ctrl Pts',(162.595213990126,225.541143327577,-1.07136521876328E-14));
#88591=CARTESIAN_POINT('Ctrl Pts',(162.589230777255,225.560033018317,-1.08089572514558E-14));
#88592=CARTESIAN_POINT('Ctrl Pts',(162.583044184862,225.578865461749,-9.70376744646794E-15));
#88593=CARTESIAN_POINT('Ctrl Pts',(162.5766542565,225.597636371203,-9.83935155574045E-15));
#88594=CARTESIAN_POINT('Ctrl Pts',(162.57141771802,225.61301910855,-9.95046256750947E-15));
#88595=CARTESIAN_POINT('Ctrl Pts',(162.566044346708,225.628361043375,-6.98833070421156E-15));
#88596=CARTESIAN_POINT('Ctrl Pts',(162.560539662732,225.643645128936,-7.14706072102445E-15));
#88597=CARTESIAN_POINT('Ctrl Pts',(162.528144649867,225.733591827165,-8.08118536097141E-15));
#88598=CARTESIAN_POINT('Ctrl Pts',(162.491164668217,225.821662225634,-4.71317433233986E-15));
#88599=CARTESIAN_POINT('Ctrl Pts',(162.449672336204,225.907413475919,-6.89032164657988E-15));
#88600=CARTESIAN_POINT('Ctrl Pts',(162.418553087193,225.971726913633,-8.52318213225989E-15));
#88601=CARTESIAN_POINT('Ctrl Pts',(162.384894495877,226.034735294909,-7.87655847841885E-15));
#88602=CARTESIAN_POINT('Ctrl Pts',(162.348709870643,226.096234697731,-9.87404602525999E-15));
#88603=CARTESIAN_POINT('Ctrl Pts',(162.334283447985,226.120753851172,-1.06704229234161E-14));
#88604=CARTESIAN_POINT('Ctrl Pts',(162.319455350187,226.14503295866,-1.36977293069563E-14));
#88605=CARTESIAN_POINT('Ctrl Pts',(162.304225832086,226.169058289372,-1.48908663177849E-14));
#88606=CARTESIAN_POINT('Ctrl Pts',(162.293796027918,226.185511829972,-1.57079759128285E-14));
#88607=CARTESIAN_POINT('Ctrl Pts',(162.283182339175,226.20183930785,-9.08136479655679E-15));
#88608=CARTESIAN_POINT('Ctrl Pts',(162.272389232672,226.21803079415,-8.60422844084496E-15));
#88609=CARTESIAN_POINT('Ctrl Pts',(162.224799544389,226.289423380297,-6.5004068553228E-15));
#88610=CARTESIAN_POINT('Ctrl Pts',(162.173700691787,226.358212217461,-5.45208773016714E-15));
#88611=CARTESIAN_POINT('Ctrl Pts',(162.119126547549,226.424044832575,-1.50227053019591E-15));
#88612=CARTESIAN_POINT('Ctrl Pts',(162.068157640418,226.485528461734,2.18661674160883E-15));
#88613=CARTESIAN_POINT('Ctrl Pts',(162.014156917713,226.544433679649,7.08152378222129E-16));
#88614=CARTESIAN_POINT('Ctrl Pts',(161.957129257532,226.600439071007,2.34621350125863E-16));
#88615=CARTESIAN_POINT('Ctrl Pts',(161.943965225959,226.613367126231,1.07305421308585E-16));
#88616=CARTESIAN_POINT('Ctrl Pts',(161.930639817331,226.626140504577,1.02173491822713E-15));
#88617=CARTESIAN_POINT('Ctrl Pts',(161.917156415839,226.638757807614,8.32667268468867E-16));
#88618=CARTESIAN_POINT('Ctrl Pts',(157.480508380744,224.998011611683,18.387416697508));
#88619=CARTESIAN_POINT('Ctrl Pts',(157.479370464687,224.866458062603,18.3957515808994));
#88620=CARTESIAN_POINT('Ctrl Pts',(157.488784817194,224.735067792401,18.4040864642907));
#88621=CARTESIAN_POINT('Ctrl Pts',(157.509319826656,224.605439283086,18.4124213476821));
#88622=CARTESIAN_POINT('Ctrl Pts',(157.639699345747,223.782410555676,18.4653406360927));
#88623=CARTESIAN_POINT('Ctrl Pts',(158.218369203279,223.030401048359,18.5182599245033));
#88624=CARTESIAN_POINT('Ctrl Pts',(158.980531962808,222.693521799041,18.5711792129139));
#88625=CARTESIAN_POINT('Ctrl Pts',(159.742694722338,222.356642549724,18.6240985013245));
#88626=CARTESIAN_POINT('Ctrl Pts',(160.688350383866,222.434893558407,18.6770177897351));
#88627=CARTESIAN_POINT('Ctrl Pts',(161.384763036137,222.892484799145,18.7299370781456));
#88628=CARTESIAN_POINT('Ctrl Pts',(162.081175688407,223.350076039884,18.7828563665562));
#88629=CARTESIAN_POINT('Ctrl Pts',(162.528345331421,224.187007512678,18.8357756549668));
#88630=CARTESIAN_POINT('Ctrl Pts',(162.521655236428,225.020262799033,18.8886949433774));
#88631=CARTESIAN_POINT('Ctrl Pts',(162.514965141436,225.853518085388,18.941614231788));
#88632=CARTESIAN_POINT('Ctrl Pts',(162.054415308437,226.683097185305,18.9945335201986));
#88633=CARTESIAN_POINT('Ctrl Pts',(161.350736540984,227.129460653096,19.0474528086092));
#88634=CARTESIAN_POINT('Ctrl Pts',(160.64705777353,227.575824120888,19.1003720970198));
#88635=CARTESIAN_POINT('Ctrl Pts',(159.700250071621,227.638971956554,19.1532913854304));
#88636=CARTESIAN_POINT('Ctrl Pts',(158.943607451517,227.289850124473,19.206210673841));
#88637=CARTESIAN_POINT('Ctrl Pts',(158.186964831412,226.940728292392,19.2591299622516));
#88638=CARTESIAN_POINT('Ctrl Pts',(157.620487293112,226.179336792563,19.3120492506622));
#88639=CARTESIAN_POINT('Ctrl Pts',(157.503322532823,225.354415263657,19.3649685390728));
#88640=CARTESIAN_POINT('Ctrl Pts',(157.486755586057,225.23777241796,19.3724512585512));
#88641=CARTESIAN_POINT('Ctrl Pts',(157.47917201796,225.119859378455,19.3799339780296));
#88642=CARTESIAN_POINT('Ctrl Pts',(157.480142558574,225.001823580074,19.387416697508));
#88643=CARTESIAN_POINT('Ctrl Pts',(159.206200717467,222.030777046254,20.));
#88644=CARTESIAN_POINT('Ctrl Pts',(158.218929051303,222.29471665351,19.9470807115894));
#88645=CARTESIAN_POINT('Ctrl Pts',(156.545695974101,223.882026824534,19.8412421347682));
#88646=CARTESIAN_POINT('Ctrl Pts',(157.18629137152,227.300991599666,19.6824842695364));
#88647=CARTESIAN_POINT('Ctrl Pts',(160.40727547618,228.609329940462,19.5237264043046));
#88648=CARTESIAN_POINT('Ctrl Pts',(163.25301142787,226.616779086673,19.3649685390728));
#88649=CARTESIAN_POINT('Ctrl Pts',(163.122801956202,223.143422649729,19.2062106738411));
#88650=CARTESIAN_POINT('Ctrl Pts',(160.13402104345,221.369750709928,19.0474528086092));
#88651=CARTESIAN_POINT('Ctrl Pts',(157.022865163748,222.918220199123,18.8886949433775));
#88652=CARTESIAN_POINT('Ctrl Pts',(156.636247501462,226.372061033706,18.7299370781457));
#88653=CARTESIAN_POINT('Ctrl Pts',(159.328201281756,228.570130672657,18.5711792129139));
#88654=CARTESIAN_POINT('Ctrl Pts',(162.634953757174,227.500846255061,18.4124213476821));
#88655=CARTESIAN_POINT('Ctrl Pts',(163.530211822273,224.142773276525,18.2536634824503));
#88656=CARTESIAN_POINT('Ctrl Pts',(161.194612857913,221.569240989169,18.0949056172185));
#88657=CARTESIAN_POINT('Ctrl Pts',(157.76570777529,222.135535923095,17.9361477519867));
#88658=CARTESIAN_POINT('Ctrl Pts',(156.38162515129,225.323389853416,17.7773898867549));
#88659=CARTESIAN_POINT('Ctrl Pts',(158.309079864678,228.215276638311,17.6186320215231));
#88660=CARTESIAN_POINT('Ctrl Pts',(161.78406422512,228.164542738612,17.4598741562913));
#88661=CARTESIAN_POINT('Ctrl Pts',(163.62627326692,225.217619271453,17.3011162910595));
#88662=CARTESIAN_POINT('Ctrl Pts',(162.14971706585,222.071530741175,17.1423584258277));
#88663=CARTESIAN_POINT('Ctrl Pts',(158.705739934788,221.605577120181,16.9836005605959));
#88664=CARTESIAN_POINT('Ctrl Pts',(156.44626954324,224.246199205187,16.8248426953641));
#88665=CARTESIAN_POINT('Ctrl Pts',(157.439173136224,227.576699738386,16.6660848301324));
#88666=CARTESIAN_POINT('Ctrl Pts',(160.775745369292,228.549004776956,16.5073269649006));
#88667=CARTESIAN_POINT('Ctrl Pts',(163.402355473271,226.273260780993,16.3485690996688));
#88668=CARTESIAN_POINT('Ctrl Pts',(162.915129980759,222.832228569406,16.189811234437));
#88669=CARTESIAN_POINT('Ctrl Pts',(159.759977645044,221.375140685337,16.0310533692052));
#88670=CARTESIAN_POINT('Ctrl Pts',(156.82449375888,223.235523903752,15.8722955039734));
#88671=CARTESIAN_POINT('Ctrl Pts',(156.795233059844,226.710755575947,15.7135376387416));
#88672=CARTESIAN_POINT('Ctrl Pts',(159.698974938352,228.620303812367,15.5547797735098));
#88673=CARTESIAN_POINT('Ctrl Pts',(162.878214941473,227.216550142046,15.396021908278));
#88674=CARTESIAN_POINT('Ctrl Pts',(163.423312743327,223.784209868902,15.2372640430462));
#88675=CARTESIAN_POINT('Ctrl Pts',(160.835394857113,221.464560675923,15.0785061778144));
#88676=CARTESIAN_POINT('Ctrl Pts',(157.482923630517,222.380545413314,14.9197483125826));
#88677=CARTESIAN_POINT('Ctrl Pts',(156.434080598292,225.693854885432,14.7609904473509));
#88678=CARTESIAN_POINT('Ctrl Pts',(158.648766862283,228.372148393688,14.6022325821191));
#88679=CARTESIAN_POINT('Ctrl Pts',(162.100101640777,227.964251824647,14.4434747168873));
#88680=CARTESIAN_POINT('Ctrl Pts',(163.629423480216,224.843472102255,14.2847168516555));
#88681=CARTESIAN_POINT('Ctrl Pts',(161.837097093285,221.865946705725,14.1259589864237));
#88682=CARTESIAN_POINT('Ctrl Pts',(158.363459518822,221.756706760871,13.9672011211919));
#88683=CARTESIAN_POINT('Ctrl Pts',(156.387583728377,224.615728660929,13.8084432559601));
#88684=CARTESIAN_POINT('Ctrl Pts',(157.717791167667,227.826435675394,13.6496853907283));
#88685=CARTESIAN_POINT('Ctrl Pts',(161.136676040562,228.450388870885,13.4909275254965));
#88686=CARTESIAN_POINT('Ctrl Pts',(163.515275045834,225.916546307426,13.3321696602647));
#88687=CARTESIAN_POINT('Ctrl Pts',(162.676694467393,222.543880599453,13.1734117950329));
#88688=CARTESIAN_POINT('Ctrl Pts',(159.388403217653,221.419055270276,13.0146539298011));
#88689=CARTESIAN_POINT('Ctrl Pts',(156.659845319066,223.571510416925,12.8558960645693));
#88690=CARTESIAN_POINT('Ctrl Pts',(156.988196853122,227.031319173831,12.6971381993375));
#88691=CARTESIAN_POINT('Ctrl Pts',(160.072950508764,228.632064702726,12.5383803341058));
#88692=CARTESIAN_POINT('Ctrl Pts',(163.090939861654,226.908744758514,12.379622468874));
#88693=CARTESIAN_POINT('Ctrl Pts',(163.280101174706,223.438541686369,12.2208646036422));
#88694=CARTESIAN_POINT('Ctrl Pts',(160.467314021654,221.397385201457,12.0621067384104));
#88695=CARTESIAN_POINT('Ctrl Pts',(157.226841094361,222.653341638501,11.9033488731786));
#88696=CARTESIAN_POINT('Ctrl Pts',(156.524363088457,226.05695971571,11.7445910079468));
#88697=CARTESIAN_POINT('Ctrl Pts',(159.002787847321,228.493248302664,11.585833142715));
#88698=CARTESIAN_POINT('Ctrl Pts',(162.393861129102,227.732516180389,11.4270752774832));
#88699=CARTESIAN_POINT('Ctrl Pts',(163.594072799666,224.470985357276,11.2683174122514));
#88700=CARTESIAN_POINT('Ctrl Pts',(161.504989185309,221.693608714381,11.1095595470196));
#88701=CARTESIAN_POINT('Ctrl Pts',(158.038539527739,221.942241246064,10.9508016817878));
#88702=CARTESIAN_POINT('Ctrl Pts',(156.36721841725,224.989334469106,10.792043816556));
#88703=CARTESIAN_POINT('Ctrl Pts',(158.020618868438,228.046188785603,10.6332859513243));
#88704=CARTESIAN_POINT('Ctrl Pts',(161.485548853394,228.315171245305,10.4745280860925));
#88705=CARTESIAN_POINT('Ctrl Pts',(163.590904586142,225.55010911167,10.3157702208607));
#88706=CARTESIAN_POINT('Ctrl Pts',(162.409864582861,222.281587140667,10.1570123556289));
#88707=CARTESIAN_POINT('Ctrl Pts',(159.023316608111,221.500956511627,9.99825449039707));
#88708=CARTESIAN_POINT('Ctrl Pts',(156.530629235211,223.922650345549,9.83949662516529));
#88709=CARTESIAN_POINT('Ctrl Pts',(157.213109849816,227.330334540859,9.68073875993349));
#88710=CARTESIAN_POINT('Ctrl Pts',(160.446152220277,228.605296656013,9.52198089470171));
#88711=CARTESIAN_POINT('Ctrl Pts',(163.270876096285,226.580691413359,9.3632230294699));
#88712=CARTESIAN_POINT('Ctrl Pts',(163.102094297597,223.109437451357,9.20446516423812));
#88713=CARTESIAN_POINT('Ctrl Pts',(160.094275919735,221.36842625953,9.04570729900632));
#88714=CARTESIAN_POINT('Ctrl Pts',(157.000176223839,222.951031212172,8.88694943377453));
#88715=CARTESIAN_POINT('Ctrl Pts',(156.65151512992,226.408852318861,8.72819156854274));
#88716=CARTESIAN_POINT('Ctrl Pts',(159.367387257422,228.57729183873,8.56943370331094));
#88717=CARTESIAN_POINT('Ctrl Pts',(162.662226542055,227.471794008467,8.41067583807916));
#88718=CARTESIAN_POINT('Ctrl Pts',(163.520596200089,224.104110398856,8.25191797284736));
#88719=CARTESIAN_POINT('Ctrl Pts',(161.156916354245,221.556344916982,8.09316010761557));
#88720=CARTESIAN_POINT('Ctrl Pts',(157.734426706491,222.160212431668,7.93440224238377));
#88721=CARTESIAN_POINT('Ctrl Pts',(156.385389647865,225.363053417219,7.77564437715199));
#88722=CARTESIAN_POINT('Ctrl Pts',(158.344443841372,228.233627929609,7.61688651192019));
#88723=CARTESIAN_POINT('Ctrl Pts',(161.818662966152,228.144786287979,7.4581286466884));
#88724=CARTESIAN_POINT('Ctrl Pts',(163.628441815827,225.177836359257,7.29937078145661));
#88725=CARTESIAN_POINT('Ctrl Pts',(162.117470858342,222.048130601536,7.14061291622482));
#88726=CARTESIAN_POINT('Ctrl Pts',(158.66859065457,221.61997560121,6.98185505099302));
#88727=CARTESIAN_POINT('Ctrl Pts',(156.438216231379,224.28521879774,6.82309718576123));
#88728=CARTESIAN_POINT('Ctrl Pts',(157.467586173166,227.604629722471,6.66433932052944));
#88729=CARTESIAN_POINT('Ctrl Pts',(160.814621149687,228.540283627621,6.50558145529764));
#88730=CARTESIAN_POINT('Ctrl Pts',(163.416114882048,226.235870095991,6.34682359006586));
#88731=CARTESIAN_POINT('Ctrl Pts',(162.891180408695,222.800388301109,6.18806572483405));
#88732=CARTESIAN_POINT('Ctrl Pts',(159.720237738997,221.377991046555,6.02930785960227));
#88733=CARTESIAN_POINT('Ctrl Pts',(156.805333479567,223.270456243762,5.87054999437047));
#88734=CARTESIAN_POINT('Ctrl Pts',(156.814187894011,226.745799818665,5.71179212913869));
#88735=CARTESIAN_POINT('Ctrl Pts',(159.738697422576,228.623387468178,5.55303426390689));
#88736=CARTESIAN_POINT('Ctrl Pts',(162.902351059725,227.184851049301,5.3942763986751));
#88737=CARTESIAN_POINT('Ctrl Pts',(163.409773121145,223.746739036021,5.2355185334433));
#88738=CARTESIAN_POINT('Ctrl Pts',(160.796570956179,221.455611407691,5.07676066821152));
#88739=CARTESIAN_POINT('Ctrl Pts',(157.454347083443,222.408308079663,4.91800280297972));
#88740=CARTESIAN_POINT('Ctrl Pts',(156.441904659834,225.732921095211,4.75924493774793));
#88741=CARTESIAN_POINT('Ctrl Pts',(158.685830951627,228.386764753245,4.60048707251613));
#88742=CARTESIAN_POINT('Ctrl Pts',(162.132484704811,227.941041442286,4.44172920728434));
#88743=CARTESIAN_POINT('Ctrl Pts',(163.627488540013,224.80367711901,4.28297134205255));
#88744=CARTESIAN_POINT('Ctrl Pts',(161.802615006038,221.845987488677,4.12421347682076));
#88745=CARTESIAN_POINT('Ctrl Pts',(158.327988289432,221.774849984717,3.96545561158897));
#88746=CARTESIAN_POINT('Ctrl Pts',(156.38358662457,224.655369647836,3.80669774635717));
#88747=CARTESIAN_POINT('Ctrl Pts',(157.748926338727,227.851294995875,3.64793988112539));
#88748=CARTESIAN_POINT('Ctrl Pts',(161.174448579081,228.437715275457,3.48918201589359));
#88749=CARTESIAN_POINT('Ctrl Pts',(163.525115526208,225.877938670865,3.3304241506618));
#88750=CARTESIAN_POINT('Ctrl Pts',(162.649596882032,222.514672627688,3.17166628543));
#88751=CARTESIAN_POINT('Ctrl Pts',(159.349167276316,221.4259781011,3.01290842019821));
#88752=CARTESIAN_POINT('Ctrl Pts',(156.644379752265,223.608228269237,2.85415055496642));
#88753=CARTESIAN_POINT('Ctrl Pts',(157.010655750008,227.064227884339,2.69539268973463));
#88754=CARTESIAN_POINT('Ctrl Pts',(160.112779481517,228.63104619244,2.53663482450283));
#88755=CARTESIAN_POINT('Ctrl Pts',(163.111687448995,226.874731226991,2.37787695927104));
#88756=CARTESIAN_POINT('Ctrl Pts',(163.262779158505,223.402662193936,2.21911909403925));
#88757=CARTESIAN_POINT('Ctrl Pts',(160.427775566504,221.392476912117,2.06036122880746));
#88758=CARTESIAN_POINT('Ctrl Pts',(157.201271676567,222.683896091561,1.90160336357566));
#88759=CARTESIAN_POINT('Ctrl Pts',(156.536164079478,226.095014570215,1.74284549834387));
#88760=CARTESIAN_POINT('Ctrl Pts',(159.041158479961,228.50397348879,1.58408763311208));
#88761=CARTESIAN_POINT('Ctrl Pts',(162.423685640744,227.706100715127,1.42532976788028));
#88762=CARTESIAN_POINT('Ctrl Pts',(163.588053642863,224.431594906927,1.2665719026485));
#88763=CARTESIAN_POINT('Ctrl Pts',(161.468639564753,221.677313682196,1.1078140374167));
#88764=CARTESIAN_POINT('Ctrl Pts',(158.005117334405,221.963912797343,0.949056172184911));
#88765=CARTESIAN_POINT('Ctrl Pts',(156.367330897151,225.029226046159,0.790298306953121));
#88766=CARTESIAN_POINT('Ctrl Pts',(158.05412312597,228.067610591205,0.631540441721325));
#88767=CARTESIAN_POINT('Ctrl Pts',(161.521864702141,228.298893654481,0.472782576489533));
#88768=CARTESIAN_POINT('Ctrl Pts',(163.59662383415,225.510249900124,0.314024711257741));
#88769=CARTESIAN_POINT('Ctrl Pts',(162.380110802063,222.256241901603,0.155266846025946));
#88770=CARTESIAN_POINT('Ctrl Pts',(158.984594388107,221.509946987359,-0.00349101920584297));
#88771=CARTESIAN_POINT('Ctrl Pts',(156.520034915627,223.964662694603,-0.162248884437635));
#88772=CARTESIAN_POINT('Ctrl Pts',(156.999831188384,226.220556762667,-0.268087461258832));
#88773=CARTESIAN_POINT('Ctrl Pts',(157.663937342304,226.99730155693,-0.32100674966943));
#88774=CARTESIAN_POINT('Ctrl Pts',(159.254067145653,222.209822430158,20.1070022498898));
#88775=CARTESIAN_POINT('Ctrl Pts',(158.326328373192,222.457846368889,20.0540829614792));
#88776=CARTESIAN_POINT('Ctrl Pts',(156.7539919492,223.949441073822,19.948244384658));
#88777=CARTESIAN_POINT('Ctrl Pts',(157.355959176676,227.162240845431,19.7894865194262));
#88778=CARTESIAN_POINT('Ctrl Pts',(160.38271659491,228.391685837985,19.6307286541944));
#88779=CARTESIAN_POINT('Ctrl Pts',(163.056853480481,226.519286632664,19.4719707889626));
#88780=CARTESIAN_POINT('Ctrl Pts',(162.934495694324,223.255375039161,19.3132129237308));
#88781=CARTESIAN_POINT('Ctrl Pts',(160.12593951857,221.588656257922,19.1544550584991));
#88782=CARTESIAN_POINT('Ctrl Pts',(157.20238763747,223.043752390359,18.9956971932673));
#88783=CARTESIAN_POINT('Ctrl Pts',(156.839083181652,226.289325180472,18.8369393280355));
#88784=CARTESIAN_POINT('Ctrl Pts',(159.368711024974,228.354850302395,18.6781814628037));
#88785=CARTESIAN_POINT('Ctrl Pts',(162.476064945398,227.350044181658,18.5194235975719));
#88786=CARTESIAN_POINT('Ctrl Pts',(163.317338575358,224.194464405884,18.3606657323401));
#88787=CARTESIAN_POINT('Ctrl Pts',(161.122577203773,221.776117190028,18.2019078671083));
#88788=CARTESIAN_POINT('Ctrl Pts',(157.900436529364,222.308264302983,18.0431500018765));
#88789=CARTESIAN_POINT('Ctrl Pts',(156.599814665512,225.303889310224,17.8843921366447));
#88790=CARTESIAN_POINT('Ctrl Pts',(158.411043054878,228.021394114489,17.7256342714129));
#88791=CARTESIAN_POINT('Ctrl Pts',(161.676484407413,227.973719490126,17.5668764061811));
#88792=CARTESIAN_POINT('Ctrl Pts',(163.407607474782,225.204496738517,17.4081185409493));
#88793=CARTESIAN_POINT('Ctrl Pts',(162.020088229169,222.248118660259,17.2493606757175));
#88794=CARTESIAN_POINT('Ctrl Pts',(158.783784357136,221.810262237168,17.0906028104858));
#88795=CARTESIAN_POINT('Ctrl Pts',(156.660560973636,224.291653707862,16.9318449452539));
#88796=CARTESIAN_POINT('Ctrl Pts',(157.593592065377,227.421323668266,16.7730870800222));
#88797=CARTESIAN_POINT('Ctrl Pts',(160.728967599613,228.334998307027,16.6143292147904));
#88798=CARTESIAN_POINT('Ctrl Pts',(163.197192017586,226.196482624251,16.4555713495586));
#88799=CARTESIAN_POINT('Ctrl Pts',(162.739346425713,222.96294609182,16.2968134843268));
#88800=CARTESIAN_POINT('Ctrl Pts',(159.774451093269,221.593721215564,16.138055619095));
#88801=CARTESIAN_POINT('Ctrl Pts',(157.015978111145,223.341922549109,15.9792977538632));
#88802=CARTESIAN_POINT('Ctrl Pts',(156.988481844478,226.607596300395,15.8205398886314));
#88803=CARTESIAN_POINT('Ctrl Pts',(159.717126875262,228.401997980831,15.6617820233996));
#88804=CARTESIAN_POINT('Ctrl Pts',(162.70465737871,227.082891242965,15.5030241581678));
#88805=CARTESIAN_POINT('Ctrl Pts',(163.216885555507,223.857522521458,15.344266292936));
#88806=CARTESIAN_POINT('Ctrl Pts',(160.785020198412,221.67774914338,15.1855084277043));
#88807=CARTESIAN_POINT('Ctrl Pts',(157.634704386597,222.538499618639,15.0267505624724));
#88808=CARTESIAN_POINT('Ctrl Pts',(156.649107027157,225.652015146123,14.8679926972407));
#88809=CARTESIAN_POINT('Ctrl Pts',(158.730246784692,228.168806437515,14.7092348320089));
#88810=CARTESIAN_POINT('Ctrl Pts',(161.973464634945,227.785506201904,14.5504769667771));
#88811=CARTESIAN_POINT('Ctrl Pts',(163.410567728901,224.852910799848,14.3917191015453));
#88812=CARTESIAN_POINT('Ctrl Pts',(161.726319371484,222.054931427987,14.2329612363135));
#88813=CARTESIAN_POINT('Ctrl Pts',(158.462143593171,221.95227869742,14.0742033710817));
#88814=CARTESIAN_POINT('Ctrl Pts',(156.605413937913,224.638900383126,13.9154455058499));
#88815=CARTESIAN_POINT('Ctrl Pts',(157.855409313188,227.656000423995,13.7566876406181));
#88816=CARTESIAN_POINT('Ctrl Pts',(161.0681340007,228.242328981268,13.5979297753863));
#88817=CARTESIAN_POINT('Ctrl Pts',(163.303302492774,225.861278182386,13.4391719101545));
#88818=CARTESIAN_POINT('Ctrl Pts',(162.515288673361,222.691985624853,13.2804140449227));
#88819=CARTESIAN_POINT('Ctrl Pts',(159.425282758999,221.634987732694,13.1216561796909));
#88820=CARTESIAN_POINT('Ctrl Pts',(156.861258041001,223.657648935247,12.9628983144592));
#88821=CARTESIAN_POINT('Ctrl Pts',(157.169809840451,226.908829779476,12.8041404492274));
#88822=CARTESIAN_POINT('Ctrl Pts',(160.068551562625,228.413049684591,12.6453825839956));
#88823=CARTESIAN_POINT('Ctrl Pts',(162.904554897381,226.793646652583,12.4866247187638));
#88824=CARTESIAN_POINT('Ctrl Pts',(163.082309704272,223.532698274665,12.327866853532));
#88825=CARTESIAN_POINT('Ctrl Pts',(160.439134791023,221.614624378073,12.1691089883002));
#88826=CARTESIAN_POINT('Ctrl Pts',(157.394063734297,222.794846117542,12.0103511230684));
#88827=CARTESIAN_POINT('Ctrl Pts',(156.733945445467,225.993224603521,11.8515932578366));
#88828=CARTESIAN_POINT('Ctrl Pts',(159.062920156511,228.282603971415,11.6928353926048));
#88829=CARTESIAN_POINT('Ctrl Pts',(162.249510303466,227.567744313755,11.534077527373));
#88830=CARTESIAN_POINT('Ctrl Pts',(163.377348709149,224.502885161121,11.3753196621412));
#88831=CARTESIAN_POINT('Ctrl Pts',(161.41423770903,221.89298548948,11.2165617969094));
#88832=CARTESIAN_POINT('Ctrl Pts',(158.15681641322,222.126625375687,11.0578039316776));
#88833=CARTESIAN_POINT('Ctrl Pts',(156.58627666355,224.989977605072,10.8990460664458));
#88834=CARTESIAN_POINT('Ctrl Pts',(158.139976377158,227.862502329901,10.7402882012141));
#88835=CARTESIAN_POINT('Ctrl Pts',(161.395969637247,228.11526503497,10.5815303359823));
#88836=CARTESIAN_POINT('Ctrl Pts',(163.374371540223,225.516937302539,10.4227724707505));
#88837=CARTESIAN_POINT('Ctrl Pts',(162.264548742281,222.445508571152,10.2640146055187));
#88838=CARTESIAN_POINT('Ctrl Pts',(159.082211024455,221.711950294994,10.1052567402869));
#88839=CARTESIAN_POINT('Ctrl Pts',(156.739833740956,223.987614979558,9.9464988750551));
#88840=CARTESIAN_POINT('Ctrl Pts',(157.381160489532,227.189814395019,9.7877410098233));
#88841=CARTESIAN_POINT('Ctrl Pts',(160.419249055105,228.387895762271,9.62898314459152));
#88842=CARTESIAN_POINT('Ctrl Pts',(163.073640901932,226.485375061119,9.47022527935972));
#88843=CARTESIAN_POINT('Ctrl Pts',(162.915036716179,223.223439162441,9.31146741412793));
#88844=CARTESIAN_POINT('Ctrl Pts',(160.08859104241,221.587411672436,9.15270954889613));
#88845=CARTESIAN_POINT('Ctrl Pts',(157.181066850111,223.074584885621,8.99395168366435));
#88846=CARTESIAN_POINT('Ctrl Pts',(156.853430165738,226.32389793577,8.83519381843254));
#88847=CARTESIAN_POINT('Ctrl Pts',(159.405534069946,228.361579647164,8.67643595320076));
#88848=CARTESIAN_POINT('Ctrl Pts',(162.501693169962,227.322743797664,8.51767808796897));
#88849=CARTESIAN_POINT('Ctrl Pts',(163.308302779206,224.158132915882,8.35892022273717));
#88850=CARTESIAN_POINT('Ctrl Pts',(161.087153815016,221.763998756378,8.20016235750538));
#88851=CARTESIAN_POINT('Ctrl Pts',(157.871041722075,222.331452807785,8.04140449227359));
#88852=CARTESIAN_POINT('Ctrl Pts',(156.603352161372,225.341161144569,7.88264662704179));
#88853=CARTESIAN_POINT('Ctrl Pts',(158.444274569011,228.038638815259,7.72388876181));
#88854=CARTESIAN_POINT('Ctrl Pts',(161.708996829914,227.955154361715,7.56513089657821));
#88855=CARTESIAN_POINT('Ctrl Pts',(163.409645259285,225.167112752539,7.40637303134642));
#88856=CARTESIAN_POINT('Ctrl Pts',(161.989786481439,222.22612955881,7.24761516611462));
#88857=CARTESIAN_POINT('Ctrl Pts',(158.748875194027,221.823792483779,7.08885730088284));
#88858=CARTESIAN_POINT('Ctrl Pts',(156.652993279842,224.328320402691,6.93009943565103));
#88859=CARTESIAN_POINT('Ctrl Pts',(157.620291784328,227.447569462648,6.77134157041925));
#88860=CARTESIAN_POINT('Ctrl Pts',(160.765499154218,228.326803046637,6.61258370518745));
#88861=CARTESIAN_POINT('Ctrl Pts',(163.210121728269,226.161346613168,6.45382583995566));
#88862=CARTESIAN_POINT('Ctrl Pts',(162.716841022844,222.933025804996,6.29506797472387));
#88863=CARTESIAN_POINT('Ctrl Pts',(159.737107520149,221.59639969881,6.13631010949208));
#88864=CARTESIAN_POINT('Ctrl Pts',(156.997973204676,223.37474845443,5.97755224426028));
#88865=CARTESIAN_POINT('Ctrl Pts',(157.006293694231,226.640527360644,5.81879437902849));
#88866=CARTESIAN_POINT('Ctrl Pts',(159.754454077101,228.404895690909,5.66003651379671));
#88867=CARTESIAN_POINT('Ctrl Pts',(162.727338078953,227.053103618748,5.50127864856491));
#88868=CARTESIAN_POINT('Ctrl Pts',(163.204162378196,223.822311195445,5.34252078333312));
#88869=CARTESIAN_POINT('Ctrl Pts',(160.748537394915,221.669339519759,5.18376291810132));
#88870=CARTESIAN_POINT('Ctrl Pts',(157.607851017243,222.564588184615,5.02500505286953));
#88871=CARTESIAN_POINT('Ctrl Pts',(156.656459294521,225.68872564714,4.86624718763774));
#88872=CARTESIAN_POINT('Ctrl Pts',(158.765075893972,228.182541424488,4.70748932240594));
#88873=CARTESIAN_POINT('Ctrl Pts',(162.003894986697,227.763695415291,4.54873145717415));
#88874=CARTESIAN_POINT('Ctrl Pts',(163.4087494664,224.815515470708,4.38997359194236));
#88875=CARTESIAN_POINT('Ctrl Pts',(161.693916568495,222.036175760061,4.23121572671057));
#88876=CARTESIAN_POINT('Ctrl Pts',(158.428811293724,221.969327877293,4.07245786147877));
#88877=CARTESIAN_POINT('Ctrl Pts',(156.601657861134,224.676151001972,3.91369999624698));
#88878=CARTESIAN_POINT('Ctrl Pts',(157.884667020433,227.679360717071,3.75494213101519));
#88879=CARTESIAN_POINT('Ctrl Pts',(161.103628839374,228.230419608936,3.5961842657834));
#88880=CARTESIAN_POINT('Ctrl Pts',(163.312549588073,225.82499860243,3.43742640055161));
#88881=CARTESIAN_POINT('Ctrl Pts',(162.489825083712,222.664538905981,3.27866853531981));
#88882=CARTESIAN_POINT('Ctrl Pts',(159.388412761308,221.641493113929,3.11991067008802));
#88883=CARTESIAN_POINT('Ctrl Pts',(156.846725054335,223.692152685734,2.96115280485623));
#88884=CARTESIAN_POINT('Ctrl Pts',(157.190914456477,226.939754080999,2.80239493962444));
#88885=CARTESIAN_POINT('Ctrl Pts',(160.105978831691,228.412092590901,2.64363707439264));
#88886=CARTESIAN_POINT('Ctrl Pts',(162.924051396542,226.761684151213,2.48487920916085));
#88887=CARTESIAN_POINT('Ctrl Pts',(163.06603221288,223.498982330607,2.32612134392906));
#88888=CARTESIAN_POINT('Ctrl Pts',(160.401980521227,221.61001206063,2.16736347869727));
#88889=CARTESIAN_POINT('Ctrl Pts',(157.370036163074,222.823558124324,2.00860561346547));
#88890=CARTESIAN_POINT('Ctrl Pts',(156.745034831803,226.028984734411,1.84984774823368));
#88891=CARTESIAN_POINT('Ctrl Pts',(159.098977023982,228.292682424339,1.69108988300189));
#88892=CARTESIAN_POINT('Ctrl Pts',(162.277536384602,227.542921712078,1.53233201777009));
#88893=CARTESIAN_POINT('Ctrl Pts',(163.371692510015,224.465869971375,1.37357415253831));
#88894=CARTESIAN_POINT('Ctrl Pts',(161.380079985771,221.87767305454,1.21481628730651));
#88895=CARTESIAN_POINT('Ctrl Pts',(158.1254095921,222.146990123374,1.05605842207472));
#88896=CARTESIAN_POINT('Ctrl Pts',(156.586382360866,225.027463703372,0.89730055684293));
#88897=CARTESIAN_POINT('Ctrl Pts',(158.171460313971,227.882632391681,0.738542691611135));
#88898=CARTESIAN_POINT('Ctrl Pts',(161.430095625151,228.099968989669,0.579784826379343));
#88899=CARTESIAN_POINT('Ctrl Pts',(163.379745915188,225.479481618092,0.421026961147551));
#88900=CARTESIAN_POINT('Ctrl Pts',(162.236589126888,222.421691660586,0.262269095915756));
#88901=CARTESIAN_POINT('Ctrl Pts',(159.045823770485,221.720398641285,0.103511230683967));
#88902=CARTESIAN_POINT('Ctrl Pts',(156.729878263267,224.027093966422,-0.0552466345478245));
#88903=CARTESIAN_POINT('Ctrl Pts',(157.180742620438,226.146956680238,-0.161085211369022));
#88904=CARTESIAN_POINT('Ctrl Pts',(157.804802895981,226.876863439079,-0.21400449977962));
#88905=CARTESIAN_POINT('Ctrl Pts',(159.301933573839,222.388867814061,20.2140044997796));
#88906=CARTESIAN_POINT('Ctrl Pts',(158.433727695081,222.620976084267,20.161085211369));
#88907=CARTESIAN_POINT('Ctrl Pts',(156.962287924299,224.01685532311,20.0552466345478));
#88908=CARTESIAN_POINT('Ctrl Pts',(157.525626981831,227.023490091198,19.896488769316));
#88909=CARTESIAN_POINT('Ctrl Pts',(160.358157713639,228.174041735507,19.7377309040842));
#88910=CARTESIAN_POINT('Ctrl Pts',(162.860695533093,226.421794178655,19.5789730388525));
#88911=CARTESIAN_POINT('Ctrl Pts',(162.746189432446,223.367327428592,19.4202151736207));
#88912=CARTESIAN_POINT('Ctrl Pts',(160.11785799369,221.807561805916,19.2614573083889));
#88913=CARTESIAN_POINT('Ctrl Pts',(157.381910111192,223.169284581594,19.1026994431571));
#88914=CARTESIAN_POINT('Ctrl Pts',(157.041918861842,226.206589327239,18.9439415779253));
#88915=CARTESIAN_POINT('Ctrl Pts',(159.409220768192,228.139569932133,18.7851837126935));
#88916=CARTESIAN_POINT('Ctrl Pts',(162.317176133621,227.199242108255,18.6264258474617));
#88917=CARTESIAN_POINT('Ctrl Pts',(163.104465328442,224.246155535242,18.4676679822299));
#88918=CARTESIAN_POINT('Ctrl Pts',(161.050541549633,221.982993390887,18.3089101169981));
#88919=CARTESIAN_POINT('Ctrl Pts',(158.035165283438,222.480992682871,18.1501522517663));
#88920=CARTESIAN_POINT('Ctrl Pts',(156.818004179734,225.284388767032,17.9913943865345));
#88921=CARTESIAN_POINT('Ctrl Pts',(158.513006245078,227.827511590667,17.8326365213027));
#88922=CARTESIAN_POINT('Ctrl Pts',(161.568904589706,227.782896241639,17.673878656071));
#88923=CARTESIAN_POINT('Ctrl Pts',(163.188941682644,225.191374205583,17.5151207908391));
#88924=CARTESIAN_POINT('Ctrl Pts',(161.890459392489,222.424706579342,17.3563629256074));
#88925=CARTESIAN_POINT('Ctrl Pts',(158.861828779484,222.014947354155,17.1976050603756));
#88926=CARTESIAN_POINT('Ctrl Pts',(156.874852404031,224.337108210537,17.0388471951438));
#88927=CARTESIAN_POINT('Ctrl Pts',(157.748010994531,227.265947598146,16.880089329912));
#88928=CARTESIAN_POINT('Ctrl Pts',(160.682189829934,228.120991837097,16.7213314646802));
#88929=CARTESIAN_POINT('Ctrl Pts',(162.992028561902,226.11970446751,16.5625735994484));
#88930=CARTESIAN_POINT('Ctrl Pts',(162.563562870667,223.093663614233,16.4038157342166));
#88931=CARTESIAN_POINT('Ctrl Pts',(159.788924541493,221.81230174579,16.2450578689848));
#88932=CARTESIAN_POINT('Ctrl Pts',(157.20746246341,223.448321194466,16.086300003753));
#88933=CARTESIAN_POINT('Ctrl Pts',(157.181730629114,226.504437024843,15.9275421385212));
#88934=CARTESIAN_POINT('Ctrl Pts',(159.735278812172,228.183692149295,15.7687842732894));
#88935=CARTESIAN_POINT('Ctrl Pts',(162.531099815947,226.949232343883,15.6100264080576));
#88936=CARTESIAN_POINT('Ctrl Pts',(163.010458367688,223.930835174013,15.4512685428259));
#88937=CARTESIAN_POINT('Ctrl Pts',(160.73464553971,221.890937610836,15.292510677594));
#88938=CARTESIAN_POINT('Ctrl Pts',(157.786485142676,222.696453823964,15.1337528123623));
#88939=CARTESIAN_POINT('Ctrl Pts',(156.864133456022,225.610175406814,14.9749949471305));
#88940=CARTESIAN_POINT('Ctrl Pts',(158.811726707101,227.965464481343,14.8162370818987));
#88941=CARTESIAN_POINT('Ctrl Pts',(161.846827629113,227.606760579161,14.6574792166669));
#88942=CARTESIAN_POINT('Ctrl Pts',(163.191711977586,224.862349497439,14.4987213514351));
#88943=CARTESIAN_POINT('Ctrl Pts',(161.615541649683,222.243916150249,14.3399634862033));
#88944=CARTESIAN_POINT('Ctrl Pts',(158.56082766752,222.14785063397,14.1812056209715));
#88945=CARTESIAN_POINT('Ctrl Pts',(156.823244147448,224.662072105324,14.0224477557397));
#88946=CARTESIAN_POINT('Ctrl Pts',(157.993027458709,227.485565172597,13.8636898905079));
#88947=CARTESIAN_POINT('Ctrl Pts',(160.999591960837,228.034269091652,13.7049320252761));
#88948=CARTESIAN_POINT('Ctrl Pts',(163.091329939715,225.806010057346,13.5461741600443));
#88949=CARTESIAN_POINT('Ctrl Pts',(162.353882879329,222.840090650254,13.3874162948126));
#88950=CARTESIAN_POINT('Ctrl Pts',(159.462162300346,221.850920195112,13.2286584295807));
#88951=CARTESIAN_POINT('Ctrl Pts',(157.062670762936,223.74378745357,13.069900564349));
#88952=CARTESIAN_POINT('Ctrl Pts',(157.351422827779,226.786340385121,12.9111426991172));
#88953=CARTESIAN_POINT('Ctrl Pts',(160.064152616487,228.194034666456,12.7523848338854));
#88954=CARTESIAN_POINT('Ctrl Pts',(162.718169933108,226.678548546653,12.5936269686536));
#88955=CARTESIAN_POINT('Ctrl Pts',(162.884518233838,223.62685486296,12.4348691034218));
#88956=CARTESIAN_POINT('Ctrl Pts',(160.410955560391,221.83186355469,12.27611123819));
#88957=CARTESIAN_POINT('Ctrl Pts',(157.561286374234,222.936350596582,12.1173533729582));
#88958=CARTESIAN_POINT('Ctrl Pts',(156.943527802478,225.929489491333,11.9585955077264));
#88959=CARTESIAN_POINT('Ctrl Pts',(159.123052465701,228.071959640166,11.7998376424946));
#88960=CARTESIAN_POINT('Ctrl Pts',(162.10515947783,227.402972447122,11.6410797772628));
#88961=CARTESIAN_POINT('Ctrl Pts',(163.160624618632,224.534784964966,11.482321912031));
#88962=CARTESIAN_POINT('Ctrl Pts',(161.32348623275,222.092362264579,11.3235640467992));
#88963=CARTESIAN_POINT('Ctrl Pts',(158.275093298701,222.31100950531,11.1648061815674));
#88964=CARTESIAN_POINT('Ctrl Pts',(156.80533490985,224.990620741038,11.0060483163357));
#88965=CARTESIAN_POINT('Ctrl Pts',(158.259333885877,227.6788158742,10.8472904511039));
#88966=CARTESIAN_POINT('Ctrl Pts',(161.306390421099,227.915358824636,10.6885325858721));
#88967=CARTESIAN_POINT('Ctrl Pts',(163.157838494304,225.483765493408,10.5297747206403));
#88968=CARTESIAN_POINT('Ctrl Pts',(162.119232901701,222.609430001637,10.3710168554085));
#88969=CARTESIAN_POINT('Ctrl Pts',(159.141105440797,221.922944078361,10.2122589901767));
#88970=CARTESIAN_POINT('Ctrl Pts',(156.949038246701,224.052579613566,10.0535011249449));
#88971=CARTESIAN_POINT('Ctrl Pts',(157.549211129248,227.049294249179,9.89474325971311));
#88972=CARTESIAN_POINT('Ctrl Pts',(160.392345889932,228.17049486853,9.73598539448132));
#88973=CARTESIAN_POINT('Ctrl Pts',(162.876405707579,226.390058708879,9.57722752924953));
#88974=CARTESIAN_POINT('Ctrl Pts',(162.727979134762,223.337440873524,9.41846966401773));
#88975=CARTESIAN_POINT('Ctrl Pts',(160.082906165086,221.806397085342,9.25971179878595));
#88976=CARTESIAN_POINT('Ctrl Pts',(157.361957476384,223.198138559069,9.10095393355415));
#88977=CARTESIAN_POINT('Ctrl Pts',(157.055345201557,226.23894355268,8.94219606832236));
#88978=CARTESIAN_POINT('Ctrl Pts',(159.443680882469,228.145867455598,8.78343820309056));
#88979=CARTESIAN_POINT('Ctrl Pts',(162.341159797869,227.173693586861,8.62468033785878));
#88980=CARTESIAN_POINT('Ctrl Pts',(163.096009358323,224.212155432907,8.46592247262698));
#88981=CARTESIAN_POINT('Ctrl Pts',(161.017391275787,221.971652595775,8.30716460739519));
#88982=CARTESIAN_POINT('Ctrl Pts',(158.007656737659,222.502693183903,8.1484067421634));
#88983=CARTESIAN_POINT('Ctrl Pts',(156.821314674878,225.319268871918,7.98964887693161));
#88984=CARTESIAN_POINT('Ctrl Pts',(158.54410529665,227.843649700909,7.83089101169981));
#88985=CARTESIAN_POINT('Ctrl Pts',(161.599330693676,227.765522435452,7.67213314646802));
#88986=CARTESIAN_POINT('Ctrl Pts',(163.190848702742,225.156389145821,7.51337528123624));
#88987=CARTESIAN_POINT('Ctrl Pts',(161.862102104535,222.404128516084,7.35461741600443));
#88988=CARTESIAN_POINT('Ctrl Pts',(158.829159733483,222.027609366348,7.19585955077264));
#88989=CARTESIAN_POINT('Ctrl Pts',(156.867770328305,224.371422007643,7.03710168554085));
#88990=CARTESIAN_POINT('Ctrl Pts',(157.77299739549,227.290509202825,6.87834382030906));
#88991=CARTESIAN_POINT('Ctrl Pts',(160.716377158748,228.113322465654,6.71958595507727));
#88992=CARTESIAN_POINT('Ctrl Pts',(163.00412857449,226.086823130344,6.56082808984547));
#88993=CARTESIAN_POINT('Ctrl Pts',(162.542501636994,223.065663308882,6.40207022461368));
#88994=CARTESIAN_POINT('Ctrl Pts',(159.753977301302,221.814808351065,6.24331235938189));
#88995=CARTESIAN_POINT('Ctrl Pts',(157.190612929784,223.479040665098,6.08455449415009));
#88996=CARTESIAN_POINT('Ctrl Pts',(157.198399494451,226.535254902624,5.92579662891831));
#88997=CARTESIAN_POINT('Ctrl Pts',(159.770210731627,228.18640391364,5.76703876368651));
#88998=CARTESIAN_POINT('Ctrl Pts',(162.552325098181,226.921356188195,5.60828089845472));
#88999=CARTESIAN_POINT('Ctrl Pts',(162.998551635248,223.89788335487,5.44952303322292));
#89000=CARTESIAN_POINT('Ctrl Pts',(160.700503833651,221.883067631827,5.29076516799114));
#89001=CARTESIAN_POINT('Ctrl Pts',(157.761354951043,222.720868289566,5.13200730275934));
#89002=CARTESIAN_POINT('Ctrl Pts',(156.871013929208,225.644530199069,4.97324943752755));
#89003=CARTESIAN_POINT('Ctrl Pts',(158.844320836317,227.978318095731,4.81449157229576));
#89004=CARTESIAN_POINT('Ctrl Pts',(161.875305268582,227.586349388296,4.65573370706397));
#89005=CARTESIAN_POINT('Ctrl Pts',(163.190010392787,224.827353822406,4.49697584183217));
#89006=CARTESIAN_POINT('Ctrl Pts',(161.585218130953,222.226364031445,4.33821797660038));
#89007=CARTESIAN_POINT('Ctrl Pts',(158.529634298016,222.163805769869,4.17946011136858));
#89008=CARTESIAN_POINT('Ctrl Pts',(156.819729097698,224.696932356107,4.0207022461368));
#89009=CARTESIAN_POINT('Ctrl Pts',(158.020407702139,227.507426438268,3.861944380905));
#89010=CARTESIAN_POINT('Ctrl Pts',(161.032809099667,228.023123942415,3.70318651567321));
#89011=CARTESIAN_POINT('Ctrl Pts',(163.099983649938,225.772058533996,3.54442865044141));
#89012=CARTESIAN_POINT('Ctrl Pts',(162.330053285392,222.814405184275,3.38567078520963));
#89013=CARTESIAN_POINT('Ctrl Pts',(159.4276582463,221.857008126758,3.22691291997783));
#89014=CARTESIAN_POINT('Ctrl Pts',(157.049070356406,223.77607710223,3.06815505474604));
#89015=CARTESIAN_POINT('Ctrl Pts',(157.371173162946,226.81528027766,2.90939718951425));
#89016=CARTESIAN_POINT('Ctrl Pts',(160.099178181865,228.193138989361,2.75063932428246));
#89017=CARTESIAN_POINT('Ctrl Pts',(162.736415344089,226.648637075436,2.59188145905066));
#89018=CARTESIAN_POINT('Ctrl Pts',(162.869285267256,223.595302467277,2.43312359381887));
#89019=CARTESIAN_POINT('Ctrl Pts',(160.37618547595,221.827547209143,2.27436572858708));
#89020=CARTESIAN_POINT('Ctrl Pts',(157.538800649579,222.963220157087,2.11560786335528));
#89021=CARTESIAN_POINT('Ctrl Pts',(156.953905584128,225.962954898605,1.95684999812349));
#89022=CARTESIAN_POINT('Ctrl Pts',(159.156795568002,228.081391359888,1.7980921328917));
#89023=CARTESIAN_POINT('Ctrl Pts',(162.131387128461,227.37974270903,1.63933426765991));
#89024=CARTESIAN_POINT('Ctrl Pts',(163.155331377166,224.500145035824,1.48057640242812));
#89025=CARTESIAN_POINT('Ctrl Pts',(161.291520406789,222.078032426884,1.32181853719632));
#89026=CARTESIAN_POINT('Ctrl Pts',(158.245701849794,222.330067449406,1.16306067196453));
#89027=CARTESIAN_POINT('Ctrl Pts',(156.805433824581,225.025701360586,1.00430280673274));
#89028=CARTESIAN_POINT('Ctrl Pts',(158.288797501971,227.697654192157,0.845544941500946));
#89029=CARTESIAN_POINT('Ctrl Pts',(161.33832654816,227.901044324858,0.686787076269153));
#89030=CARTESIAN_POINT('Ctrl Pts',(163.162867996227,225.448713336061,0.528029211037362));
#89031=CARTESIAN_POINT('Ctrl Pts',(162.093067451714,222.58714141957,0.369271345805566));
#89032=CARTESIAN_POINT('Ctrl Pts',(159.107053152862,221.930850295212,0.210513480573777));
#89033=CARTESIAN_POINT('Ctrl Pts',(156.939721610906,224.08952523824,0.0517556153419854));
#89034=CARTESIAN_POINT('Ctrl Pts',(157.361654052493,226.073356597808,-0.0540829614792118));
#89035=CARTESIAN_POINT('Ctrl Pts',(157.945668449658,226.756425321227,-0.10700224988981));
#89036=CARTESIAN_POINT('Ctrl Pts',(159.349800002025,222.567913197965,20.3210067496694));
#89037=CARTESIAN_POINT('Ctrl Pts',(158.541127016969,222.784105799646,20.2680874612588));
#89038=CARTESIAN_POINT('Ctrl Pts',(157.170583899398,224.084269572398,20.1622488844377));
#89039=CARTESIAN_POINT('Ctrl Pts',(157.695294786986,226.884739336963,20.0034910192058));
#89040=CARTESIAN_POINT('Ctrl Pts',(160.333598832368,227.956397633029,19.8447331539741));
#89041=CARTESIAN_POINT('Ctrl Pts',(162.664537585704,226.324301724646,19.6859752887423));
#89042=CARTESIAN_POINT('Ctrl Pts',(162.557883170567,223.479279818023,19.5272174235105));
#89043=CARTESIAN_POINT('Ctrl Pts',(160.10977646881,222.02646735391,19.3684595582787));
#89044=CARTESIAN_POINT('Ctrl Pts',(157.561432584915,223.29481677283,19.2097016930469));
#89045=CARTESIAN_POINT('Ctrl Pts',(157.244754542031,226.123853474005,19.0509438278151));
#89046=CARTESIAN_POINT('Ctrl Pts',(159.449730511411,227.924289561872,18.8921859625833));
#89047=CARTESIAN_POINT('Ctrl Pts',(162.158287321844,227.048440034851,18.7334280973515));
#89048=CARTESIAN_POINT('Ctrl Pts',(162.891592081527,224.297846664601,18.5746702321197));
#89049=CARTESIAN_POINT('Ctrl Pts',(160.978505895493,222.189869591746,18.4159123668879));
#89050=CARTESIAN_POINT('Ctrl Pts',(158.169894037512,222.653721062759,18.2571545016561));
#89051=CARTESIAN_POINT('Ctrl Pts',(157.036193693956,225.26488822384,18.0983966364243));
#89052=CARTESIAN_POINT('Ctrl Pts',(158.614969435278,227.633629066845,17.9396387711925));
#89053=CARTESIAN_POINT('Ctrl Pts',(161.461324771999,227.592072993153,17.7808809059608));
#89054=CARTESIAN_POINT('Ctrl Pts',(162.970275890506,225.178251672648,17.622123040729));
#89055=CARTESIAN_POINT('Ctrl Pts',(161.760830555808,222.601294498425,17.4633651754972));
#89056=CARTESIAN_POINT('Ctrl Pts',(158.939873201832,222.219632471142,17.3046073102654));
#89057=CARTESIAN_POINT('Ctrl Pts',(157.089143834426,224.382562713212,17.1458494450336));
#89058=CARTESIAN_POINT('Ctrl Pts',(157.902429923685,227.110571528026,16.9870915798018));
#89059=CARTESIAN_POINT('Ctrl Pts',(160.635412060255,227.906985367167,16.82833371457));
#89060=CARTESIAN_POINT('Ctrl Pts',(162.786865106217,226.042926310769,16.6695758493382));
#89061=CARTESIAN_POINT('Ctrl Pts',(162.387779315621,223.224381136646,16.5108179841064));
#89062=CARTESIAN_POINT('Ctrl Pts',(159.803397989718,222.030882276016,16.3520601188746));
#89063=CARTESIAN_POINT('Ctrl Pts',(157.398946815676,223.554719839823,16.1933022536428));
#89064=CARTESIAN_POINT('Ctrl Pts',(157.374979413748,226.401277749291,16.034544388411));
#89065=CARTESIAN_POINT('Ctrl Pts',(159.753430749081,227.965386317759,15.8757865231793));
#89066=CARTESIAN_POINT('Ctrl Pts',(162.357542253183,226.815573444802,15.7170286579474));
#89067=CARTESIAN_POINT('Ctrl Pts',(162.804031179868,224.004147826569,15.5582707927157));
#89068=CARTESIAN_POINT('Ctrl Pts',(160.684270881009,222.104126078293,15.3995129274839));
#89069=CARTESIAN_POINT('Ctrl Pts',(157.938265898756,222.854408029289,15.2407550622521));
#89070=CARTESIAN_POINT('Ctrl Pts',(157.079159884887,225.568335667504,15.0819971970203));
#89071=CARTESIAN_POINT('Ctrl Pts',(158.89320662951,227.76212252517,14.9232393317885));
#89072=CARTESIAN_POINT('Ctrl Pts',(161.720190623281,227.428014956417,14.7644814665567));
#89073=CARTESIAN_POINT('Ctrl Pts',(162.972856226271,224.871788195031,14.6057236013249));
#89074=CARTESIAN_POINT('Ctrl Pts',(161.504763927882,222.432900872511,14.4469657360931));
#89075=CARTESIAN_POINT('Ctrl Pts',(158.659511741869,222.34342257052,14.2882078708613));
#89076=CARTESIAN_POINT('Ctrl Pts',(157.041074356984,224.685243827522,14.1294500056295));
#89077=CARTESIAN_POINT('Ctrl Pts',(158.13064560423,227.315129921198,13.9706921403977));
#89078=CARTESIAN_POINT('Ctrl Pts',(160.931049920975,227.826209202034,13.8119342751659));
#89079=CARTESIAN_POINT('Ctrl Pts',(162.879357386656,225.750741932307,13.6531764099341));
#89080=CARTESIAN_POINT('Ctrl Pts',(162.192477085297,222.988195675654,13.4944185447024));
#89081=CARTESIAN_POINT('Ctrl Pts',(159.499041841692,222.06685265753,13.3356606794706));
#89082=CARTESIAN_POINT('Ctrl Pts',(157.26408348487,223.829925971892,13.1769028142388));
#89083=CARTESIAN_POINT('Ctrl Pts',(157.533035815108,226.663850990766,13.018144949007));
#89084=CARTESIAN_POINT('Ctrl Pts',(160.059753670348,227.97501964832,12.8593870837752));
#89085=CARTESIAN_POINT('Ctrl Pts',(162.531784968835,226.563450440722,12.7006292185434));
#89086=CARTESIAN_POINT('Ctrl Pts',(162.686726763404,223.721011451256,12.5418713533116));
#89087=CARTESIAN_POINT('Ctrl Pts',(160.382776329759,222.049102731306,12.3831134880798));
#89088=CARTESIAN_POINT('Ctrl Pts',(157.728509014171,223.077855075623,12.224355622848));
#89089=CARTESIAN_POINT('Ctrl Pts',(157.153110159489,225.865754379144,12.0655977576162));
#89090=CARTESIAN_POINT('Ctrl Pts',(159.183184774892,227.861315308917,11.9068398923844));
#89091=CARTESIAN_POINT('Ctrl Pts',(161.960808652193,227.238200580488,11.7480820271526));
#89092=CARTESIAN_POINT('Ctrl Pts',(162.943900528114,224.566684768811,11.5893241619208));
#89093=CARTESIAN_POINT('Ctrl Pts',(161.232734756471,222.291739039679,11.4305662966891));
#89094=CARTESIAN_POINT('Ctrl Pts',(158.393370184182,222.495393634933,11.2718084314573));
#89095=CARTESIAN_POINT('Ctrl Pts',(157.02439315615,224.991263877004,11.1130505662255));
#89096=CARTESIAN_POINT('Ctrl Pts',(158.378691394597,227.495129418499,10.9542927009937));
#89097=CARTESIAN_POINT('Ctrl Pts',(161.216811204952,227.715452614301,10.7955348357619));
#89098=CARTESIAN_POINT('Ctrl Pts',(162.941305448385,225.450593684278,10.6367769705301));
#89099=CARTESIAN_POINT('Ctrl Pts',(161.97391706112,222.773351432123,10.4780191052983));
#89100=CARTESIAN_POINT('Ctrl Pts',(159.19999985714,222.133937861728,10.3192612400665));
#89101=CARTESIAN_POINT('Ctrl Pts',(157.158242752446,224.117544247575,10.1605033748347));
#89102=CARTESIAN_POINT('Ctrl Pts',(157.717261768964,226.908774103339,10.0017455096029));
#89103=CARTESIAN_POINT('Ctrl Pts',(160.365442724759,227.953093974789,9.84298764437114));
#89104=CARTESIAN_POINT('Ctrl Pts',(162.679170513225,226.294742356639,9.68422977913933));
#89105=CARTESIAN_POINT('Ctrl Pts',(162.540921553344,223.451442584608,9.52547191390755));
#89106=CARTESIAN_POINT('Ctrl Pts',(160.077221287761,222.025382498248,9.36671404867575));
#89107=CARTESIAN_POINT('Ctrl Pts',(157.542848102656,223.321692232518,9.20795618344397));
#89108=CARTESIAN_POINT('Ctrl Pts',(157.257260237375,226.153989169589,9.04919831821217));
#89109=CARTESIAN_POINT('Ctrl Pts',(159.481827694993,227.930155264032,8.89044045298037));
#89110=CARTESIAN_POINT('Ctrl Pts',(162.180626425776,227.024643376059,8.73168258774859));
#89111=CARTESIAN_POINT('Ctrl Pts',(162.88371593744,224.266177949933,8.57292472251679));
#89112=CARTESIAN_POINT('Ctrl Pts',(160.947628736558,222.179306435172,8.41416685728499));
#89113=CARTESIAN_POINT('Ctrl Pts',(158.144271753243,222.67393356002,8.25540899205321));
#89114=CARTESIAN_POINT('Ctrl Pts',(157.039277188385,225.297376599268,8.09665112682141));
#89115=CARTESIAN_POINT('Ctrl Pts',(158.643936024289,227.648660586559,7.93789326158962));
#89116=CARTESIAN_POINT('Ctrl Pts',(161.489664557439,227.575890509188,7.77913539635783));
#89117=CARTESIAN_POINT('Ctrl Pts',(162.9720521462,225.145665539102,7.62037753112604));
#89118=CARTESIAN_POINT('Ctrl Pts',(161.734417727632,222.582127473359,7.46161966589424));
#89119=CARTESIAN_POINT('Ctrl Pts',(158.90944427294,222.231426248916,7.30286180066245));
#89120=CARTESIAN_POINT('Ctrl Pts',(157.082547376768,224.414523612595,7.14410393543066));
#89121=CARTESIAN_POINT('Ctrl Pts',(157.925703006652,227.133448943003,6.98534607019887));
#89122=CARTESIAN_POINT('Ctrl Pts',(160.667255163279,227.899841884671,6.82658820496708));
#89123=CARTESIAN_POINT('Ctrl Pts',(162.798135420711,226.012299647521,6.66783033973528));
#89124=CARTESIAN_POINT('Ctrl Pts',(162.368162251143,223.198300812768,6.50907247450349));
#89125=CARTESIAN_POINT('Ctrl Pts',(159.770847082455,222.03321700332,6.3503146092717));
#89126=CARTESIAN_POINT('Ctrl Pts',(157.383252654892,223.583332875767,6.1915567440399));
#89127=CARTESIAN_POINT('Ctrl Pts',(157.390505294671,226.429982444603,6.03279887880811));
#89128=CARTESIAN_POINT('Ctrl Pts',(159.785967386151,227.967912136371,5.87404101357632));
#89129=CARTESIAN_POINT('Ctrl Pts',(162.377312117409,226.789608757643,5.71528314834453));
#89130=CARTESIAN_POINT('Ctrl Pts',(162.792940892299,223.973455514294,5.55652528311274));
#89131=CARTESIAN_POINT('Ctrl Pts',(160.652470272387,222.096795743895,5.39776741788094));
#89132=CARTESIAN_POINT('Ctrl Pts',(157.914858884844,222.877148394518,5.23900955264915));
#89133=CARTESIAN_POINT('Ctrl Pts',(157.085568563895,225.600334750998,5.08025168741735));
#89134=CARTESIAN_POINT('Ctrl Pts',(158.923565778663,227.774094766974,4.92149382218557));
#89135=CARTESIAN_POINT('Ctrl Pts',(161.746715550468,227.4090033613,4.76273595695377));
#89136=CARTESIAN_POINT('Ctrl Pts',(162.971271319174,224.839192174104,4.60397809172198));
#89137=CARTESIAN_POINT('Ctrl Pts',(161.476519693411,222.416552302829,4.44522022649019));
#89138=CARTESIAN_POINT('Ctrl Pts',(158.630457302308,222.358283662445,4.28646236125839));
#89139=CARTESIAN_POINT('Ctrl Pts',(157.037800334262,224.717713710242,4.1277044960266));
#89140=CARTESIAN_POINT('Ctrl Pts',(158.156148383844,227.335492159465,3.96894663079481));
#89141=CARTESIAN_POINT('Ctrl Pts',(160.96198935996,227.815828275895,3.81018876556302));
#89142=CARTESIAN_POINT('Ctrl Pts',(162.887417711804,225.719118465561,3.65143090033123));
#89143=CARTESIAN_POINT('Ctrl Pts',(162.170281487072,222.964271462568,3.49267303509943));
#89144=CARTESIAN_POINT('Ctrl Pts',(159.466903731292,222.072523139587,3.33391516986765));
#89145=CARTESIAN_POINT('Ctrl Pts',(157.251415658476,223.860001518727,3.17515730463585));
#89146=CARTESIAN_POINT('Ctrl Pts',(157.551431869414,226.69080647432,3.01639943940406));
#89147=CARTESIAN_POINT('Ctrl Pts',(160.092377532038,227.974185387821,2.85764157417226));
#89148=CARTESIAN_POINT('Ctrl Pts',(162.548779291636,226.535589999658,2.69888370894047));
#89149=CARTESIAN_POINT('Ctrl Pts',(162.672538321632,223.691622603948,2.54012584370868));
#89150=CARTESIAN_POINT('Ctrl Pts',(160.350390430673,222.045082357655,2.38136797847689));
#89151=CARTESIAN_POINT('Ctrl Pts',(157.707565136085,223.102882189851,2.22261011324509));
#89152=CARTESIAN_POINT('Ctrl Pts',(157.162776336452,225.8969250628,2.0638522480133));
#89153=CARTESIAN_POINT('Ctrl Pts',(159.214614112023,227.870100295438,1.90509438278151));
#89154=CARTESIAN_POINT('Ctrl Pts',(161.985237872319,227.216563705981,1.74633651754972));
#89155=CARTESIAN_POINT('Ctrl Pts',(162.938970244317,224.534420100273,1.58757865231793));
#89156=CARTESIAN_POINT('Ctrl Pts',(161.202960827807,222.278391799228,1.42882078708613));
#89157=CARTESIAN_POINT('Ctrl Pts',(158.365994107488,222.513144775438,1.27006292185434));
#89158=CARTESIAN_POINT('Ctrl Pts',(157.024485288296,225.023939017799,1.11130505662255));
#89159=CARTESIAN_POINT('Ctrl Pts',(158.406134689972,227.512675992633,0.952547191390755));
#89160=CARTESIAN_POINT('Ctrl Pts',(161.24655747117,227.702119660047,0.793789326158964));
#89161=CARTESIAN_POINT('Ctrl Pts',(162.945990077265,225.41794505403,0.635031460927171));
#89162=CARTESIAN_POINT('Ctrl Pts',(161.949545776539,222.752591178553,0.476273595695376));
#89163=CARTESIAN_POINT('Ctrl Pts',(159.16828253524,222.141301949138,0.317515730463587));
#89164=CARTESIAN_POINT('Ctrl Pts',(157.149564958546,224.151956510058,0.158757865231795));
#89165=CARTESIAN_POINT('Ctrl Pts',(157.542565484547,225.999756515378,0.0529192884105984));
#89166=CARTESIAN_POINT('Ctrl Pts',(158.086534003335,226.635987203375,0.));
#89167=CARTESIAN_POINT('Ctrl Pts',(158.086534003335,226.635987203375,0.));
#89168=CARTESIAN_POINT('Ctrl Pts',(158.02493814877,226.578102225091,3.88510873360859E-16));
#89169=CARTESIAN_POINT('Ctrl Pts',(157.966714247614,226.517065561656,3.25162993585481E-15));
#89170=CARTESIAN_POINT('Ctrl Pts',(157.911858668619,226.45326227157,2.88657986402541E-15));
#89171=CARTESIAN_POINT('Ctrl Pts',(157.855549069167,226.38776778998,2.51185365200075E-15));
#89172=CARTESIAN_POINT('Ctrl Pts',(157.802788287295,226.31935764003,1.57974842293527E-15));
#89173=CARTESIAN_POINT('Ctrl Pts',(157.753597957701,226.248399766245,4.16333634234434E-15));
#89174=CARTESIAN_POINT('Ctrl Pts',(157.70270970509,226.174992610086,6.83610303803933E-15));
#89175=CARTESIAN_POINT('Ctrl Pts',(157.655642062481,226.098858291382,5.567414283278E-15));
#89176=CARTESIAN_POINT('Ctrl Pts',(157.612453916939,226.020360183052,6.60582699651968E-15));
#89177=CARTESIAN_POINT('Ctrl Pts',(157.593559103265,225.986017260658,7.06013255856292E-15));
#89178=CARTESIAN_POINT('Ctrl Pts',(157.575407343554,225.951221387756,1.38955512833555E-15));
#89179=CARTESIAN_POINT('Ctrl Pts',(157.558006013615,225.91600090403,1.0547118733939E-15));
#89180=CARTESIAN_POINT('Ctrl Pts',(157.548478053374,225.896716207413,8.71371103972259E-16));
#89181=CARTESIAN_POINT('Ctrl Pts',(157.539175101023,225.877304191743,3.02150505445988E-15));
#89182=CARTESIAN_POINT('Ctrl Pts',(157.53009857257,225.857769379394,3.21964677141295E-15));
#89183=CARTESIAN_POINT('Ctrl Pts',(157.521442422622,225.839139319921,3.40861157460151E-15));
#89184=CARTESIAN_POINT('Ctrl Pts',(157.51298971229,225.820391557714,6.07713703975296E-15));
#89185=CARTESIAN_POINT('Ctrl Pts',(157.504755793001,225.801562868206,5.71764857681956E-15));
#89186=CARTESIAN_POINT('Ctrl Pts',(157.468216330129,225.718007251847,4.1223553897749E-15));
#89187=CARTESIAN_POINT('Ctrl Pts',(157.435936281972,225.632767982619,4.36828787014081E-15));
#89188=CARTESIAN_POINT('Ctrl Pts',(157.407939344588,225.546244309043,4.8017145815038E-15));
#89189=CARTESIAN_POINT('Ctrl Pts',(157.379477860582,225.458284968426,5.24233304072434E-15));
#89190=CARTESIAN_POINT('Ctrl Pts',(157.355442312615,225.368997490439,6.89313887191085E-16));
#89191=CARTESIAN_POINT('Ctrl Pts',(157.335896709461,225.278764189872,1.33226762955019E-15));
#89192=CARTESIAN_POINT('Ctrl Pts',(157.316694687441,225.190117049601,1.96391925071255E-15));
#89193=CARTESIAN_POINT('Ctrl Pts',(157.30182589002,225.100556136381,8.25976945391393E-15));
#89194=CARTESIAN_POINT('Ctrl Pts',(157.291393655264,225.010421131899,9.07607322631065E-15));
#89195=CARTESIAN_POINT('Ctrl Pts',(157.287259729619,224.974703817709,9.39954553855482E-15));
#89196=CARTESIAN_POINT('Ctrl Pts',(157.283822955362,224.938896175082,7.48833909922335E-15));
#89197=CARTESIAN_POINT('Ctrl Pts',(157.28109180216,224.903018802931,7.88258347483861E-15));
#89198=CARTESIAN_POINT('Ctrl Pts',(157.279473595435,224.881761480246,8.1161730441672E-15));
#89199=CARTESIAN_POINT('Ctrl Pts',(157.27810312366,224.860479674496,9.69815673100317E-15));
#89200=CARTESIAN_POINT('Ctrl Pts',(157.276982352986,224.839177647246,1.01030295240889E-14));
#89201=CARTESIAN_POINT('Ctrl Pts',(157.276240353188,224.825074762242,1.03710732353788E-14));
#89202=CARTESIAN_POINT('Ctrl Pts',(157.275607880765,224.810963101263,1.12280289430315E-14));
#89203=CARTESIAN_POINT('Ctrl Pts',(157.275085847944,224.796858298822,1.10467190950203E-14));
#89204=CARTESIAN_POINT('Ctrl Pts',(157.271562839589,224.701670151936,9.82312532148025E-15));
#89205=CARTESIAN_POINT('Ctrl Pts',(157.273056577644,224.606632807943,6.53173546723879E-15));
#89206=CARTESIAN_POINT('Ctrl Pts',(157.279625133053,224.512145564813,7.105427357601E-15));
#89207=CARTESIAN_POINT('Ctrl Pts',(157.286171954436,224.417970960931,7.6772210170925E-15));
#89208=CARTESIAN_POINT('Ctrl Pts',(157.29775970648,224.324341869061,8.22264820408673E-15));
#89209=CARTESIAN_POINT('Ctrl Pts',(157.314493894775,224.231635735225,9.79771819231701E-15));
#89210=CARTESIAN_POINT('Ctrl Pts',(157.316398182771,224.221086124168,9.97695526191135E-15));
#89211=CARTESIAN_POINT('Ctrl Pts',(157.318369169726,224.210548454971,6.40383101223916E-15));
#89212=CARTESIAN_POINT('Ctrl Pts',(157.320407053956,224.200023277725,6.38378239159465E-15));
#89213=CARTESIAN_POINT('Ctrl Pts',(157.337940261685,224.109468516937,6.21335718039711E-15));
#89214=CARTESIAN_POINT('Ctrl Pts',(157.360420988526,224.019838133689,1.13008504771569E-14));
#89215=CARTESIAN_POINT('Ctrl Pts',(157.387574332193,223.931369727859,1.29896093881143E-14));
#89216=CARTESIAN_POINT('Ctrl Pts',(157.398274583748,223.896507200109,1.36550944711156E-14));
#89217=CARTESIAN_POINT('Ctrl Pts',(157.40970101855,223.861825165636,7.03342696341441E-15));
#89218=CARTESIAN_POINT('Ctrl Pts',(157.421838980151,223.827338502461,7.41073868937292E-15));
#89219=CARTESIAN_POINT('Ctrl Pts',(157.427149340729,223.812250580568,7.57581264337371E-15));
#89220=CARTESIAN_POINT('Ctrl Pts',(157.432595907216,223.79720005763,6.38525469805514E-15));
#89221=CARTESIAN_POINT('Ctrl Pts',(157.438177521516,223.782188198706,6.32827124036339E-15));
#89222=CARTESIAN_POINT('Ctrl Pts',(157.442598261446,223.770298533707,6.28313930661066E-15));
#89223=CARTESIAN_POINT('Ctrl Pts',(157.447103314523,223.75843433437,5.8191034780375E-15));
#89224=CARTESIAN_POINT('Ctrl Pts',(157.451688373109,223.746605388579,6.07847105982273E-15));
#89225=CARTESIAN_POINT('Ctrl Pts',(157.485446723974,223.659512564152,7.98811336120978E-15));
#89226=CARTESIAN_POINT('Ctrl Pts',(157.523588046527,223.574194570567,1.3532532634904E-14));
#89227=CARTESIAN_POINT('Ctrl Pts',(157.565779073504,223.490882142242,1.33643096589253E-14));
#89228=CARTESIAN_POINT('Ctrl Pts',(157.609552429182,223.404445171664,1.31897776627071E-14));
#89229=CARTESIAN_POINT('Ctrl Pts',(157.657685066682,223.320166301312,1.07282401440124E-14));
#89230=CARTESIAN_POINT('Ctrl Pts',(157.709860882353,223.238306243802,1.13520304267922E-14));
#89231=CARTESIAN_POINT('Ctrl Pts',(157.762638398375,223.15550216223,1.19830143648678E-14));
#89232=CARTESIAN_POINT('Ctrl Pts',(157.819553294228,223.075172188621,1.73211728058691E-14));
#89233=CARTESIAN_POINT('Ctrl Pts',(157.88033030919,222.99760095645,1.5931700403371E-14));
#89234=CARTESIAN_POINT('Ctrl Pts',(157.92312949277,222.942975282447,1.495323371707E-14));
#89235=CARTESIAN_POINT('Ctrl Pts',(157.967844993907,222.889717949271,1.86083952223982E-14));
#89236=CARTESIAN_POINT('Ctrl Pts',(158.014394107949,222.83793607413,1.92346139016308E-14));
#89237=CARTESIAN_POINT('Ctrl Pts',(158.025600423893,222.825470014036,1.9385370892694E-14));
#89238=CARTESIAN_POINT('Ctrl Pts',(158.036913653601,222.81308897035,1.06179758662295E-14));
#89239=CARTESIAN_POINT('Ctrl Pts',(158.048321402091,222.800806370086,1.10883524584438E-14));
#89240=CARTESIAN_POINT('Ctrl Pts',(158.116987698191,222.726874106645,1.39196752552947E-14));
#89241=CARTESIAN_POINT('Ctrl Pts',(158.189166938781,222.656402926642,2.01694406300404E-14));
#89242=CARTESIAN_POINT('Ctrl Pts',(158.26454599322,222.589679804418,1.73125402902485E-14));
#89243=CARTESIAN_POINT('Ctrl Pts',(158.329365962863,222.532303245515,1.48558340516762E-14));
#89244=CARTESIAN_POINT('Ctrl Pts',(158.396553121545,222.477698163774,1.06264985383864E-14));
#89245=CARTESIAN_POINT('Ctrl Pts',(158.465934582306,222.426062335657,8.84015083357781E-15));
#89246=CARTESIAN_POINT('Ctrl Pts',(158.491454268484,222.407069796228,8.1831016401346E-15));
#89247=CARTESIAN_POINT('Ctrl Pts',(158.517271035126,222.38847913505,6.96638787698447E-15));
#89248=CARTESIAN_POINT('Ctrl Pts',(158.543376988089,222.370300845808,5.81479309147426E-15));
#89249=CARTESIAN_POINT('Ctrl Pts',(158.560069502231,222.358677391546,5.07844716031687E-15));
#89250=CARTESIAN_POINT('Ctrl Pts',(158.576881299093,222.347221964069,1.4774855333679E-14));
#89251=CARTESIAN_POINT('Ctrl Pts',(158.593795529517,222.335946953852,1.42247325030098E-14));
#89252=CARTESIAN_POINT('Ctrl Pts',(158.679989199738,222.278490333717,1.14213471488789E-14));
#89253=CARTESIAN_POINT('Ctrl Pts',(158.768924528117,222.225655835067,3.46784439453926E-15));
#89254=CARTESIAN_POINT('Ctrl Pts',(158.860295151837,222.17776281636,2.90739654573713E-15));
#89255=CARTESIAN_POINT('Ctrl Pts',(158.951665775557,222.129869797652,2.346948696935E-15));
#89256=CARTESIAN_POINT('Ctrl Pts',(159.045472333248,222.086917356743,2.82861414654592E-16));
#89257=CARTESIAN_POINT('Ctrl Pts',(159.141446275838,222.049265302153,-1.79847456371895E-15));
#89258=CARTESIAN_POINT('Ctrl Pts',(159.162330716112,222.04107201485,-2.25850751576755E-15));
#89259=CARTESIAN_POINT('Ctrl Pts',(159.183317907923,222.033129893401,-3.50002483407811E-15));
#89260=CARTESIAN_POINT('Ctrl Pts',(159.204403756968,222.025437709964,-3.71924713249427E-15));
#89261=CARTESIAN_POINT('Ctrl Pts',(157.485690591028,225.001427433753,19.112583302492));
#89262=CARTESIAN_POINT('Ctrl Pts',(157.484001218019,225.327429254226,19.092036810933));
#89263=CARTESIAN_POINT('Ctrl Pts',(157.542838162647,225.652846145079,19.071490319374));
#89264=CARTESIAN_POINT('Ctrl Pts',(157.665030210741,225.952420038454,19.0509438278151));
#89265=CARTESIAN_POINT('Ctrl Pts',(157.979746531824,226.723998836627,18.9980245394045));
#89266=CARTESIAN_POINT('Ctrl Pts',(158.714738521617,227.32414419925,18.9451052509939));
#89267=CARTESIAN_POINT('Ctrl Pts',(159.533660651586,227.478241959391,18.8921859625833));
#89268=CARTESIAN_POINT('Ctrl Pts',(160.352582781555,227.632339719532,18.8392666741727));
#89269=CARTESIAN_POINT('Ctrl Pts',(161.255435051699,227.340389877191,18.7863473857621));
#89270=CARTESIAN_POINT('Ctrl Pts',(161.829078646719,226.735982727646,18.7334280973515));
#89271=CARTESIAN_POINT('Ctrl Pts',(162.402722241738,226.131575578101,18.6805088089409));
#89272=CARTESIAN_POINT('Ctrl Pts',(162.647157161632,225.214711121351,18.6275895205303));
#89273=CARTESIAN_POINT('Ctrl Pts',(162.450526923907,224.404949380834,18.5746702321197));
#89274=CARTESIAN_POINT('Ctrl Pts',(162.253896686182,223.595187640316,18.5217509437091));
#89275=CARTESIAN_POINT('Ctrl Pts',(161.616201290837,222.892528616031,18.4688316552985));
#89276=CARTESIAN_POINT('Ctrl Pts',(160.829251616835,222.618507682391,18.4159123668879));
#89277=CARTESIAN_POINT('Ctrl Pts',(160.042301942833,222.344486748751,18.3629930784773));
#89278=CARTESIAN_POINT('Ctrl Pts',(159.106097990172,222.499103905755,18.3100737900667));
#89279=CARTESIAN_POINT('Ctrl Pts',(158.449045956583,223.011607011104,18.2571545016561));
#89280=CARTESIAN_POINT('Ctrl Pts',(157.850708354407,223.478312634838,18.2089641019347));
#89281=CARTESIAN_POINT('Ctrl Pts',(157.483861524418,224.241800364934,18.1607737022134));
#89282=CARTESIAN_POINT('Ctrl Pts',(157.479093530148,225.001296842243,18.112583302492));
#89283=CARTESIAN_POINT('Origin',(0.,225.,22.2084234471774));
#89284=CARTESIAN_POINT('Ctrl Pts',(-3.07632864029364,225.002216919788,19.7084234471775));
#89285=CARTESIAN_POINT('Ctrl Pts',(-3.07751543998229,225.146316230092,19.7009407276991));
#89286=CARTESIAN_POINT('Ctrl Pts',(-3.002794304667,226.308308938777,19.6405387198101));
#89287=CARTESIAN_POINT('Ctrl Pts',(-1.52182622034608,228.298871155631,19.5272174235105));
#89288=CARTESIAN_POINT('Ctrl Pts',(1.94583867854751,228.067542026651,19.3684595582787));
#89289=CARTESIAN_POINT('Ctrl Pts',(3.63261192033118,225.029235473214,19.2097016930469));
#89290=CARTESIAN_POINT('Ctrl Pts',(1.99484850327397,221.96395749968,19.0509438278151));
#89291=CARTESIAN_POINT('Ctrl Pts',(-1.46861477289244,221.67737141594,18.8921859625833));
#89292=CARTESIAN_POINT('Ctrl Pts',(-2.99280343380595,223.658124429256,18.7780125023708));
#89293=CARTESIAN_POINT('Ctrl Pts',(-3.07726971933124,224.836966997831,18.7167583305688));
#89294=CARTESIAN_POINT('Ctrl Pts',(-3.07588051624417,224.997572007392,18.7084234471775));
#89295=CARTESIAN_POINT('Ctrl Pts',(-3.07038312444426,224.996706709974,19.7915765528225));
#89296=CARTESIAN_POINT('Ctrl Pts',(-3.06508366964555,225.700112229625,19.7552124583938));
#89297=CARTESIAN_POINT('Ctrl Pts',(-2.47776202454432,227.437543589317,19.6659290755545));
#89298=CARTESIAN_POINT('Ctrl Pts',(0.407268901123991,228.609154817042,19.5237264043046));
#89299=CARTESIAN_POINT('Ctrl Pts',(3.25295011294267,226.616814793291,19.3649685390728));
#89300=CARTESIAN_POINT('Ctrl Pts',(3.12275731293263,223.14341933887,19.206210673841));
#89301=CARTESIAN_POINT('Ctrl Pts',(0.134013646578404,221.369829208712,19.0474528086092));
#89302=CARTESIAN_POINT('Ctrl Pts',(-2.57444317314689,222.717848478559,18.9092414349364));
#89303=CARTESIAN_POINT('Ctrl Pts',(-3.06630351957984,224.374665598836,18.8239493496742));
#89304=CARTESIAN_POINT('Ctrl Pts',(-3.06955363737172,225.001741577652,18.7915765528225));
#89305=CARTESIAN_POINT('Ctrl Pts',(1.91346599666507,226.635987203375,20.));
#89306=CARTESIAN_POINT('Ctrl Pts',(2.45743451545281,225.999756515378,19.9470807115894));
#89307=CARTESIAN_POINT('Ctrl Pts',(2.85075747508451,224.152305503521,19.8412421347682));
#89308=CARTESIAN_POINT('Ctrl Pts',(0.831598276500719,222.14123234529,19.6824842695364));
#89309=CARTESIAN_POINT('Ctrl Pts',(-1.94946050932766,222.75270577452,19.5237264043046));
#89310=CARTESIAN_POINT('Ctrl Pts',(-2.9459653310193,225.417892776033,19.3649685390728));
#89311=CARTESIAN_POINT('Ctrl Pts',(-1.24652595077964,227.702101231267,19.206210673841));
#89312=CARTESIAN_POINT('Ctrl Pts',(1.59383402415598,227.512619831493,19.0474528086093));
#89313=CARTESIAN_POINT('Ctrl Pts',(2.97546787357532,225.023946739488,18.8886949433774));
#89314=CARTESIAN_POINT('Ctrl Pts',(1.63397791019756,222.513181391067,18.7299370781457));
#89315=CARTESIAN_POINT('Ctrl Pts',(-1.20294052082536,222.278439088866,18.5711792129139));
#89316=CARTESIAN_POINT('Ctrl Pts',(-2.93892195162375,224.5344265124,18.4124213476821));
#89317=CARTESIAN_POINT('Ctrl Pts',(-1.9852050243123,227.216527803386,18.2536634824503));
#89318=CARTESIAN_POINT('Ctrl Pts',(0.785372889255974,227.870052581747,18.0949056172185));
#89319=CARTESIAN_POINT('Ctrl Pts',(2.83717686333081,225.896910448037,17.9361477519867));
#89320=CARTESIAN_POINT('Ctrl Pts',(2.29239702935025,223.102913397598,17.7773898867549));
#89321=CARTESIAN_POINT('Ctrl Pts',(-0.350384645949477,222.04513116686,17.6186320215231));
#89322=CARTESIAN_POINT('Ctrl Pts',(-2.67249422325434,223.691644167573,17.4598741562913));
#89323=CARTESIAN_POINT('Ctrl Pts',(-2.54873723378948,226.535564674241,17.3011162910595));
#89324=CARTESIAN_POINT('Ctrl Pts',(-0.0923760078729938,227.974136303935,
17.1423584258278));
#89325=CARTESIAN_POINT('Ctrl Pts',(2.44852772681453,226.690778577842,16.9836005605959));
#89326=CARTESIAN_POINT('Ctrl Pts',(2.74853898713179,223.860020328042,16.8248426953642));
#89327=CARTESIAN_POINT('Ctrl Pts',(0.533087472085183,222.072571446793,16.6660848301324));
#89328=CARTESIAN_POINT('Ctrl Pts',(-2.17024567525691,222.964305053653,16.5073269649006));
#89329=CARTESIAN_POINT('Ctrl Pts',(-2.88737006653445,225.719106599626,16.3485690996688));
#89330=CARTESIAN_POINT('Ctrl Pts',(-0.961973486173353,227.815781811798,
16.189811234437));
#89331=CARTESIAN_POINT('Ctrl Pts',(1.84382119076242,227.335453621575,16.0310533692052));
#89332=CARTESIAN_POINT('Ctrl Pts',(2.96215078648909,224.717718368216,15.8722955039734));
#89333=CARTESIAN_POINT('Ctrl Pts',(1.36952009887017,222.358327253417,15.7135376387416));
#89334=CARTESIAN_POINT('Ctrl Pts',(-1.47649532936267,222.416594932285,15.5547797735098));
#89335=CARTESIAN_POINT('Ctrl Pts',(-2.97122229023292,224.839194827597,15.396021908278));
#89336=CARTESIAN_POINT('Ctrl Pts',(-1.74668672791837,227.408963610339,15.2372640430462));
#89337=CARTESIAN_POINT('Ctrl Pts',(1.07641645909825,227.774048991643,15.0785061778144));
#89338=CARTESIAN_POINT('Ctrl Pts',(2.91438334507821,225.600324844875,14.9197483125826));
#89339=CARTESIAN_POINT('Ctrl Pts',(2.08510670824745,222.877183423688,14.7609904473508));
#89340=CARTESIAN_POINT('Ctrl Pts',(-0.652459505976317,222.096843649662,
14.6022325821191));
#89341=CARTESIAN_POINT('Ctrl Pts',(-2.79289480598801,223.973472453302,14.4434747168873));
#89342=CARTESIAN_POINT('Ctrl Pts',(-2.37727288938734,226.789579227313,14.2847168516555));
#89343=CARTESIAN_POINT('Ctrl Pts',(0.214029082096596,227.96786316286,14.1259589864237));
#89344=CARTESIAN_POINT('Ctrl Pts',(2.60945164606224,226.429958848466,13.9672011211919));
#89345=CARTESIAN_POINT('Ctrl Pts',(2.61670416616591,223.583356252188,13.8084432559601));
#89346=CARTESIAN_POINT('Ctrl Pts',(0.229149136293932,222.033265958199,13.6496853907283));
#89347=CARTESIAN_POINT('Ctrl Pts',(-2.36812317410319,223.198330542602,13.4909275254965));
#89348=CARTESIAN_POINT('Ctrl Pts',(-2.79808924868524,226.012282943567,13.3321696602647));
#89349=CARTESIAN_POINT('Ctrl Pts',(-0.667244152902773,227.899794034386,
13.1734117950329));
#89350=CARTESIAN_POINT('Ctrl Pts',(2.07426276537758,227.133413738967,13.0146539298011));
#89351=CARTESIAN_POINT('Ctrl Pts',(2.91740448235278,224.41453327354,12.8558960645693));
#89352=CARTESIAN_POINT('Ctrl Pts',(1.09053773180285,222.231471933146,12.6971381993376));
#89353=CARTESIAN_POINT('Ctrl Pts',(-1.73438910800869,222.582167370667,12.5383803341058));
#89354=CARTESIAN_POINT('Ctrl Pts',(-2.97200310437387,225.145663135475,12.379622468874));
#89355=CARTESIAN_POINT('Ctrl Pts',(-1.48963997648728,227.575848004424,12.2208646036422));
#89356=CARTESIAN_POINT('Ctrl Pts',(1.35604159930179,227.648616881017,12.0621067384104));
#89357=CARTESIAN_POINT('Ctrl Pts',(2.96067395673492,225.297371692257,11.9033488731786));
#89358=CARTESIAN_POINT('Ctrl Pts',(1.85569762538991,222.673971942438,11.7445910079468));
#89359=CARTESIAN_POINT('Ctrl Pts',(-0.947613099738392,222.17935297943,11.585833142715));
#89360=CARTESIAN_POINT('Ctrl Pts',(-2.8836683532501,224.266190058729,11.4270752774832));
#89361=CARTESIAN_POINT('Ctrl Pts',(-2.18059044326484,227.024609967423,11.2683174122514));
#89362=CARTESIAN_POINT('Ctrl Pts',(0.518163754646772,227.930106913546,11.1095595470196));
#89363=CARTESIAN_POINT('Ctrl Pts',(2.74269450468196,226.153970127617,10.9508016817878));
#89364=CARTESIAN_POINT('Ctrl Pts',(2.45711135188605,223.321719926271,10.792043816556));
#89365=CARTESIAN_POINT('Ctrl Pts',(-0.0772200135324106,222.025431582405,
10.6332859513243));
#89366=CARTESIAN_POINT('Ctrl Pts',(-2.5408796256026,223.45146813735,10.4745280860925));
#89367=CARTESIAN_POINT('Ctrl Pts',(-2.67912630423898,226.294720992098,10.3157702208607));
#89368=CARTESIAN_POINT('Ctrl Pts',(-0.365436694589916,227.953045245792,
10.1570123556289));
#89369=CARTESIAN_POINT('Ctrl Pts',(2.28270056357738,226.908742606662,9.99825449039707));
#89370=CARTESIAN_POINT('Ctrl Pts',(2.84171035572368,224.117558808975,9.83949662516529));
#89371=CARTESIAN_POINT('Ctrl Pts',(0.799986942059197,222.133985154613,9.68073875993349));
#89372=CARTESIAN_POINT('Ctrl Pts',(-1.97388448951912,222.773388174046,9.5219808947017));
#89373=CARTESIAN_POINT('Ctrl Pts',(-2.94125691391068,225.450586249032,9.36322302946991));
#89374=CARTESIAN_POINT('Ctrl Pts',(-1.21679112635331,227.715407806623,9.20446516423812));
#89375=CARTESIAN_POINT('Ctrl Pts',(1.62128185219347,227.495088246374,9.04570729900632));
#89376=CARTESIAN_POINT('Ctrl Pts',(2.97555774336814,224.99126402116,8.88694943377453));
#89377=CARTESIAN_POINT('Ctrl Pts',(1.60660330482325,222.495434963437,8.72819156854274));
#89378=CARTESIAN_POINT('Ctrl Pts',(-1.23271441511773,222.291783728687,8.56943370331094));
#89379=CARTESIAN_POINT('Ctrl Pts',(-2.94385195081828,224.566691918945,8.41067583807916));
#89380=CARTESIAN_POINT('Ctrl Pts',(-1.96077629689413,227.238163647945,8.25191797284736));
#89381=CARTESIAN_POINT('Ctrl Pts',(0.816801746841883,227.861268094359,8.09316010761557));
#89382=CARTESIAN_POINT('Ctrl Pts',(2.84684286398815,225.865740093333,7.93440224238377));
#89383=CARTESIAN_POINT('Ctrl Pts',(2.27145350396183,223.077886792932,7.77564437715199));
#89384=CARTESIAN_POINT('Ctrl Pts',(-0.38277001356761,222.049151424055,7.61688651192019));
#89385=CARTESIAN_POINT('Ctrl Pts',(-2.68668242973203,223.721032555843,7.45812864668841));
#89386=CARTESIAN_POINT('Ctrl Pts',(-2.53174319185694,226.563424642229,7.2993707814566));
#89387=CARTESIAN_POINT('Ctrl Pts',(-0.0597526843527511,227.974970557528,
7.14061291622481));
#89388=CARTESIAN_POINT('Ctrl Pts',(2.46692347752136,226.663823535564,6.98185505099302));
#89389=CARTESIAN_POINT('Ctrl Pts',(2.73587136977733,223.829945279281,6.82309718576122));
#89390=CARTESIAN_POINT('Ctrl Pts',(0.500949891998614,222.066901057388,6.66433932052944));
#89391=CARTESIAN_POINT('Ctrl Pts',(-2.19244090723784,222.988228872432,6.50558145529764));
#89392=CARTESIAN_POINT('Ctrl Pts',(-2.87930987438589,225.750729544315,6.34682359006585));
#89393=CARTESIAN_POINT('Ctrl Pts',(-0.931034557722079,227.826162566763,
6.18806572483406));
#89394=CARTESIAN_POINT('Ctrl Pts',(1.86932354955694,227.315091719245,6.02930785960227));
#89395=CARTESIAN_POINT('Ctrl Pts',(2.95887681779079,224.685249021313,5.87054999437047));
#89396=CARTESIAN_POINT('Ctrl Pts',(1.34046613873754,222.343466406698,5.71179212913869));
#89397=CARTESIAN_POINT('Ctrl Pts',(-1.50473909777578,222.432943232208,5.55303426390689));
#89398=CARTESIAN_POINT('Ctrl Pts',(-2.97280717117708,224.871790310653,5.3942763986751));
#89399=CARTESIAN_POINT('Ctrl Pts',(-1.72016223842006,227.427974891748,5.23551853344331));
#89400=CARTESIAN_POINT('Ctrl Pts',(1.10677510729556,227.762076947392,5.07676066821151));
#89401=CARTESIAN_POINT('Ctrl Pts',(2.92079191833656,225.568326289399,4.91800280297972));
#89402=CARTESIAN_POINT('Ctrl Pts',(2.06170008057449,222.854443433697,4.75924493774793));
#89403=CARTESIAN_POINT('Ctrl Pts',(-0.68425958985738,222.104173863102,4.60048707251613));
#89404=CARTESIAN_POINT('Ctrl Pts',(-2.80398491055471,224.004164259125,4.44172920728435));
#89405=CARTESIAN_POINT('Ctrl Pts',(-2.35750335138642,226.815543486026,4.28297134205255));
#89406=CARTESIAN_POINT('Ctrl Pts',(0.24656518228451,227.965337385933,4.12421347682076));
#89407=CARTESIAN_POINT('Ctrl Pts',(2.62497727078325,226.401254626798,3.96545561158896));
#89408=CARTESIAN_POINT('Ctrl Pts',(2.60101026436985,223.554743688413,3.80669774635717));
#89409=CARTESIAN_POINT('Ctrl Pts',(0.196598766116914,222.030931269372,3.64793988112538));
#89410=CARTESIAN_POINT('Ctrl Pts',(-2.38773991480887,223.224410436226,3.48918201589359));
#89411=CARTESIAN_POINT('Ctrl Pts',(-2.78681912030052,226.042909101251,3.33042415066179));
#89412=CARTESIAN_POINT('Ctrl Pts',(-0.635401575053557,227.90693739939,3.17166628543));
#89413=CARTESIAN_POINT('Ctrl Pts',(2.09753546379433,227.110536700736,3.01290842019821));
#89414=CARTESIAN_POINT('Ctrl Pts',(2.91080813455441,224.38257290303,2.85415055496642));
#89415=CARTESIAN_POINT('Ctrl Pts',(1.06010930306564,222.219678347057,2.69539268973462));
#89416=CARTESIAN_POINT('Ctrl Pts',(-1.76080149659037,222.6013340852,2.53663482450284));
#89417=CARTESIAN_POINT('Ctrl Pts',(-2.97022688518523,225.178248720063,2.37787695927104));
#89418=CARTESIAN_POINT('Ctrl Pts',(-1.46130064497296,227.592030243376,2.21911909403925));
#89419=CARTESIAN_POINT('Ctrl Pts',(1.38500768436501,227.633585566377,2.06036122880745));
#89420=CARTESIAN_POINT('Ctrl Pts',(2.96375744914242,225.264883936543,1.90160336357567));
#89421=CARTESIAN_POINT('Ctrl Pts',(1.83007567274748,222.6537596164,1.74284549834387));
#89422=CARTESIAN_POINT('Ctrl Pts',(-0.978489580748851,222.189916275707,
1.58408763311209));
#89423=CARTESIAN_POINT('Ctrl Pts',(-2.89154467470074,224.297857645524,1.42532976788028));
#89424=CARTESIAN_POINT('Ctrl Pts',(-2.15825115583635,227.048407395618,1.2665719026485));
#89425=CARTESIAN_POINT('Ctrl Pts',(0.550259436798537,227.924239087672,1.1078140374167));
#89426=CARTESIAN_POINT('Ctrl Pts',(2.75520165707748,226.123839149338,0.94905617218491));
#89427=CARTESIAN_POINT('Ctrl Pts',(2.43852444180769,223.294836940432,0.790298306953122));
#89428=CARTESIAN_POINT('Ctrl Pts',(-0.10977043955631,222.026531358032,0.631540441721324));
#89429=CARTESIAN_POINT('Ctrl Pts',(-2.55784675572612,223.479277150759,0.472782576489534));
#89430=CARTESIAN_POINT('Ctrl Pts',(-2.66448757984816,226.324330789744,0.314024711257741));
#89431=CARTESIAN_POINT('Ctrl Pts',(-0.33359347540508,227.956254895383,0.155266846025945));
#89432=CARTESIAN_POINT('Ctrl Pts',(2.30464641624464,226.884864210807,-0.00349101920584165));
#89433=CARTESIAN_POINT('Ctrl Pts',(2.82948413440186,224.083799326414,-0.162248884437639));
#89434=CARTESIAN_POINT('Ctrl Pts',(1.45887298303089,222.784105799646,-0.268087461258832));
#89435=CARTESIAN_POINT('Ctrl Pts',(0.65019999797512,222.567913197965,-0.32100674966943));
#89436=CARTESIAN_POINT('Ctrl Pts',(2.0543315503421,226.756425321227,20.1070022498898));
#89437=CARTESIAN_POINT('Ctrl Pts',(2.63834594750733,226.073356597808,20.0540829614792));
#89438=CARTESIAN_POINT('Ctrl Pts',(3.06062455964552,224.089899923906,19.948244384658));
#89439=CARTESIAN_POINT('Ctrl Pts',(0.892818884476147,221.930775567268,19.7894865194262));
#89440=CARTESIAN_POINT('Ctrl Pts',(-2.0929759073,222.587264451862,19.6307286541944));
#89441=CARTESIAN_POINT('Ctrl Pts',(-3.16284142821185,225.448657209463,19.4719707889627));
#89442=CARTESIAN_POINT('Ctrl Pts',(-1.33829270730179,227.901024539389,19.3132129237308));
#89443=CARTESIAN_POINT('Ctrl Pts',(1.71116890895316,227.697593896546,19.1544550584991));
#89444=CARTESIAN_POINT('Ctrl Pts',(3.19451588916061,225.02570965073,18.9956971932673));
#89445=CARTESIAN_POINT('Ctrl Pts',(1.75426810788969,222.330106760605,18.8369393280355));
#89446=CARTESIAN_POINT('Ctrl Pts',(-1.29149860484772,222.078083197891,18.6781814628037));
#89447=CARTESIAN_POINT('Ctrl Pts',(-3.15527952926067,224.50015192,18.5194235975719));
#89448=CARTESIAN_POINT('Ctrl Pts',(-2.1313518622491,227.379704163357,18.3606657323401));
#89449=CARTESIAN_POINT('Ctrl Pts',(0.843190476336583,228.081340133611,18.2019078671083));
#89450=CARTESIAN_POINT('Ctrl Pts',(3.04604417031683,225.962939207932,18.0431500018765));
#89451=CARTESIAN_POINT('Ctrl Pts',(2.46115873055101,222.963253662288,17.8843921366447));
#89452=CARTESIAN_POINT('Ctrl Pts',(-0.376179265366609,221.827599611583,
17.7256342714129));
#89453=CARTESIAN_POINT('Ctrl Pts',(-2.86923792244393,223.595325618373,17.5668764061811));
#89454=CARTESIAN_POINT('Ctrl Pts',(-2.73637019002741,226.648609885612,17.4081185409494));
#89455=CARTESIAN_POINT('Ctrl Pts',(-0.0991765454933055,228.193086292017,
17.2493606757175));
#89456=CARTESIAN_POINT('Ctrl Pts',(2.62878345883821,226.815250327498,17.0906028104858));
#89457=CARTESIAN_POINT('Ctrl Pts',(2.9508809503023,223.77609729625,16.931844945254));
#89458=CARTESIAN_POINT('Ctrl Pts',(0.572332309487286,221.857059990244,16.7730870800222));
#89459=CARTESIAN_POINT('Ctrl Pts',(-2.33001483718247,222.814441248269,16.6143292147904));
#89460=CARTESIAN_POINT('Ctrl Pts',(-3.09993249711944,225.772045794514,16.4555713495586));
#89461=CARTESIAN_POINT('Ctrl Pts',(-1.0327920572839,228.023074057724,16.2968134843268));
#89462=CARTESIAN_POINT('Ctrl Pts',(1.97955963261133,227.507385063296,16.138055619095));
#89463=CARTESIAN_POINT('Ctrl Pts',(3.18021842466029,224.696937356992,15.9792977538632));
#89464=CARTESIAN_POINT('Ctrl Pts',(1.47034143948213,222.163852569921,15.8205398886314));
#89465=CARTESIAN_POINT('Ctrl Pts',(-1.58519197327205,222.226409799197,15.6617820233996));
#89466=CARTESIAN_POINT('Ctrl Pts',(-3.18995775443279,224.827356671244,15.5030241581678));
#89467=CARTESIAN_POINT('Ctrl Pts',(-1.87527432417426,227.586306710948,15.344266292936));
#89468=CARTESIAN_POINT('Ctrl Pts',(1.15566009382299,227.978268950512,15.1855084277043));
#89469=CARTESIAN_POINT('Ctrl Pts',(3.12893443939975,225.644519563677,15.0267505624724));
#89470=CARTESIAN_POINT('Ctrl Pts',(2.2386081090797,222.720905897514,14.8679926972407));
#89471=CARTESIAN_POINT('Ctrl Pts',(-0.70049227463872,221.883119064321,14.7092348320089));
#89472=CARTESIAN_POINT('Ctrl Pts',(-2.99850215615409,223.897901540894,14.5504769667771));
#89473=CARTESIAN_POINT('Ctrl Pts',(-2.55228298227041,226.921324483901,14.3917191015453));
#89474=CARTESIAN_POINT('Ctrl Pts',(0.229785476621013,228.186351334796,14.2329612363135));
#89475=CARTESIAN_POINT('Ctrl Pts',(2.801554276345,226.535229569386,14.0742033710817));
#89476=CARTESIAN_POINT('Ctrl Pts',(2.80934071252649,223.479065762445,13.9154455058499));
#89477=CARTESIAN_POINT('Ctrl Pts',(0.246018639078369,221.814860909905,13.7566876406181));
#89478=CARTESIAN_POINT('Ctrl Pts',(-2.54245968317983,223.065695227367,13.5979297753863));
#89479=CARTESIAN_POINT('Ctrl Pts',(-3.00407900337164,226.086805196678,13.4391719101545));
#89480=CARTESIAN_POINT('Ctrl Pts',(-0.716365337810284,228.113271092727,
13.2804140449227));
#89481=CARTESIAN_POINT('Ctrl Pts',(2.22696585674466,227.290471407138,13.1216561796909));
#89482=CARTESIAN_POINT('Ctrl Pts',(3.13217798678021,224.371432379807,12.9628983144591));
#89483=CARTESIAN_POINT('Ctrl Pts',(1.17082094648441,222.027658413759,12.8041404492274));
#89484=CARTESIAN_POINT('Ctrl Pts',(-1.86207137799251,222.404171350554,12.6453825839956));
#89485=CARTESIAN_POINT('Ctrl Pts',(-3.19079605055485,225.156386565244,12.4866247187638));
#89486=CARTESIAN_POINT('Ctrl Pts',(-1.59930430312442,227.765476801572,12.327866853532));
#89487=CARTESIAN_POINT('Ctrl Pts',(1.45587067963436,227.843602777852,12.1691089883002));
#89488=CARTESIAN_POINT('Ctrl Pts',(3.17863287364251,225.319263603663,12.0103511230684));
#89489=CARTESIAN_POINT('Ctrl Pts',(1.99231038668972,222.502734391957,11.8515932578366));
#89490=CARTESIAN_POINT('Ctrl Pts',(-1.01737448781578,221.971702566529,11.6928353926048));
#89491=CARTESIAN_POINT('Ctrl Pts',(-3.09595827107957,224.212168433128,11.534077527373));
#89492=CARTESIAN_POINT('Ctrl Pts',(-2.34112116639695,227.173657718748,11.3753196621412));
#89493=CARTESIAN_POINT('Ctrl Pts',(0.556309937709806,228.145815545646,11.2165617969094));
#89494=CARTESIAN_POINT('Ctrl Pts',(2.94460620870091,226.238923108876,11.0578039316776));
#89495=CARTESIAN_POINT('Ctrl Pts',(2.63799899328275,223.198168291581,10.8990460664458));
#89496=CARTESIAN_POINT('Ctrl Pts',(-0.0829047970509779,221.806449782977,
10.7402882012141));
#89497=CARTESIAN_POINT('Ctrl Pts',(-2.7279341203838,223.337468307408,10.5815303359823));
#89498=CARTESIAN_POINT('Ctrl Pts',(-2.8763582440148,226.390035771523,10.4227724707505));
#89499=CARTESIAN_POINT('Ctrl Pts',(-0.392339415833482,228.170442552201,
10.2640146055187));
#89500=CARTESIAN_POINT('Ctrl Pts',(2.45074843029026,227.04926043378,10.1052567402869));
#89501=CARTESIAN_POINT('Ctrl Pts',(3.05091140938569,224.052595246948,9.9464988750551));
#89502=CARTESIAN_POINT('Ctrl Pts',(0.858880386585508,221.922994852854,9.7877410098233));
#89503=CARTESIAN_POINT('Ctrl Pts',(-2.11919793224307,222.609469448427,9.62898314459151));
#89504=CARTESIAN_POINT('Ctrl Pts',(-3.15778638681823,225.483757510795,9.47022527935972));
#89505=CARTESIAN_POINT('Ctrl Pts',(-1.3063688643543,227.915310718306,9.31146741412792));
#89506=CARTESIAN_POINT('Ctrl Pts',(1.74063739139499,227.678771671066,9.15270954889614));
#89507=CARTESIAN_POINT('Ctrl Pts',(3.19461237498849,224.990620895806,8.99395168366434));
#89508=CARTESIAN_POINT('Ctrl Pts',(1.72487823861759,222.311053876336,8.83519381843255));
#89509=CARTESIAN_POINT('Ctrl Pts',(-1.32346439390693,222.092410243503,8.67643595320076));
#89510=CARTESIAN_POINT('Ctrl Pts',(-3.1605724651718,224.534792641478,8.51767808796896));
#89511=CARTESIAN_POINT('Ctrl Pts',(-2.10512474059796,227.402932795679,8.35892022273718));
#89512=CARTESIAN_POINT('Ctrl Pts',(0.876933063789126,228.071908949767,8.20016235750537));
#89513=CARTESIAN_POINT('Ctrl Pts',(3.05642176268095,225.929474153829,8.04140449227359));
#89514=CARTESIAN_POINT('Ctrl Pts',(2.43867338455803,222.936384648857,7.88264662704178));
#89515=CARTESIAN_POINT('Ctrl Pts',(-0.410948779213894,221.831915832102,
7.72388876181));
#89516=CARTESIAN_POINT('Ctrl Pts',(-2.88447063640942,223.626877521225,7.56513089657821));
#89517=CARTESIAN_POINT('Ctrl Pts',(-2.71812508059212,226.678520848926,7.40637303134642));
#89518=CARTESIAN_POINT('Ctrl Pts',(-0.064151557904577,228.193981961697,
7.24761516611462));
#89519=CARTESIAN_POINT('Ctrl Pts',(2.64853346805454,226.786310908722,7.08885730088283));
#89520=CARTESIAN_POINT('Ctrl Pts',(2.93728076820118,223.74380818233,6.93009943565104));
#89521=CARTESIAN_POINT('Ctrl Pts',(0.537828824795869,221.850972158071,6.77134157041925));
#89522=CARTESIAN_POINT('Ctrl Pts',(-2.35384403791301,222.840126290913,6.61258370518745));
#89523=CARTESIAN_POINT('Ctrl Pts',(-3.09127892968659,225.805996757376,6.45382583995566));
#89524=CARTESIAN_POINT('Ctrl Pts',(-0.999575466572595,228.034219023184,
6.29506797472387));
#89525=CARTESIAN_POINT('Ctrl Pts',(2.0069394242413,227.485524158292,6.13631010949207));
#89526=CARTESIAN_POINT('Ctrl Pts',(3.17670343291052,224.662077681472,5.97755224426029));
#89527=CARTESIAN_POINT('Ctrl Pts',(1.43914858470087,222.14789769728,5.81879437902849));
#89528=CARTESIAN_POINT('Ctrl Pts',(-1.61551499163388,222.243961628382,5.6600365137967));
#89529=CARTESIAN_POINT('Ctrl Pts',(-3.19165931115384,224.86235176881,5.50127864856491));
#89530=CARTESIAN_POINT('Ctrl Pts',(-1.84679715461491,227.60671756501,5.34252078333311));
#89531=CARTESIAN_POINT('Ctrl Pts',(1.18825368520437,227.96541554822,5.18376291810132));
#89532=CARTESIAN_POINT('Ctrl Pts',(3.13581479905091,225.610165338311,5.02500505286953));
#89533=CARTESIAN_POINT('Ctrl Pts',(2.21347833212026,222.696491834775,4.86624718763774));
#89534=CARTESIAN_POINT('Ctrl Pts',(-0.734633417326518,221.890988913467,
4.70748932240595));
#89535=CARTESIAN_POINT('Ctrl Pts',(-3.01040869211954,223.930852816301,4.54873145717415));
#89536=CARTESIAN_POINT('Ctrl Pts',(-2.53105805027697,226.949200179601,4.38997359194236));
#89537=CARTESIAN_POINT('Ctrl Pts',(0.264716819669501,228.183639615205,4.23121572671057));
#89538=CARTESIAN_POINT('Ctrl Pts',(2.81822286661979,226.504412200118,4.07245786147877));
#89539=CARTESIAN_POINT('Ctrl Pts',(2.79249145695371,223.448346798741,3.91369999624699));
#89540=CARTESIAN_POINT('Ctrl Pts',(0.211071975512616,221.812354345939,3.75494213101519));
#89541=CARTESIAN_POINT('Ctrl Pts',(-2.56352056924564,223.09369507079,3.5961842657834));
#89542=CARTESIAN_POINT('Ctrl Pts',(-2.99197919059342,226.119685991062,3.43742640055161));
#89543=CARTESIAN_POINT('Ctrl Pts',(-0.682178572833074,228.120940338027,
3.27866853531981));
#89544=CARTESIAN_POINT('Ctrl Pts',(2.25195184484294,227.26591020694,3.11991067008802));
#89545=CARTESIAN_POINT('Ctrl Pts',(3.12509602900158,224.337119150509,2.96115280485623));
#89546=CARTESIAN_POINT('Ctrl Pts',(1.13815243745883,222.014996607363,2.80239493962443));
#89547=CARTESIAN_POINT('Ctrl Pts',(-1.89042819398914,222.424749080416,2.64363707439265));
#89548=CARTESIAN_POINT('Ctrl Pts',(-3.18888906964905,225.191371035635,2.48487920916085));
#89549=CARTESIAN_POINT('Ctrl Pts',(-1.5688786864963,227.782850344709,2.32612134392906));
#89550=CARTESIAN_POINT('Ctrl Pts',(1.48696919015871,227.827464887782,2.16736347869726));
#89551=CARTESIAN_POINT('Ctrl Pts',(3.18194336661653,225.284384164112,2.00860561346548));
#89552=CARTESIAN_POINT('Ctrl Pts',(1.96480219695107,222.481034074754,1.84984774823368));
#89553=CARTESIAN_POINT('Ctrl Pts',(-1.05052403383013,221.983043511628,1.69108988300189));
#89554=CARTESIAN_POINT('Ctrl Pts',(-3.10441443162012,224.246167324559,1.53233201777009));
#89555=CARTESIAN_POINT('Ctrl Pts',(-2.31713730514386,227.199207066186,1.37357415253831));
#89556=CARTESIAN_POINT('Ctrl Pts',(0.59076844002395,228.139515742124,1.21481628730651));
#89557=CARTESIAN_POINT('Ctrl Pts',(2.95803411273257,226.206573948019,1.05605842207472));
#89558=CARTESIAN_POINT('Ctrl Pts',(2.6180437519229,223.169306233895,0.897300556842932));
#89559=CARTESIAN_POINT('Ctrl Pts',(-0.117851520574949,221.807630521893,
0.738542691611135));
#89560=CARTESIAN_POINT('Ctrl Pts',(-2.74615033681632,223.367324564969,0.579784826379343));
#89561=CARTESIAN_POINT('Ctrl Pts',(-2.86064184590518,226.421825383467,0.421026961147552));
#89562=CARTESIAN_POINT('Ctrl Pts',(-0.3581519623068,228.173888489799,0.262269095915755));
#89563=CARTESIAN_POINT('Ctrl Pts',(2.47430989289899,227.023624158005,0.103511230683968));
#89564=CARTESIAN_POINT('Ctrl Pts',(3.03778511801357,224.016350458554,-0.0552466345478283));
#89565=CARTESIAN_POINT('Ctrl Pts',(1.56627230491969,222.620976084267,-0.161085211369022));
#89566=CARTESIAN_POINT('Ctrl Pts',(0.698066426161045,222.388867814061,-0.21400449977962));
#89567=CARTESIAN_POINT('Ctrl Pts',(2.19519710401913,226.876863439079,20.2140044997796));
#89568=CARTESIAN_POINT('Ctrl Pts',(2.81925737956185,226.146956680238,20.161085211369));
#89569=CARTESIAN_POINT('Ctrl Pts',(3.27049164420653,224.027494344291,20.0552466345478));
#89570=CARTESIAN_POINT('Ctrl Pts',(0.954039492451579,221.720318789244,19.896488769316));
#89571=CARTESIAN_POINT('Ctrl Pts',(-2.23649130527235,222.421823129205,19.7377309040842));
#89572=CARTESIAN_POINT('Ctrl Pts',(-3.3797175254044,225.479421642892,19.5789730388525));
#89573=CARTESIAN_POINT('Ctrl Pts',(-1.43005946382394,228.09994784751,19.4202151736207));
#89574=CARTESIAN_POINT('Ctrl Pts',(1.82850379375034,227.882567961598,19.2614573083888));
#89575=CARTESIAN_POINT('Ctrl Pts',(3.41356390474589,225.027472561972,19.1026994431571));
#89576=CARTESIAN_POINT('Ctrl Pts',(1.87455830558183,222.147032130142,18.9439415779253));
#89577=CARTESIAN_POINT('Ctrl Pts',(-1.38005668887008,221.877727306915,18.7851837126935));
#89578=CARTESIAN_POINT('Ctrl Pts',(-3.37163710689758,224.465877327599,18.6264258474617));
#89579=CARTESIAN_POINT('Ctrl Pts',(-2.27749870018589,227.542880523328,18.4676679822299));
#89580=CARTESIAN_POINT('Ctrl Pts',(0.90100806341719,228.292627685475,18.3089101169981));
#89581=CARTESIAN_POINT('Ctrl Pts',(3.25491147730285,226.028967967827,18.1501522517663));
#89582=CARTESIAN_POINT('Ctrl Pts',(2.62992043175177,222.823593926977,17.9913943865345));
#89583=CARTESIAN_POINT('Ctrl Pts',(-0.401973884783737,221.610068056307,
17.8326365213027));
#89584=CARTESIAN_POINT('Ctrl Pts',(-3.06598162163353,223.499007069173,17.6738786560709));
#89585=CARTESIAN_POINT('Ctrl Pts',(-2.92400314626534,226.761655096983,17.5151207908392));
#89586=CARTESIAN_POINT('Ctrl Pts',(-0.105977083113621,228.412036280099,
17.3563629256073));
#89587=CARTESIAN_POINT('Ctrl Pts',(2.8090391908619,226.939722077155,17.1976050603756));
#89588=CARTESIAN_POINT('Ctrl Pts',(3.15322291347281,223.692174264458,17.0388471951438));
#89589=CARTESIAN_POINT('Ctrl Pts',(0.611577146889394,221.641548533695,16.880089329912));
#89590=CARTESIAN_POINT('Ctrl Pts',(-2.48978399910804,222.664577442884,16.7213314646802));
#89591=CARTESIAN_POINT('Ctrl Pts',(-3.31249492770443,225.824984989402,16.5625735994484));
#89592=CARTESIAN_POINT('Ctrl Pts',(-1.10361062839445,228.230366303651,16.4038157342166));
#89593=CARTESIAN_POINT('Ctrl Pts',(2.11529807446024,227.679316505017,16.2450578689848));
#89594=CARTESIAN_POINT('Ctrl Pts',(3.39828606283148,224.676156345768,16.086300003753));
#89595=CARTESIAN_POINT('Ctrl Pts',(1.5711627800941,221.969377886425,15.9275421385212));
#89596=CARTESIAN_POINT('Ctrl Pts',(-1.69388861718143,222.036224666109,15.7687842732894));
#89597=CARTESIAN_POINT('Ctrl Pts',(-3.40869321863266,224.815518514891,15.6100264080576));
#89598=CARTESIAN_POINT('Ctrl Pts',(-2.00386192043016,227.763649811556,15.4512685428258));
#89599=CARTESIAN_POINT('Ctrl Pts',(1.23490372854773,228.18248890938,15.2925106775941));
#89600=CARTESIAN_POINT('Ctrl Pts',(3.3434855337213,225.688714282479,15.1337528123623));
#89601=CARTESIAN_POINT('Ctrl Pts',(2.39210950991196,222.56462837134,14.9749949471305));
#89602=CARTESIAN_POINT('Ctrl Pts',(-0.748525043301124,221.66939447898,14.8162370818987));
#89603=CARTESIAN_POINT('Ctrl Pts',(-3.20410950632018,223.822330628485,14.6574792166669));
#89604=CARTESIAN_POINT('Ctrl Pts',(-2.72729307515348,227.05306974049,14.4987213514351));
#89605=CARTESIAN_POINT('Ctrl Pts',(0.245541871145432,228.404839506733,14.3399634862033));
#89606=CARTESIAN_POINT('Ctrl Pts',(2.99365690662777,226.640500290306,14.1812056209715));
#89607=CARTESIAN_POINT('Ctrl Pts',(3.00197725888707,223.374775272702,14.0224477557397));
#89608=CARTESIAN_POINT('Ctrl Pts',(0.262888141862807,221.596455861611,13.8636898905079));
#89609=CARTESIAN_POINT('Ctrl Pts',(-2.71679619225647,222.933059912132,13.7049320252761));
#89610=CARTESIAN_POINT('Ctrl Pts',(-3.21006875805803,226.161327449789,13.5461741600443));
#89611=CARTESIAN_POINT('Ctrl Pts',(-0.765486522717795,228.326748151068,
13.3874162948126));
#89612=CARTESIAN_POINT('Ctrl Pts',(2.37966894811175,227.44752907531,13.2286584295807));
#89613=CARTESIAN_POINT('Ctrl Pts',(3.34695149120764,224.328331486075,13.069900564349));
#89614=CARTESIAN_POINT('Ctrl Pts',(1.25110416116596,221.823844894372,12.9111426991172));
#89615=CARTESIAN_POINT('Ctrl Pts',(-1.98975364797633,222.22617533044,12.7523848338854));
#89616=CARTESIAN_POINT('Ctrl Pts',(-3.40958899673583,225.167109995012,12.5936269686536));
#89617=CARTESIAN_POINT('Ctrl Pts',(-1.70896862976155,227.95510559872,12.4348691034218));
#89618=CARTESIAN_POINT('Ctrl Pts',(1.55569975996694,228.038588674687,12.27611123819));
#89619=CARTESIAN_POINT('Ctrl Pts',(3.39659179055011,225.34115551507,12.1173533729582));
#89620=CARTESIAN_POINT('Ctrl Pts',(2.12892314798953,222.331496841476,11.9585955077264));
#89621=CARTESIAN_POINT('Ctrl Pts',(-1.08713587589318,221.764052153628,11.7998376424946));
#89622=CARTESIAN_POINT('Ctrl Pts',(-3.30824818890903,224.158146807528,11.6410797772628));
#89623=CARTESIAN_POINT('Ctrl Pts',(-2.50165188952906,227.322705470074,11.482321912031));
#89624=CARTESIAN_POINT('Ctrl Pts',(0.594456120772842,228.361524177746,11.3235640467992));
#89625=CARTESIAN_POINT('Ctrl Pts',(3.14651791271986,226.323876090134,11.1648061815675));
#89626=CARTESIAN_POINT('Ctrl Pts',(2.81888663467947,223.074616656891,11.0060483163356));
#89627=CARTESIAN_POINT('Ctrl Pts',(-0.0885895805695465,221.587467983548,
10.8472904511039));
#89628=CARTESIAN_POINT('Ctrl Pts',(-2.914988615165,223.223468477467,10.6885325858721));
#89629=CARTESIAN_POINT('Ctrl Pts',(-3.07359018379062,226.485350550948,10.5297747206403));
#89630=CARTESIAN_POINT('Ctrl Pts',(-0.419242137077048,228.387839858611,
10.3710168554085));
#89631=CARTESIAN_POINT('Ctrl Pts',(2.61879629700314,227.189778260897,10.2122589901767));
#89632=CARTESIAN_POINT('Ctrl Pts',(3.26011246304771,223.987631684921,10.0535011249449));
#89633=CARTESIAN_POINT('Ctrl Pts',(0.917773831111815,221.712004551095,9.89474325971311));
#89634=CARTESIAN_POINT('Ctrl Pts',(-2.26451137496702,222.445550722809,9.73598539448132));
#89635=CARTESIAN_POINT('Ctrl Pts',(-3.37431585972579,225.516928772558,9.57722752924953));
#89636=CARTESIAN_POINT('Ctrl Pts',(-1.39594660235529,228.115213629989,9.41846966401773));
#89637=CARTESIAN_POINT('Ctrl Pts',(1.85999293059652,227.862455095757,9.25971179878594));
#89638=CARTESIAN_POINT('Ctrl Pts',(3.41366700660884,224.989977770452,9.10095393355415));
#89639=CARTESIAN_POINT('Ctrl Pts',(1.84315317241193,222.126672789235,8.94219606832236));
#89640=CARTESIAN_POINT('Ctrl Pts',(-1.41421437269613,221.893036758319,8.78343820309056));
#89641=CARTESIAN_POINT('Ctrl Pts',(-3.37729297952532,224.502893364011,8.62468033785877));
#89642=CARTESIAN_POINT('Ctrl Pts',(-2.24947318430178,227.567701943412,8.46592247262699));
#89643=CARTESIAN_POINT('Ctrl Pts',(0.937064380736367,228.282549805174,8.30716460739518));
#89644=CARTESIAN_POINT('Ctrl Pts',(3.26600066137376,225.993208214324,8.14840674216341));
#89645=CARTESIAN_POINT('Ctrl Pts',(2.60589326515423,222.794882504782,7.98964887693159));
#89646=CARTESIAN_POINT('Ctrl Pts',(-0.439127544860177,221.614680240149,
7.83089101169981));
#89647=CARTESIAN_POINT('Ctrl Pts',(-3.08225884308682,223.532722486607,7.67213314646803));
#89648=CARTESIAN_POINT('Ctrl Pts',(-2.90450696932731,226.793617055623,7.51337528123622));
#89649=CARTESIAN_POINT('Ctrl Pts',(-0.0685504314564027,228.412993365865,
7.35461741600444));
#89650=CARTESIAN_POINT('Ctrl Pts',(2.83014345858772,226.90879828188,7.19585955077264));
#89651=CARTESIAN_POINT('Ctrl Pts',(3.13869016662505,223.65767108538,7.03710168554085));
#89652=CARTESIAN_POINT('Ctrl Pts',(0.574707757593123,221.635043258754,6.87834382030906));
#89653=CARTESIAN_POINT('Ctrl Pts',(-2.51524716858818,222.692023709393,6.71958595507726));
#89654=CARTESIAN_POINT('Ctrl Pts',(-3.30324798498729,225.861263970437,6.56082808984547));
#89655=CARTESIAN_POINT('Ctrl Pts',(-1.06811637542311,228.242275479605,6.40207022461368));
#89656=CARTESIAN_POINT('Ctrl Pts',(2.14455529892566,227.655956597338,6.24331235938189));
#89657=CARTESIAN_POINT('Ctrl Pts',(3.39453004803023,224.63890634163,6.08455449415009));
#89658=CARTESIAN_POINT('Ctrl Pts',(1.53783103066421,221.952328987863,5.9257966289183));
#89659=CARTESIAN_POINT('Ctrl Pts',(-1.72629088549199,222.054980024556,5.76703876368652));
#89660=CARTESIAN_POINT('Ctrl Pts',(-3.41051145113059,224.852913226966,5.60828089845471));
#89661=CARTESIAN_POINT('Ctrl Pts',(-1.97343207080975,227.785460238272,5.44952303322293));
#89662=CARTESIAN_POINT('Ctrl Pts',(1.26973226311318,228.168754149048,5.29076516799113));
#89663=CARTESIAN_POINT('Ctrl Pts',(3.35083767976526,225.652004387222,5.13200730275934));
#89664=CARTESIAN_POINT('Ctrl Pts',(2.36525658366603,222.538540235852,4.97324943752754));
#89665=CARTESIAN_POINT('Ctrl Pts',(-0.785007244795656,221.677803963833,
4.81449157229576));
#89666=CARTESIAN_POINT('Ctrl Pts',(-3.21683247368438,223.857541373477,4.65573370706396));
#89667=CARTESIAN_POINT('Ctrl Pts',(-2.70461274916752,227.082856873177,4.49697584183217));
#89668=CARTESIAN_POINT('Ctrl Pts',(0.282868457054493,228.401941844477,4.33821797660038));
#89669=CARTESIAN_POINT('Ctrl Pts',(3.01146846245633,226.607569773438,4.17946011136859));
#89670=CARTESIAN_POINT('Ctrl Pts',(2.98397264953758,223.34194990907,4.02070224613679));
#89671=CARTESIAN_POINT('Ctrl Pts',(0.225545184908317,221.593777422506,3.861944380905));
#89672=CARTESIAN_POINT('Ctrl Pts',(-2.73930122368241,222.962979705353,3.70318651567321));
#89673=CARTESIAN_POINT('Ctrl Pts',(-3.19713926088632,226.196462880873,3.54442865044142));
#89674=CARTESIAN_POINT('Ctrl Pts',(-0.728955570612594,228.334943276665,
3.38567078520962));
#89675=CARTESIAN_POINT('Ctrl Pts',(2.40636822589155,227.421283713145,3.22691291997783));
#89676=CARTESIAN_POINT('Ctrl Pts',(3.33938392344875,224.291665397987,3.06815505474604));
#89677=CARTESIAN_POINT('Ctrl Pts',(1.21619557185201,221.81031486767,2.90939718951424));
#89678=CARTESIAN_POINT('Ctrl Pts',(-2.02005489138791,222.248164075633,2.75063932428246));
#89679=CARTESIAN_POINT('Ctrl Pts',(-3.40755125411287,225.204493351206,2.59188145905066));
#89680=CARTESIAN_POINT('Ctrl Pts',(-1.67645672801963,227.973670446042,2.43312359381887));
#89681=CARTESIAN_POINT('Ctrl Pts',(1.58893069595241,228.021344209186,2.27436572858707));
#89682=CARTESIAN_POINT('Ctrl Pts',(3.40012928409063,225.303884391681,2.11560786335529));
#89683=CARTESIAN_POINT('Ctrl Pts',(2.09952872115466,222.308308533108,1.95684999812349));
#89684=CARTESIAN_POINT('Ctrl Pts',(-1.1225584869114,221.776170747549,1.7980921328917));
#89685=CARTESIAN_POINT('Ctrl Pts',(-3.3172841885395,224.194477003594,1.6393342676599));
#89686=CARTESIAN_POINT('Ctrl Pts',(-2.47602345445138,227.350006736754,1.48057640242812));
#89687=CARTESIAN_POINT('Ctrl Pts',(0.631277443249367,228.354792396575,1.32181853719632));
#89688=CARTESIAN_POINT('Ctrl Pts',(3.16086656838766,226.289308746699,1.16306067196453));
#89689=CARTESIAN_POINT('Ctrl Pts',(2.7975630620381,223.043775527358,1.00430280673274));
#89690=CARTESIAN_POINT('Ctrl Pts',(-0.125932601593587,221.588729685755,
0.845544941500944));
#89691=CARTESIAN_POINT('Ctrl Pts',(-2.93445391790652,223.255371979179,0.686787076269154));
#89692=CARTESIAN_POINT('Ctrl Pts',(-3.05679611196219,226.519319977191,0.528029211037361));
#89693=CARTESIAN_POINT('Ctrl Pts',(-0.382710449208524,228.391522084216,
0.369271345805566));
#89694=CARTESIAN_POINT('Ctrl Pts',(2.64397336955335,227.162384105202,0.210513480573778));
#89695=CARTESIAN_POINT('Ctrl Pts',(3.24608610162528,223.948901590694,0.0517556153419817));
#89696=CARTESIAN_POINT('Ctrl Pts',(1.6736716268085,222.457846368889,-0.0540829614792118));
#89697=CARTESIAN_POINT('Ctrl Pts',(0.745932854346969,222.209822430158,-0.10700224988981));
#89698=CARTESIAN_POINT('Ctrl Pts',(2.33606265769616,226.997301556931,20.3210067496694));
#89699=CARTESIAN_POINT('Ctrl Pts',(3.00016881161637,226.220556762668,20.2680874612588));
#89700=CARTESIAN_POINT('Ctrl Pts',(3.48035872876753,223.965088764676,20.1622488844376));
#89701=CARTESIAN_POINT('Ctrl Pts',(1.01526010042701,221.509862011222,20.0034910192058));
#89702=CARTESIAN_POINT('Ctrl Pts',(-2.3800067032447,222.256381806548,19.844733153974));
#89703=CARTESIAN_POINT('Ctrl Pts',(-3.59659362259695,225.510186076321,19.6859752887423));
#89704=CARTESIAN_POINT('Ctrl Pts',(-1.52182622034608,228.298871155631,19.5272174235105));
#89705=CARTESIAN_POINT('Ctrl Pts',(1.94583867854751,228.067542026651,19.3684595582787));
#89706=CARTESIAN_POINT('Ctrl Pts',(3.63261192033118,225.029235473214,19.2097016930469));
#89707=CARTESIAN_POINT('Ctrl Pts',(1.99484850327397,221.96395749968,19.0509438278151));
#89708=CARTESIAN_POINT('Ctrl Pts',(-1.46861477289244,221.67737141594,18.8921859625833));
#89709=CARTESIAN_POINT('Ctrl Pts',(-3.5879946845345,224.431602735199,18.7334280973515));
#89710=CARTESIAN_POINT('Ctrl Pts',(-2.42364553812269,227.7060568833,18.5746702321197));
#89711=CARTESIAN_POINT('Ctrl Pts',(0.958825650497796,228.503915237338,18.4159123668879));
#89712=CARTESIAN_POINT('Ctrl Pts',(3.46377878428887,226.094996727722,18.2571545016561));
#89713=CARTESIAN_POINT('Ctrl Pts',(2.79868213295254,222.683934191666,18.0983966364244));
#89714=CARTESIAN_POINT('Ctrl Pts',(-0.427768504200867,221.39253650103,17.9396387711925));
#89715=CARTESIAN_POINT('Ctrl Pts',(-3.26272532082312,223.402688519974,17.7808809059608));
#89716=CARTESIAN_POINT('Ctrl Pts',(-3.11163610250327,226.874700308353,17.622123040729));
#89717=CARTESIAN_POINT('Ctrl Pts',(-0.112777620733934,228.630986268181,
17.4633651754972));
#89718=CARTESIAN_POINT('Ctrl Pts',(2.98929492288558,227.064193826811,17.3046073102654));
#89719=CARTESIAN_POINT('Ctrl Pts',(3.35556487664332,223.608251232666,17.1458494450336));
#89720=CARTESIAN_POINT('Ctrl Pts',(0.650821984291496,221.426037077147,16.9870915798018));
#89721=CARTESIAN_POINT('Ctrl Pts',(-2.6495531610336,222.514713637499,16.82833371457));
#89722=CARTESIAN_POINT('Ctrl Pts',(-3.52505735828943,225.87792418429,16.6695758493382));
#89723=CARTESIAN_POINT('Ctrl Pts',(-1.174429199505,228.437658549578,16.5108179841064));
#89724=CARTESIAN_POINT('Ctrl Pts',(2.25103651630915,227.851247946737,16.3520601188746));
#89725=CARTESIAN_POINT('Ctrl Pts',(3.61635370100267,224.655375334543,16.1933022536428));
#89726=CARTESIAN_POINT('Ctrl Pts',(1.67198412070606,221.77490320293,16.034544388411));
#89727=CARTESIAN_POINT('Ctrl Pts',(-1.80258526109082,221.84603953302,15.8757865231792));
#89728=CARTESIAN_POINT('Ctrl Pts',(-3.62742868283253,224.803680358538,15.7170286579475));
#89729=CARTESIAN_POINT('Ctrl Pts',(-2.13244951668605,227.940992912165,15.5582707927156));
#89730=CARTESIAN_POINT('Ctrl Pts',(1.31414736327247,228.386708868249,15.3995129274839));
#89731=CARTESIAN_POINT('Ctrl Pts',(3.55803662804284,225.732909001281,15.2407550622521));
#89732=CARTESIAN_POINT('Ctrl Pts',(2.54561091074421,222.408350845166,15.0819971970203));
#89733=CARTESIAN_POINT('Ctrl Pts',(-0.796557811963526,221.455669893639,
14.9232393317885));
#89734=CARTESIAN_POINT('Ctrl Pts',(-3.40971685648626,223.746759716077,14.7644814665567));
#89735=CARTESIAN_POINT('Ctrl Pts',(-2.90230316803655,227.184814997078,14.6057236013249));
#89736=CARTESIAN_POINT('Ctrl Pts',(0.261298265669851,228.62332767867,14.4469657360931));
#89737=CARTESIAN_POINT('Ctrl Pts',(3.18575953691054,226.745771011226,14.2882078708613));
#89738=CARTESIAN_POINT('Ctrl Pts',(3.19461380524764,223.270484782959,14.1294500056295));
#89739=CARTESIAN_POINT('Ctrl Pts',(0.279757644647243,221.378050813317,13.9706921403977));
#89740=CARTESIAN_POINT('Ctrl Pts',(-2.89113270133312,222.800424596897,13.8119342751659));
#89741=CARTESIAN_POINT('Ctrl Pts',(-3.41605851274443,226.235849702901,13.6531764099342));
#89742=CARTESIAN_POINT('Ctrl Pts',(-0.814607707625303,228.540225209408,
13.4944185447024));
#89743=CARTESIAN_POINT('Ctrl Pts',(2.53237203947883,227.604586743482,13.3356606794706));
#89744=CARTESIAN_POINT('Ctrl Pts',(3.56172499563507,224.285230592343,13.1769028142388));
#89745=CARTESIAN_POINT('Ctrl Pts',(1.33138737584751,221.620031374985,13.018144949007));
#89746=CARTESIAN_POINT('Ctrl Pts',(-2.11743591796015,222.048179310326,12.8593870837752));
#89747=CARTESIAN_POINT('Ctrl Pts',(-3.62838194291682,225.17783342478,12.7006292185434));
#89748=CARTESIAN_POINT('Ctrl Pts',(-1.81863295639868,228.144734395868,12.5418713533116));
#89749=CARTESIAN_POINT('Ctrl Pts',(1.65552884029951,228.233574571522,12.3831134880798));
#89750=CARTESIAN_POINT('Ctrl Pts',(3.6145507074577,225.363047426476,12.224355622848));
#89751=CARTESIAN_POINT('Ctrl Pts',(2.26553590928934,222.160259290996,12.0655977576162));
#89752=CARTESIAN_POINT('Ctrl Pts',(-1.15689726397057,221.556401740727,11.9068398923844));
#89753=CARTESIAN_POINT('Ctrl Pts',(-3.5205381067385,224.104125181928,11.7480820271526));
#89754=CARTESIAN_POINT('Ctrl Pts',(-2.66218261266118,227.471753221399,11.5893241619208));
#89755=CARTESIAN_POINT('Ctrl Pts',(0.632602303835877,228.577232809845,11.430566296689));
#89756=CARTESIAN_POINT('Ctrl Pts',(3.34842961673882,226.408829071393,11.2718084314573));
#89757=CARTESIAN_POINT('Ctrl Pts',(2.99977427607618,222.951065022201,11.1130505662255));
#89758=CARTESIAN_POINT('Ctrl Pts',(-0.0942743640881148,221.36848618412,
10.9542927009937));
#89759=CARTESIAN_POINT('Ctrl Pts',(-3.10204310994621,223.109468647525,10.7955348357619));
#89760=CARTESIAN_POINT('Ctrl Pts',(-3.27082212356644,226.580665330373,10.6367769705301));
#89761=CARTESIAN_POINT('Ctrl Pts',(-0.446144858320614,228.605237165021,
10.4780191052983));
#89762=CARTESIAN_POINT('Ctrl Pts',(2.78684416371602,227.330296088014,10.3192612400665));
#89763=CARTESIAN_POINT('Ctrl Pts',(3.46931351670972,223.922668122894,10.1605033748347));
#89764=CARTESIAN_POINT('Ctrl Pts',(0.976667275638124,221.501014249336,10.0017455096029));
#89765=CARTESIAN_POINT('Ctrl Pts',(-2.40982481769097,222.281631997191,9.84298764437114));
#89766=CARTESIAN_POINT('Ctrl Pts',(-3.59084533263335,225.55010003432,9.68422977913934));
#89767=CARTESIAN_POINT('Ctrl Pts',(-1.48552434035628,228.315116541671,9.52547191390755));
#89768=CARTESIAN_POINT('Ctrl Pts',(1.97934846979805,228.046138520449,9.36671404867575));
#89769=CARTESIAN_POINT('Ctrl Pts',(3.63272163822919,224.989334645098,9.20795618344396));
#89770=CARTESIAN_POINT('Ctrl Pts',(1.96142810620627,221.942291702134,9.04919831821217));
#89771=CARTESIAN_POINT('Ctrl Pts',(-1.50496435148532,221.693663273135,8.89044045298037));
#89772=CARTESIAN_POINT('Ctrl Pts',(-3.59401349387884,224.470994086545,8.73168258774859));
#89773=CARTESIAN_POINT('Ctrl Pts',(-2.39382162800561,227.732471091145,8.57292472251679));
#89774=CARTESIAN_POINT('Ctrl Pts',(0.997195697683612,228.493190660582,8.41416685728499));
#89775=CARTESIAN_POINT('Ctrl Pts',(3.47557956006656,226.05694227482,8.25540899205321));
#89776=CARTESIAN_POINT('Ctrl Pts',(2.77311314575043,222.653380360706,8.09665112682141));
#89777=CARTESIAN_POINT('Ctrl Pts',(-0.467306310506461,221.397444648195,
7.93789326158963));
#89778=CARTESIAN_POINT('Ctrl Pts',(-3.28004704976421,223.43856745199,7.77913539635783));
#89779=CARTESIAN_POINT('Ctrl Pts',(-3.09088885806249,226.90871326232,7.62037753112604));
#89780=CARTESIAN_POINT('Ctrl Pts',(-0.0729493050082294,228.632004770035,
7.46161966589425));
#89781=CARTESIAN_POINT('Ctrl Pts',(3.01175344912091,227.031285655038,7.30286180066245));
#89782=CARTESIAN_POINT('Ctrl Pts',(3.3400995650489,223.571533988429,7.14410393543066));
#89783=CARTESIAN_POINT('Ctrl Pts',(0.611586690390379,221.419114359437,6.98534607019887));
#89784=CARTESIAN_POINT('Ctrl Pts',(-2.67665029926335,222.543921127873,6.82658820496707));
#89785=CARTESIAN_POINT('Ctrl Pts',(-3.51521704028799,225.916531183497,6.66783033973528));
#89786=CARTESIAN_POINT('Ctrl Pts',(-1.13665728427362,228.450331936026,6.50907247450349));
#89787=CARTESIAN_POINT('Ctrl Pts',(2.28217117361002,227.826389036385,6.3503146092717));
#89788=CARTESIAN_POINT('Ctrl Pts',(3.61235666314995,224.615735001789,6.1915567440399));
#89789=CARTESIAN_POINT('Ctrl Pts',(1.63651347662755,221.756760278445,6.03279887880811));
#89790=CARTESIAN_POINT('Ctrl Pts',(-1.83706677935009,221.865998420731,5.87404101357633));
#89791=CARTESIAN_POINT('Ctrl Pts',(-3.62936359110735,224.843474685122,5.71528314834452));
#89792=CARTESIAN_POINT('Ctrl Pts',(-2.1000669870046,227.964202911534,5.55652528311274));
#89793=CARTESIAN_POINT('Ctrl Pts',(1.35121084102199,228.372092749875,5.39776741788093));
#89794=CARTESIAN_POINT('Ctrl Pts',(3.56586056047961,225.693843436134,5.23900955264916));
#89795=CARTESIAN_POINT('Ctrl Pts',(2.51703483521181,222.380588636929,5.08025168741735));
#89796=CARTESIAN_POINT('Ctrl Pts',(-0.835381072264795,221.464619014198,
4.92149382218557));
#89797=CARTESIAN_POINT('Ctrl Pts',(-3.42325625524921,223.784229930654,4.76273595695377));
#89798=CARTESIAN_POINT('Ctrl Pts',(-2.87816744805807,227.216513566753,4.60397809172198));
#89799=CARTESIAN_POINT('Ctrl Pts',(0.301020094439488,228.620244073749,4.44522022649019));
#89800=CARTESIAN_POINT('Ctrl Pts',(3.20471405829287,226.710727346758,4.28646236125839));
#89801=CARTESIAN_POINT('Ctrl Pts',(3.17545384212145,223.235553019399,4.12770449602661));
#89802=CARTESIAN_POINT('Ctrl Pts',(0.24001839430402,221.375200499072,3.96894663079481));
#89803=CARTESIAN_POINT('Ctrl Pts',(-2.91508187811918,222.832264339917,3.81018876556302));
#89804=CARTESIAN_POINT('Ctrl Pts',(-3.40229933117922,226.273239770683,3.65143090033123));
#89805=CARTESIAN_POINT('Ctrl Pts',(-0.77573256839211,228.548946215303,3.49267303509943));
#89806=CARTESIAN_POINT('Ctrl Pts',(2.56078460694016,227.576657219349,3.33391516986764));
#89807=CARTESIAN_POINT('Ctrl Pts',(3.55367181789592,224.246211645467,3.17515730463585));
#89808=CARTESIAN_POINT('Ctrl Pts',(1.2942387062452,221.605633127976,3.01639943940405));
#89809=CARTESIAN_POINT('Ctrl Pts',(-2.14968158878668,222.071579070849,2.85764157417227));
#89810=CARTESIAN_POINT('Ctrl Pts',(-3.62621343857669,225.217615666778,2.69888370894047));
#89811=CARTESIAN_POINT('Ctrl Pts',(-1.78403476954297,228.164490547375,2.54012584370868));
#89812=CARTESIAN_POINT('Ctrl Pts',(1.69089220174611,228.21522353059,2.38136797847689));
#89813=CARTESIAN_POINT('Ctrl Pts',(3.61831520156474,225.323384619251,2.22261011324509));
#89814=CARTESIAN_POINT('Ctrl Pts',(2.23425524535826,222.135582991462,2.0638522480133));
#89815=CARTESIAN_POINT('Ctrl Pts',(-1.19459293999268,221.56929798347,1.90509438278151));
#89816=CARTESIAN_POINT('Ctrl Pts',(-3.53015394545888,224.142786682629,1.74633651754971));
#89817=CARTESIAN_POINT('Ctrl Pts',(-2.6349096037589,227.500806407321,1.58757865231793));
#89818=CARTESIAN_POINT('Ctrl Pts',(0.671786446474784,228.570069051027,1.42882078708613));
#89819=CARTESIAN_POINT('Ctrl Pts',(3.36369902404275,226.372043545379,1.27006292185434));
#89820=CARTESIAN_POINT('Ctrl Pts',(2.97708237215331,222.918244820821,1.11130505662255));
#89821=CARTESIAN_POINT('Ctrl Pts',(-0.134013682612229,221.369828849617,
0.952547191390754));
#89822=CARTESIAN_POINT('Ctrl Pts',(-3.12275749899671,223.143419393389,0.793789326158964));
#89823=CARTESIAN_POINT('Ctrl Pts',(-3.25295037801921,226.616814570914,0.635031460927171));
#89824=CARTESIAN_POINT('Ctrl Pts',(-0.407268936110244,228.609155678633,
0.476273595695376));
#89825=CARTESIAN_POINT('Ctrl Pts',(2.8136368462077,227.3011440524,0.317515730463589));
#89826=CARTESIAN_POINT('Ctrl Pts',(3.45438708523699,223.881452722834,0.158757865231792));
#89827=CARTESIAN_POINT('Ctrl Pts',(1.7810709486973,222.29471665351,0.0529192884105984));
#89828=CARTESIAN_POINT('Ctrl Pts',(0.793799282532894,222.030777046254,0.));
#89829=CARTESIAN_POINT('Ctrl Pts',(0.793799282532894,222.030777046254,0.));
#89830=CARTESIAN_POINT('Ctrl Pts',(0.886846191183898,222.064814021077,-1.38596869938627E-16));
#89831=CARTESIAN_POINT('Ctrl Pts',(0.977825993756427,222.103621402683,2.39308088689558E-15));
#89832=CARTESIAN_POINT('Ctrl Pts',(1.06653099078737,222.146870208338,1.49880108324396E-15));
#89833=CARTESIAN_POINT('Ctrl Pts',(1.1572090782491,222.191081009455,5.84629560049093E-16));
#89834=CARTESIAN_POINT('Ctrl Pts',(1.24551070332407,222.239933633085,-4.06870172435856E-15));
#89835=CARTESIAN_POINT('Ctrl Pts',(1.33118506358561,222.293122211572,-4.44089209850063E-15));
#89836=CARTESIAN_POINT('Ctrl Pts',(1.41411876188254,222.344609325192,-4.80117636679151E-15));
#89837=CARTESIAN_POINT('Ctrl Pts',(1.49459091967829,222.400160285979,-9.26260121771311E-16));
#89838=CARTESIAN_POINT('Ctrl Pts',(1.57234035477895,222.459528324875,-1.77635683940025E-15));
#89839=CARTESIAN_POINT('Ctrl Pts',(1.64037111049203,222.511475358909,-2.52019146732557E-15));
#89840=CARTESIAN_POINT('Ctrl Pts',(1.70631698504278,222.566345560034,-2.4936108625525E-15));
#89841=CARTESIAN_POINT('Ctrl Pts',(1.76997776289673,222.623986577848,-4.71844785465692E-15));
#89842=CARTESIAN_POINT('Ctrl Pts',(1.78334871497265,222.63609317335,-5.18574011530746E-15));
#89843=CARTESIAN_POINT('Ctrl Pts',(1.79662066694636,222.648323938157,-1.20584228596178E-15));
#89844=CARTESIAN_POINT('Ctrl Pts',(1.80977449464236,222.660661071479,-1.22124532708767E-15));
#89845=CARTESIAN_POINT('Ctrl Pts',(1.88220120936656,222.728590958986,-1.30605650838734E-15));
#89846=CARTESIAN_POINT('Ctrl Pts',(1.95116218959374,222.799842420315,8.00223029047533E-15));
#89847=CARTESIAN_POINT('Ctrl Pts',(2.01641813121821,222.874123957972,6.85562717706034E-15));
#89848=CARTESIAN_POINT('Ctrl Pts',(2.08131424640546,222.947995901339,5.71534652414354E-15));
#89849=CARTESIAN_POINT('Ctrl Pts',(2.14254655535901,223.024865395635,-1.30534801110875E-16));
#89850=CARTESIAN_POINT('Ctrl Pts',(2.19983607468768,223.104472485275,-8.32667268468867E-16));
#89851=CARTESIAN_POINT('Ctrl Pts',(2.25566842116609,223.182054749239,-1.51694082584268E-15));
#89852=CARTESIAN_POINT('Ctrl Pts',(2.30775626506218,223.262237857311,-5.95467361534588E-15));
#89853=CARTESIAN_POINT('Ctrl Pts',(2.35579457812553,223.344795283462,-8.90953977261688E-15));
#89854=CARTESIAN_POINT('Ctrl Pts',(2.37650832906487,223.380393410341,-1.01836553220135E-14));
#89855=CARTESIAN_POINT('Ctrl Pts',(2.39646854028631,223.416433103221,2.5576910520071E-15));
#89856=CARTESIAN_POINT('Ctrl Pts',(2.41564778277341,223.452896532503,3.02535774210355E-15));
#89857=CARTESIAN_POINT('Ctrl Pts',(2.42885130513818,223.477998968344,3.34731245987215E-15));
#89858=CARTESIAN_POINT('Ctrl Pts',(2.44168466279926,223.503302229722,-4.14100659545732E-15));
#89859=CARTESIAN_POINT('Ctrl Pts',(2.45413837672965,223.528800502852,-4.32986979603811E-15));
#89860=CARTESIAN_POINT('Ctrl Pts',(2.46035286582353,223.541524316901,-4.42411383494947E-15));
#89861=CARTESIAN_POINT('Ctrl Pts',(2.46647227743221,223.554295737379,2.15191029731381E-15));
#89862=CARTESIAN_POINT('Ctrl Pts',(2.47249022824328,223.56710248546,2.3037127760972E-15));
#89863=CARTESIAN_POINT('Ctrl Pts',(2.51269154441903,223.652654552092,3.31778876930894E-15));
#89864=CARTESIAN_POINT('Ctrl Pts',(2.5484363396718,223.739918159891,6.98524591958814E-16));
#89865=CARTESIAN_POINT('Ctrl Pts',(2.57947353285492,223.82865573719,2.77555756156289E-17));
#89866=CARTESIAN_POINT('Ctrl Pts',(2.60982487234774,223.915432409246,-6.28190921098164E-16));
#89867=CARTESIAN_POINT('Ctrl Pts',(2.63567458362555,224.003619302437,5.15344782426835E-15));
#89868=CARTESIAN_POINT('Ctrl Pts',(2.65673873200962,224.093003025007,6.60582699651968E-15));
#89869=CARTESIAN_POINT('Ctrl Pts',(2.66036635111496,224.108396483778,6.85595239145078E-15));
#89870=CARTESIAN_POINT('Ctrl Pts',(2.66385191074304,224.123825446915,3.8409637378969E-15));
#89871=CARTESIAN_POINT('Ctrl Pts',(2.66719380198884,224.13928882952,3.99680288865056E-15));
#89872=CARTESIAN_POINT('Ctrl Pts',(2.6873209483154,224.232419856686,4.90868829782107E-15));
#89873=CARTESIAN_POINT('Ctrl Pts',(2.70224094539991,224.326800411483,3.07486859462122E-15));
#89874=CARTESIAN_POINT('Ctrl Pts',(2.71203217769051,224.422021924685,4.13558076672871E-15));
#89875=CARTESIAN_POINT('Ctrl Pts',(2.71529423454605,224.453746020357,4.48896870709092E-15));
#89876=CARTESIAN_POINT('Ctrl Pts',(2.71798660578109,224.485563339469,2.05641129816516E-15));
#89877=CARTESIAN_POINT('Ctrl Pts',(2.72011099118565,224.517458314697,2.05391259555654E-15));
#89878=CARTESIAN_POINT('Ctrl Pts',(2.72133532130525,224.535840091728,2.05247253818413E-15));
#89879=CARTESIAN_POINT('Ctrl Pts',(2.7223709858767,224.554247656756,7.55656642889705E-15));
#89880=CARTESIAN_POINT('Ctrl Pts',(2.72321822484737,224.572677981456,8.13238365537927E-15));
#89881=CARTESIAN_POINT('Ctrl Pts',(2.72379251502994,224.585170743124,8.52269405370954E-15));
#89882=CARTESIAN_POINT('Ctrl Pts',(2.72428011160068,224.597672344381,8.79861093759093E-15));
#89883=CARTESIAN_POINT('Ctrl Pts',(2.72468096993961,224.610172448783,8.57647286522933E-15));
#89884=CARTESIAN_POINT('Ctrl Pts',(2.72766933700557,224.703359733888,6.92045118606972E-15));
#89885=CARTESIAN_POINT('Ctrl Pts',(2.72584870249446,224.796609966936,-5.66219201085476E-16));
#89886=CARTESIAN_POINT('Ctrl Pts',(2.71935795287165,224.889548302923,8.46545056276682E-16));
#89887=CARTESIAN_POINT('Ctrl Pts',(2.71285435385017,224.982670624088,2.2621060893908E-15));
#89888=CARTESIAN_POINT('Ctrl Pts',(2.70166174783478,225.07548079302,5.9470159394075E-15));
#89889=CARTESIAN_POINT('Ctrl Pts',(2.68586881074027,225.167589714791,5.89805981832114E-15));
#89890=CARTESIAN_POINT('Ctrl Pts',(2.67029892991559,225.258397708661,5.84979514365098E-15));
#89891=CARTESIAN_POINT('Ctrl Pts',(2.65025728119255,225.348524970524,1.95015538798884E-16));
#89892=CARTESIAN_POINT('Ctrl Pts',(2.62578579099026,225.437573501206,8.88178419700125E-16));
#89893=CARTESIAN_POINT('Ctrl Pts',(2.61627026001682,225.472199265507,1.15770891450574E-15));
#89894=CARTESIAN_POINT('Ctrl Pts',(2.60608451887964,225.506661589206,3.62406394873002E-15));
#89895=CARTESIAN_POINT('Ctrl Pts',(2.59522946518981,225.540935610117,4.08006961549745E-15));
#89896=CARTESIAN_POINT('Ctrl Pts',(2.58886805642713,225.561021282946,4.34730352583022E-15));
#89897=CARTESIAN_POINT('Ctrl Pts',(2.58227676746916,225.581042269272,7.67942111821871E-15));
#89898=CARTESIAN_POINT('Ctrl Pts',(2.57545564888798,225.600993409454,8.14626144318709E-15));
#89899=CARTESIAN_POINT('Ctrl Pts',(2.57042451361342,225.615709014225,8.49059453145984E-15));
#89900=CARTESIAN_POINT('Ctrl Pts',(2.56526853205797,225.630385839234,1.02262120206335E-15));
#89901=CARTESIAN_POINT('Ctrl Pts',(2.5599923386753,225.645009655912,1.77635683940025E-15));
#89902=CARTESIAN_POINT('Ctrl Pts',(2.52758850675101,225.73482207622,6.40543715094128E-15));
#89903=CARTESIAN_POINT('Ctrl Pts',(2.4906131496606,225.822761175715,9.4868431892647E-15));
#89904=CARTESIAN_POINT('Ctrl Pts',(2.44913842341953,225.90838531885,8.70137295549966E-15));
#89905=CARTESIAN_POINT('Ctrl Pts',(2.41803237873873,225.972603426202,8.11227028017589E-15));
#89906=CARTESIAN_POINT('Ctrl Pts',(2.38439430103246,226.035518835997,2.83514090577719E-15));
#89907=CARTESIAN_POINT('Ctrl Pts',(2.34823741362777,226.09692820208,3.10862446895044E-15));
#89908=CARTESIAN_POINT('Ctrl Pts',(2.33712251184633,226.115805907587,3.19269539323893E-15));
#89909=CARTESIAN_POINT('Ctrl Pts',(2.32576948659689,226.134541170905,6.20229766951161E-15));
#89910=CARTESIAN_POINT('Ctrl Pts',(2.31417847054799,226.153127742234,6.19643225618915E-15));
#89911=CARTESIAN_POINT('Ctrl Pts',(2.30318790659673,226.17075146909,6.19087069023592E-15));
#89912=CARTESIAN_POINT('Ctrl Pts',(2.29198235378028,226.18824280901,8.27692394682741E-16));
#89913=CARTESIAN_POINT('Ctrl Pts',(2.28057388545861,226.205578703977,1.50573997714787E-15));
#89914=CARTESIAN_POINT('Ctrl Pts',(2.23335304213644,226.277333785992,4.31224982174617E-15));
#89915=CARTESIAN_POINT('Ctrl Pts',(2.18261517567617,226.346499716342,-4.49298739505873E-15));
#89916=CARTESIAN_POINT('Ctrl Pts',(2.12839610130427,226.412725093439,-3.25087179398054E-15));
#89917=CARTESIAN_POINT('Ctrl Pts',(2.0747094208182,226.478300183044,-2.02095291073937E-15));
#89918=CARTESIAN_POINT('Ctrl Pts',(2.0176092036947,226.54099277136,5.93088889512619E-15));
#89919=CARTESIAN_POINT('Ctrl Pts',(1.95710209621334,226.600419913581,4.67247768254353E-15));
#89920=CARTESIAN_POINT('Ctrl Pts',(1.9439378552628,226.613349191673,4.39195893259633E-15));
#89921=CARTESIAN_POINT('Ctrl Pts',(1.93061225296776,226.626123721938,9.20546864075757E-16));
#89922=CARTESIAN_POINT('Ctrl Pts',(1.91712867315962,226.638742108209,9.43689570931383E-16));
#89923=CARTESIAN_POINT('Ctrl Pts',(-2.51944987787367,224.998011234297,18.387416697508));
#89924=CARTESIAN_POINT('Ctrl Pts',(-2.52058777238211,224.866459872146,18.3957515808994));
#89925=CARTESIAN_POINT('Ctrl Pts',(-2.51117357035687,224.735071803788,18.4040864642907));
#89926=CARTESIAN_POINT('Ctrl Pts',(-2.49063889193878,224.605445490309,18.4124213476821));
#89927=CARTESIAN_POINT('Ctrl Pts',(-2.36026147469096,223.782430704556,18.4653406360927));
#89928=CARTESIAN_POINT('Ctrl Pts',(-1.78160099775816,223.030434896711,18.5182599245033));
#89929=CARTESIAN_POINT('Ctrl Pts',(-1.01945102078794,222.693560709822,18.5711792129139));
#89930=CARTESIAN_POINT('Ctrl Pts',(-0.257301043817723,222.356686522933,
18.6240985013245));
#89931=CARTESIAN_POINT('Ctrl Pts',(0.688338433189915,222.434933957,18.6770177897351));
#89932=CARTESIAN_POINT('Ctrl Pts',(1.3847398322567,222.892518565437,18.7299370781457));
#89933=CARTESIAN_POINT('Ctrl Pts',(2.08114123132348,223.350103173874,18.7828563665563));
#89934=CARTESIAN_POINT('Ctrl Pts',(2.5283045524494,224.187024956681,18.8357756549668));
#89935=CARTESIAN_POINT('Ctrl Pts',(2.5216139047758,225.020264696752,18.8886949433774));
#89936=CARTESIAN_POINT('Ctrl Pts',(2.51492325710221,225.853504436823,18.941614231788));
#89937=CARTESIAN_POINT('Ctrl Pts',(2.05437864062909,226.683062134158,18.9945335201987));
#89938=CARTESIAN_POINT('Ctrl Pts',(1.3507130032366,227.129421216121,19.0474528086093));
#89939=CARTESIAN_POINT('Ctrl Pts',(0.647047365844105,227.575780298084,19.1003720970199));
#89940=CARTESIAN_POINT('Ctrl Pts',(-0.299739292467768,227.638940764676,
19.1532913854304));
#89941=CARTESIAN_POINT('Ctrl Pts',(-1.05637251833031,227.289819588766,19.206210673841));
#89942=CARTESIAN_POINT('Ctrl Pts',(-1.81300574419286,226.940698412856,19.2591299622516));
#89943=CARTESIAN_POINT('Ctrl Pts',(-2.37948553760609,226.179295594445,19.3120492506622));
#89944=CARTESIAN_POINT('Ctrl Pts',(-2.49664129736409,225.354396351653,19.3649685390728));
#89945=CARTESIAN_POINT('Ctrl Pts',(-2.51320697146662,225.237756657184,19.3724512585512));
#89946=CARTESIAN_POINT('Ctrl Pts',(-2.52078904185958,225.119847440786,19.3799339780296));
#89947=CARTESIAN_POINT('Ctrl Pts',(-2.51981693572124,225.001815876221,19.387416697508));
#89948=CARTESIAN_POINT('Ctrl Pts',(-0.793799282532863,222.030777046254,
20.));
#89949=CARTESIAN_POINT('Ctrl Pts',(-1.78107094869726,222.29471665351,19.9470807115894));
#89950=CARTESIAN_POINT('Ctrl Pts',(-3.45438749280176,223.881450010451,19.8412421347682));
#89951=CARTESIAN_POINT('Ctrl Pts',(-2.81363649299402,227.301144948027,19.6824842695364));
#89952=CARTESIAN_POINT('Ctrl Pts',(0.407268901123991,228.609154817042,19.5237264043046));
#89953=CARTESIAN_POINT('Ctrl Pts',(3.25295011294267,226.616814793291,19.3649685390728));
#89954=CARTESIAN_POINT('Ctrl Pts',(3.12275731293263,223.14341933887,19.206210673841));
#89955=CARTESIAN_POINT('Ctrl Pts',(0.134013646578404,221.369829208712,19.0474528086092));
#89956=CARTESIAN_POINT('Ctrl Pts',(-2.97708214348246,222.918244913477,18.8886949433774));
#89957=CARTESIAN_POINT('Ctrl Pts',(-3.36369879634767,226.37204347757,18.7299370781457));
#89958=CARTESIAN_POINT('Ctrl Pts',(-0.671786392406203,228.570068782136,
18.5711792129139));
#89959=CARTESIAN_POINT('Ctrl Pts',(2.6349094131999,227.500806238298,18.4124213476821));
#89960=CARTESIAN_POINT('Ctrl Pts',(3.53015369719777,224.142786739032,18.2536634824503));
#89961=CARTESIAN_POINT('Ctrl Pts',(1.19459285411968,221.569298229067,18.0949056172185));
#89962=CARTESIAN_POINT('Ctrl Pts',(-2.23425508627908,222.135583193393,17.9361477519867));
#89963=CARTESIAN_POINT('Ctrl Pts',(-3.61831494530944,225.323384596945,17.7773898867549));
#89964=CARTESIAN_POINT('Ctrl Pts',(-1.69089208164927,228.215223302252,17.6186320215231));
#89965=CARTESIAN_POINT('Ctrl Pts',(1.7840346429268,228.164490323129,17.4598741562913));
#89966=CARTESIAN_POINT('Ctrl Pts',(3.6262131814702,225.217615651258,17.3011162910595));
#89967=CARTESIAN_POINT('Ctrl Pts',(2.14968143631101,222.071579278568,17.1423584258277));
#89968=CARTESIAN_POINT('Ctrl Pts',(-1.29423861444767,221.60563336867,16.9836005605959));
#89969=CARTESIAN_POINT('Ctrl Pts',(-3.55367156588917,224.246211698934,16.8248426953642));
#89970=CARTESIAN_POINT('Ctrl Pts',(-2.56078442533408,227.576657036616,16.6660848301324));
#89971=CARTESIAN_POINT('Ctrl Pts',(0.77573251337774,228.548945963627,16.5073269649006));
#89972=CARTESIAN_POINT('Ctrl Pts',(3.40229908990077,226.273239680388,16.3485690996688));
#89973=CARTESIAN_POINT('Ctrl Pts',(2.91508167139093,222.832264493646,16.189811234437));
#89974=CARTESIAN_POINT('Ctrl Pts',(-0.24001837728243,221.37520075613,16.0310533692052));
#89975=CARTESIAN_POINT('Ctrl Pts',(-3.17545361692919,223.235553144528,15.8722955039734));
#89976=CARTESIAN_POINT('Ctrl Pts',(-3.20471383102538,226.710727225439,15.7135376387416));
#89977=CARTESIAN_POINT('Ctrl Pts',(-0.301020073092202,228.620243817014,
15.5547797735098));
#89978=CARTESIAN_POINT('Ctrl Pts',(2.87816724394823,227.216513409565,15.396021908278));
#89979=CARTESIAN_POINT('Ctrl Pts',(3.4232560124835,223.784230016872,15.2372640430462));
#89980=CARTESIAN_POINT('Ctrl Pts',(0.835381013022407,221.464619264915,15.0785061778144));
#89981=CARTESIAN_POINT('Ctrl Pts',(-2.51703465671226,222.380588822689,14.9197483125826));
#89982=CARTESIAN_POINT('Ctrl Pts',(-3.56586030760089,225.693843386929,14.7609904473508));
#89983=CARTESIAN_POINT('Ctrl Pts',(-1.35121074519871,228.372092510738,14.6022325821191));
#89984=CARTESIAN_POINT('Ctrl Pts',(2.10006683807499,227.964202701323,14.4434747168873));
#89985=CARTESIAN_POINT('Ctrl Pts',(3.62936333372522,224.843474696222,14.2847168516555));
#89986=CARTESIAN_POINT('Ctrl Pts',(1.83706664907154,221.865998642983,14.1259589864237));
#89987=CARTESIAN_POINT('Ctrl Pts',(-1.6365133605716,221.756760508445,13.9672011211919));
#89988=CARTESIAN_POINT('Ctrl Pts',(-3.61235640697389,224.61573502904,13.8084432559601));
#89989=CARTESIAN_POINT('Ctrl Pts',(-2.2821710117662,227.826388835947,13.6496853907283));
#89990=CARTESIAN_POINT('Ctrl Pts',(1.13665720366575,228.45033169134,13.4909275254965));
#89991=CARTESIAN_POINT('Ctrl Pts',(3.51521679100075,225.9165311185,13.3321696602647));
#89992=CARTESIAN_POINT('Ctrl Pts',(2.6766501094444,222.54392130205,13.1734117950329));
#89993=CARTESIAN_POINT('Ctrl Pts',(-0.611586647018769,221.419114613381,
13.0146539298011));
#89994=CARTESIAN_POINT('Ctrl Pts',(-3.3400993281804,223.571534089731,12.8558960645693));
#89995=CARTESIAN_POINT('Ctrl Pts',(-3.01175323553757,227.031285510986,12.6971381993375));
#89996=CARTESIAN_POINT('Ctrl Pts',(0.0729492998349137,228.632004512465,
12.5383803341058));
#89997=CARTESIAN_POINT('Ctrl Pts',(3.09088863886716,226.908713126961,12.3796224688739));
#89998=CARTESIAN_POINT('Ctrl Pts',(3.28004681715442,223.438567562721,12.2208646036422));
#89999=CARTESIAN_POINT('Ctrl Pts',(0.46730627736665,221.397444903677,12.0621067384104));
#90000=CARTESIAN_POINT('Ctrl Pts',(-2.7731129490907,222.65338052712,11.9033488731786));
#90001=CARTESIAN_POINT('Ctrl Pts',(-3.47557931359025,226.056942199865,11.7445910079468));
#90002=CARTESIAN_POINT('Ctrl Pts',(-0.997195626965866,228.493190412856,
11.585833142715));
#90003=CARTESIAN_POINT('Ctrl Pts',(2.39382145824392,227.732470897368,11.4270752774832));
#90004=CARTESIAN_POINT('Ctrl Pts',(3.59401323900362,224.47099412406,11.2683174122514));
#90005=CARTESIAN_POINT('Ctrl Pts',(1.50496424475834,221.69366350761,11.1095595470196));
#90006=CARTESIAN_POINT('Ctrl Pts',(-1.9614279671085,221.942291918976,10.9508016817878));
#90007=CARTESIAN_POINT('Ctrl Pts',(-3.6327213806089,224.989334645854,10.792043816556));
#90008=CARTESIAN_POINT('Ctrl Pts',(-1.97934832942936,228.046138304427,10.6332859513243));
#90009=CARTESIAN_POINT('Ctrl Pts',(1.48552423500794,228.315116306574,10.4745280860925));
#90010=CARTESIAN_POINT('Ctrl Pts',(3.59084507798282,225.550099995309,10.3157702208607));
#90011=CARTESIAN_POINT('Ctrl Pts',(2.40982464679436,222.281632189969,10.1570123556289));
#90012=CARTESIAN_POINT('Ctrl Pts',(-0.976667206376252,221.501014497472,
9.99825449039707));
#90013=CARTESIAN_POINT('Ctrl Pts',(-3.4693132706778,223.922668199295,9.83949662516529));
#90014=CARTESIAN_POINT('Ctrl Pts',(-2.78684396608248,227.330295922758,9.68073875993348));
#90015=CARTESIAN_POINT('Ctrl Pts',(0.446144826681538,228.60523690935,9.5219808947017));
#90016=CARTESIAN_POINT('Ctrl Pts',(3.27082189161085,226.580665218277,9.36322302946991));
#90017=CARTESIAN_POINT('Ctrl Pts',(3.10204288995985,223.109468781596,9.20446516423812));
#90018=CARTESIAN_POINT('Ctrl Pts',(0.094274357402458,221.368486441654,9.04570729900631));
#90019=CARTESIAN_POINT('Ctrl Pts',(-2.9997740633424,222.951065167505,8.88694943377453));
#90020=CARTESIAN_POINT('Ctrl Pts',(-3.34842937927955,226.408828971483,8.72819156854274));
#90021=CARTESIAN_POINT('Ctrl Pts',(-0.632602258973873,228.57723255616,8.56943370331094));
#90022=CARTESIAN_POINT('Ctrl Pts',(2.66218242386824,227.471753046111,8.41067583807915));
#90023=CARTESIAN_POINT('Ctrl Pts',(3.52053785707391,224.10412524546,8.25191797284736));
#90024=CARTESIAN_POINT('Ctrl Pts',(1.15689718192732,221.556401984935,8.09316010761557));
#90025=CARTESIAN_POINT('Ctrl Pts',(-2.26553574862528,222.160259492381,7.93440224238377));
#90026=CARTESIAN_POINT('Ctrl Pts',(-3.61455045112604,225.36304740073,7.77564437715198));
#90027=CARTESIAN_POINT('Ctrl Pts',(-1.65552872289502,228.233574342207,7.61688651192019));
#90028=CARTESIAN_POINT('Ctrl Pts',(1.81863282742744,228.144734172854,7.4581286466884));
#90029=CARTESIAN_POINT('Ctrl Pts',(3.62838168560431,225.177833412168,7.2993707814566));
#90030=CARTESIAN_POINT('Ctrl Pts',(2.11743576779875,222.048179519659,7.14061291622482));
#90031=CARTESIAN_POINT('Ctrl Pts',(-1.33138728143009,221.620031614681,6.98185505099302));
#90032=CARTESIAN_POINT('Ctrl Pts',(-3.56172474304964,224.285230643032,6.82309718576122));
#90033=CARTESIAN_POINT('Ctrl Pts',(-2.53237185989158,227.604586558773,6.66433932052944));
#90034=CARTESIAN_POINT('Ctrl Pts',(0.814607649856128,228.540224958348,6.50558145529764));
#90035=CARTESIAN_POINT('Ctrl Pts',(3.41605827048919,226.235849615258,6.34682359006585));
#90036=CARTESIAN_POINT('Ctrl Pts',(2.89113249630378,222.800424752883,6.18806572483406));
#90037=CARTESIAN_POINT('Ctrl Pts',(-0.279757624807835,221.378051070173,
6.02930785960226));
#90038=CARTESIAN_POINT('Ctrl Pts',(-3.19461357869652,223.270484905611,5.87054999437047));
#90039=CARTESIAN_POINT('Ctrl Pts',(-3.18575931098727,226.745770887422,5.71179212913868));
#90040=CARTESIAN_POINT('Ctrl Pts',(-0.261298247139434,228.623327421715,
5.55303426390689));
#90041=CARTESIAN_POINT('Ctrl Pts',(2.9023029622151,227.184814842139,5.39427639867509));
#90042=CARTESIAN_POINT('Ctrl Pts',(3.40971661468071,223.746759804953,5.2355185334433));
#90043=CARTESIAN_POINT('Ctrl Pts',(0.796557755474301,221.455670144991,5.07676066821152));
#90044=CARTESIAN_POINT('Ctrl Pts',(-2.54561073021817,222.408351028957,4.91800280297971));
#90045=CARTESIAN_POINT('Ctrl Pts',(-3.55803637571897,225.732908949305,4.75924493774792));
#90046=CARTESIAN_POINT('Ctrl Pts',(-1.31414727007755,228.386708628075,4.60048707251613));
#90047=CARTESIAN_POINT('Ctrl Pts',(2.13244936546002,227.9409927036,4.44172920728434));
#90048=CARTESIAN_POINT('Ctrl Pts',(3.62742842558762,224.80368037246,4.28297134205255));
#90049=CARTESIAN_POINT('Ctrl Pts',(1.80258513325755,221.846039756688,4.12421347682075));
#90050=CARTESIAN_POINT('Ctrl Pts',(-1.67198400213467,221.774903431643,3.96545561158896));
#90051=CARTESIAN_POINT('Ctrl Pts',(-3.61635344454317,224.655375358983,3.80669774635717));
#90052=CARTESIAN_POINT('Ctrl Pts',(-2.25103635667323,227.851247744537,3.64793988112538));
#90053=CARTESIAN_POINT('Ctrl Pts',(1.17442911621855,228.437658305789,3.48918201589358));
#90054=CARTESIAN_POINT('Ctrl Pts',(3.52505710830432,225.877924122033,3.33042415066179));
#90055=CARTESIAN_POINT('Ctrl Pts',(2.64955297313634,222.514713813743,3.17166628543));
#90056=CARTESIAN_POINT('Ctrl Pts',(-0.650821938137665,221.426037330607,
3.01290842019821));
#90057=CARTESIAN_POINT('Ctrl Pts',(-3.35556463867761,223.60825133135,2.85415055496642));
#90058=CARTESIAN_POINT('Ctrl Pts',(-2.98929471089608,227.064193680453,2.69539268973462));
#90059=CARTESIAN_POINT('Ctrl Pts',(0.112777612738978,228.630986010631,2.53663482450283));
#90060=CARTESIAN_POINT('Ctrl Pts',(3.11163588183028,226.874700175507,2.37787695927104));
#90061=CARTESIAN_POINT('Ctrl Pts',(3.26272508945618,223.402688633055,2.21911909403925));
#90062=CARTESIAN_POINT('Ctrl Pts',(0.42776847383237,221.392536757232,2.06036122880745));
#90063=CARTESIAN_POINT('Ctrl Pts',(-2.7986819344071,222.683934355202,1.90160336357566));
#90064=CARTESIAN_POINT('Ctrl Pts',(-3.46377853880955,226.09499665142,1.74284549834387));
#90065=CARTESIAN_POINT('Ctrl Pts',(-0.958825582149559,228.5039149863,1.58408763311207));
#90066=CARTESIAN_POINT('Ctrl Pts',(2.42364536547895,227.706056696193,1.42532976788028));
#90067=CARTESIAN_POINT('Ctrl Pts',(3.58799443175235,224.431602766551,1.26657190264849));
#90068=CARTESIAN_POINT('Ctrl Pts',(1.46861466513916,221.677371668161,1.1078140374167));
#90069=CARTESIAN_POINT('Ctrl Pts',(-1.99484835403995,221.963957684538,0.949056172184904));
#90070=CARTESIAN_POINT('Ctrl Pts',(-3.63261167939862,225.029235526384,0.790298306953113));
#90071=CARTESIAN_POINT('Ctrl Pts',(-1.94583850483642,228.067541710309,0.631540441721317));
#90072=CARTESIAN_POINT('Ctrl Pts',(1.52182603612892,228.298871095165,0.472782576489527));
#90073=CARTESIAN_POINT('Ctrl Pts',(3.59659353011021,225.51018574291,0.314024711257735));
#90074=CARTESIAN_POINT('Ctrl Pts',(2.38000618637172,222.256382496769,0.155266846025939));
#90075=CARTESIAN_POINT('Ctrl Pts',(-1.01525930202285,221.509861473209,-0.00349101920584771));
#90076=CARTESIAN_POINT('Ctrl Pts',(-3.48036060104862,223.965090769095,-0.162248884437644));
#90077=CARTESIAN_POINT('Ctrl Pts',(-3.00016881161633,226.220556762668,-0.268087461258838));
#90078=CARTESIAN_POINT('Ctrl Pts',(-2.33606265769611,226.997301556931,-0.321006749669435));
#90079=CARTESIAN_POINT('Ctrl Pts',(-0.745932854346946,222.209822430158,
20.1070022498898));
#90080=CARTESIAN_POINT('Ctrl Pts',(-1.67367162680846,222.457846368889,20.0540829614792));
#90081=CARTESIAN_POINT('Ctrl Pts',(-3.24608648461372,223.948899041869,19.948244384658));
#90082=CARTESIAN_POINT('Ctrl Pts',(-2.64397303763859,227.162384946822,19.7894865194262));
#90083=CARTESIAN_POINT('Ctrl Pts',(0.382710416331961,228.39152127458,19.6307286541944));
#90084=CARTESIAN_POINT('Ctrl Pts',(3.05679586286989,226.519320186158,19.4719707889626));
#90085=CARTESIAN_POINT('Ctrl Pts',(2.93445374306217,223.255371927948,19.3132129237308));
#90086=CARTESIAN_POINT('Ctrl Pts',(0.125932567732614,221.588730023197,19.1544550584991));
#90087=CARTESIAN_POINT('Ctrl Pts',(-2.79756284715621,223.043775614427,18.9956971932672));
#90088=CARTESIAN_POINT('Ctrl Pts',(-3.16086635442269,226.289308682979,18.8369393280355));
#90089=CARTESIAN_POINT('Ctrl Pts',(-0.631277392441138,228.354792143898,
18.6781814628037));
#90090=CARTESIAN_POINT('Ctrl Pts',(2.47602327538317,227.350006577922,18.5194235975719));
#90091=CARTESIAN_POINT('Ctrl Pts',(3.31728395524864,224.194477056596,18.3606657323401));
#90092=CARTESIAN_POINT('Ctrl Pts',(1.12255840621658,221.776170978336,18.2019078671083));
#90093=CARTESIAN_POINT('Ctrl Pts',(-2.09952857166804,222.308308722862,18.0431500018765));
#90094=CARTESIAN_POINT('Ctrl Pts',(-3.40012904328763,225.30388437072,17.8843921366447));
#90095=CARTESIAN_POINT('Ctrl Pts',(-1.58893058309745,228.021343994616,17.7256342714129));
#90096=CARTESIAN_POINT('Ctrl Pts',(1.67645660903848,227.973670235318,17.5668764061811));
#90097=CARTESIAN_POINT('Ctrl Pts',(3.40755101251001,225.204493336622,17.4081185409494));
#90098=CARTESIAN_POINT('Ctrl Pts',(2.02005474810658,222.248164270826,17.2493606757175));
#90099=CARTESIAN_POINT('Ctrl Pts',(-1.21619548558992,221.81031509385,17.0906028104858));
#90100=CARTESIAN_POINT('Ctrl Pts',(-3.33938368663811,224.291665448231,16.931844945254));
#90101=CARTESIAN_POINT('Ctrl Pts',(-2.40636805523639,227.42128354143,16.7730870800222));
#90102=CARTESIAN_POINT('Ctrl Pts',(0.728955518915619,228.334943040165,16.6143292147904));
#90103=CARTESIAN_POINT('Ctrl Pts',(3.19713903415707,226.196462796022,16.4555713495586));
#90104=CARTESIAN_POINT('Ctrl Pts',(2.73930102941996,222.962979849813,16.2968134843268));
#90105=CARTESIAN_POINT('Ctrl Pts',(-0.225545168913144,221.593777664063,
16.138055619095));
#90106=CARTESIAN_POINT('Ctrl Pts',(-2.98397243792452,223.341950026654,15.9792977538632));
#90107=CARTESIAN_POINT('Ctrl Pts',(-3.01146824889316,226.607569659434,15.8205398886314));
#90108=CARTESIAN_POINT('Ctrl Pts',(-0.282868436994453,228.401941603223,
15.6617820233996));
#90109=CARTESIAN_POINT('Ctrl Pts',(2.7046125573656,227.082856725468,15.5030241581678));
#90110=CARTESIAN_POINT('Ctrl Pts',(3.21683224555754,223.857541454497,15.344266292936));
#90111=CARTESIAN_POINT('Ctrl Pts',(0.785007189125602,221.677804199431,15.1855084277042));
#90112=CARTESIAN_POINT('Ctrl Pts',(-2.36525641593009,222.538540410411,15.0267505624725));
#90113=CARTESIAN_POINT('Ctrl Pts',(-3.35083744213523,225.652004340984,14.8679926972406));
#90114=CARTESIAN_POINT('Ctrl Pts',(-1.26973217306808,228.168753924331,14.7092348320089));
#90115=CARTESIAN_POINT('Ctrl Pts',(1.97343193086066,227.785460040736,14.5504769667771));
#90116=CARTESIAN_POINT('Ctrl Pts',(3.41051120926871,224.852913237397,14.3917191015453));
#90117=CARTESIAN_POINT('Ctrl Pts',(1.72629076306928,222.054980233407,14.2329612363135));
#90118=CARTESIAN_POINT('Ctrl Pts',(-1.53783092160648,221.952329203993,14.0742033710817));
#90119=CARTESIAN_POINT('Ctrl Pts',(-3.3945298073017,224.638906367238,13.9154455058499));
#90120=CARTESIAN_POINT('Ctrl Pts',(-2.14455514684108,227.655956408987,13.7566876406181));
#90121=CARTESIAN_POINT('Ctrl Pts',(1.06811629967593,228.242275249674,13.5979297753863));
#90122=CARTESIAN_POINT('Ctrl Pts',(3.30324775073217,225.861263909359,13.4391719101545));
#90123=CARTESIAN_POINT('Ctrl Pts',(2.51524699021539,222.692023873067,13.2804140449227));
#90124=CARTESIAN_POINT('Ctrl Pts',(-0.574707716836846,221.635043497385,
13.1216561796909));
#90125=CARTESIAN_POINT('Ctrl Pts',(-3.13868994403982,223.657671180573,12.9628983144591));
#90126=CARTESIAN_POINT('Ctrl Pts',(-2.83014325788355,226.908798146515,12.8041404492274));
#90127=CARTESIAN_POINT('Ctrl Pts',(0.068550426595048,228.412993123827,12.6453825839956));
#90128=CARTESIAN_POINT('Ctrl Pts',(2.90450676334955,226.793616928427,12.4866247187638));
#90129=CARTESIAN_POINT('Ctrl Pts',(3.08225862450349,223.532722590661,12.327866853532));
#90130=CARTESIAN_POINT('Ctrl Pts',(0.439127513718703,221.614680480224,12.1691089883002));
#90131=CARTESIAN_POINT('Ctrl Pts',(-2.60589308035317,222.794882661161,12.0103511230684));
#90132=CARTESIAN_POINT('Ctrl Pts',(-3.26600042976007,225.993208143889,11.8515932578366));
#90133=CARTESIAN_POINT('Ctrl Pts',(-0.937064314282925,228.282549572387,
11.6928353926048));
#90134=CARTESIAN_POINT('Ctrl Pts',(2.2494730247768,227.567701761319,11.534077527373));
#90135=CARTESIAN_POINT('Ctrl Pts',(3.37729274001918,224.502893399264,11.3753196621412));
#90136=CARTESIAN_POINT('Ctrl Pts',(1.41421427240481,221.893036978655,11.2165617969094));
#90137=CARTESIAN_POINT('Ctrl Pts',(-1.84315304170182,222.126672993002,11.0578039316776));
#90138=CARTESIAN_POINT('Ctrl Pts',(-3.41366676452317,224.989977771163,10.8990460664458));
#90139=CARTESIAN_POINT('Ctrl Pts',(-1.85999279869212,227.862454892762,10.7402882012141));
#90140=CARTESIAN_POINT('Ctrl Pts',(1.39594650335951,228.115213409068,10.5815303359823));
#90141=CARTESIAN_POINT('Ctrl Pts',(3.37431562043079,225.516928735899,10.4227724707505));
#90142=CARTESIAN_POINT('Ctrl Pts',(2.26451121437554,222.445550903962,10.2640146055187));
#90143=CARTESIAN_POINT('Ctrl Pts',(-0.91777376602647,221.712004784268,10.1052567402869));
#90144=CARTESIAN_POINT('Ctrl Pts',(-3.26011223185162,223.987631756715,9.9464988750551));
#90145=CARTESIAN_POINT('Ctrl Pts',(-2.61879611128699,227.189778105605,9.7877410098233));
#90146=CARTESIAN_POINT('Ctrl Pts',(0.419242107345829,228.387839618357,9.62898314459151));
#90147=CARTESIAN_POINT('Ctrl Pts',(3.07358996582205,226.485350445612,9.47022527935971));
#90148=CARTESIAN_POINT('Ctrl Pts',(2.91498840844391,223.223468603453,9.31146741412792));
#90149=CARTESIAN_POINT('Ctrl Pts',(0.0885895742870307,221.587468225553,
9.15270954889613));
#90150=CARTESIAN_POINT('Ctrl Pts',(-2.81888643477362,223.074616793433,8.99395168366434));
#90151=CARTESIAN_POINT('Ctrl Pts',(-3.14651768957949,226.323875996249,8.83519381843255));
#90152=CARTESIAN_POINT('Ctrl Pts',(-0.594456078616027,228.361523939358,
8.67643595320075));
#90153=CARTESIAN_POINT('Ctrl Pts',(2.50165171212042,227.322705305355,8.51767808796897));
#90154=CARTESIAN_POINT('Ctrl Pts',(3.30824795429932,224.158146867229,8.35892022273716));
#90155=CARTESIAN_POINT('Ctrl Pts',(1.08713579879716,221.76405238311,8.20016235750538));
#90156=CARTESIAN_POINT('Ctrl Pts',(-2.12892299701359,222.331497030718,8.04140449227358));
#90157=CARTESIAN_POINT('Ctrl Pts',(-3.39659154967535,225.341155490876,7.88264662704179));
#90158=CARTESIAN_POINT('Ctrl Pts',(-1.55569964964197,228.0385884592,7.72388876181));
#90159=CARTESIAN_POINT('Ctrl Pts',(1.70896850856733,227.955105389154,7.5651308965782));
#90160=CARTESIAN_POINT('Ctrl Pts',(3.40958875493938,225.167109983161,7.40637303134642));
#90161=CARTESIAN_POINT('Ctrl Pts',(1.98975350686972,222.22617552715,7.24761516611462));
#90162=CARTESIAN_POINT('Ctrl Pts',(-1.25110407244195,221.823845119614,7.08885730088283));
#90163=CARTESIAN_POINT('Ctrl Pts',(-3.34695125385322,224.328331533708,6.93009943565103));
#90164=CARTESIAN_POINT('Ctrl Pts',(-2.37966877935368,227.447528901739,6.77134157041924));
#90165=CARTESIAN_POINT('Ctrl Pts',(0.765486468432129,228.326747915146,6.61258370518745));
#90166=CARTESIAN_POINT('Ctrl Pts',(3.21006853041089,226.161327367432,6.45382583995566));
#90167=CARTESIAN_POINT('Ctrl Pts',(2.71679599959049,222.933060058712,6.29506797472387));
#90168=CARTESIAN_POINT('Ctrl Pts',(-0.26288812321973,221.596456102979,6.13631010949208));
#90169=CARTESIAN_POINT('Ctrl Pts',(-3.00197704599707,223.374775387958,5.97755224426028));
#90170=CARTESIAN_POINT('Ctrl Pts',(-2.99365669432777,226.640500173968,5.81879437902849));
#90171=CARTESIAN_POINT('Ctrl Pts',(-0.245541853732399,228.404839265273,
5.66003651379669));
#90172=CARTESIAN_POINT('Ctrl Pts',(2.72729288174315,227.053069594893,5.50127864856491));
#90173=CARTESIAN_POINT('Ctrl Pts',(3.2041092790956,223.822330712001,5.34252078333311));
#90174=CARTESIAN_POINT('Ctrl Pts',(0.748524990218216,221.669394715176,5.18376291810132));
#90175=CARTESIAN_POINT('Ctrl Pts',(-2.39210934027172,222.564628544048,5.02500505286953));
#90176=CARTESIAN_POINT('Ctrl Pts',(-3.34348529661266,225.688714233638,4.86624718763773));
#90177=CARTESIAN_POINT('Ctrl Pts',(-1.2349036409725,228.182488683689,4.70748932240594));
#90178=CARTESIAN_POINT('Ctrl Pts',(2.00386177832312,227.763649615568,4.54873145717415));
#90179=CARTESIAN_POINT('Ctrl Pts',(3.40869297689972,224.815518527974,4.38997359194236));
#90180=CARTESIAN_POINT('Ctrl Pts',(1.69388849705656,222.036224876289,4.23121572671056));
#90181=CARTESIAN_POINT('Ctrl Pts',(-1.57116266867262,221.969378101347,4.07245786147877));
#90182=CARTESIAN_POINT('Ctrl Pts',(-3.39828582183659,224.676156368734,3.91369999624698));
#90183=CARTESIAN_POINT('Ctrl Pts',(-2.11529792445043,227.679316315009,3.75494213101518));
#90184=CARTESIAN_POINT('Ctrl Pts',(1.10361055013022,228.230366074564,3.5961842657834));
#90185=CARTESIAN_POINT('Ctrl Pts',(3.31249469279354,225.824984930898,3.4374264005516));
#90186=CARTESIAN_POINT('Ctrl Pts',(2.48978382254105,222.664577608501,3.27866853531981));
#90187=CARTESIAN_POINT('Ctrl Pts',(-0.611577103518663,221.641548771872,
3.11991067008801));
#90188=CARTESIAN_POINT('Ctrl Pts',(-3.15322268985653,223.692174357191,2.96115280485623));
#90189=CARTESIAN_POINT('Ctrl Pts',(-2.80903899165545,226.939721939622,2.80239493962443));
#90190=CARTESIAN_POINT('Ctrl Pts',(0.105977075600772,228.41203603808,2.64363707439264));
#90191=CARTESIAN_POINT('Ctrl Pts',(2.92400293889902,226.761654972147,2.48487920916085));
#90192=CARTESIAN_POINT('Ctrl Pts',(3.06598140421811,223.499007175436,2.32612134392906));
#90193=CARTESIAN_POINT('Ctrl Pts',(0.401973856246465,221.610068297059,2.16736347869726));
#90194=CARTESIAN_POINT('Ctrl Pts',(-2.62992024517871,222.823594080652,2.00860561346547));
#90195=CARTESIAN_POINT('Ctrl Pts',(-3.25491124662603,226.028967896126,1.84984774823368));
#90196=CARTESIAN_POINT('Ctrl Pts',(-0.901007999190373,228.292627449574,
1.69108988300189));
#90197=CARTESIAN_POINT('Ctrl Pts',(2.27749853795265,227.542880347504,1.53233201777009));
#90198=CARTESIAN_POINT('Ctrl Pts',(3.3716368693583,224.465877357061,1.3735741525383));
#90199=CARTESIAN_POINT('Ctrl Pts',(1.38005658761437,221.877727543927,1.2148162873065));
#90200=CARTESIAN_POINT('Ctrl Pts',(-1.8745581653467,222.147032303853,1.05605842207472));
#90201=CARTESIAN_POINT('Ctrl Pts',(-3.41356367834167,225.027472611936,0.897300556842921));
#90202=CARTESIAN_POINT('Ctrl Pts',(-1.82850363051409,227.882567664331,0.738542691611129));
#90203=CARTESIAN_POINT('Ctrl Pts',(1.43005929071516,228.09994779069,0.579784826379336));
#90204=CARTESIAN_POINT('Ctrl Pts',(3.37971743849465,225.479421329585,0.421026961147546));
#90205=CARTESIAN_POINT('Ctrl Pts',(2.23649081956702,222.421823777806,0.262269095915749));
#90206=CARTESIAN_POINT('Ctrl Pts',(-0.954038742191529,221.720318283674,
0.103511230683963));
#90207=CARTESIAN_POINT('Ctrl Pts',(-3.27049340358829,224.027496227842,-0.0552466345478343));
#90208=CARTESIAN_POINT('Ctrl Pts',(-2.81925737956181,226.146956680238,-0.161085211369028));
#90209=CARTESIAN_POINT('Ctrl Pts',(-2.19519710401908,226.876863439079,-0.214004499779625));
#90210=CARTESIAN_POINT('Ctrl Pts',(-0.698066426161029,222.388867814061,
20.2140044997796));
#90211=CARTESIAN_POINT('Ctrl Pts',(-1.56627230491966,222.620976084267,20.161085211369));
#90212=CARTESIAN_POINT('Ctrl Pts',(-3.03778547642569,224.016348073287,20.0552466345478));
#90213=CARTESIAN_POINT('Ctrl Pts',(-2.47430958228317,227.023624945618,19.896488769316));
#90214=CARTESIAN_POINT('Ctrl Pts',(0.358151931539931,228.173887732117,19.7377309040843));
#90215=CARTESIAN_POINT('Ctrl Pts',(2.86064161279711,226.421825579025,19.5789730388524));
#90216=CARTESIAN_POINT('Ctrl Pts',(2.74615017319171,223.367324517025,19.4202151736207));
#90217=CARTESIAN_POINT('Ctrl Pts',(0.117851488886823,221.807630837682,19.2614573083889));
#90218=CARTESIAN_POINT('Ctrl Pts',(-2.61804355082996,223.169306315376,19.1026994431571));
#90219=CARTESIAN_POINT('Ctrl Pts',(-2.9580339124977,226.206573888388,18.9439415779253));
#90220=CARTESIAN_POINT('Ctrl Pts',(-0.590768392476075,228.139515505661,
18.7851837126935));
#90221=CARTESIAN_POINT('Ctrl Pts',(2.31713713756645,227.199206917547,18.6264258474617));
#90222=CARTESIAN_POINT('Ctrl Pts',(3.10441421329951,224.24616737416,18.4676679822299));
#90223=CARTESIAN_POINT('Ctrl Pts',(1.05052395831347,221.983043727605,18.3089101169981));
#90224=CARTESIAN_POINT('Ctrl Pts',(-1.96480205705699,222.481034252332,18.1501522517663));
#90225=CARTESIAN_POINT('Ctrl Pts',(-3.18194314126583,225.284384144496,17.9913943865345));
#90226=CARTESIAN_POINT('Ctrl Pts',(-1.48696908454564,227.827464686981,17.8326365213028));
#90227=CARTESIAN_POINT('Ctrl Pts',(1.56887857515016,227.782850147507,17.6738786560709));
#90228=CARTESIAN_POINT('Ctrl Pts',(3.18888884354982,225.191371021987,17.5151207908392));
#90229=CARTESIAN_POINT('Ctrl Pts',(1.89042805990215,222.424749263084,17.3563629256074));
#90230=CARTESIAN_POINT('Ctrl Pts',(-1.13815235673217,222.01499681903,17.1976050603756));
#90231=CARTESIAN_POINT('Ctrl Pts',(-3.12509580738706,224.337119197528,17.0388471951438));
#90232=CARTESIAN_POINT('Ctrl Pts',(-2.2519516851387,227.265910046244,16.880089329912));
#90233=CARTESIAN_POINT('Ctrl Pts',(0.682178524453497,228.120940116704,16.7213314646802));
#90234=CARTESIAN_POINT('Ctrl Pts',(2.99197897841337,226.119685911656,16.5625735994484));
#90235=CARTESIAN_POINT('Ctrl Pts',(2.56352038744898,223.093695205979,16.4038157342166));
#90236=CARTESIAN_POINT('Ctrl Pts',(-0.211071960543857,221.812354571995,
16.2450578689848));
#90237=CARTESIAN_POINT('Ctrl Pts',(-2.79249125891984,223.44834690878,16.086300003753));
#90238=CARTESIAN_POINT('Ctrl Pts',(-2.81822266676094,226.50441209343,15.9275421385212));
#90239=CARTESIAN_POINT('Ctrl Pts',(-0.264716800896706,228.183639389432,
15.7687842732894));
#90240=CARTESIAN_POINT('Ctrl Pts',(2.53105787078296,226.949200041371,15.6100264080576));
#90241=CARTESIAN_POINT('Ctrl Pts',(3.01040847863157,223.930852892121,15.4512685428258));
#90242=CARTESIAN_POINT('Ctrl Pts',(0.734633365228797,221.890989133948,15.292510677594));
#90243=CARTESIAN_POINT('Ctrl Pts',(-2.21347817514792,222.696491998132,15.1337528123623));
#90244=CARTESIAN_POINT('Ctrl Pts',(-3.13581457666957,225.61016529504,14.9749949471305));
#90245=CARTESIAN_POINT('Ctrl Pts',(-1.18825360093744,227.965415337923,14.8162370818987));
#90246=CARTESIAN_POINT('Ctrl Pts',(1.84679702364634,227.60671738015,14.6574792166669));
#90247=CARTESIAN_POINT('Ctrl Pts',(3.19165908481221,224.862351778571,14.4987213514351));
#90248=CARTESIAN_POINT('Ctrl Pts',(1.61551487706703,222.243961823831,14.3399634862033));
#90249=CARTESIAN_POINT('Ctrl Pts',(-1.43914848264138,222.147897899542,14.1812056209715));
#90250=CARTESIAN_POINT('Ctrl Pts',(-3.1767032076295,224.662077705436,14.0224477557397));
#90251=CARTESIAN_POINT('Ctrl Pts',(-2.00693928191597,227.485523982027,13.8636898905079));
#90252=CARTESIAN_POINT('Ctrl Pts',(0.999575395686113,228.034218808007,13.7049320252761));
#90253=CARTESIAN_POINT('Ctrl Pts',(3.0912787104636,225.805996700218,13.5461741600443));
#90254=CARTESIAN_POINT('Ctrl Pts',(2.35384387098638,222.840126444083,13.3874162948126));
#90255=CARTESIAN_POINT('Ctrl Pts',(-0.537828786654925,221.850972381389,
13.2286584295807));
#90256=CARTESIAN_POINT('Ctrl Pts',(-2.93728055989923,223.743808271415,13.069900564349));
#90257=CARTESIAN_POINT('Ctrl Pts',(-2.64853328022953,226.786310782043,12.9111426991172));
#90258=CARTESIAN_POINT('Ctrl Pts',(0.0641515533551816,228.19398173519,12.7523848338854));
#90259=CARTESIAN_POINT('Ctrl Pts',(2.71812488783194,226.678520729892,12.5936269686536));
#90260=CARTESIAN_POINT('Ctrl Pts',(2.88447043185256,223.626877618602,12.4348691034218));
#90261=CARTESIAN_POINT('Ctrl Pts',(0.410948750070758,221.831916056771,12.27611123819));
#90262=CARTESIAN_POINT('Ctrl Pts',(-2.43867321161564,222.936384795201,12.1173533729582));
#90263=CARTESIAN_POINT('Ctrl Pts',(-3.05642154592989,225.929474087914,11.9585955077264));
#90264=CARTESIAN_POINT('Ctrl Pts',(-0.876933001599986,228.071908731918,
11.7998376424946));
#90265=CARTESIAN_POINT('Ctrl Pts',(2.10512459130967,227.402932625271,11.6410797772628));
#90266=CARTESIAN_POINT('Ctrl Pts',(3.16057224103474,224.534792674469,11.482321912031));
#90267=CARTESIAN_POINT('Ctrl Pts',(1.32346430005129,222.092410449699,11.3235640467992));
#90268=CARTESIAN_POINT('Ctrl Pts',(-1.72487811629514,222.311054067027,11.1648061815675));
#90269=CARTESIAN_POINT('Ctrl Pts',(-3.19461214843743,224.990620896471,11.0060483163357));
#90270=CARTESIAN_POINT('Ctrl Pts',(-1.74063726795488,227.678771481096,10.8472904511039));
#90271=CARTESIAN_POINT('Ctrl Pts',(1.30636877171108,227.915310511562,10.6885325858721));
#90272=CARTESIAN_POINT('Ctrl Pts',(3.15778616287877,225.483757476488,10.5297747206403));
#90273=CARTESIAN_POINT('Ctrl Pts',(2.11919778195673,222.609469617956,10.3710168554085));
#90274=CARTESIAN_POINT('Ctrl Pts',(-0.858880325676687,221.922995071065,
10.2122589901767));
#90275=CARTESIAN_POINT('Ctrl Pts',(-3.05091119302543,224.052595314135,10.0535011249449));
#90276=CARTESIAN_POINT('Ctrl Pts',(-2.45074825649149,227.049260288453,9.8947432597131));
#90277=CARTESIAN_POINT('Ctrl Pts',(0.392339388010119,228.170442327365,9.73598539448133));
#90278=CARTESIAN_POINT('Ctrl Pts',(2.87635804003325,226.390035672946,9.57722752924952));
#90279=CARTESIAN_POINT('Ctrl Pts',(2.72793392692798,223.33746842531,9.41846966401774));
#90280=CARTESIAN_POINT('Ctrl Pts',(0.0829047911716047,221.806450009452,
9.25971179878593));
#90281=CARTESIAN_POINT('Ctrl Pts',(-2.63799880620485,223.198168419361,9.10095393355416));
#90282=CARTESIAN_POINT('Ctrl Pts',(-2.94460599987943,226.238923021015,8.94219606832235));
#90283=CARTESIAN_POINT('Ctrl Pts',(-0.556309898258184,228.145815322556,
8.78343820309056));
#90284=CARTESIAN_POINT('Ctrl Pts',(2.34112100037261,227.1736575646,8.62468033785877));
#90285=CARTESIAN_POINT('Ctrl Pts',(3.09595805152473,224.212168488999,8.46592247262698));
#90286=CARTESIAN_POINT('Ctrl Pts',(1.017374415667,221.971702781286,8.30716460739518));
#90287=CARTESIAN_POINT('Ctrl Pts',(-1.99231024540189,222.502734569055,8.1484067421634));
#90288=CARTESIAN_POINT('Ctrl Pts',(-3.17863264822466,225.319263581023,7.9896488769316));
#90289=CARTESIAN_POINT('Ctrl Pts',(-1.45587057638894,227.843602576193,7.83089101169981));
#90290=CARTESIAN_POINT('Ctrl Pts',(1.59930418970722,227.765476605454,7.67213314646802));
#90291=CARTESIAN_POINT('Ctrl Pts',(3.19079582427445,225.156386554153,7.51337528123622));
#90292=CARTESIAN_POINT('Ctrl Pts',(1.86207124594069,222.404171534641,7.35461741600444));
#90293=CARTESIAN_POINT('Ctrl Pts',(-1.17082086345382,222.027658624547,7.19585955077263));
#90294=CARTESIAN_POINT('Ctrl Pts',(-3.1321777646568,224.371432424383,7.03710168554085));
#90295=CARTESIAN_POINT('Ctrl Pts',(-2.22696569881578,227.290471244706,6.87834382030905));
#90296=CARTESIAN_POINT('Ctrl Pts',(0.71636528700813,228.113270871944,6.71958595507726));
#90297=CARTESIAN_POINT('Ctrl Pts',(3.00407879033259,226.086805119606,6.56082808984547));
#90298=CARTESIAN_POINT('Ctrl Pts',(2.54245950287719,223.065695364541,6.40207022461367));
#90299=CARTESIAN_POINT('Ctrl Pts',(-0.246018621631624,221.814861135784,
6.24331235938189));
#90300=CARTESIAN_POINT('Ctrl Pts',(-2.80934051329762,223.479065870305,6.08455449415009));
#90301=CARTESIAN_POINT('Ctrl Pts',(-2.80155407766827,226.535229460513,5.9257966289183));
#90302=CARTESIAN_POINT('Ctrl Pts',(-0.229785460325367,228.186351108831,
5.7670387636865));
#90303=CARTESIAN_POINT('Ctrl Pts',(2.55228280127121,226.921324347647,5.60828089845472));
#90304=CARTESIAN_POINT('Ctrl Pts',(2.99850194351049,223.897901619051,5.44952303322292));
#90305=CARTESIAN_POINT('Ctrl Pts',(0.700492224962129,221.88311928536,5.29076516799113));
#90306=CARTESIAN_POINT('Ctrl Pts',(-2.23860795032526,222.72090605914,5.13200730275934));
#90307=CARTESIAN_POINT('Ctrl Pts',(-3.12893421750635,225.64451951797,4.97324943752754));
#90308=CARTESIAN_POINT('Ctrl Pts',(-1.15566001186744,227.978268739303,4.81449157229575));
#90309=CARTESIAN_POINT('Ctrl Pts',(1.87527419118623,227.586306527535,4.65573370706396));
#90310=CARTESIAN_POINT('Ctrl Pts',(3.18995752821183,224.827356683487,4.49697584183217));
#90311=CARTESIAN_POINT('Ctrl Pts',(1.58519186085557,222.22640999589,4.33821797660037));
#90312=CARTESIAN_POINT('Ctrl Pts',(-1.47034133521057,222.163852771051,4.17946011136858));
#90313=CARTESIAN_POINT('Ctrl Pts',(-3.18021819913001,224.696937378484,4.02070224613679));
#90314=CARTESIAN_POINT('Ctrl Pts',(-1.97955949222763,227.507384885481,3.86194438090499));
#90315=CARTESIAN_POINT('Ctrl Pts',(1.03279198404188,228.023073843338,3.70318651567321));
#90316=CARTESIAN_POINT('Ctrl Pts',(3.09993227728275,225.772045739765,3.54442865044141));
#90317=CARTESIAN_POINT('Ctrl Pts',(2.33001467194577,222.814441403258,3.38567078520962));
#90318=CARTESIAN_POINT('Ctrl Pts',(-0.57233226889966,221.857060213137,3.22691291997783));
#90319=CARTESIAN_POINT('Ctrl Pts',(-2.95088074103546,223.776097383032,3.06815505474604));
#90320=CARTESIAN_POINT('Ctrl Pts',(-2.62878327241482,226.815250198791,2.90939718951424));
#90321=CARTESIAN_POINT('Ctrl Pts',(0.0991765384625657,228.193086065528,
2.75063932428245));
#90322=CARTESIAN_POINT('Ctrl Pts',(2.73636999596777,226.648609768787,2.59188145905066));
#90323=CARTESIAN_POINT('Ctrl Pts',(2.86923771898004,223.595325717816,2.43312359381887));
#90324=CARTESIAN_POINT('Ctrl Pts',(0.376179238660561,221.827599836887,2.27436572858707));
#90325=CARTESIAN_POINT('Ctrl Pts',(-2.46115855595033,222.963253806101,2.11560786335528));
#90326=CARTESIAN_POINT('Ctrl Pts',(-3.04604395444252,225.962939140832,1.95684999812349));
#90327=CARTESIAN_POINT('Ctrl Pts',(-0.843190416231185,228.081339912848,
1.7980921328917));
#90328=CARTESIAN_POINT('Ctrl Pts',(2.13135171042635,227.379703998816,1.6393342676599));
#90329=CARTESIAN_POINT('Ctrl Pts',(3.15527930696426,224.500151947571,1.48057640242811));
#90330=CARTESIAN_POINT('Ctrl Pts',(1.29149851008957,222.078083419693,1.32181853719631));
#90331=CARTESIAN_POINT('Ctrl Pts',(-1.75426797665344,222.330106923169,1.16306067196453));
#90332=CARTESIAN_POINT('Ctrl Pts',(-3.19451567728472,225.025709697487,1.00430280673273));
#90333=CARTESIAN_POINT('Ctrl Pts',(-1.71116875619176,227.697593618355,0.845544941500938));
#90334=CARTESIAN_POINT('Ctrl Pts',(1.33829254530139,227.901024486215,0.686787076269146));
#90335=CARTESIAN_POINT('Ctrl Pts',(3.16284134687909,225.448656916261,0.528029211037355));
#90336=CARTESIAN_POINT('Ctrl Pts',(2.09297545276232,222.587265058842,0.36927134580556));
#90337=CARTESIAN_POINT('Ctrl Pts',(-0.892818182360209,221.930775094139,
0.210513480573772));
#90338=CARTESIAN_POINT('Ctrl Pts',(-3.06062620612795,224.08990168659,0.0517556153419759));
#90339=CARTESIAN_POINT('Ctrl Pts',(-2.63834594750729,226.073356597808,-0.0540829614792177));
#90340=CARTESIAN_POINT('Ctrl Pts',(-2.05433155034205,226.756425321227,-0.107002249889815));
#90341=CARTESIAN_POINT('Ctrl Pts',(-0.650199997975112,222.567913197965,
20.3210067496694));
#90342=CARTESIAN_POINT('Ctrl Pts',(-1.45887298303087,222.784105799646,20.2680874612588));
#90343=CARTESIAN_POINT('Ctrl Pts',(-2.82948446823766,224.083797104705,20.1622488844376));
#90344=CARTESIAN_POINT('Ctrl Pts',(-2.30464612692774,226.884864944414,20.0034910192058));
#90345=CARTESIAN_POINT('Ctrl Pts',(0.3335934467479,227.956254189655,19.8447331539741));
#90346=CARTESIAN_POINT('Ctrl Pts',(2.66448736272432,226.324330971892,19.6859752887423));
#90347=CARTESIAN_POINT('Ctrl Pts',(2.55784660332125,223.479277106103,19.5272174235105));
#90348=CARTESIAN_POINT('Ctrl Pts',(0.109770410041031,222.026531652166,19.3684595582787));
#90349=CARTESIAN_POINT('Ctrl Pts',(-2.4385242545037,223.294837016326,19.2097016930469));
#90350=CARTESIAN_POINT('Ctrl Pts',(-2.75520147057272,226.123839093796,19.0509438278151));
#90351=CARTESIAN_POINT('Ctrl Pts',(-0.550259392511009,227.924238867424,
18.8921859625833));
#90352=CARTESIAN_POINT('Ctrl Pts',(2.15825099974972,227.048407257171,18.7334280973515));
#90353=CARTESIAN_POINT('Ctrl Pts',(2.89154447135037,224.297857691724,18.5746702321197));
#90354=CARTESIAN_POINT('Ctrl Pts',(0.97848951041037,222.189916476875,18.4159123668879));
#90355=CARTESIAN_POINT('Ctrl Pts',(-1.83007554244595,222.653759781801,18.2571545016561));
#90356=CARTESIAN_POINT('Ctrl Pts',(-2.96375723924402,225.264883918272,18.0983966364243));
#90357=CARTESIAN_POINT('Ctrl Pts',(-1.38500758599382,227.633585379346,17.9396387711926));
#90358=CARTESIAN_POINT('Ctrl Pts',(1.46130054126183,227.592030059696,17.7808809059607));
#90359=CARTESIAN_POINT('Ctrl Pts',(2.97022667458963,225.178248707351,17.622123040729));
#90360=CARTESIAN_POINT('Ctrl Pts',(1.76080137169772,222.601334255342,17.4633651754972));
#90361=CARTESIAN_POINT('Ctrl Pts',(-1.06010922787442,222.219678544209,17.3046073102654));
#90362=CARTESIAN_POINT('Ctrl Pts',(-2.910807928136,224.382572946825,17.1458494450336));
#90363=CARTESIAN_POINT('Ctrl Pts',(-2.09753531504101,227.110536551059,16.9870915798018));
#90364=CARTESIAN_POINT('Ctrl Pts',(0.635401529991375,227.906937193242,16.82833371457));
#90365=CARTESIAN_POINT('Ctrl Pts',(2.78681892266966,226.04290902729,16.6695758493382));
#90366=CARTESIAN_POINT('Ctrl Pts',(2.38773974547801,223.224410562146,16.5108179841064));
#90367=CARTESIAN_POINT('Ctrl Pts',(-0.196598752174572,222.030931479928,
16.3520601188746));
#90368=CARTESIAN_POINT('Ctrl Pts',(-2.60101007991516,223.554743790905,16.1933022536428));
#90369=CARTESIAN_POINT('Ctrl Pts',(-2.62497708462872,226.401254527426,16.034544388411));
#90370=CARTESIAN_POINT('Ctrl Pts',(-0.246565164798955,227.965337175641,
15.8757865231793));
#90371=CARTESIAN_POINT('Ctrl Pts',(2.35750318420032,226.815543357274,15.7170286579475));
#90372=CARTESIAN_POINT('Ctrl Pts',(2.80398471170561,224.004164329746,15.5582707927157));
#90373=CARTESIAN_POINT('Ctrl Pts',(0.68425954133199,222.104174068464,15.3995129274838));
#90374=CARTESIAN_POINT('Ctrl Pts',(-2.06169993436575,222.854443585853,15.2407550622521));
#90375=CARTESIAN_POINT('Ctrl Pts',(-2.92079171120392,225.568326249095,15.0819971970203));
#90376=CARTESIAN_POINT('Ctrl Pts',(-1.10677502880681,227.762076751515,14.9232393317885));
#90377=CARTESIAN_POINT('Ctrl Pts',(1.72016211643202,227.427974719564,14.7644814665567));
#90378=CARTESIAN_POINT('Ctrl Pts',(2.9728069603557,224.871790319746,14.6057236013249));
#90379=CARTESIAN_POINT('Ctrl Pts',(1.50473899106477,222.432943414254,14.4469657360931));
#90380=CARTESIAN_POINT('Ctrl Pts',(-1.34046604367627,222.34346659509,14.2882078708613));
#90381=CARTESIAN_POINT('Ctrl Pts',(-2.95887660795731,224.685249043634,14.1294500056295));
#90382=CARTESIAN_POINT('Ctrl Pts',(-1.86932341699085,227.315091555066,13.9706921403977));
#90383=CARTESIAN_POINT('Ctrl Pts',(0.931034491696291,227.826162366341,13.8119342751659));
#90384=CARTESIAN_POINT('Ctrl Pts',(2.87930967019502,225.750729491076,13.6531764099342));
#90385=CARTESIAN_POINT('Ctrl Pts',(2.19244075175736,222.9882290151,13.4944185447024));
#90386=CARTESIAN_POINT('Ctrl Pts',(-0.500949856473002,222.066901265393,
13.3356606794706));
#90387=CARTESIAN_POINT('Ctrl Pts',(-2.73587117575864,223.829945362257,13.1769028142388));
#90388=CARTESIAN_POINT('Ctrl Pts',(-2.46692330257551,226.663823417572,13.018144949007));
#90389=CARTESIAN_POINT('Ctrl Pts',(0.0597526801153146,227.974970346553,
12.8593870837752));
#90390=CARTESIAN_POINT('Ctrl Pts',(2.53174301231433,226.563424531357,12.7006292185434));
#90391=CARTESIAN_POINT('Ctrl Pts',(2.68668223920164,223.721032646543,12.5418713533116));
#90392=CARTESIAN_POINT('Ctrl Pts',(0.382769986422813,222.049151633319,12.3831134880798));
#90393=CARTESIAN_POINT('Ctrl Pts',(-2.27145334287811,223.077886929242,12.224355622848));
#90394=CARTESIAN_POINT('Ctrl Pts',(-2.84684266209971,225.865740031938,12.0655977576162));
#90395=CARTESIAN_POINT('Ctrl Pts',(-0.816801688917045,227.861267891448,
11.9068398923844));
#90396=CARTESIAN_POINT('Ctrl Pts',(1.96077615784255,227.238163489222,11.7480820271526));
#90397=CARTESIAN_POINT('Ctrl Pts',(2.9438517420503,224.566691949673,11.5893241619208));
#90398=CARTESIAN_POINT('Ctrl Pts',(1.23271432769777,222.291783920744,11.4305662966891));
#90399=CARTESIAN_POINT('Ctrl Pts',(-1.60660319088846,222.495435141052,11.2718084314573));
#90400=CARTESIAN_POINT('Ctrl Pts',(-2.97555753235169,224.991264021779,11.1130505662255));
#90401=CARTESIAN_POINT('Ctrl Pts',(-1.62128173721763,227.495088069431,10.9542927009937));
#90402=CARTESIAN_POINT('Ctrl Pts',(1.21679104006264,227.715407614056,10.7955348357619));
#90403=CARTESIAN_POINT('Ctrl Pts',(2.94125670532674,225.450586217078,10.6367769705301));
#90404=CARTESIAN_POINT('Ctrl Pts',(1.97388434953791,222.773388331949,10.4780191052983));
#90405=CARTESIAN_POINT('Ctrl Pts',(-0.799986885326904,222.133985357861,
10.3192612400665));
#90406=CARTESIAN_POINT('Ctrl Pts',(-2.84171015419925,224.117558871555,10.1605033748347));
#90407=CARTESIAN_POINT('Ctrl Pts',(-2.28270040169599,226.908742471301,10.0017455096029));
#90408=CARTESIAN_POINT('Ctrl Pts',(0.365436668674411,227.953045036372,9.84298764437113));
#90409=CARTESIAN_POINT('Ctrl Pts',(2.67912611424445,226.29472090028,9.68422977913933));
#90410=CARTESIAN_POINT('Ctrl Pts',(2.54087944541204,223.451468247167,9.52547191390754));
#90411=CARTESIAN_POINT('Ctrl Pts',(0.0772200080561768,222.025431793351,
9.36671404867575));
#90412=CARTESIAN_POINT('Ctrl Pts',(-2.45711117763608,223.321720045289,9.20795618344396));
#90413=CARTESIAN_POINT('Ctrl Pts',(-2.74269431017936,226.153970045781,9.04919831821217));
#90414=CARTESIAN_POINT('Ctrl Pts',(-0.51816371790034,227.930106705753,8.89044045298038));
#90415=CARTESIAN_POINT('Ctrl Pts',(2.18059028862479,227.024609823844,8.73168258774858));
#90416=CARTESIAN_POINT('Ctrl Pts',(2.88366814875014,224.266190110768,8.57292472251679));
#90417=CARTESIAN_POINT('Ctrl Pts',(0.947613032536847,222.179353179461,8.41416685728499));
#90418=CARTESIAN_POINT('Ctrl Pts',(-1.8556974937902,222.673972107392,8.25540899205321));
#90419=CARTESIAN_POINT('Ctrl Pts',(-2.96067374677397,225.297371671169,8.0966511268214));
#90420=CARTESIAN_POINT('Ctrl Pts',(-1.3560415031359,227.648616693186,7.93789326158962));
#90421=CARTESIAN_POINT('Ctrl Pts',(1.48963987084711,227.575847821754,7.77913539635783));
#90422=CARTESIAN_POINT('Ctrl Pts',(2.97200289360952,225.145663125145,7.62037753112604));
#90423=CARTESIAN_POINT('Ctrl Pts',(1.73438898501166,222.582167542132,7.46161966589423));
#90424=CARTESIAN_POINT('Ctrl Pts',(-1.09053765446568,222.23147212948,7.30286180066245));
#90425=CARTESIAN_POINT('Ctrl Pts',(-2.91740427546038,224.414533315059,7.14410393543066));
#90426=CARTESIAN_POINT('Ctrl Pts',(-2.07426261827787,227.133413587672,6.98534607019886));
#90427=CARTESIAN_POINT('Ctrl Pts',(0.667244105584131,227.899793828743,6.82658820496708));
#90428=CARTESIAN_POINT('Ctrl Pts',(2.79808905025428,226.012282871779,6.66783033973528));
#90429=CARTESIAN_POINT('Ctrl Pts',(2.3681230061639,223.19833067037,6.50907247450349));
#90430=CARTESIAN_POINT('Ctrl Pts',(-0.229149120043518,222.03326616859,6.35031460927169));
#90431=CARTESIAN_POINT('Ctrl Pts',(-2.61670398059818,223.583356352652,6.1915567440399));
#90432=CARTESIAN_POINT('Ctrl Pts',(-2.60945146100876,226.429958747059,6.03279887880811));
#90433=CARTESIAN_POINT('Ctrl Pts',(-0.214029066918333,227.967862952389,
5.87404101357631));
#90434=CARTESIAN_POINT('Ctrl Pts',(2.37727272079926,226.789579100402,5.71528314834453));
#90435=CARTESIAN_POINT('Ctrl Pts',(2.79289460792538,223.9734725261,5.55652528311272));
#90436=CARTESIAN_POINT('Ctrl Pts',(0.652459459706044,222.096843855544,5.39776741788095));
#90437=CARTESIAN_POINT('Ctrl Pts',(-2.08510656037881,222.877183574231,5.23900955264914));
#90438=CARTESIAN_POINT('Ctrl Pts',(-2.91438313840003,225.600324802303,5.08025168741736));
#90439=CARTESIAN_POINT('Ctrl Pts',(-1.07641638276239,227.774048794917,4.92149382218556));
#90440=CARTESIAN_POINT('Ctrl Pts',(1.74668660404933,227.408963439503,4.76273595695377));
#90441=CARTESIAN_POINT('Ctrl Pts',(2.97122207952394,224.839194839001,4.60397809172198));
#90442=CARTESIAN_POINT('Ctrl Pts',(1.47649522465458,222.416595115491,4.44522022649018));
#90443=CARTESIAN_POINT('Ctrl Pts',(-1.36952000174851,222.358327440755,4.28646236125839));
#90444=CARTESIAN_POINT('Ctrl Pts',(-2.96215057642344,224.717718388235,4.1277044960266));
#90445=CARTESIAN_POINT('Ctrl Pts',(-1.84382106000483,227.335453455953,3.96894663079481));
#90446=CARTESIAN_POINT('Ctrl Pts',(0.96197341795355,227.815781612112,3.81018876556301));
#90447=CARTESIAN_POINT('Ctrl Pts',(2.88736986177197,225.719106548631,3.65143090033122));
#90448=CARTESIAN_POINT('Ctrl Pts',(2.17024552135048,222.964305198015,3.49267303509943));
#90449=CARTESIAN_POINT('Ctrl Pts',(-0.533087434280658,222.072571654402,
3.33391516986763));
#90450=CARTESIAN_POINT('Ctrl Pts',(-2.74853879221438,223.860020408874,3.17515730463585));
#90451=CARTESIAN_POINT('Ctrl Pts',(-2.44852755317419,226.69077845796,3.01639943940405));
#90452=CARTESIAN_POINT('Ctrl Pts',(0.0923760013243574,227.974136092977,
2.85764157417226));
#90453=CARTESIAN_POINT('Ctrl Pts',(2.54873705303652,226.535564565427,2.69888370894047));
#90454=CARTESIAN_POINT('Ctrl Pts',(2.67249403374196,223.691644260197,2.54012584370867));
#90455=CARTESIAN_POINT('Ctrl Pts',(0.350384621074658,222.045131376714,2.38136797847688));
#90456=CARTESIAN_POINT('Ctrl Pts',(-2.29239686672194,223.102913531551,2.22261011324509));
#90457=CARTESIAN_POINT('Ctrl Pts',(-2.837176662259,225.896910385537,2.0638522480133));
#90458=CARTESIAN_POINT('Ctrl Pts',(-0.785372833271999,227.870052376122,
1.90509438278151));
#90459=CARTESIAN_POINT('Ctrl Pts',(1.98520488290005,227.216527650127,1.74633651754971));
#90460=CARTESIAN_POINT('Ctrl Pts',(2.93892174457021,224.534426538081,1.58757865231792));
#90461=CARTESIAN_POINT('Ctrl Pts',(1.20294043256477,222.27843929546,1.42882078708613));
#90462=CARTESIAN_POINT('Ctrl Pts',(-1.63397778796018,222.513181542484,1.27006292185433));
#90463=CARTESIAN_POINT('Ctrl Pts',(-2.97546767622777,225.023946783039,1.11130505662254));
#90464=CARTESIAN_POINT('Ctrl Pts',(-1.59383388186942,227.512619572377,0.952547191390748));
#90465=CARTESIAN_POINT('Ctrl Pts',(1.24652579988762,227.70210118174,0.793789326158957));
#90466=CARTESIAN_POINT('Ctrl Pts',(2.94596525526353,225.417892502936,0.635031460927166));
#90467=CARTESIAN_POINT('Ctrl Pts',(1.94946008595763,222.752706339879,0.47627359569537));
#90468=CARTESIAN_POINT('Ctrl Pts',(-0.83159762252889,222.141231904605,0.317515730463582));
#90469=CARTESIAN_POINT('Ctrl Pts',(-2.85075900866762,224.152307145338,0.158757865231786));
#90470=CARTESIAN_POINT('Ctrl Pts',(-2.45743451545277,225.999756515379,0.0529192884105924));
#90471=CARTESIAN_POINT('Ctrl Pts',(-1.91346599666502,226.635987203375,-4.44089209850063E-15));
#90472=CARTESIAN_POINT('Ctrl Pts',(-1.91346599666502,226.635987203375,-4.44089209850063E-15));
#90473=CARTESIAN_POINT('Ctrl Pts',(-1.97507207771062,226.578092614711,-4.89329144937181E-15));
#90474=CARTESIAN_POINT('Ctrl Pts',(-2.03330671663252,226.517047060303,-8.96290615499113E-15));
#90475=CARTESIAN_POINT('Ctrl Pts',(-2.0881732164084,226.453235441036,-9.04831765069503E-15));
#90476=CARTESIAN_POINT('Ctrl Pts',(-2.14449293498847,226.387733678504,-9.13599139371118E-15));
#90477=CARTESIAN_POINT('Ctrl Pts',(-2.1972641669798,226.3193169524,-4.39530143014281E-15));
#90478=CARTESIAN_POINT('Ctrl Pts',(-2.24646493105837,226.24835301163,-4.05231403988182E-15));
#90479=CARTESIAN_POINT('Ctrl Pts',(-2.29735461880039,226.174953078634,-3.69755285849117E-15));
#90480=CARTESIAN_POINT('Ctrl Pts',(-2.34442508449272,226.09882752961,-3.93155570548555E-15));
#90481=CARTESIAN_POINT('Ctrl Pts',(-2.38761709048648,226.020339322605,-4.27435864480685E-15));
#90482=CARTESIAN_POINT('Ctrl Pts',(-2.40651359310875,225.98600073204,-4.42433493075992E-15));
#90483=CARTESIAN_POINT('Ctrl Pts',(-2.42466724057222,225.951209407906,-7.20234639837333E-15));
#90484=CARTESIAN_POINT('Ctrl Pts',(-2.44207062867183,225.915993656427,-7.32747196252603E-15));
#90485=CARTESIAN_POINT('Ctrl Pts',(-2.45159445688031,225.896722192423,-7.39594566262734E-15));
#90486=CARTESIAN_POINT('Ctrl Pts',(-2.46089357651441,225.877323604807,-4.29996776038342E-15));
#90487=CARTESIAN_POINT('Ctrl Pts',(-2.46996656934727,225.857802403079,-4.38538094726937E-15));
#90488=CARTESIAN_POINT('Ctrl Pts',(-2.4786193151025,225.839185393399,-4.46683792666765E-15));
#90489=CARTESIAN_POINT('Ctrl Pts',(-2.48706888952069,225.820450858377,-5.8504930511398E-15));
#90490=CARTESIAN_POINT('Ctrl Pts',(-2.49529995223353,225.801635520385,-5.99520433297585E-15));
#90491=CARTESIAN_POINT('Ctrl Pts',(-2.53185235388015,225.718080599787,-6.6378364062587E-15));
#90492=CARTESIAN_POINT('Ctrl Pts',(-2.56414485209629,225.632842160853,-7.06865270289981E-15));
#90493=CARTESIAN_POINT('Ctrl Pts',(-2.5921533868293,225.546319206983,-7.91033905045424E-15));
#90494=CARTESIAN_POINT('Ctrl Pts',(-2.62062510855391,225.458365392588,-8.76594466122256E-15));
#90495=CARTESIAN_POINT('Ctrl Pts',(-2.64467049608575,225.369083471302,-1.42490890091117E-14));
#90496=CARTESIAN_POINT('Ctrl Pts',(-2.66422516627309,225.278855438708,-1.57374113740616E-14));
#90497=CARTESIAN_POINT('Ctrl Pts',(-2.6834344396825,225.190221116027,-1.71994453002682E-14));
#90498=CARTESIAN_POINT('Ctrl Pts',(-2.69831049024112,225.100672899581,-4.96279256628846E-15));
#90499=CARTESIAN_POINT('Ctrl Pts',(-2.70874964711037,225.010550082124,-3.58046925441613E-15));
#90500=CARTESIAN_POINT('Ctrl Pts',(-2.71288570289571,224.974842888027,-3.03278457040537E-15));
#90501=CARTESIAN_POINT('Ctrl Pts',(-2.71632476189001,224.939045312261,-1.00261591147195E-14));
#90502=CARTESIAN_POINT('Ctrl Pts',(-2.71905833761488,224.903177920343,-1.0019762797242E-14));
#90503=CARTESIAN_POINT('Ctrl Pts',(-2.72067831003024,224.88192217645,-1.00159722097785E-14));
#90504=CARTESIAN_POINT('Ctrl Pts',(-2.72205049483485,224.860641909081,-1.11437171572486E-14));
#90505=CARTESIAN_POINT('Ctrl Pts',(-2.72317292126621,224.839341375436,-1.16573417585641E-14));
#90506=CARTESIAN_POINT('Ctrl Pts',(-2.72391594666752,224.825240818715,-1.19973516824731E-14));
#90507=CARTESIAN_POINT('Ctrl Pts',(-2.72454944019077,224.811131472036,-1.79062259471769E-16));
#90508=CARTESIAN_POINT('Ctrl Pts',(-2.72507248770474,224.797028960929,-3.05311331771918E-16));
#90509=CARTESIAN_POINT('Ctrl Pts',(-2.72860269395363,224.701846837876,-1.15740459682122E-15));
#90510=CARTESIAN_POINT('Ctrl Pts',(-2.72711487623298,224.606814542,-1.19300801555276E-14));
#90511=CARTESIAN_POINT('Ctrl Pts',(-2.72055058832908,224.512331015797,-1.1740608485411E-14));
#90512=CARTESIAN_POINT('Ctrl Pts',(-2.71400847489059,224.418166659277,-1.15517768592805E-14));
#90513=CARTESIAN_POINT('Ctrl Pts',(-2.70242448973437,224.324546417287,-5.8005117148528E-15));
#90514=CARTESIAN_POINT('Ctrl Pts',(-2.6856927726943,224.231847303625,-5.05151476204446E-15));
#90515=CARTESIAN_POINT('Ctrl Pts',(-2.68378876806322,224.221298503326,-4.96628180816443E-15));
#90516=CARTESIAN_POINT('Ctrl Pts',(-2.68181804784731,224.210761621159,-1.04055797883408E-14));
#90517=CARTESIAN_POINT('Ctrl Pts',(-2.67978041320572,224.200237206572,-1.04083408558608E-14));
#90518=CARTESIAN_POINT('Ctrl Pts',(-2.66224980411456,224.109691338203,-1.04064054973758E-14));
#90519=CARTESIAN_POINT('Ctrl Pts',(-2.63977066177727,224.020067997417,-6.8127980350163E-15));
#90520=CARTESIAN_POINT('Ctrl Pts',(-2.61261810729545,223.931605005111,-6.07847105982273E-15));
#90521=CARTESIAN_POINT('Ctrl Pts',(-2.60191965458823,223.896749458088,-5.78913686767505E-15));
#90522=CARTESIAN_POINT('Ctrl Pts',(-2.59049509704381,223.862074101058,-7.49266670012035E-15));
#90523=CARTESIAN_POINT('Ctrl Pts',(-2.57835909838488,223.827593818547,-7.04991620636974E-15));
#90524=CARTESIAN_POINT('Ctrl Pts',(-2.57307244820024,223.812573613203,-6.85704646030921E-15));
#90525=CARTESIAN_POINT('Ctrl Pts',(-2.56765077825727,223.797590429269,-9.27411057059242E-15));
#90526=CARTESIAN_POINT('Ctrl Pts',(-2.562095232492,223.782645516012,-9.32587340685131E-15));
#90527=CARTESIAN_POINT('Ctrl Pts',(-2.55767628878723,223.7707581636,-9.36704615010494E-15));
#90528=CARTESIAN_POINT('Ctrl Pts',(-2.55317299678642,223.758896106066,-8.65625838009356E-15));
#90529=CARTESIAN_POINT('Ctrl Pts',(-2.5485897169222,223.747069278679,-8.60422844084496E-15));
#90530=CARTESIAN_POINT('Ctrl Pts',(-2.51484042770109,223.659981640598,-8.2211024874061E-15));
#90531=CARTESIAN_POINT('Ctrl Pts',(-2.4767077009188,223.574666891679,-1.01908969297783E-14));
#90532=CARTESIAN_POINT('Ctrl Pts',(-2.43452501819882,223.49135596505,-1.10744746706359E-14));
#90533=CARTESIAN_POINT('Ctrl Pts',(-2.39075748174647,223.404914947481,-1.19912494817165E-14));
#90534=CARTESIAN_POINT('Ctrl Pts',(-2.34262982770305,223.320630433717,-1.39073301009351E-14));
#90535=CARTESIAN_POINT('Ctrl Pts',(-2.29045846029114,223.23876337662,-1.66533453693773E-14));
#90536=CARTESIAN_POINT('Ctrl Pts',(-2.23768305960534,223.155948473434,-1.94311536437352E-14));
#90537=CARTESIAN_POINT('Ctrl Pts',(-2.1807693575821,223.075606513649,-1.23608385957802E-14));
#90538=CARTESIAN_POINT('Ctrl Pts',(-2.11999295375159,222.998022388435,-1.25177646026486E-14));
#90539=CARTESIAN_POINT('Ctrl Pts',(-2.07727773114182,222.94349426616,-1.26280562437161E-14));
#90540=CARTESIAN_POINT('Ctrl Pts',(-2.03265337236878,222.890328702756,-1.32724496364774E-14));
#90541=CARTESIAN_POINT('Ctrl Pts',(-1.98620222285849,222.838632264833,-1.29063426612674E-14));
#90542=CARTESIAN_POINT('Ctrl Pts',(-1.9748381431076,222.825984947176,-1.28167761186198E-14));
#90543=CARTESIAN_POINT('Ctrl Pts',(-1.96336393095075,222.813424902219,-1.62360964966543E-14));
#90544=CARTESIAN_POINT('Ctrl Pts',(-1.95179246873506,222.8009660948,-1.60427227058335E-14));
#90545=CARTESIAN_POINT('Ctrl Pts',(-1.8831185473061,222.727025987158,-1.48950944917225E-14));
#90546=CARTESIAN_POINT('Ctrl Pts',(-1.8109316641223,222.656546584352,-2.25517043828303E-15));
#90547=CARTESIAN_POINT('Ctrl Pts',(-1.735545247337,222.589815149064,-6.30745455865167E-15));
#90548=CARTESIAN_POINT('Ctrl Pts',(-1.67071550898282,222.532428398584,-9.7922802137621E-15));
#90549=CARTESIAN_POINT('Ctrl Pts',(-1.60351853762922,222.477813351873,-1.37421915177158E-14));
#90550=CARTESIAN_POINT('Ctrl Pts',(-1.5341274349756,222.426167995139,-1.41275879883551E-14));
#90551=CARTESIAN_POINT('Ctrl Pts',(-1.50861567308636,222.407180488193,-1.4269279683917E-14));
#90552=CARTESIAN_POINT('Ctrl Pts',(-1.4828071207238,222.388594557367,-1.78319144411338E-14));
#90553=CARTESIAN_POINT('Ctrl Pts',(-1.45670967205871,222.370420692607,-1.85407245112401E-14));
#90554=CARTESIAN_POINT('Ctrl Pts',(-1.43999809309774,222.358783004194,-1.89946131501996E-14));
#90555=CARTESIAN_POINT('Ctrl Pts',(-1.42316698931895,222.347313703686,-1.1605964273452E-14));
#90556=CARTESIAN_POINT('Ctrl Pts',(-1.40623326051012,222.336025220852,-1.15879528195251E-14));
#90557=CARTESIAN_POINT('Ctrl Pts',(-1.32003067627284,222.278560240554,-1.14962639840711E-14));
#90558=CARTESIAN_POINT('Ctrl Pts',(-1.2310870933596,222.225717965425,-7.07423916875325E-15));
#90559=CARTESIAN_POINT('Ctrl Pts',(-1.13970920235716,222.177818076848,-3.37230243729891E-15));
#90560=CARTESIAN_POINT('Ctrl Pts',(-1.04833131135472,222.129918188271,3.29634294155433E-16));
#90561=CARTESIAN_POINT('Ctrl Pts',(-0.954518472994722,222.086959783478,
-9.90042614199229E-16));
#90562=CARTESIAN_POINT('Ctrl Pts',(-0.858539567548663,222.049302996692,
1.81105130891979E-15));
#90563=CARTESIAN_POINT('Ctrl Pts',(-0.837654053215665,222.041108681946,
2.43149121055914E-15));
#90564=CARTESIAN_POINT('Ctrl Pts',(-0.816665849837719,222.033165591267,
1.08805921371938E-15));
#90565=CARTESIAN_POINT('Ctrl Pts',(-0.795579049799863,222.025472494795,
1.02695629777827E-15));
#90566=CARTESIAN_POINT('Ctrl Pts',(-2.51426753931457,225.001426524072,19.112583302492));
#90567=CARTESIAN_POINT('Ctrl Pts',(-2.51595717399498,225.327423730599,19.092036810933));
#90568=CARTESIAN_POINT('Ctrl Pts',(-2.45712149670304,225.65283607352,19.071490319374));
#90569=CARTESIAN_POINT('Ctrl Pts',(-2.33493158821761,225.952405376489,19.0509438278151));
#90570=CARTESIAN_POINT('Ctrl Pts',(-2.0202207778855,226.723972351672,18.9980245394045));
#90571=CARTESIAN_POINT('Ctrl Pts',(-1.28524008519825,227.324105609548,18.9451052509939));
#90572=CARTESIAN_POINT('Ctrl Pts',(-0.466331340144507,227.478200303444,
18.8921859625833));
#90573=CARTESIAN_POINT('Ctrl Pts',(0.352577404909238,227.632294997339,18.8392666741727));
#90574=CARTESIAN_POINT('Ctrl Pts',(1.25541420232948,227.340351127255,18.7863473857621));
#90575=CARTESIAN_POINT('Ctrl Pts',(1.82904817963972,226.735954264639,18.7334280973515));
#90576=CARTESIAN_POINT('Ctrl Pts',(2.40268215694995,226.131557402022,18.6805088089409));
#90577=CARTESIAN_POINT('Ctrl Pts',(2.64711331415017,225.214707546873,18.6275895205303));
#90578=CARTESIAN_POINT('Ctrl Pts',(2.45048639926028,224.40495908349,18.5746702321197));
#90579=CARTESIAN_POINT('Ctrl Pts',(2.25385948437039,223.595210620107,18.5217509437091));
#90580=CARTESIAN_POINT('Ctrl Pts',(1.61617449739038,222.892563548491,18.4688316552985));
#90581=CARTESIAN_POINT('Ctrl Pts',(0.829237828424323,222.618547230171,18.4159123668879));
#90582=CARTESIAN_POINT('Ctrl Pts',(0.0423011594582637,222.34453091185,18.3629930784773));
#90583=CARTESIAN_POINT('Ctrl Pts',(-0.893887191493852,222.499145346826,
18.3100737900667));
#90584=CARTESIAN_POINT('Ctrl Pts',(-1.55092831643626,223.011639920392,18.2571545016561));
#90585=CARTESIAN_POINT('Ctrl Pts',(-2.14925598476556,223.478337774746,18.2089641019347));
#90586=CARTESIAN_POINT('Ctrl Pts',(-2.51609677269774,224.24181291764,18.1607737022134));
#90587=CARTESIAN_POINT('Ctrl Pts',(-2.52086470301557,225.001296835693,18.112583302492));
#90588=CARTESIAN_POINT('Origin',(0.,225.,10.));
#90589=CARTESIAN_POINT('Origin',(160.,-225.,10.));
#90590=CARTESIAN_POINT('Origin',(-160.,-225.,10.));
#90591=CARTESIAN_POINT('Origin',(0.,-225.,10.));
#90592=CARTESIAN_POINT('Origin',(-160.,225.,10.));
#90593=CARTESIAN_POINT('Origin',(160.,225.,10.));
#90594=CARTESIAN_POINT('Origin',(325.,275.,0.));
#90595=CARTESIAN_POINT('',(325.,275.,0.));
#90596=CARTESIAN_POINT('',(-325.,275.,0.));
#90597=CARTESIAN_POINT('',(325.,275.,0.));
#90598=CARTESIAN_POINT('',(-325.,275.,0.));
#90599=CARTESIAN_POINT('',(325.,275.,0.));
#90600=CARTESIAN_POINT('Origin',(325.,-275.,0.));
#90601=CARTESIAN_POINT('',(325.,-275.,0.));
#90602=CARTESIAN_POINT('',(325.,-275.,0.));
#90603=CARTESIAN_POINT('',(325.,-275.,0.));
#90604=CARTESIAN_POINT('Origin',(-325.,-275.,0.));
#90605=CARTESIAN_POINT('',(-325.,-275.,0.));
#90606=CARTESIAN_POINT('',(-325.,-275.,0.));
#90607=CARTESIAN_POINT('',(-325.,-275.,0.));
#90608=CARTESIAN_POINT('Origin',(-325.,275.,0.));
#90609=CARTESIAN_POINT('',(-325.,275.,0.));
#90610=CARTESIAN_POINT('Origin',(0.,0.,0.));
#97448=UNCERTAINTY_MEASURE_WITH_UNIT(LENGTH_MEASURE(0.01),#97476,
'DISTANCE_ACCURACY_VALUE',
'Maximum model space distance between geometric entities at asserted c
onnectivities');
#97452=UNCERTAINTY_MEASURE_WITH_UNIT(LENGTH_MEASURE(0.01),#97476,
'DISTANCE_ACCURACY_VALUE',
'Maximum model space distance between geometric entities at asserted c
onnectivities');
#97471=(
GEOMETRIC_REPRESENTATION_CONTEXT(3)
GLOBAL_UNCERTAINTY_ASSIGNED_CONTEXT((#97448))
GLOBAL_UNIT_ASSIGNED_CONTEXT((#97476,#97478,#97479))
REPRESENTATION_CONTEXT('','3D')
);
#97475=(
GEOMETRIC_REPRESENTATION_CONTEXT(3)
GLOBAL_UNCERTAINTY_ASSIGNED_CONTEXT((#97452))
GLOBAL_UNIT_ASSIGNED_CONTEXT((#97476,#97478,#97479))
REPRESENTATION_CONTEXT('','3D')
);
#97476=(
LENGTH_UNIT()
NAMED_UNIT(*)
SI_UNIT(.MILLI.,.METRE.)
);
#97478=(
NAMED_UNIT(*)
PLANE_ANGLE_UNIT()
SI_UNIT($,.RADIAN.)
);
#97479=(
NAMED_UNIT(*)
SI_UNIT($,.STERADIAN.)
SOLID_ANGLE_UNIT()
);
#97498=SHAPE_DEFINITION_REPRESENTATION(#97560,#97621);
#97560=PRODUCT_DEFINITION_SHAPE('',$,#97644);
#97621=SHAPE_REPRESENTATION('',(#23042),#97471);
#97625=PRODUCT_DEFINITION_CONTEXT('part definition',#97693,'design');
#97644=PRODUCT_DEFINITION('Worktop','Worktop',#97666,#97625);
#97666=PRODUCT_DEFINITION_FORMATION('',$,#97713);
#97693=APPLICATION_CONTEXT(
'Core Data for Automotive Mechanical Design Process');
#97694=PRODUCT_CONTEXT('part definition',#97693,'mechanical');
#97713=PRODUCT('Worktop','Worktop',
'Aluminum fixture worktop. Six M6x1 through attachment holes; 650 x 55
0 x 20 mm stock.',(#97694));
#97721=PRESENTATION_STYLE_ASSIGNMENT((#97728));
#97728=SURFACE_STYLE_USAGE(.BOTH.,#97735);
#97735=SURFACE_SIDE_STYLE('',(#97742));
#97742=SURFACE_STYLE_FILL_AREA(#97749);
#97749=FILL_AREA_STYLE('Light gray',(#97756));
#97756=FILL_AREA_STYLE_COLOUR('Light gray',#97763);
#97763=COLOUR_RGB('Light gray',0.725490196078431,0.752941176470588,0.792156862745098);
ENDSEC;
END-ISO-10303-21;
